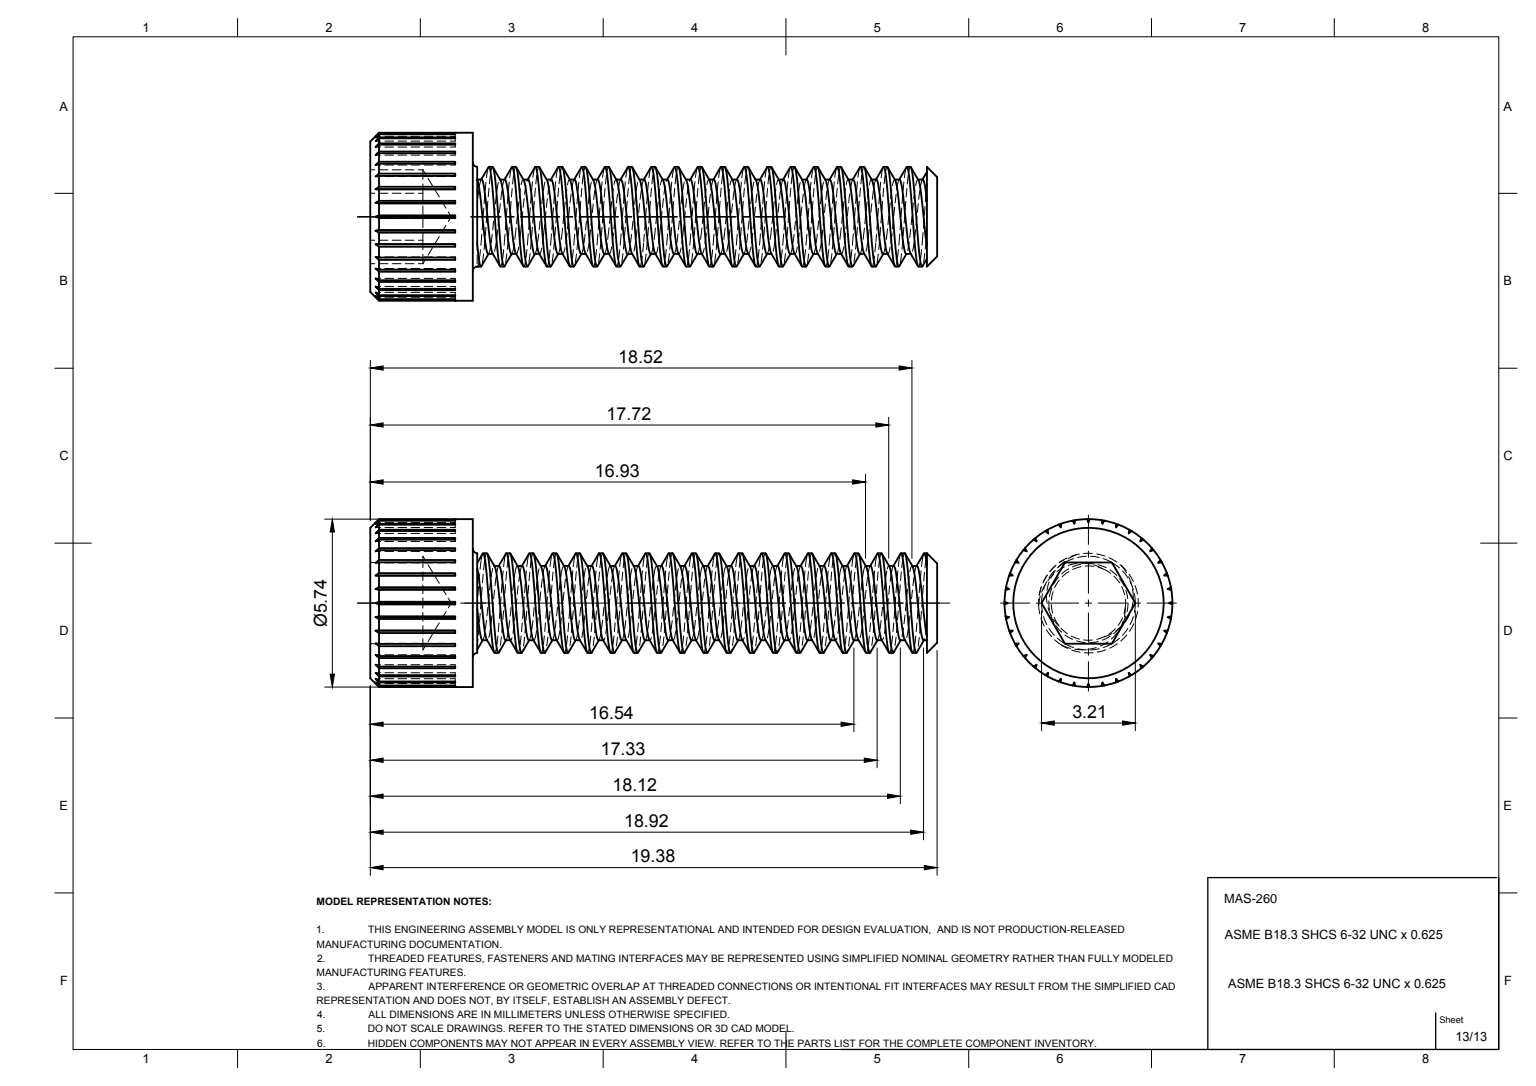
ISO-10303-21;
HEADER;
/* Generated by software containing ST-Developer
 * from STEP Tools, Inc. (www.steptools.com) 
 */

FILE_DESCRIPTION(
/* description */ (''),
/* implementation_level */ '2;1');

FILE_NAME(
/* name */ 'ASME B18.3 SHCS 6-32 UNC x 0.625.step',
/* time_stamp */ '2026-10-15T13:29:10-07:00',
/* author */ (''),
/* organization */ (''),
/* preprocessor_version */ 'ST-DEVELOPER v20.2',
/* originating_system */ 'Autodesk Translation Framework v15.15.0.0',
/* authorisation */ '');

FILE_SCHEMA (('AUTOMOTIVE_DESIGN { 1 0 10303 214 3 1 1 }'));
ENDSEC;

DATA;
#10=MECHANICAL_DESIGN_GEOMETRIC_PRESENTATION_REPRESENTATION('',(#944),#83219);
#425=(
BOUNDED_CURVE()
B_SPLINE_CURVE(2,(#82193,#82194,#82195),.UNSPECIFIED.,.F.,.F.)
B_SPLINE_CURVE_WITH_KNOTS((3,3),(0.,0.0169283274323949),.UNSPECIFIED.)
CURVE()
GEOMETRIC_REPRESENTATION_ITEM()
RATIONAL_B_SPLINE_CURVE((1.,1.00067437544385,1.00082963689528))
REPRESENTATION_ITEM('')
);
#426=(
BOUNDED_CURVE()
B_SPLINE_CURVE(2,(#82200,#82201,#82202),.UNSPECIFIED.,.F.,.F.)
B_SPLINE_CURVE_WITH_KNOTS((3,3),(0.027054491341878,0.0439828187741921),
 .UNSPECIFIED.)
CURVE()
GEOMETRIC_REPRESENTATION_ITEM()
RATIONAL_B_SPLINE_CURVE((1.00082963691689,1.00067437546141,1.))
REPRESENTATION_ITEM('')
);
#427=(
BOUNDED_CURVE()
B_SPLINE_CURVE(2,(#82209,#82210,#82211),.UNSPECIFIED.,.F.,.F.)
B_SPLINE_CURVE_WITH_KNOTS((3,3),(0.0270544913416899,0.0439828187741926),
 .UNSPECIFIED.)
CURVE()
GEOMETRIC_REPRESENTATION_ITEM()
RATIONAL_B_SPLINE_CURVE((1.00082963689398,1.0006743754428,1.))
REPRESENTATION_ITEM('')
);
#428=(
BOUNDED_CURVE()
B_SPLINE_CURVE(2,(#82215,#82216,#82217),.UNSPECIFIED.,.F.,.F.)
B_SPLINE_CURVE_WITH_KNOTS((3,3),(0.,0.016928327432378),.UNSPECIFIED.)
CURVE()
GEOMETRIC_REPRESENTATION_ITEM()
RATIONAL_B_SPLINE_CURVE((1.,1.00067437544454,1.00082963689613))
REPRESENTATION_ITEM('')
);
#429=(
BOUNDED_CURVE()
B_SPLINE_CURVE(2,(#82219,#82220,#82221),.UNSPECIFIED.,.F.,.F.)
B_SPLINE_CURVE_WITH_KNOTS((3,3),(0.0270544913417352,0.0439828187741927),
 .UNSPECIFIED.)
CURVE()
GEOMETRIC_REPRESENTATION_ITEM()
RATIONAL_B_SPLINE_CURVE((1.00082963690354,1.00067437545056,1.))
REPRESENTATION_ITEM('')
);
#430=(
BOUNDED_CURVE()
B_SPLINE_CURVE(2,(#82225,#82226,#82227),.UNSPECIFIED.,.F.,.F.)
B_SPLINE_CURVE_WITH_KNOTS((3,3),(0.,0.0169283274324875),.UNSPECIFIED.)
CURVE()
GEOMETRIC_REPRESENTATION_ITEM()
RATIONAL_B_SPLINE_CURVE((1.,1.00067437544421,1.00082963689573))
REPRESENTATION_ITEM('')
);
#431=(
BOUNDED_CURVE()
B_SPLINE_CURVE(2,(#82229,#82230,#82231),.UNSPECIFIED.,.F.,.F.)
B_SPLINE_CURVE_WITH_KNOTS((3,3),(0.0270544913417807,0.0439828187741914),
 .UNSPECIFIED.)
CURVE()
GEOMETRIC_REPRESENTATION_ITEM()
RATIONAL_B_SPLINE_CURVE((1.00082963690149,1.0006743754489,1.))
REPRESENTATION_ITEM('')
);
#432=(
BOUNDED_CURVE()
B_SPLINE_CURVE(2,(#82235,#82236,#82237),.UNSPECIFIED.,.F.,.F.)
B_SPLINE_CURVE_WITH_KNOTS((3,3),(0.,0.0169283274326477),.UNSPECIFIED.)
CURVE()
GEOMETRIC_REPRESENTATION_ITEM()
RATIONAL_B_SPLINE_CURVE((1.,1.00067437542316,1.00082963686982))
REPRESENTATION_ITEM('')
);
#433=(
BOUNDED_CURVE()
B_SPLINE_CURVE(2,(#82239,#82240,#82241),.UNSPECIFIED.,.F.,.F.)
B_SPLINE_CURVE_WITH_KNOTS((3,3),(0.0270544913419272,0.0439828187741907),
 .UNSPECIFIED.)
CURVE()
GEOMETRIC_REPRESENTATION_ITEM()
RATIONAL_B_SPLINE_CURVE((1.00082963692254,1.000674375466,1.))
REPRESENTATION_ITEM('')
);
#434=(
BOUNDED_CURVE()
B_SPLINE_CURVE(2,(#82245,#82246,#82247),.UNSPECIFIED.,.F.,.F.)
B_SPLINE_CURVE_WITH_KNOTS((3,3),(0.,0.0169283274324231),.UNSPECIFIED.)
CURVE()
GEOMETRIC_REPRESENTATION_ITEM()
RATIONAL_B_SPLINE_CURVE((1.,1.00067437544818,1.00082963690061))
REPRESENTATION_ITEM('')
);
#435=(
BOUNDED_CURVE()
B_SPLINE_CURVE(2,(#82249,#82250,#82251),.UNSPECIFIED.,.F.,.F.)
B_SPLINE_CURVE_WITH_KNOTS((3,3),(0.0270544913416623,0.0439828187741918),
 .UNSPECIFIED.)
CURVE()
GEOMETRIC_REPRESENTATION_ITEM()
RATIONAL_B_SPLINE_CURVE((1.00082963688688,1.00067437543703,1.))
REPRESENTATION_ITEM('')
);
#436=(
BOUNDED_CURVE()
B_SPLINE_CURVE(2,(#82255,#82256,#82257),.UNSPECIFIED.,.F.,.F.)
B_SPLINE_CURVE_WITH_KNOTS((3,3),(0.,0.016928327432524),.UNSPECIFIED.)
CURVE()
GEOMETRIC_REPRESENTATION_ITEM()
RATIONAL_B_SPLINE_CURVE((1.,1.00067437543311,1.00082963688207))
REPRESENTATION_ITEM('')
);
#437=(
BOUNDED_CURVE()
B_SPLINE_CURVE(2,(#82259,#82260,#82261),.UNSPECIFIED.,.F.,.F.)
B_SPLINE_CURVE_WITH_KNOTS((3,3),(0.0270544913417664,0.0439828187741907),
 .UNSPECIFIED.)
CURVE()
GEOMETRIC_REPRESENTATION_ITEM()
RATIONAL_B_SPLINE_CURVE((1.00082963689261,1.00067437544168,1.))
REPRESENTATION_ITEM('')
);
#438=(
BOUNDED_CURVE()
B_SPLINE_CURVE(2,(#82265,#82266,#82267),.UNSPECIFIED.,.F.,.F.)
B_SPLINE_CURVE_WITH_KNOTS((3,3),(0.,0.0169283274324059),.UNSPECIFIED.)
CURVE()
GEOMETRIC_REPRESENTATION_ITEM()
RATIONAL_B_SPLINE_CURVE((1.,1.00067437545304,1.00082963690658))
REPRESENTATION_ITEM('')
);
#439=(
BOUNDED_CURVE()
B_SPLINE_CURVE(2,(#82269,#82270,#82271),.UNSPECIFIED.,.F.,.F.)
B_SPLINE_CURVE_WITH_KNOTS((3,3),(0.0270544913417434,0.0439828187741902),
 .UNSPECIFIED.)
CURVE()
GEOMETRIC_REPRESENTATION_ITEM()
RATIONAL_B_SPLINE_CURVE((1.0008296368963,1.00067437544468,1.))
REPRESENTATION_ITEM('')
);
#440=(
BOUNDED_CURVE()
B_SPLINE_CURVE(2,(#82275,#82276,#82277),.UNSPECIFIED.,.F.,.F.)
B_SPLINE_CURVE_WITH_KNOTS((3,3),(0.,0.0169283274323925),.UNSPECIFIED.)
CURVE()
GEOMETRIC_REPRESENTATION_ITEM()
RATIONAL_B_SPLINE_CURVE((1.,1.00067437545304,1.00082963690659))
REPRESENTATION_ITEM('')
);
#441=(
BOUNDED_CURVE()
B_SPLINE_CURVE(2,(#82279,#82280,#82281),.UNSPECIFIED.,.F.,.F.)
B_SPLINE_CURVE_WITH_KNOTS((3,3),(0.0270544913417717,0.0439828187741908),
 .UNSPECIFIED.)
CURVE()
GEOMETRIC_REPRESENTATION_ITEM()
RATIONAL_B_SPLINE_CURVE((1.00082963689559,1.0006743754441,1.))
REPRESENTATION_ITEM('')
);
#442=(
BOUNDED_CURVE()
B_SPLINE_CURVE(2,(#82285,#82286,#82287),.UNSPECIFIED.,.F.,.F.)
B_SPLINE_CURVE_WITH_KNOTS((3,3),(0.,0.0169283274324336),.UNSPECIFIED.)
CURVE()
GEOMETRIC_REPRESENTATION_ITEM()
RATIONAL_B_SPLINE_CURVE((1.,1.00067437544179,1.00082963689274))
REPRESENTATION_ITEM('')
);
#443=(
BOUNDED_CURVE()
B_SPLINE_CURVE(2,(#82289,#82290,#82291),.UNSPECIFIED.,.F.,.F.)
B_SPLINE_CURVE_WITH_KNOTS((3,3),(0.0270544913417271,0.04398281877419),
 .UNSPECIFIED.)
CURVE()
GEOMETRIC_REPRESENTATION_ITEM()
RATIONAL_B_SPLINE_CURVE((1.00082963690167,1.00067437544904,1.))
REPRESENTATION_ITEM('')
);
#444=(
BOUNDED_CURVE()
B_SPLINE_CURVE(2,(#82295,#82296,#82297),.UNSPECIFIED.,.F.,.F.)
B_SPLINE_CURVE_WITH_KNOTS((3,3),(0.,0.0169283274323986),.UNSPECIFIED.)
CURVE()
GEOMETRIC_REPRESENTATION_ITEM()
RATIONAL_B_SPLINE_CURVE((1.,1.00067437544723,1.00082963689944))
REPRESENTATION_ITEM('')
);
#445=(
BOUNDED_CURVE()
B_SPLINE_CURVE(2,(#82299,#82300,#82301),.UNSPECIFIED.,.F.,.F.)
B_SPLINE_CURVE_WITH_KNOTS((3,3),(0.0270544913417658,0.0439828187741907),
 .UNSPECIFIED.)
CURVE()
GEOMETRIC_REPRESENTATION_ITEM()
RATIONAL_B_SPLINE_CURVE((1.00082963689458,1.00067437544328,1.))
REPRESENTATION_ITEM('')
);
#446=(
BOUNDED_CURVE()
B_SPLINE_CURVE(2,(#82305,#82306,#82307),.UNSPECIFIED.,.F.,.F.)
B_SPLINE_CURVE_WITH_KNOTS((3,3),(0.,0.0169283274323524),.UNSPECIFIED.)
CURVE()
GEOMETRIC_REPRESENTATION_ITEM()
RATIONAL_B_SPLINE_CURVE((1.,1.00067437545192,1.00082963690521))
REPRESENTATION_ITEM('')
);
#447=(
BOUNDED_CURVE()
B_SPLINE_CURVE(2,(#82309,#82310,#82311),.UNSPECIFIED.,.F.,.F.)
B_SPLINE_CURVE_WITH_KNOTS((3,3),(0.0270544913417437,0.0439828187741922),
 .UNSPECIFIED.)
CURVE()
GEOMETRIC_REPRESENTATION_ITEM()
RATIONAL_B_SPLINE_CURVE((1.0008296368979,1.00067437544598,1.))
REPRESENTATION_ITEM('')
);
#448=(
BOUNDED_CURVE()
B_SPLINE_CURVE(2,(#82315,#82316,#82317),.UNSPECIFIED.,.F.,.F.)
B_SPLINE_CURVE_WITH_KNOTS((3,3),(0.,0.0169283274322953),.UNSPECIFIED.)
CURVE()
GEOMETRIC_REPRESENTATION_ITEM()
RATIONAL_B_SPLINE_CURVE((1.,1.00067437546283,1.00082963691863))
REPRESENTATION_ITEM('')
);
#449=(
BOUNDED_CURVE()
B_SPLINE_CURVE(2,(#82319,#82320,#82321),.UNSPECIFIED.,.F.,.F.)
B_SPLINE_CURVE_WITH_KNOTS((3,3),(0.027054491341941,0.0439828187741898),
 .UNSPECIFIED.)
CURVE()
GEOMETRIC_REPRESENTATION_ITEM()
RATIONAL_B_SPLINE_CURVE((1.00082963692429,1.00067437546742,1.))
REPRESENTATION_ITEM('')
);
#450=(
BOUNDED_CURVE()
B_SPLINE_CURVE(2,(#82325,#82326,#82327),.UNSPECIFIED.,.F.,.F.)
B_SPLINE_CURVE_WITH_KNOTS((3,3),(0.,0.0169283274322328),.UNSPECIFIED.)
CURVE()
GEOMETRIC_REPRESENTATION_ITEM()
RATIONAL_B_SPLINE_CURVE((1.,1.00067437546617,1.00082963692274))
REPRESENTATION_ITEM('')
);
#451=(
BOUNDED_CURVE()
B_SPLINE_CURVE(2,(#82329,#82330,#82331),.UNSPECIFIED.,.F.,.F.)
B_SPLINE_CURVE_WITH_KNOTS((3,3),(0.0270544913418974,0.0439828187741896),
 .UNSPECIFIED.)
CURVE()
GEOMETRIC_REPRESENTATION_ITEM()
RATIONAL_B_SPLINE_CURVE((1.00082963691993,1.00067437546389,1.))
REPRESENTATION_ITEM('')
);
#452=(
BOUNDED_CURVE()
B_SPLINE_CURVE(2,(#82335,#82336,#82337),.UNSPECIFIED.,.F.,.F.)
B_SPLINE_CURVE_WITH_KNOTS((3,3),(0.,0.0169283274324175),.UNSPECIFIED.)
CURVE()
GEOMETRIC_REPRESENTATION_ITEM()
RATIONAL_B_SPLINE_CURVE((1.,1.00067437544813,1.00082963690054))
REPRESENTATION_ITEM('')
);
#453=(
BOUNDED_CURVE()
B_SPLINE_CURVE(2,(#82339,#82340,#82341),.UNSPECIFIED.,.F.,.F.)
B_SPLINE_CURVE_WITH_KNOTS((3,3),(0.0270544913419329,0.0439828187741885),
 .UNSPECIFIED.)
CURVE()
GEOMETRIC_REPRESENTATION_ITEM()
RATIONAL_B_SPLINE_CURVE((1.00082963691274,1.00067437545804,1.))
REPRESENTATION_ITEM('')
);
#454=(
BOUNDED_CURVE()
B_SPLINE_CURVE(2,(#82345,#82346,#82347),.UNSPECIFIED.,.F.,.F.)
B_SPLINE_CURVE_WITH_KNOTS((3,3),(0.,0.0169283274323868),.UNSPECIFIED.)
CURVE()
GEOMETRIC_REPRESENTATION_ITEM()
RATIONAL_B_SPLINE_CURVE((1.,1.00067437545154,1.00082963690474))
REPRESENTATION_ITEM('')
);
#455=(
BOUNDED_CURVE()
B_SPLINE_CURVE(2,(#82349,#82350,#82351),.UNSPECIFIED.,.F.,.F.)
B_SPLINE_CURVE_WITH_KNOTS((3,3),(0.0270544913418465,0.0439828187741911),
 .UNSPECIFIED.)
CURVE()
GEOMETRIC_REPRESENTATION_ITEM()
RATIONAL_B_SPLINE_CURVE((1.00082963692434,1.00067437546747,1.))
REPRESENTATION_ITEM('')
);
#456=(
BOUNDED_CURVE()
B_SPLINE_CURVE(2,(#82355,#82356,#82357),.UNSPECIFIED.,.F.,.F.)
B_SPLINE_CURVE_WITH_KNOTS((3,3),(0.,0.016928327432223),.UNSPECIFIED.)
CURVE()
GEOMETRIC_REPRESENTATION_ITEM()
RATIONAL_B_SPLINE_CURVE((1.,1.00067437546906,1.00082963692629))
REPRESENTATION_ITEM('')
);
#457=(
BOUNDED_CURVE()
B_SPLINE_CURVE(2,(#82359,#82360,#82361),.UNSPECIFIED.,.F.,.F.)
B_SPLINE_CURVE_WITH_KNOTS((3,3),(0.0270544913418792,0.0439828187741897),
 .UNSPECIFIED.)
CURVE()
GEOMETRIC_REPRESENTATION_ITEM()
RATIONAL_B_SPLINE_CURVE((1.0008296369223,1.00067437546581,1.))
REPRESENTATION_ITEM('')
);
#458=(
BOUNDED_CURVE()
B_SPLINE_CURVE(2,(#82365,#82366,#82367),.UNSPECIFIED.,.F.,.F.)
B_SPLINE_CURVE_WITH_KNOTS((3,3),(0.,0.0169283274325481),.UNSPECIFIED.)
CURVE()
GEOMETRIC_REPRESENTATION_ITEM()
RATIONAL_B_SPLINE_CURVE((1.,1.00067437544352,1.00082963689487))
REPRESENTATION_ITEM('')
);
#459=(
BOUNDED_CURVE()
B_SPLINE_CURVE(2,(#82369,#82370,#82371),.UNSPECIFIED.,.F.,.F.)
B_SPLINE_CURVE_WITH_KNOTS((3,3),(0.0270544913417793,0.0439828187741915),
 .UNSPECIFIED.)
CURVE()
GEOMETRIC_REPRESENTATION_ITEM()
RATIONAL_B_SPLINE_CURVE((1.00082963691087,1.00067437545653,1.))
REPRESENTATION_ITEM('')
);
#460=(
BOUNDED_CURVE()
B_SPLINE_CURVE(2,(#82375,#82376,#82377),.UNSPECIFIED.,.F.,.F.)
B_SPLINE_CURVE_WITH_KNOTS((3,3),(0.,0.0169283274323758),.UNSPECIFIED.)
CURVE()
GEOMETRIC_REPRESENTATION_ITEM()
RATIONAL_B_SPLINE_CURVE((1.,1.00067437544934,1.00082963690204))
REPRESENTATION_ITEM('')
);
#461=(
BOUNDED_CURVE()
B_SPLINE_CURVE(2,(#82379,#82380,#82381),.UNSPECIFIED.,.F.,.F.)
B_SPLINE_CURVE_WITH_KNOTS((3,3),(0.0270544913417685,0.0439828187741897),
 .UNSPECIFIED.)
CURVE()
GEOMETRIC_REPRESENTATION_ITEM()
RATIONAL_B_SPLINE_CURVE((1.00082963689898,1.00067437544686,1.))
REPRESENTATION_ITEM('')
);
#462=(
BOUNDED_CURVE()
B_SPLINE_CURVE(2,(#82385,#82386,#82387),.UNSPECIFIED.,.F.,.F.)
B_SPLINE_CURVE_WITH_KNOTS((3,3),(0.,0.0169283274324469),.UNSPECIFIED.)
CURVE()
GEOMETRIC_REPRESENTATION_ITEM()
RATIONAL_B_SPLINE_CURVE((1.,1.00067437544897,1.00082963690158))
REPRESENTATION_ITEM('')
);
#463=(
BOUNDED_CURVE()
B_SPLINE_CURVE(2,(#82389,#82390,#82391),.UNSPECIFIED.,.F.,.F.)
B_SPLINE_CURVE_WITH_KNOTS((3,3),(0.0270544913418427,0.04398281877419),
 .UNSPECIFIED.)
CURVE()
GEOMETRIC_REPRESENTATION_ITEM()
RATIONAL_B_SPLINE_CURVE((1.00082963692428,1.00067437546742,1.))
REPRESENTATION_ITEM('')
);
#464=(
BOUNDED_CURVE()
B_SPLINE_CURVE(2,(#82396,#82397,#82398),.UNSPECIFIED.,.F.,.F.)
B_SPLINE_CURVE_WITH_KNOTS((3,3),(0.,0.0169283274326309),.UNSPECIFIED.)
CURVE()
GEOMETRIC_REPRESENTATION_ITEM()
RATIONAL_B_SPLINE_CURVE((1.,1.00067437542865,1.00082963687657))
REPRESENTATION_ITEM('')
);
#465=(
BOUNDED_CURVE()
B_SPLINE_CURVE(2,(#82400,#82401,#82402),.UNSPECIFIED.,.F.,.F.)
B_SPLINE_CURVE_WITH_KNOTS((3,3),(0.0270544913417494,0.0439828187741933),
 .UNSPECIFIED.)
CURVE()
GEOMETRIC_REPRESENTATION_ITEM()
RATIONAL_B_SPLINE_CURVE((1.00082963689727,1.00067437544547,1.))
REPRESENTATION_ITEM('')
);
#466=(
BOUNDED_CURVE()
B_SPLINE_CURVE(2,(#82406,#82407,#82408),.UNSPECIFIED.,.F.,.F.)
B_SPLINE_CURVE_WITH_KNOTS((3,3),(0.,0.0169283274321813),.UNSPECIFIED.)
CURVE()
GEOMETRIC_REPRESENTATION_ITEM()
RATIONAL_B_SPLINE_CURVE((1.,1.00067437546612,1.00082963692269))
REPRESENTATION_ITEM('')
);
#467=(
BOUNDED_CURVE()
B_SPLINE_CURVE(2,(#82410,#82411,#82412),.UNSPECIFIED.,.F.,.F.)
B_SPLINE_CURVE_WITH_KNOTS((3,3),(0.0270544913418634,0.0439828187741926),
 .UNSPECIFIED.)
CURVE()
GEOMETRIC_REPRESENTATION_ITEM()
RATIONAL_B_SPLINE_CURVE((1.00082963691427,1.00067437545928,1.))
REPRESENTATION_ITEM('')
);
#468=(
BOUNDED_CURVE()
B_SPLINE_CURVE(2,(#82416,#82417,#82418),.UNSPECIFIED.,.F.,.F.)
B_SPLINE_CURVE_WITH_KNOTS((3,3),(0.,0.0169283274324664),.UNSPECIFIED.)
CURVE()
GEOMETRIC_REPRESENTATION_ITEM()
RATIONAL_B_SPLINE_CURVE((1.,1.00067437544028,1.00082963689088))
REPRESENTATION_ITEM('')
);
#469=(
BOUNDED_CURVE()
B_SPLINE_CURVE(2,(#82420,#82421,#82422),.UNSPECIFIED.,.F.,.F.)
B_SPLINE_CURVE_WITH_KNOTS((3,3),(0.0270544913418777,0.0439828187741926),
 .UNSPECIFIED.)
CURVE()
GEOMETRIC_REPRESENTATION_ITEM()
RATIONAL_B_SPLINE_CURVE((1.00082963691853,1.00067437546274,1.))
REPRESENTATION_ITEM('')
);
#470=(
BOUNDED_CURVE()
B_SPLINE_CURVE(2,(#82426,#82427,#82428),.UNSPECIFIED.,.F.,.F.)
B_SPLINE_CURVE_WITH_KNOTS((3,3),(0.,0.0169283274323108),.UNSPECIFIED.)
CURVE()
GEOMETRIC_REPRESENTATION_ITEM()
RATIONAL_B_SPLINE_CURVE((1.,1.00067437545943,1.00082963691444))
REPRESENTATION_ITEM('')
);
#471=(
BOUNDED_CURVE()
B_SPLINE_CURVE(2,(#82430,#82431,#82432),.UNSPECIFIED.,.F.,.F.)
B_SPLINE_CURVE_WITH_KNOTS((3,3),(0.0270544913417395,0.0439828187741916),
 .UNSPECIFIED.)
CURVE()
GEOMETRIC_REPRESENTATION_ITEM()
RATIONAL_B_SPLINE_CURVE((1.00082963689027,1.00067437543978,1.))
REPRESENTATION_ITEM('')
);
#472=(
BOUNDED_CURVE()
B_SPLINE_CURVE(2,(#82436,#82437,#82438),.UNSPECIFIED.,.F.,.F.)
B_SPLINE_CURVE_WITH_KNOTS((3,3),(0.,0.0169283274323638),.UNSPECIFIED.)
CURVE()
GEOMETRIC_REPRESENTATION_ITEM()
RATIONAL_B_SPLINE_CURVE((1.,1.00067437545187,1.00082963690515))
REPRESENTATION_ITEM('')
);
#473=(
BOUNDED_CURVE()
B_SPLINE_CURVE(2,(#82440,#82441,#82442),.UNSPECIFIED.,.F.,.F.)
B_SPLINE_CURVE_WITH_KNOTS((3,3),(0.0270544913417076,0.0439828187741916),
 .UNSPECIFIED.)
CURVE()
GEOMETRIC_REPRESENTATION_ITEM()
RATIONAL_B_SPLINE_CURVE((1.00082963689143,1.00067437544072,1.))
REPRESENTATION_ITEM('')
);
#474=(
BOUNDED_CURVE()
B_SPLINE_CURVE(2,(#82446,#82447,#82448),.UNSPECIFIED.,.F.,.F.)
B_SPLINE_CURVE_WITH_KNOTS((3,3),(0.,0.0169283274324132),.UNSPECIFIED.)
CURVE()
GEOMETRIC_REPRESENTATION_ITEM()
RATIONAL_B_SPLINE_CURVE((1.,1.00067437545166,1.00082963690489))
REPRESENTATION_ITEM('')
);
#475=(
BOUNDED_CURVE()
B_SPLINE_CURVE(2,(#82450,#82451,#82452),.UNSPECIFIED.,.F.,.F.)
B_SPLINE_CURVE_WITH_KNOTS((3,3),(0.0270544913417581,0.0439828187741926),
 .UNSPECIFIED.)
CURVE()
GEOMETRIC_REPRESENTATION_ITEM()
RATIONAL_B_SPLINE_CURVE((1.00082963689712,1.00067437544534,1.))
REPRESENTATION_ITEM('')
);
#476=(
BOUNDED_CURVE()
B_SPLINE_CURVE(2,(#82456,#82457,#82458),.UNSPECIFIED.,.F.,.F.)
B_SPLINE_CURVE_WITH_KNOTS((3,3),(0.,0.0169283274323258),.UNSPECIFIED.)
CURVE()
GEOMETRIC_REPRESENTATION_ITEM()
RATIONAL_B_SPLINE_CURVE((1.,1.00067437545421,1.00082963690803))
REPRESENTATION_ITEM('')
);
#477=(
BOUNDED_CURVE()
B_SPLINE_CURVE(2,(#82460,#82461,#82462),.UNSPECIFIED.,.F.,.F.)
B_SPLINE_CURVE_WITH_KNOTS((3,3),(0.0270544913417721,0.0439828187741926),
 .UNSPECIFIED.)
CURVE()
GEOMETRIC_REPRESENTATION_ITEM()
RATIONAL_B_SPLINE_CURVE((1.00082963689922,1.00067437544705,1.))
REPRESENTATION_ITEM('')
);
#478=(
BOUNDED_CURVE()
B_SPLINE_CURVE(2,(#82466,#82467,#82468),.UNSPECIFIED.,.F.,.F.)
B_SPLINE_CURVE_WITH_KNOTS((3,3),(0.,0.0169283274323368),.UNSPECIFIED.)
CURVE()
GEOMETRIC_REPRESENTATION_ITEM()
RATIONAL_B_SPLINE_CURVE((1.,1.00067437545165,1.00082963690488))
REPRESENTATION_ITEM('')
);
#479=(
BOUNDED_CURVE()
B_SPLINE_CURVE(2,(#82470,#82471,#82472),.UNSPECIFIED.,.F.,.F.)
B_SPLINE_CURVE_WITH_KNOTS((3,3),(0.0270544913418129,0.0439828187741918),
 .UNSPECIFIED.)
CURVE()
GEOMETRIC_REPRESENTATION_ITEM()
RATIONAL_B_SPLINE_CURVE((1.00082963690488,1.00067437545165,1.))
REPRESENTATION_ITEM('')
);
#480=(
BOUNDED_CURVE()
B_SPLINE_CURVE(2,(#82476,#82477,#82478),.UNSPECIFIED.,.F.,.F.)
B_SPLINE_CURVE_WITH_KNOTS((3,3),(0.,0.0169283274323829),.UNSPECIFIED.)
CURVE()
GEOMETRIC_REPRESENTATION_ITEM()
RATIONAL_B_SPLINE_CURVE((1.,1.00067437545407,1.00082963690785))
REPRESENTATION_ITEM('')
);
#481=(
BOUNDED_CURVE()
B_SPLINE_CURVE(2,(#82480,#82481,#82482),.UNSPECIFIED.,.F.,.F.)
B_SPLINE_CURVE_WITH_KNOTS((3,3),(0.0270544913418384,0.0439828187741921),
 .UNSPECIFIED.)
CURVE()
GEOMETRIC_REPRESENTATION_ITEM()
RATIONAL_B_SPLINE_CURVE((1.00082963690821,1.00067437545436,1.))
REPRESENTATION_ITEM('')
);
#482=(
BOUNDED_CURVE()
B_SPLINE_CURVE(2,(#82486,#82487,#82488),.UNSPECIFIED.,.F.,.F.)
B_SPLINE_CURVE_WITH_KNOTS((3,3),(0.,0.0169283274323058),.UNSPECIFIED.)
CURVE()
GEOMETRIC_REPRESENTATION_ITEM()
RATIONAL_B_SPLINE_CURVE((1.,1.00067437546416,1.00082963692027))
REPRESENTATION_ITEM('')
);
#483=(
BOUNDED_CURVE()
B_SPLINE_CURVE(2,(#82490,#82491,#82492),.UNSPECIFIED.,.F.,.F.)
B_SPLINE_CURVE_WITH_KNOTS((3,3),(0.0270544913418702,0.0439828187741907),
 .UNSPECIFIED.)
CURVE()
GEOMETRIC_REPRESENTATION_ITEM()
RATIONAL_B_SPLINE_CURVE((1.00082963692018,1.00067437546409,1.))
REPRESENTATION_ITEM('')
);
#484=(
BOUNDED_CURVE()
B_SPLINE_CURVE(2,(#82496,#82497,#82498),.UNSPECIFIED.,.F.,.F.)
B_SPLINE_CURVE_WITH_KNOTS((3,3),(0.,0.0169283274324372),.UNSPECIFIED.)
CURVE()
GEOMETRIC_REPRESENTATION_ITEM()
RATIONAL_B_SPLINE_CURVE((1.,1.00067437545102,1.0008296369041))
REPRESENTATION_ITEM('')
);
#485=(
BOUNDED_CURVE()
B_SPLINE_CURVE(2,(#82500,#82501,#82502),.UNSPECIFIED.,.F.,.F.)
B_SPLINE_CURVE_WITH_KNOTS((3,3),(0.0270544913418863,0.0439828187741916),
 .UNSPECIFIED.)
CURVE()
GEOMETRIC_REPRESENTATION_ITEM()
RATIONAL_B_SPLINE_CURVE((1.00082963691192,1.00067437545738,1.))
REPRESENTATION_ITEM('')
);
#486=(
BOUNDED_CURVE()
B_SPLINE_CURVE(2,(#82506,#82507,#82508),.UNSPECIFIED.,.F.,.F.)
B_SPLINE_CURVE_WITH_KNOTS((3,3),(0.,0.0169283274323833),.UNSPECIFIED.)
CURVE()
GEOMETRIC_REPRESENTATION_ITEM()
RATIONAL_B_SPLINE_CURVE((1.,1.00067437544615,1.00082963689811))
REPRESENTATION_ITEM('')
);
#487=(
BOUNDED_CURVE()
B_SPLINE_CURVE(2,(#82510,#82511,#82512),.UNSPECIFIED.,.F.,.F.)
B_SPLINE_CURVE_WITH_KNOTS((3,3),(0.0270544913417211,0.0439828187741927),
 .UNSPECIFIED.)
CURVE()
GEOMETRIC_REPRESENTATION_ITEM()
RATIONAL_B_SPLINE_CURVE((1.00082963690189,1.00067437544923,1.))
REPRESENTATION_ITEM('')
);
#488=(
BOUNDED_CURVE()
B_SPLINE_CURVE(2,(#82516,#82517,#82518),.UNSPECIFIED.,.F.,.F.)
B_SPLINE_CURVE_WITH_KNOTS((3,3),(0.,0.0169283274324049),.UNSPECIFIED.)
CURVE()
GEOMETRIC_REPRESENTATION_ITEM()
RATIONAL_B_SPLINE_CURVE((1.,1.00067437545222,1.00082963690557))
REPRESENTATION_ITEM('')
);
#489=(
BOUNDED_CURVE()
B_SPLINE_CURVE(2,(#82520,#82521,#82522),.UNSPECIFIED.,.F.,.F.)
B_SPLINE_CURVE_WITH_KNOTS((3,3),(0.0270544913418404,0.0439828187741917),
 .UNSPECIFIED.)
CURVE()
GEOMETRIC_REPRESENTATION_ITEM()
RATIONAL_B_SPLINE_CURVE((1.00082963691628,1.00067437546092,1.))
REPRESENTATION_ITEM('')
);
#490=(
BOUNDED_CURVE()
B_SPLINE_CURVE(2,(#82526,#82527,#82528),.UNSPECIFIED.,.F.,.F.)
B_SPLINE_CURVE_WITH_KNOTS((3,3),(0.,0.016928327432346),.UNSPECIFIED.)
CURVE()
GEOMETRIC_REPRESENTATION_ITEM()
RATIONAL_B_SPLINE_CURVE((1.,1.00067437545423,1.00082963690805))
REPRESENTATION_ITEM('')
);
#491=(
BOUNDED_CURVE()
B_SPLINE_CURVE(2,(#82530,#82531,#82532),.UNSPECIFIED.,.F.,.F.)
B_SPLINE_CURVE_WITH_KNOTS((3,3),(0.0270544913418446,0.0439828187741916),
 .UNSPECIFIED.)
CURVE()
GEOMETRIC_REPRESENTATION_ITEM()
RATIONAL_B_SPLINE_CURVE((1.00082963690992,1.00067437545575,1.))
REPRESENTATION_ITEM('')
);
#492=(
BOUNDED_CURVE()
B_SPLINE_CURVE(2,(#82536,#82537,#82538),.UNSPECIFIED.,.F.,.F.)
B_SPLINE_CURVE_WITH_KNOTS((3,3),(0.,0.0169283274324851),.UNSPECIFIED.)
CURVE()
GEOMETRIC_REPRESENTATION_ITEM()
RATIONAL_B_SPLINE_CURVE((1.,1.00067437545061,1.00082963690359))
REPRESENTATION_ITEM('')
);
#493=(
BOUNDED_CURVE()
B_SPLINE_CURVE(2,(#82540,#82541,#82542),.UNSPECIFIED.,.F.,.F.)
B_SPLINE_CURVE_WITH_KNOTS((3,3),(0.0270544913417195,0.0439828187741921),
 .UNSPECIFIED.)
CURVE()
GEOMETRIC_REPRESENTATION_ITEM()
RATIONAL_B_SPLINE_CURVE((1.00082963689352,1.00067437544242,1.))
REPRESENTATION_ITEM('')
);
#494=(
BOUNDED_CURVE()
B_SPLINE_CURVE(2,(#82546,#82547,#82548),.UNSPECIFIED.,.F.,.F.)
B_SPLINE_CURVE_WITH_KNOTS((3,3),(0.,0.0169283274324387),.UNSPECIFIED.)
CURVE()
GEOMETRIC_REPRESENTATION_ITEM()
RATIONAL_B_SPLINE_CURVE((1.,1.00067437545353,1.00082963690719))
REPRESENTATION_ITEM('')
);
#495=(
BOUNDED_CURVE()
B_SPLINE_CURVE(2,(#82550,#82551,#82552),.UNSPECIFIED.,.F.,.F.)
B_SPLINE_CURVE_WITH_KNOTS((3,3),(0.0270544913416745,0.0439828187741916),
 .UNSPECIFIED.)
CURVE()
GEOMETRIC_REPRESENTATION_ITEM()
RATIONAL_B_SPLINE_CURVE((1.00082963688426,1.00067437543489,1.))
REPRESENTATION_ITEM('')
);
#496=(
BOUNDED_CURVE()
B_SPLINE_CURVE(2,(#82555,#82556,#82557),.UNSPECIFIED.,.F.,.F.)
B_SPLINE_CURVE_WITH_KNOTS((3,3),(0.,0.0169283274326045),.UNSPECIFIED.)
CURVE()
GEOMETRIC_REPRESENTATION_ITEM()
RATIONAL_B_SPLINE_CURVE((1.,1.0006743754289,1.00082963687688))
REPRESENTATION_ITEM('')
);
#507=TOROIDAL_SURFACE('',#28959,1.85434,0.15);
#754=B_SPLINE_CURVE_WITH_KNOTS('',3,(#66842,#66843,#66844,#66845,#66846,
#66847,#66848,#66849,#66850,#66851,#66852,#66853,#66854,#66855,#66856,#66857,
#66858,#66859,#66860,#66861,#66862,#66863,#66864,#66865,#66866,#66867,#66868,
#66869,#66870,#66871,#66872,#66873,#66874,#66875,#66876,#66877,#66878,#66879,
#66880,#66881,#66882,#66883,#66884,#66885,#66886,#66887,#66888,#66889,#66890,
#66891,#66892,#66893,#66894,#66895,#66896,#66897,#66898,#66899,#66900,#66901,
#66902,#66903,#66904,#66905,#66906,#66907,#66908,#66909,#66910,#66911,#66912,
#66913,#66914,#66915,#66916,#66917,#66918,#66919,#66920,#66921,#66922,#66923,
#66924,#66925,#66926,#66927,#66928,#66929,#66930,#66931,#66932,#66933,#66934,
#66935,#66936,#66937,#66938,#66939,#66940,#66941,#66942,#66943,#66944,#66945,
#66946,#66947,#66948,#66949,#66950,#66951,#66952,#66953,#66954,#66955,#66956,
#66957,#66958,#66959,#66960,#66961,#66962,#66963,#66964,#66965,#66966,#66967,
#66968,#66969,#66970,#66971,#66972,#66973,#66974,#66975,#66976,#66977,#66978,
#66979,#66980,#66981,#66982,#66983,#66984,#66985,#66986,#66987,#66988,#66989,
#66990,#66991),.UNSPECIFIED.,.F.,.F.,(4,2,2,2,2,2,2,2,2,2,2,2,2,2,2,2,2,
2,2,2,2,2,2,2,2,2,2,2,2,2,2,2,2,2,2,2,2,2,2,2,2,2,2,2,2,2,2,2,2,2,2,2,2,
2,2,2,2,2,2,2,2,2,2,2,2,2,2,2,2,2,2,2,2,2,4),(-0.57814561136758,-0.576296413092534,
-0.573641255529324,-0.570575982215014,-0.565100054282956,-0.539917695991999,
-0.517394447378374,-0.513602331908594,-0.511741570723418,-0.510242310430281,
-0.508340948528616,-0.504346832441546,-0.498825097755031,-0.482729724369596,
-0.457683189040658,-0.452468380911234,-0.449158815326736,-0.44649911229893,
-0.443438658618413,-0.437998831205895,-0.420540876202223,-0.396348568164452,
-0.388039555375418,-0.385470635862254,-0.383865857222333,-0.382305956175603,
-0.379915741966088,-0.372455557398866,-0.358639298966442,-0.329684380929608,
-0.324675436110595,-0.321438891082664,-0.31880269342991,-0.315730719856977,
-0.310163725739934,-0.291420708773143,-0.262555131157506,-0.258796386401061,
-0.256948163636404,-0.25545280771485,-0.253551211796978,-0.249556076524077,
-0.244035210720099,-0.227979871153349,-0.202571226003975,-0.197332498520712,
-0.194009001551785,-0.191338924841252,-0.188267212494532,-0.182807842087583,
-0.165030475351221,-0.139231601339638,-0.132653249078248,-0.130320744596009,
-0.1288153480515,-0.127227747985358,-0.124700541689401,-0.116313972219858,
-0.0993334415849082,-0.0765628114683407,-0.0713569283432376,-0.0680324326380281,
-0.0653451663167553,-0.0622341911963431,-0.0566479026914896,-0.0370860220512205,
-0.017582256991236,-0.0174599552727001,-0.0173504481393084,-0.0172524828413307,
-0.0117389265183658,-0.00594267422071392,-0.00373663500168019,-0.00222440479797267,
-0.00170432960837967),.UNSPECIFIED.);
#755=B_SPLINE_CURVE_WITH_KNOTS('',3,(#66994,#66995,#66996,#66997,#66998,
#66999,#67000,#67001,#67002,#67003,#67004,#67005,#67006,#67007,#67008,#67009,
#67010,#67011,#67012,#67013,#67014,#67015,#67016,#67017,#67018,#67019,#67020,
#67021,#67022,#67023,#67024,#67025,#67026,#67027,#67028,#67029,#67030,#67031,
#67032,#67033,#67034,#67035,#67036,#67037,#67038,#67039,#67040,#67041,#67042,
#67043,#67044,#67045,#67046,#67047,#67048,#67049,#67050,#67051,#67052,#67053,
#67054,#67055,#67056,#67057,#67058,#67059,#67060,#67061,#67062,#67063,#67064,
#67065,#67066,#67067,#67068,#67069,#67070,#67071,#67072,#67073,#67074,#67075,
#67076,#67077,#67078,#67079,#67080,#67081,#67082,#67083,#67084,#67085,#67086,
#67087,#67088,#67089,#67090,#67091,#67092,#67093,#67094,#67095),
 .UNSPECIFIED.,.F.,.F.,(4,2,2,2,2,2,2,2,2,2,2,2,2,2,2,2,2,2,2,2,2,2,2,2,
2,2,2,2,2,2,2,2,2,2,2,2,2,2,2,2,2,2,2,2,2,2,2,2,2,2,4),(-1.318649661076,
-1.31743164617652,-1.31596386436676,-1.31264394085227,-1.29594709662516,
-1.28122934432088,-1.26838464214962,-1.26496788072465,-1.26168833677219,
-1.25870792832702,-1.25486579200619,-1.24618731091111,-1.21648393904188,
-1.20318656193115,-1.19816844726018,-1.19454224790336,-1.19301372216914,
-1.19149228574573,-1.1898443744577,-1.18691776961928,-1.17008318442145,
-1.14747114229976,-1.1394250167213,-1.13330473980141,-1.13019933198268,
-1.12766982200797,-1.12472587504508,-1.11956287795595,-1.08684999296772,
-1.0740249365971,-1.0669291365151,-1.06464970615256,-1.0631437366511,-1.06174272516908,
-1.05978387397002,-1.05448060749719,-1.02076562574725,-1.00652926771878,
-1.00219769891924,-0.999348512279982,-0.996615935546906,-0.992744443746673,
-0.983330401145941,-0.952120651371644,-0.941214068805748,-0.938480088912673,
-0.936816205379131,-0.935259751531581,-0.932908357310751,-0.926522568567024,
-0.912197827138135),.UNSPECIFIED.);
#756=B_SPLINE_CURVE_WITH_KNOTS('',3,(#67100,#67101,#67102,#67103,#67104,
#67105,#67106,#67107,#67108,#67109,#67110,#67111,#67112,#67113,#67114,#67115,
#67116,#67117,#67118,#67119,#67120,#67121,#67122,#67123,#67124,#67125,#67126,
#67127,#67128,#67129,#67130,#67131,#67132,#67133,#67134,#67135,#67136,#67137,
#67138,#67139,#67140,#67141,#67142,#67143,#67144,#67145,#67146,#67147,#67148,
#67149,#67150,#67151,#67152,#67153,#67154,#67155,#67156,#67157,#67158,#67159,
#67160,#67161,#67162,#67163,#67164,#67165,#67166,#67167,#67168,#67169,#67170,
#67171,#67172,#67173,#67174,#67175,#67176,#67177,#67178,#67179,#67180,#67181,
#67182,#67183,#67184,#67185,#67186,#67187,#67188,#67189,#67190,#67191,#67192,
#67193,#67194,#67195,#67196,#67197,#67198,#67199,#67200,#67201,#67202,#67203,
#67204,#67205,#67206,#67207,#67208,#67209,#67210,#67211,#67212,#67213,#67214,
#67215,#67216,#67217,#67218,#67219,#67220,#67221,#67222,#67223,#67224,#67225,
#67226,#67227,#67228,#67229,#67230,#67231,#67232,#67233,#67234,#67235,#67236,
#67237,#67238,#67239,#67240,#67241,#67242,#67243,#67244,#67245,#67246,#67247,
#67248,#67249,#67250,#67251,#67252,#67253,#67254,#67255,#67256,#67257,#67258,
#67259,#67260,#67261,#67262,#67263,#67264,#67265,#67266,#67267,#67268,#67269,
#67270,#67271,#67272,#67273,#67274,#67275,#67276,#67277,#67278,#67279,#67280,
#67281,#67282,#67283,#67284,#67285,#67286,#67287,#67288,#67289,#67290,#67291,
#67292,#67293,#67294,#67295,#67296,#67297,#67298,#67299,#67300,#67301,#67302,
#67303,#67304,#67305,#67306,#67307,#67308,#67309,#67310,#67311),
 .UNSPECIFIED.,.F.,.F.,(4,2,2,2,2,2,2,2,2,2,2,2,2,2,2,2,2,2,2,2,2,2,2,2,
2,2,2,2,2,2,2,2,2,2,2,2,2,2,2,2,2,2,2,2,2,2,2,2,2,2,2,2,2,2,2,2,2,2,2,2,
2,2,2,2,2,2,2,2,2,2,2,2,2,2,2,2,2,2,2,2,2,2,2,2,2,2,2,2,2,2,2,2,2,2,2,2,
2,2,2,2,2,2,2,2,2,4),(-1.38023582942697,-1.36727393991216,-1.35371560626455,
-1.34758612233084,-1.343921800107,-1.34061316589332,-1.34053112229902,-1.34043931642608,
-1.3403365203079,-1.34022134355601,-1.34016271070482,-1.34005242700723,
-1.3398468093432,-1.33815809251505,-1.3352377643514,-1.33045180817441,-1.30897662302457,
-1.29157501945926,-1.28356639925018,-1.27834115990851,-1.27623369214961,
-1.27471833837372,-1.2730058302725,-1.27001812086406,-1.25111770200688,
-1.23630570255573,-1.22495364593259,-1.21701636660591,-1.2134933524464,
-1.21081513541201,-1.20788795402808,-1.20306977280792,-1.18130948763523,
-1.16531976172926,-1.15249883204994,-1.14968381557519,-1.14802568515435,
-1.14650719484141,-1.14428686846135,-1.13870173312281,-1.11507890758532,
-1.09356250686361,-1.0881856924398,-1.08514186799305,-1.08248619566579,
-1.07916826209924,-1.07391367594643,-1.05284974270858,-1.03360977196564,
-1.02908537693002,-1.02372351079304,-1.02159526136499,-1.02007689873916,
-1.01837468805536,-1.01535478228218,-0.996529384285813,-0.981837080157525,
-0.970362461890046,-0.962365079993149,-0.958832057740846,-0.956152418464221,
-0.953229721601869,-0.948433077774452,-0.926850209827973,-0.909849783859956,
-0.897749210878761,-0.894973132600081,-0.89332330855354,-0.891799870665586,
-0.889554584404612,-0.883818167363212,-0.860336468657881,-0.838906369534903,
-0.833529741113932,-0.830485237382186,-0.827828474640885,-0.82450847685547,
-0.819249072614846,-0.796357484571786,-0.774587966790706,-0.769099095389485,
-0.766951592457606,-0.765430332989124,-0.763738186037086,-0.760761742328727,
-0.745207332653177,-0.712064927175208,-0.706929528343931,-0.703647324266641,
-0.70099576924898,-0.697929682490364,-0.692438811248146,-0.688696612541937,
-0.677483780053588,-0.66254578946903,-0.644895009679777,-0.641016489589638,
-0.639141075648444,-0.6376458447114,-0.635770121516414,-0.63189410665383,
-0.626587603279061,-0.611607150850109,-0.584751885349557,-0.579588767808115,
-0.57814561136758),.UNSPECIFIED.);
#757=B_SPLINE_CURVE_WITH_KNOTS('',3,(#67312,#67313,#67314,#67315,#67316,
#67317,#67318,#67319,#67320,#67321,#67322,#67323,#67324,#67325,#67326,#67327,
#67328,#67329,#67330,#67331,#67332,#67333,#67334,#67335,#67336,#67337,#67338,
#67339,#67340,#67341,#67342,#67343,#67344,#67345,#67346,#67347,#67348,#67349,
#67350,#67351,#67352,#67353,#67354,#67355,#67356,#67357,#67358,#67359,#67360,
#67361,#67362,#67363,#67364,#67365,#67366,#67367,#67368,#67369,#67370,#67371,
#67372,#67373,#67374,#67375,#67376,#67377,#67378,#67379,#67380,#67381,#67382,
#67383,#67384,#67385,#67386,#67387,#67388,#67389,#67390,#67391,#67392,#67393,
#67394,#67395,#67396,#67397,#67398,#67399,#67400,#67401,#67402,#67403,#67404,
#67405,#67406,#67407,#67408,#67409,#67410,#67411,#67412,#67413,#67414,#67415,
#67416,#67417,#67418,#67419,#67420,#67421,#67422,#67423,#67424,#67425,#67426,
#67427,#67428,#67429,#67430,#67431,#67432,#67433,#67434,#67435,#67436,#67437,
#67438,#67439,#67440,#67441,#67442,#67443,#67444,#67445,#67446,#67447,#67448,
#67449,#67450,#67451,#67452,#67453,#67454,#67455,#67456,#67457,#67458,#67459,
#67460,#67461,#67462,#67463,#67464,#67465,#67466,#67467,#67468,#67469,#67470,
#67471,#67472,#67473,#67474,#67475,#67476,#67477,#67478,#67479,#67480,#67481,
#67482,#67483,#67484,#67485,#67486,#67487,#67488,#67489,#67490,#67491,#67492,
#67493,#67494,#67495,#67496,#67497,#67498,#67499,#67500,#67501,#67502,#67503,
#67504,#67505,#67506,#67507,#67508,#67509,#67510,#67511,#67512,#67513),
 .UNSPECIFIED.,.F.,.F.,(4,2,2,2,2,2,2,2,2,2,2,2,2,2,2,2,2,2,2,2,2,2,2,2,
2,2,2,2,2,2,2,2,2,2,2,2,2,2,2,2,2,2,2,2,2,2,2,2,2,2,2,2,2,2,2,2,2,2,2,2,
2,2,2,2,2,2,2,2,2,2,2,2,2,2,2,2,2,2,2,2,2,2,2,2,2,2,2,2,2,2,2,2,2,2,2,2,
2,2,2,2,4),(-0.912197827138135,-0.900546199742846,-0.882740080166755,-0.877276848729105,
-0.87420458867794,-0.871534938336999,-0.868213171824111,-0.862979623827371,
-0.837294669421898,-0.821399737697169,-0.813292325056683,-0.810819299780855,
-0.80923232690993,-0.807836500252428,-0.805894466986116,-0.800715257100852,
-0.776732509135995,-0.761472510343384,-0.754898003265771,-0.749603032302451,
-0.746587085452515,-0.743945875155078,-0.740633716807298,-0.73536514512806,
-0.714333990831212,-0.694904842353685,-0.690355086583755,-0.684978663816953,
-0.682856691221549,-0.681344773564849,-0.679647540897774,-0.676651654041828,
-0.659567615862423,-0.630502651288208,-0.623210744390032,-0.619794566198917,
-0.617125366538986,-0.614134142471098,-0.609026791915333,-0.602763321734904,
-0.588717224411485,-0.567800480516633,-0.558812807840408,-0.556173769635394,
-0.554550706351212,-0.552988099678455,-0.550623966689748,-0.543493671585025,
-0.521319091753183,-0.499125206562843,-0.494346049589137,-0.491426211160512,
-0.488744113011381,-0.485200319950247,-0.477143785509341,-0.465548377900303,
-0.450939542629863,-0.432147184684293,-0.429128115647081,-0.427425965017967,
-0.425908121779637,-0.423780793358204,-0.418420538617579,-0.413897923689911,
-0.394664734957041,-0.373611549271333,-0.368362614572839,-0.36504734986907,
-0.362393387126308,-0.359351140731567,-0.353976464165174,-0.350340390713623,
-0.344436566516383,-0.321981988903486,-0.30472263868096,-0.301726802314854,
-0.300030506500816,-0.298510672817766,-0.296372371615432,-0.29094522638229,
-0.286342433098,-0.266490459338093,-0.244342140841239,-0.239561670201648,
-0.236641836214504,-0.233960285335861,-0.230418016471577,-0.222368375240227,
-0.210784316703314,-0.196186938439091,-0.177412056360276,-0.174428152598249,
-0.172716017721806,-0.171199851310539,-0.169089469839861,-0.163847025814943,
-0.155802938334471,-0.125431168164938,-0.11525581156426,-0.111303140211141,
-0.109929022958247),.UNSPECIFIED.);
#758=B_SPLINE_CURVE_WITH_KNOTS('',3,(#67519,#67520,#67521,#67522,#67523,
#67524,#67525,#67526,#67527,#67528),.UNSPECIFIED.,.F.,.F.,(4,1,1,1,1,1,
1,4),(21.9911545791849,22.3044925686794,23.3019991506414,24.2995057326034,
25.2970123145654,26.2945188965274,27.2920254784894,27.4168483341474),
 .UNSPECIFIED.);
#759=B_SPLINE_CURVE_WITH_KNOTS('',3,(#67529,#67530,#67531,#67532,#67533,
#67534,#67535,#67536,#67537,#67538,#67539,#67540,#67541,#67542,#67543,#67544,
#67545,#67546,#67547,#67548,#67549,#67550,#67551,#67552,#67553,#67554,#67555,
#67556,#67557,#67558,#67559,#67560),.UNSPECIFIED.,.F.,.F.,(4,2,2,2,2,2,
2,2,2,2,2,2,2,2,2,4),(-1.48989964064444,-1.47872022988109,-1.47217755902933,
-1.46929575414241,-1.46681092895138,-1.46413326237901,-1.46067282223444,
-1.45288472447889,-1.43040071064657,-1.40874861758075,-1.40514874379073,
-1.4032474542522,-1.40175146608248,-1.3998993055758,-1.39614539370723,-1.38023582942697),
 .UNSPECIFIED.);
#760=B_SPLINE_CURVE_WITH_KNOTS('',3,(#67562,#67563,#67564,#67565,#67566,
#67567,#67568,#67569,#67570,#67571,#67572,#67573,#67574,#67575,#67576,#67577,
#67578,#67579,#67580,#67581,#67582,#67583,#67584,#67585,#67586,#67587,#67588,
#67589,#67590,#67591,#67592,#67593,#67594,#67595,#67596,#67597,#67598,#67599,
#67600,#67601,#67602,#67603,#67604,#67605),.UNSPECIFIED.,.F.,.F.,(4,2,2,
2,2,2,2,2,2,2,2,2,2,2,2,2,2,2,2,2,2,4),(-0.109929022958247,-0.108827709523117,
-0.106248753533545,-0.106095865042436,-0.105952645963057,-0.105816458283612,
-0.105685184526301,-0.105557054470989,-0.105430525151244,-0.105304193208834,
-0.100925002687213,-0.0956454561187019,-0.0849423192460175,-0.0694325087816073,
-0.0514614323326723,-0.0475756570868673,-0.0456981019448579,-0.0442024164935431,
-0.0423276341335334,-0.0402635563262763,-0.0367985916153872,-0.000389969001955371),
 .UNSPECIFIED.);
#761=B_SPLINE_CURVE_WITH_KNOTS('',3,(#67606,#67607,#67608,#67609,#67610,
#67611,#67612,#67613,#67614,#67615,#67616,#67617,#67618,#67619,#67620,#67621,
#67622,#67623,#67624,#67625,#67626,#67627,#67628,#67629,#67630,#67631,#67632,
#67633,#67634,#67635,#67636,#67637,#67638,#67639,#67640,#67641,#67642,#67643,
#67644,#67645,#67646,#67647,#67648,#67649,#67650,#67651,#67652,#67653,#67654,
#67655,#67656,#67657,#67658,#67659,#67660,#67661,#67662,#67663,#67664,#67665,
#67666,#67667,#67668,#67669,#67670,#67671,#67672,#67673,#67674,#67675,#67676,
#67677,#67678,#67679,#67680,#67681,#67682,#67683,#67684,#67685,#67686,#67687,
#67688,#67689,#67690,#67691,#67692,#67693,#67694,#67695,#67696,#67697,#67698,
#67699,#67700,#67701,#67702,#67703,#67704,#67705,#67706,#67707,#67708,#67709,
#67710,#67711,#67712,#67713,#67714,#67715,#67716,#67717,#67718,#67719,#67720,
#67721,#67722,#67723,#67724,#67725,#67726,#67727,#67728,#67729,#67730,#67731,
#67732,#67733,#67734,#67735,#67736,#67737,#67738,#67739,#67740,#67741,#67742,
#67743,#67744,#67745,#67746,#67747,#67748,#67749,#67750,#67751,#67752,#67753,
#67754,#67755,#67756,#67757,#67758,#67759,#67760,#67761,#67762,#67763,#67764,
#67765,#67766,#67767,#67768,#67769,#67770,#67771,#67772,#67773,#67774,#67775,
#67776,#67777,#67778,#67779,#67780,#67781),.UNSPECIFIED.,.F.,.F.,(4,2,2,
2,2,2,2,2,2,2,2,2,2,2,2,2,2,2,2,2,2,2,2,2,2,2,2,2,2,2,2,2,2,2,2,2,2,2,2,
2,2,2,2,2,2,2,2,2,2,2,2,2,2,2,2,2,2,2,2,2,2,2,2,2,2,2,2,2,2,2,2,2,2,2,2,
2,2,2,2,2,2,2,2,2,2,2,2,4),(-1.60461143394934,-1.59295583522918,-1.58969687259461,
-1.58713600117349,-1.58451749098691,-1.58149594130956,-1.57635988095943,
-1.55789254442106,-1.53793233666413,-1.52799106328758,-1.52446079448715,
-1.52256847341829,-1.52107323202754,-1.51921418095462,-1.51542278630807,
-1.49295974405678,-1.47525451432197,-1.46808444180388,-1.46246476417511,
-1.45941196083208,-1.45749341864908,-1.45456735868366,-1.44975155583518,
-1.42814941060129,-1.40790908203135,-1.40325759170159,-1.40060691652397,
-1.39696135527566,-1.39513067587716,-1.39363427417778,-1.39170975578545,
-1.38771530778068,-1.36256333362951,-1.34692128107798,-1.3402419467513,
-1.33487658102878,-1.33183556894149,-1.32918028494435,-1.32586012847097,
-1.32059644333714,-1.29962069938713,-1.2803288228966,-1.27579792561704,
-1.27043101560275,-1.26830231871488,-1.26678420378276,-1.26508299821651,
-1.26206630302482,-1.24331580779254,-1.22875190546966,-1.2171608299765,
-1.20910765074542,-1.20556623807487,-1.20288623849692,-1.19996899848059,
-1.19519499774944,-1.17386657817923,-1.15334122879147,-1.1486545687781,
-1.14316002326754,-1.14101223813451,-1.13949113827345,-1.13779867465427,
-1.1348229722397,-1.11931676464173,-1.09624305828531,-1.08329387931814,
-1.07911748213852,-1.07632425774352,-1.07361263495037,-1.06971616812769,
-1.0599397115774,-1.03356449037147,-1.01873843399882,-1.01502843688923,
-1.01318511128668,-1.01183862153077,-1.0100068733807,-1.00635586413724,
-0.976963805699658,-0.958363358717214,-0.952935416933458,-0.949881461472766,
-0.947227494290107,-0.943925476865805,-0.938724461420196,-0.912842892704958,
-0.912048192097026),.UNSPECIFIED.);
#762=B_SPLINE_CURVE_WITH_KNOTS('',3,(#67787,#67788,#67789,#67790,#67791,
#67792,#67793,#67794,#67795,#67796,#67797,#67798,#67799,#67800,#67801,#67802,
#67803,#67804,#67805,#67806,#67807,#67808,#67809,#67810,#67811,#67812,#67813,
#67814,#67815,#67816,#67817,#67818,#67819,#67820,#67821,#67822,#67823,#67824,
#67825,#67826,#67827,#67828,#67829,#67830,#67831,#67832,#67833,#67834,#67835,
#67836,#67837,#67838,#67839,#67840,#67841,#67842,#67843,#67844,#67845,#67846,
#67847,#67848,#67849,#67850,#67851,#67852,#67853,#67854,#67855,#67856,#67857,
#67858,#67859,#67860,#67861,#67862,#67863,#67864,#67865,#67866,#67867,#67868,
#67869,#67870,#67871,#67872,#67873,#67874,#67875,#67876,#67877,#67878,#67879,
#67880,#67881,#67882,#67883,#67884,#67885,#67886,#67887,#67888,#67889,#67890,
#67891,#67892,#67893,#67894,#67895,#67896,#67897,#67898,#67899,#67900,#67901,
#67902,#67903,#67904,#67905,#67906,#67907,#67908,#67909,#67910,#67911,#67912,
#67913,#67914,#67915,#67916,#67917,#67918,#67919,#67920,#67921,#67922,#67923,
#67924,#67925,#67926,#67927,#67928,#67929,#67930,#67931,#67932,#67933,#67934,
#67935,#67936,#67937),.UNSPECIFIED.,.F.,.F.,(4,3,3,3,3,3,3,3,3,3,3,3,3,
3,3,3,3,3,3,3,3,3,3,3,3,3,3,3,3,3,3,3,3,3,3,3,3,3,3,3,3,3,3,3,3,3,3,3,3,
3,4),(28.274333882308,28.2895320604514,28.4070356534716,28.5243230424993,
28.641491343524,28.758590535659,28.8756704853353,28.9928648252044,29.1101222354136,
29.2275986095123,29.2870386424133,29.4045422337205,29.5218296210103,29.6389979202831,
29.7560971106555,29.8731770585619,29.9903713966644,30.1076288051063,30.2251051774572,
30.2845452243753,30.402048815337,30.5193362022627,30.6365045011601,30.7536036911465,
30.8706836386574,30.9878779763524,31.1051353843795,31.2226117563091,31.2820518063373,
31.3995553979145,31.516842785472,31.6340110850108,31.7511102756471,31.8681902238148,
31.9853845621724,32.1026419708661,32.220118343461,32.2795583882993,32.3970619796289,
32.5143493669347,32.6315176662193,32.7486168565995,32.8656968045097,32.9828911426097,
33.1001485510454,33.2176249233846,33.2770649702613,33.3945293996392,33.5118245182542,
33.6289923657488,33.6995813315044),.UNSPECIFIED.);
#763=B_SPLINE_CURVE_WITH_KNOTS('',3,(#67938,#67939,#67940,#67941),
 .UNSPECIFIED.,.F.,.F.,(4,4),(27.4168483341474,28.2743318237622),
 .UNSPECIFIED.);
#764=B_SPLINE_CURVE_WITH_KNOTS('',3,(#67942,#67943,#67944,#67945,#67946,
#67947,#67948,#67949,#67950,#67951,#67952,#67953,#67954,#67955,#67956,#67957,
#67958,#67959,#67960,#67961,#67962,#67963,#67964,#67965,#67966,#67967,#67968,
#67969,#67970,#67971,#67972,#67973,#67974,#67975,#67976,#67977,#67978,#67979,
#67980,#67981,#67982,#67983,#67984,#67985,#67986,#67987,#67988,#67989,#67990,
#67991,#67992,#67993,#67994,#67995,#67996,#67997,#67998,#67999,#68000,#68001,
#68002,#68003,#68004,#68005,#68006,#68007,#68008,#68009,#68010,#68011,#68012,
#68013,#68014,#68015,#68016,#68017,#68018,#68019,#68020,#68021,#68022,#68023,
#68024,#68025,#68026,#68027,#68028,#68029,#68030,#68031,#68032,#68033,#68034,
#68035,#68036,#68037,#68038,#68039,#68040,#68041,#68042,#68043,#68044,#68045,
#68046,#68047,#68048,#68049,#68050,#68051,#68052,#68053,#68054,#68055,#68056,
#68057,#68058,#68059,#68060,#68061,#68062,#68063,#68064,#68065,#68066,#68067,
#68068,#68069,#68070,#68071,#68072,#68073,#68074,#68075,#68076,#68077,#68078,
#68079,#68080,#68081,#68082,#68083,#68084,#68085,#68086,#68087,#68088,#68089,
#68090,#68091,#68092,#68093,#68094,#68095,#68096,#68097,#68098,#68099,#68100,
#68101,#68102,#68103,#68104,#68105,#68106,#68107,#68108,#68109,#68110,#68111,
#68112,#68113,#68114,#68115,#68116,#68117,#68118,#68119,#68120,#68121,#68122,
#68123,#68124,#68125,#68126,#68127,#68128,#68129,#68130,#68131,#68132,#68133,
#68134,#68135,#68136,#68137,#68138,#68139,#68140,#68141,#68142,#68143,#68144,
#68145,#68146,#68147,#68148,#68149,#68150,#68151,#68152,#68153,#68154,#68155,
#68156,#68157,#68158,#68159,#68160,#68161,#68162,#68163,#68164,#68165,#68166,
#68167,#68168,#68169,#68170,#68171,#68172,#68173,#68174,#68175,#68176,#68177),
 .UNSPECIFIED.,.F.,.F.,(4,2,2,2,2,2,2,2,2,2,2,2,2,2,2,2,2,2,2,2,2,2,2,2,
2,2,2,2,2,2,2,2,2,2,2,2,2,2,2,2,2,2,2,2,2,2,2,2,2,2,2,2,2,2,2,2,2,2,2,2,
2,2,2,2,2,2,2,2,2,2,2,2,2,2,2,2,2,2,2,2,2,2,2,2,2,2,2,2,2,2,2,2,2,2,2,2,
2,2,2,2,2,2,2,2,2,2,2,2,2,2,2,2,2,2,2,2,2,4),(-0.912048192097026,-0.897193903287954,
-0.891757102115713,-0.887811118919318,-0.885922525591254,-0.884427183118311,
-0.88256419929221,-0.878752693007088,-0.850190635474282,-0.836498509102547,
-0.827479694830447,-0.823787281105917,-0.821084199625904,-0.818569687361485,
-0.814391705207285,-0.802414353835596,-0.779607145104645,-0.762851750132384,
-0.7598577723789,-0.758161361658475,-0.756641500768136,-0.754502139473377,
-0.749064550920135,-0.74444826372594,-0.724483251978669,-0.702499382731449,
-0.697719977415738,-0.694801478857277,-0.692121624438214,-0.688582337773265,
-0.680543390283385,-0.668979946117005,-0.654359167188749,-0.635569575467892,
-0.632551594375238,-0.630850023407637,-0.629331811870553,-0.627203361849867,
-0.621838686723182,-0.617311109419045,-0.598038984964131,-0.577067020851179,
-0.571809318759909,-0.568490700330377,-0.56583530328618,-0.562792697539817,
-0.557420605019109,-0.553787263814848,-0.547889788586742,-0.525473155924292,
-0.508198632944983,-0.505202328971343,-0.50350533819836,-0.501985511723585,
-0.499846959060263,-0.494415466537649,-0.489806777428288,-0.469903386628048,
-0.447836519810407,-0.44305742056549,-0.440138840658775,-0.437458738378408,
-0.433918867993808,-0.425877396242107,-0.414309130225609,-0.399691403202778,
-0.380902685852573,-0.377884550080002,-0.376182865732762,-0.374664532663339,
-0.372535885587055,-0.367170577308199,-0.362642384942705,-0.343366735527645,
-0.322396451717294,-0.317137973073629,-0.313818991267101,-0.311163381019295,
-0.308120615355241,-0.302748470388934,-0.299115177246632,-0.293217966750355,
-0.270804648438807,-0.253522142301399,-0.250525578724478,-0.248828450724155,
-0.247308508850699,-0.245169803805127,-0.23973797677519,-0.235129035217801,
-0.215224924478593,-0.193155313723836,-0.188375855415121,-0.18545705244339,
-0.182776742868282,-0.179236595040061,-0.17119447587694,-0.159625261368032,
-0.145006469060257,-0.126229055672179,-0.123238412258239,-0.121525367815816,
-0.120055790287089,-0.120024690568117,-0.119993873759491,-0.119963297723458,
-0.119932922280232,-0.119902709036972,-0.119872621203619,-0.119842623226302,
-0.119812680682742,-0.119782760123177,-0.119752828823599,-0.119722854653954,
-0.117625590987786,-0.115048214893327,-0.110212516818048,-0.109970659150362),
 .UNSPECIFIED.);
#765=B_SPLINE_CURVE_WITH_KNOTS('',3,(#68183,#68184,#68185,#68186,#68187,
#68188,#68189,#68190,#68191,#68192,#68193,#68194,#68195,#68196,#68197,#68198,
#68199,#68200,#68201,#68202,#68203,#68204,#68205,#68206,#68207,#68208,#68209,
#68210,#68211,#68212,#68213,#68214,#68215,#68216,#68217,#68218,#68219,#68220,
#68221,#68222,#68223,#68224,#68225,#68226,#68227,#68228,#68229,#68230,#68231,
#68232,#68233,#68234,#68235,#68236,#68237,#68238,#68239,#68240,#68241,#68242,
#68243,#68244,#68245,#68246,#68247,#68248,#68249,#68250,#68251,#68252,#68253,
#68254,#68255,#68256,#68257,#68258,#68259,#68260,#68261,#68262,#68263,#68264,
#68265,#68266,#68267,#68268,#68269,#68270,#68271,#68272,#68273,#68274,#68275,
#68276,#68277,#68278,#68279,#68280,#68281,#68282,#68283,#68284,#68285,#68286,
#68287,#68288,#68289,#68290,#68291,#68292,#68293,#68294,#68295,#68296,#68297,
#68298,#68299,#68300,#68301,#68302,#68303,#68304,#68305,#68306,#68307,#68308,
#68309,#68310,#68311,#68312,#68313,#68314,#68315,#68316,#68317,#68318,#68319,
#68320,#68321,#68322,#68323,#68324,#68325,#68326,#68327,#68328,#68329,#68330,
#68331,#68332,#68333,#68334,#68335,#68336,#68337,#68338,#68339,#68340,#68341,
#68342,#68343,#68344,#68345,#68346,#68347,#68348,#68349,#68350,#68351,#68352,
#68353,#68354,#68355,#68356,#68357,#68358,#68359,#68360,#68361,#68362,#68363,
#68364,#68365,#68366,#68367,#68368,#68369,#68370,#68371,#68372,#68373,#68374,
#68375,#68376,#68377,#68378,#68379,#68380,#68381,#68382,#68383,#68384,#68385,
#68386,#68387,#68388,#68389,#68390),.UNSPECIFIED.,.F.,.F.,(4,2,2,2,2,2,
2,2,2,2,2,2,2,2,2,2,2,2,2,2,2,2,2,2,2,2,2,2,2,2,2,2,2,2,2,2,2,2,2,2,2,2,
2,2,2,2,2,2,2,2,2,2,2,2,2,2,2,2,2,2,2,2,2,2,2,2,2,2,2,2,2,2,2,2,2,2,2,2,
2,2,2,2,2,2,2,2,2,2,2,2,2,2,2,2,2,2,2,2,2,2,2,2,2,4),(-0.693066393259155,
-0.674906229938858,-0.669695437266216,-0.666390072292241,-0.663735182271511,
-0.660682084047088,-0.655260976408456,-0.648490228107516,-0.632483582971117,
-0.607027920981691,-0.603539708069288,-0.60171810338321,-0.600370683697547,
-0.598515383348405,-0.594745496399711,-0.579381515359838,-0.55142437542294,
-0.543304037998711,-0.540014044368528,-0.537299532118133,-0.534508079932375,
-0.530343570696701,-0.517522269532378,-0.494928775281844,-0.47876086670957,
-0.475771234080074,-0.474075444722218,-0.472554735866463,-0.470412193829133,
-0.464955793622309,-0.46031697425351,-0.44017427137986,-0.418475759716522,
-0.413662641585343,-0.410736487363225,-0.408057883529762,-0.404532424216253,
-0.396581116946435,-0.385198662333336,-0.370389535867719,-0.351483909403705,
-0.348496175341454,-0.346783637871101,-0.345268161446529,-0.343160519728219,
-0.337934638715828,-0.329926235081169,-0.31265927996927,-0.291108173467055,
-0.286312740235186,-0.283390244756187,-0.280710430450574,-0.277176655060345,
-0.26917546318399,-0.257690932346598,-0.242984492870763,-0.224144302180962,
-0.221123943979906,-0.219421521998448,-0.217902888230671,-0.215774257034712,
-0.210411162278677,-0.205886022501703,-0.186635319604914,-0.165623919848117,
-0.160369570075876,-0.157051343434937,-0.154395180834349,-0.154174079737939,
-0.154055433945555,-0.153992186195788,-0.153876447869909,-0.153773081919531,
-0.153680678727045,-0.153597999905942,-0.153523957238636,-0.153457593715937,
-0.153398066757247,-0.153344633533162,-0.153296638187705,-0.153253500756339,
-0.15321470760693,-0.15317980316396,-0.153148382734162,-0.153120086296268,
-0.149541605852723,-0.140967508289976,-0.128183370529552,-0.102955114776677,
-0.0957076419459197,-0.0932565679957738,-0.0918335628704321,-0.0902758157150152,
-0.0886796347272504,-0.0843793562968723,-0.0689392068738299,-0.044875813738082,
-0.0346653684092674,-0.030707667992101,-0.0282312462253062,-0.0257169962615631,
-0.0230399161961442,-0.0194315076543716,-0.000374860171283078),
 .UNSPECIFIED.);
#766=B_SPLINE_CURVE_WITH_KNOTS('',3,(#68391,#68392,#68393,#68394,#68395,
#68396,#68397,#68398,#68399,#68400,#68401,#68402,#68403,#68404,#68405,#68406,
#68407,#68408,#68409,#68410,#68411,#68412),.UNSPECIFIED.,.F.,.F.,(4,3,3,
3,3,3,3,4),(33.6995813315044,33.8166629614849,33.9338446683203,34.0510716663033,
34.168532981513,34.2745715522233,34.4195088297933,34.557519189051),
 .UNSPECIFIED.);
#767=B_SPLINE_CURVE_WITH_KNOTS('',3,(#68414,#68415,#68416,#68417,#68418,
#68419,#68420,#68421,#68422,#68423,#68424,#68425,#68426,#68427,#68428,#68429,
#68430,#68431,#68432,#68433,#68434,#68435),.UNSPECIFIED.,.F.,.F.,(4,2,2,
2,2,2,2,2,2,2,4),(-0.109970659150362,-0.0881264654925452,-0.0658920433884551,
-0.0610673507265949,-0.0581389916306896,-0.0554614768900394,-0.0519420341948714,
-0.0440255142552692,-0.0327138928635081,-0.0179861676643662,-0.000375331772795134),
 .UNSPECIFIED.);
#768=B_SPLINE_CURVE_WITH_KNOTS('',3,(#68436,#68437,#68438,#68439,#68440,
#68441,#68442,#68443,#68444,#68445,#68446,#68447,#68448,#68449,#68450,#68451,
#68452,#68453,#68454,#68455,#68456,#68457,#68458,#68459,#68460,#68461,#68462,
#68463,#68464,#68465,#68466,#68467,#68468,#68469,#68470,#68471,#68472,#68473,
#68474,#68475,#68476,#68477,#68478,#68479,#68480,#68481,#68482,#68483,#68484,
#68485,#68486,#68487,#68488,#68489,#68490,#68491,#68492,#68493,#68494,#68495,
#68496,#68497,#68498,#68499,#68500,#68501,#68502,#68503,#68504,#68505,#68506,
#68507,#68508,#68509,#68510,#68511,#68512,#68513,#68514,#68515,#68516,#68517,
#68518,#68519,#68520,#68521,#68522,#68523,#68524,#68525,#68526,#68527,#68528,
#68529,#68530,#68531,#68532,#68533,#68534,#68535,#68536,#68537,#68538,#68539,
#68540,#68541,#68542,#68543,#68544,#68545,#68546,#68547,#68548,#68549,#68550,
#68551,#68552,#68553,#68554,#68555,#68556,#68557,#68558,#68559,#68560,#68561,
#68562,#68563,#68564,#68565,#68566,#68567,#68568,#68569,#68570,#68571,#68572,
#68573,#68574,#68575,#68576,#68577,#68578,#68579,#68580,#68581,#68582,#68583,
#68584,#68585,#68586,#68587,#68588,#68589,#68590,#68591,#68592,#68593,#68594,
#68595,#68596,#68597,#68598,#68599,#68600,#68601,#68602,#68603,#68604,#68605,
#68606,#68607,#68608,#68609,#68610,#68611,#68612,#68613),.UNSPECIFIED.,
 .F.,.F.,(4,2,2,2,2,2,2,2,2,2,2,2,2,2,2,2,2,2,2,2,2,2,2,2,2,2,2,2,2,2,2,
2,2,2,2,2,2,2,2,2,2,2,2,2,2,2,2,2,2,2,2,2,2,2,2,2,2,2,2,2,2,2,2,2,2,2,2,
2,2,2,2,2,2,2,2,2,2,2,2,2,2,2,2,2,2,2,2,2,4),(-1.60470189091564,-1.60095296946403,
-1.59939692088769,-1.59798940636926,-1.59636898833446,-1.59372612825631,
-1.58456665102568,-1.55978920851748,-1.5439158864618,-1.53853080173819,
-1.53548568883745,-1.53283081567452,-1.52951641732134,-1.52427270745507,
-1.50351491174043,-1.48402315765339,-1.47792196713859,-1.4749089175248,
-1.47302320633092,-1.47130543585475,-1.47014973497877,-1.46833082152723,
-1.46485381500265,-1.43936845750963,-1.42340057789767,-1.41344590430104,
-1.409620351403,-1.40689432887467,-1.40440892972212,-1.4003946874682,-1.38976272433269,
-1.35972748074174,-1.34803177816093,-1.34528019380035,-1.34363605206564,
-1.34211094764519,-1.33985282440251,-1.33403117898286,-1.31061400033734,
-1.28919254965368,-1.28382908980427,-1.28078824474108,-1.27813258973901,
-1.2748112880841,-1.26954437090681,-1.24859297383053,-1.2292822783375,-1.22474869996889,
-1.21937938066883,-1.21725015513871,-1.21573180788214,-1.21403050204633,
-1.21101397507488,-1.19227787196204,-1.17774379359185,-1.16612242505057,
-1.15805428939221,-1.15451014228935,-1.15182947945072,-1.14891287937641,
-1.14414308683646,-1.12289296271921,-1.10521218902712,-1.09721589268933,
-1.09199644049164,-1.08989009137095,-1.08837514244797,-1.08666272030503,
-1.08367435703639,-1.06474582095933,-1.04960625416472,-1.03845921299609,
-1.03473264958251,-1.02925778352664,-1.02619393570368,-1.02354052724862,
-1.02025106870403,-1.01509398528379,-0.988145335134789,-0.973213482996621,
-0.967916857538369,-0.964046995923919,-0.962172691461779,-0.960677244249893,
-0.958799786534675,-0.954913358189951,-0.936681336444259,-0.914454034042733,
-0.912213000320031),.UNSPECIFIED.);
#769=B_SPLINE_CURVE_WITH_KNOTS('',3,(#68618,#68619,#68620,#68621,#68622,
#68623,#68624,#68625,#68626,#68627,#68628,#68629,#68630,#68631,#68632,#68633,
#68634,#68635,#68636,#68637,#68638,#68639,#68640,#68641,#68642,#68643,#68644,
#68645,#68646,#68647,#68648,#68649,#68650,#68651,#68652,#68653,#68654,#68655,
#68656,#68657,#68658,#68659,#68660,#68661,#68662,#68663,#68664,#68665,#68666,
#68667,#68668,#68669,#68670,#68671,#68672,#68673,#68674,#68675,#68676,#68677,
#68678,#68679,#68680,#68681,#68682,#68683,#68684,#68685,#68686,#68687,#68688,
#68689,#68690,#68691,#68692,#68693,#68694,#68695,#68696,#68697,#68698,#68699,
#68700,#68701,#68702,#68703,#68704,#68705,#68706,#68707,#68708,#68709,#68710,
#68711,#68712,#68713,#68714,#68715,#68716,#68717,#68718,#68719,#68720,#68721,
#68722,#68723,#68724,#68725,#68726,#68727,#68728,#68729,#68730,#68731,#68732,
#68733,#68734,#68735,#68736,#68737,#68738,#68739,#68740,#68741,#68742,#68743,
#68744,#68745,#68746,#68747,#68748,#68749,#68750,#68751,#68752,#68753,#68754,
#68755,#68756,#68757,#68758,#68759,#68760,#68761,#68762,#68763,#68764,#68765,
#68766,#68767,#68768,#68769,#68770,#68771,#68772,#68773,#68774,#68775,#68776,
#68777,#68778,#68779,#68780,#68781,#68782,#68783,#68784,#68785,#68786,#68787,
#68788,#68789,#68790,#68791,#68792,#68793,#68794,#68795,#68796,#68797,#68798,
#68799,#68800,#68801,#68802,#68803,#68804,#68805,#68806,#68807,#68808,#68809,
#68810,#68811,#68812,#68813,#68814,#68815,#68816,#68817,#68818,#68819,#68820,
#68821,#68822,#68823,#68824,#68825,#68826,#68827),.UNSPECIFIED.,.F.,.F.,
(4,2,2,2,2,2,2,2,2,2,2,2,2,2,2,2,2,2,2,2,2,2,2,2,2,2,2,2,2,2,2,2,2,2,2,
2,2,2,2,2,2,2,2,2,2,2,2,2,2,2,2,2,2,2,2,2,2,2,2,2,2,2,2,2,2,2,2,2,2,2,2,
2,2,2,2,2,2,2,2,2,2,2,2,2,2,2,2,2,2,2,2,2,2,2,2,2,2,2,2,2,2,2,2,2,4),(-1.49506358435903,
-1.49459316852251,-1.49295987179869,-1.49154761020416,-1.48962849527195,
-1.48551958585863,-1.46046986416288,-1.44482595301145,-1.43814582163569,
-1.43277974809073,-1.42973818189258,-1.42708230725347,-1.42376125009147,
-1.41849573727524,-1.39753559702045,-1.37823521492406,-1.37370308742887,
-1.36833490836962,-1.36620574026705,-1.36468728335974,-1.3629856394231,
-1.35996799539036,-1.34120155414277,-1.32660700712414,-1.31504458880383,
-1.30700497676871,-1.30346531738608,-1.30078506395088,-1.29786599430001,
-1.29308533386462,-1.27101074170306,-1.25108718660959,-1.24647507935482,
-1.2410411040156,-1.23890203920943,-1.23738204310009,-1.23568497927446,
-1.2326888299206,-1.21529497939766,-1.19300466725329,-1.18712646617886,
-1.18350184059288,-1.1781388591753,-1.17509792701522,-1.17244197261471,
-1.16911998099,-1.16385125390158,-1.14292542497544,-1.12360274830032,-1.11906770775998,
-1.11369711877518,-1.11156758305447,-1.11004906650738,-1.10834758789171,
-1.10533073310359,-1.08658844294957,-1.07203881844943,-1.06043475903791,
-1.05237497387356,-1.04883199938223,-1.04615127770301,-1.04323367904321,
-1.03846003478107,-1.01567016700984,-0.996298126047144,-0.991756634007073,
-0.986380699161068,-0.984250339448056,-0.982731681019322,-0.981030554158052,
-0.9780154135377,-0.959327927490739,-0.944888424427529,-0.933184684646064,
-0.925076761712725,-0.921525888972868,-0.918844029195806,-0.915929870677276,
-0.911172694588434,-0.890231472159465,-0.869370980182679,-0.864643600490223,
-0.86196101666687,-0.858282821276543,-0.856445487354999,-0.855098928911026,
-0.85326049452433,-0.84969181577703,-0.825081844443449,-0.802669500212144,
-0.797234870802052,-0.793865129126414,-0.791204984213659,-0.788195458326038,
-0.782983957580618,-0.757313399843094,-0.734785802988896,-0.730994798142771,
-0.729135461641677,-0.727639632896396,-0.725746069217201,-0.721775278484118,
-0.716293897360636,-0.700409747126883,-0.693066393259155),.UNSPECIFIED.);
#770=B_SPLINE_CURVE_WITH_KNOTS('',3,(#68828,#68829,#68830,#68831,#68832,
#68833,#68834,#68835,#68836,#68837,#68838,#68839,#68840,#68841,#68842,#68843,
#68844,#68845,#68846,#68847,#68848,#68849,#68850,#68851,#68852,#68853,#68854,
#68855,#68856,#68857,#68858,#68859,#68860,#68861,#68862,#68863,#68864,#68865,
#68866,#68867,#68868,#68869,#68870,#68871,#68872,#68873,#68874,#68875,#68876,
#68877,#68878,#68879,#68880,#68881,#68882,#68883,#68884,#68885,#68886,#68887,
#68888,#68889,#68890,#68891,#68892,#68893,#68894,#68895,#68896,#68897,#68898,
#68899,#68900,#68901,#68902,#68903,#68904,#68905,#68906,#68907,#68908,#68909,
#68910,#68911,#68912,#68913,#68914,#68915,#68916,#68917,#68918,#68919,#68920,
#68921,#68922,#68923,#68924,#68925,#68926,#68927,#68928,#68929,#68930,#68931,
#68932,#68933,#68934,#68935,#68936,#68937,#68938,#68939,#68940,#68941,#68942,
#68943,#68944,#68945,#68946,#68947,#68948,#68949,#68950,#68951,#68952,#68953,
#68954,#68955,#68956,#68957,#68958,#68959,#68960,#68961,#68962,#68963,#68964,
#68965,#68966,#68967,#68968,#68969,#68970,#68971,#68972,#68973,#68974,#68975,
#68976,#68977,#68978,#68979,#68980,#68981,#68982,#68983,#68984,#68985,#68986,
#68987,#68988,#68989,#68990,#68991,#68992,#68993,#68994,#68995,#68996,#68997,
#68998,#68999,#69000,#69001,#69002,#69003,#69004,#69005,#69006,#69007,#69008,
#69009,#69010,#69011,#69012,#69013,#69014,#69015,#69016,#69017,#69018,#69019,
#69020,#69021,#69022,#69023,#69024,#69025,#69026,#69027,#69028,#69029,#69030,
#69031,#69032,#69033,#69034,#69035),.UNSPECIFIED.,.F.,.F.,(4,2,2,2,2,2,
2,2,2,2,2,2,2,2,2,2,2,2,2,2,2,2,2,2,2,2,2,2,2,2,2,2,2,2,2,2,2,2,2,2,2,2,
2,2,2,2,2,2,2,2,2,2,2,2,2,2,2,2,2,2,2,2,2,2,2,2,2,2,2,2,2,2,2,2,2,2,2,2,
2,2,2,2,2,2,2,2,2,2,2,2,2,2,2,2,2,2,2,2,2,2,2,2,2,4),(-0.912213000320031,
-0.904185423138655,-0.900317621453881,-0.897583697094516,-0.895105821397266,
-0.891771599658252,-0.883373245940542,-0.855674846088848,-0.840393111228322,
-0.836632359294594,-0.834778978194245,-0.83343184280948,-0.831609016922357,
-0.828114371926604,-0.802747979360156,-0.780655750146395,-0.775386105046824,
-0.772063877217642,-0.769407992278481,-0.766367435977363,-0.76100606058388,
-0.754332480936613,-0.731470781708606,-0.713230871208786,-0.709343001741131,
-0.707465204914766,-0.705969674854692,-0.704095500623492,-0.70022664158367,
-0.694932836332411,-0.68001305162414,-0.653087045578872,-0.647931078922335,
-0.644641816397422,-0.641988270290673,-0.638923933862759,-0.633447353207738,
-0.629718945058427,-0.618563751311103,-0.603406768578255,-0.584458957476656,
-0.581470020876322,-0.579757389404236,-0.578242301674307,-0.576135894239818,
-0.570916648870514,-0.562922445546916,-0.545340521356904,-0.524037115108987,
-0.519263324649768,-0.516345708352359,-0.513665017725299,-0.510122185999156,
-0.502063748135204,-0.49046085173145,-0.475878189141995,-0.457107752539287,
-0.454090021396908,-0.452388338554731,-0.450869839211915,-0.448740729155319,
-0.443373053732892,-0.438842153232241,-0.419546980548521,-0.398603840424228,
-0.393341804662594,-0.390021650092343,-0.387365757321423,-0.384323381401009,
-0.378953868555389,-0.375323062539216,-0.352806882741564,-0.331041127461899,
-0.327245160261254,-0.32538486817583,-0.323889076332513,-0.321996624786792,
-0.318031747338709,-0.312561416596615,-0.296736860055886,-0.27113719570378,
-0.26592825929231,-0.262623433317465,-0.259968605248771,-0.256915189675632,
-0.251492511506997,-0.244719280205865,-0.228703630202243,-0.203251925941467,
-0.199762220196112,-0.197940303071016,-0.196592920664014,-0.194738055494788,
-0.190970402351699,-0.17562791302048,-0.147739595214316,-0.139545989277664,
-0.136244228670731,-0.13363872417429,-0.131130223575698,-0.128417538892109,
-0.124710172973325,-0.118469338295433,-0.110007165866594),.UNSPECIFIED.);
#771=B_SPLINE_CURVE_WITH_KNOTS('',3,(#69041,#69042,#69043,#69044,#69045,
#69046,#69047,#69048,#69049,#69050,#69051,#69052,#69053,#69054,#69055,#69056,
#69057,#69058,#69059,#69060,#69061,#69062,#69063,#69064,#69065,#69066,#69067,
#69068,#69069,#69070,#69071,#69072,#69073,#69074,#69075,#69076,#69077,#69078,
#69079,#69080,#69081,#69082,#69083,#69084,#69085,#69086,#69087,#69088,#69089,
#69090,#69091,#69092,#69093,#69094,#69095,#69096,#69097,#69098,#69099,#69100,
#69101,#69102,#69103,#69104,#69105,#69106,#69107,#69108,#69109,#69110,#69111,
#69112,#69113,#69114,#69115,#69116,#69117,#69118,#69119,#69120,#69121,#69122,
#69123,#69124,#69125,#69126,#69127,#69128,#69129,#69130,#69131,#69132,#69133,
#69134,#69135,#69136,#69137,#69138,#69139,#69140,#69141,#69142,#69143,#69144,
#69145,#69146,#69147,#69148,#69149,#69150,#69151,#69152,#69153,#69154,#69155,
#69156,#69157,#69158,#69159,#69160,#69161,#69162,#69163,#69164,#69165,#69166,
#69167,#69168,#69169,#69170,#69171,#69172,#69173,#69174,#69175,#69176,#69177,
#69178,#69179,#69180,#69181,#69182,#69183,#69184,#69185,#69186,#69187,#69188,
#69189,#69190,#69191,#69192,#69193,#69194,#69195,#69196,#69197,#69198,#69199,
#69200,#69201,#69202,#69203,#69204,#69205,#69206,#69207,#69208,#69209,#69210,
#69211,#69212,#69213,#69214,#69215,#69216,#69217,#69218,#69219,#69220,#69221,
#69222),.UNSPECIFIED.,.F.,.F.,(4,2,2,2,2,2,2,2,2,2,2,2,2,2,2,2,2,2,2,2,
2,2,2,2,2,2,2,2,2,2,2,2,2,2,2,2,2,2,2,2,2,2,2,2,2,2,2,2,2,2,2,2,2,2,2,2,
2,2,2,2,2,2,2,2,2,2,2,2,2,2,2,2,2,2,2,2,2,2,2,2,2,2,2,2,2,2,2,2,2,2,4),
(-0.692976027751027,-0.690677018759155,-0.67607130447192,-0.657289354510635,
-0.654305699491911,-0.652594027778611,-0.651078206133527,-0.648968571102928,
-0.643730147392798,-0.635694444396294,-0.604956671733111,-0.600515487569622,
-0.593586963882524,-0.59023955066128,-0.587581085193234,-0.584556430275175,
-0.579273628352794,-0.554770843352943,-0.530999517730569,-0.527332048054737,
-0.52549660458651,-0.524149656932507,-0.5223085422684,-0.518612169647566,
-0.503913952439148,-0.477897660548173,-0.467760697986265,-0.463813346606405,
-0.461338762878883,-0.458599929607237,-0.454708557941114,-0.444265211086943,
-0.426993496985563,-0.403687880719116,-0.399990519196653,-0.398149190010454,
-0.396802416097306,-0.394967212275677,-0.391301078978969,-0.388630827177835,
-0.383933295963051,-0.363314832917524,-0.342122444417286,-0.337354427756351,
-0.334437562698699,-0.33175574471474,-0.328208700088314,-0.320127680685125,
-0.308478835162429,-0.293945782556724,-0.275201555131824,-0.272184190010179,
-0.270482330080033,-0.268963364564397,-0.266833126430772,-0.261460020954143,
-0.256922903642597,-0.237581456219421,-0.214771826489122,-0.210003316459699,
-0.207086302125691,-0.204404445719564,-0.200857497082934,-0.192777387695453,
-0.181130547859992,-0.166594637629413,-0.149280265482203,-0.145396393218514,
-0.143519047756513,-0.143149369139958,-0.141661755510349,-0.13963305064656,
-0.137286949418663,-0.133083790273205,-0.122934175346161,-0.0886229696348173,
-0.0832480468122925,-0.080173330431059,-0.0775452588392117,-0.0742800389403422,
-0.0679988256869937,-0.0653883053324759,-0.0389927124813264,-0.0236378442675931,
-0.0186759487146624,-0.0167512895609681,-0.015218376560855,-0.0138244657348888,
-0.0121928527065857,-0.00981889569000219,-0.000374665579676547),
 .UNSPECIFIED.);
#772=B_SPLINE_CURVE_WITH_KNOTS('',3,(#69223,#69224,#69225,#69226,#69227,
#69228,#69229,#69230,#69231,#69232,#69233,#69234,#69235,#69236,#69237,#69238,
#69239,#69240,#69241,#69242,#69243,#69244,#69245,#69246,#69247,#69248),
 .UNSPECIFIED.,.F.,.F.,(4,2,2,2,2,2,2,2,2,2,2,2,4),(-1.60472169846197,-1.57239004611136,
-1.56559352016807,-1.56167378571222,-1.55812169644377,-1.55543974735561,
-1.55252629288628,-1.54777211810372,-1.52692702746105,-1.51024911685062,
-1.50136262048626,-1.49750125048159,-1.49506358435903),.UNSPECIFIED.);
#773=B_SPLINE_CURVE_WITH_KNOTS('',3,(#69250,#69251,#69252,#69253,#69254,
#69255,#69256,#69257,#69258,#69259,#69260,#69261,#69262,#69263,#69264,#69265,
#69266,#69267,#69268,#69269,#69270,#69271,#69272,#69273,#69274,#69275,#69276,
#69277,#69278,#69279,#69280,#69281),.UNSPECIFIED.,.F.,.F.,(4,2,2,2,2,2,
2,2,2,2,2,2,2,2,2,4),(-0.110007165866594,-0.104507449886709,-0.0838701566740523,
-0.0743878709420968,-0.0717087400849561,-0.070080137279803,-0.0685271391723869,
-0.0662040699472125,-0.0594070965096256,-0.0271399959987747,-0.0136759747962797,
-0.0094316992061634,-0.00659078795257742,-0.0040613220566676,-0.00213809552869001,
-0.000374875370209125),.UNSPECIFIED.);
#774=B_SPLINE_CURVE_WITH_KNOTS('',3,(#69282,#69283,#69284,#69285,#69286,
#69287,#69288,#69289,#69290,#69291,#69292,#69293,#69294,#69295,#69296,#69297,
#69298,#69299,#69300,#69301,#69302,#69303,#69304,#69305,#69306,#69307,#69308,
#69309,#69310,#69311,#69312,#69313,#69314,#69315,#69316,#69317,#69318,#69319,
#69320,#69321,#69322,#69323,#69324,#69325,#69326,#69327,#69328,#69329,#69330,
#69331,#69332,#69333,#69334,#69335,#69336,#69337,#69338,#69339,#69340,#69341,
#69342,#69343,#69344,#69345,#69346,#69347,#69348,#69349,#69350,#69351,#69352,
#69353,#69354,#69355,#69356,#69357,#69358,#69359,#69360,#69361,#69362,#69363,
#69364,#69365,#69366,#69367,#69368,#69369,#69370,#69371,#69372,#69373,#69374,
#69375,#69376,#69377,#69378,#69379,#69380,#69381,#69382,#69383,#69384,#69385,
#69386,#69387,#69388,#69389,#69390,#69391,#69392,#69393,#69394,#69395,#69396,
#69397,#69398,#69399,#69400,#69401,#69402,#69403,#69404,#69405,#69406,#69407,
#69408,#69409,#69410,#69411,#69412,#69413,#69414,#69415,#69416,#69417,#69418,
#69419,#69420,#69421,#69422,#69423,#69424,#69425,#69426,#69427,#69428,#69429,
#69430,#69431,#69432,#69433,#69434,#69435,#69436,#69437,#69438,#69439,#69440,
#69441,#69442,#69443,#69444,#69445,#69446,#69447,#69448,#69449,#69450,#69451,
#69452,#69453,#69454,#69455,#69456,#69457,#69458,#69459,#69460,#69461,#69462,
#69463,#69464,#69465,#69466,#69467,#69468,#69469),.UNSPECIFIED.,.F.,.F.,
(4,2,2,2,2,2,2,2,2,2,2,2,2,2,2,2,2,2,2,2,2,2,2,2,2,2,2,2,2,2,2,2,2,2,2,
2,2,2,2,2,2,2,2,2,2,2,2,2,2,2,2,2,2,2,2,2,2,2,2,2,2,2,2,2,2,2,2,2,2,2,2,
2,2,2,2,2,2,2,2,2,2,2,2,2,2,2,2,2,2,2,2,2,2,4),(-1.60452966110218,-1.60139615323569,
-1.59616027114913,-1.56214671608205,-1.55475260021891,-1.55132820008312,
-1.54855456450182,-1.54690569049585,-1.5453831863967,-1.54313905556618,
-1.53740448052939,-1.51391364726702,-1.50993883305555,-1.49735969596893,
-1.48883954439345,-1.48601194681116,-1.48583118372699,-1.48565234088406,
-1.48546628960481,-1.48526013381114,-1.48501062067329,-1.48465960553332,
-1.48430764242497,-1.48172843252811,-1.4785606293793,-1.47286449254571,
-1.45188293756239,-1.4325561589479,-1.42802054955213,-1.42264960637224,
-1.42052017864715,-1.4190018392707,-1.41730071655422,-1.41428488655772,
-1.39556802960809,-1.38107110745189,-1.36941682586789,-1.36133287342369,
-1.35778621133186,-1.35510526685074,-1.35218992934655,-1.34742584068909,
-1.32628988116273,-1.30847623438016,-1.30048590753895,-1.29526923715334,
-1.29316335962203,-1.29164851785947,-1.28993594881599,-1.28694677947623,
-1.26799407701781,-1.25313665781787,-1.24184119467159,-1.23393194577901,
-1.23041408233831,-1.22773709605892,-1.22480864945179,-1.21998228990476,
-1.19687346179318,-1.17782592331505,-1.1733269434758,-1.16798626922089,
-1.16586139991853,-1.16434373602964,-1.1626404142586,-1.15961434941508,
-1.14060822875449,-1.12571158699456,-1.11447183778685,-1.10658996355613,
-1.10307662914097,-1.10040022105723,-1.09746958854071,-1.09263296286064,
-1.07041839422467,-1.05068522648163,-1.04609718990203,-1.04068304386393,
-1.0385470867333,-1.03702771353008,-1.03532957428315,-1.03232783478608,
-1.014245127035,-0.983252200262885,-0.977814412117494,-0.97475835951896,
-0.972104490284592,-0.968805094204545,-0.963613320763827,-0.937452959056019,
-0.921995285602853,-0.916595328301845,-0.912669276484203,-0.912009248555571),
 .UNSPECIFIED.);
#775=B_SPLINE_CURVE_WITH_KNOTS('',3,(#69474,#69475,#69476,#69477,#69478,
#69479,#69480,#69481,#69482,#69483,#69484,#69485,#69486,#69487,#69488,#69489,
#69490,#69491,#69492,#69493,#69494,#69495,#69496,#69497,#69498,#69499,#69500,
#69501,#69502,#69503,#69504,#69505,#69506,#69507,#69508,#69509,#69510,#69511,
#69512,#69513,#69514,#69515,#69516,#69517,#69518,#69519,#69520,#69521,#69522,
#69523,#69524,#69525,#69526,#69527,#69528,#69529,#69530,#69531,#69532,#69533,
#69534,#69535,#69536,#69537,#69538,#69539,#69540,#69541,#69542,#69543,#69544,
#69545,#69546,#69547,#69548,#69549,#69550,#69551,#69552,#69553,#69554,#69555,
#69556,#69557,#69558,#69559,#69560,#69561,#69562,#69563,#69564,#69565,#69566,
#69567,#69568,#69569,#69570,#69571,#69572,#69573,#69574,#69575,#69576,#69577,
#69578,#69579,#69580,#69581,#69582,#69583,#69584,#69585,#69586,#69587,#69588,
#69589,#69590,#69591,#69592,#69593,#69594,#69595,#69596,#69597,#69598,#69599,
#69600,#69601,#69602,#69603,#69604,#69605,#69606,#69607,#69608,#69609,#69610,
#69611,#69612,#69613,#69614,#69615,#69616,#69617,#69618,#69619,#69620,#69621,
#69622,#69623,#69624,#69625,#69626,#69627,#69628,#69629,#69630,#69631,#69632,
#69633,#69634,#69635,#69636,#69637,#69638,#69639,#69640,#69641,#69642,#69643,
#69644,#69645,#69646,#69647,#69648,#69649,#69650,#69651,#69652,#69653,#69654,
#69655,#69656,#69657,#69658,#69659,#69660,#69661,#69662,#69663,#69664,#69665,
#69666,#69667,#69668,#69669,#69670,#69671,#69672,#69673,#69674,#69675),
 .UNSPECIFIED.,.F.,.F.,(4,2,2,2,2,2,2,2,2,2,2,2,2,2,2,2,2,2,2,2,2,2,2,2,
2,2,2,2,2,2,2,2,2,2,2,2,2,2,2,2,2,2,2,2,2,2,2,2,2,2,2,2,2,2,2,2,2,2,2,2,
2,2,2,2,2,2,2,2,2,2,2,2,2,2,2,2,2,2,2,2,2,2,2,2,2,2,2,2,2,2,2,2,2,2,2,2,
2,2,2,2,4),(-1.49507327327653,-1.48719252098069,-1.48294770072824,-1.4820471916439,
-1.48178889420644,-1.47920758896041,-1.47633380858346,-1.47168614324768,
-1.45076975322874,-1.42986725872078,-1.42513502986856,-1.42245047904512,
-1.41877036451753,-1.41693274391433,-1.41558627954368,-1.41374842139644,
-1.41006710169774,-1.38662246729157,-1.36946824406393,-1.35906816612427,
-1.35518316866157,-1.35244602895658,-1.34997111299487,-1.34601923465861,
-1.33584610277006,-1.3098440644049,-1.29514873571344,-1.29145317741713,
-1.28961248262459,-1.28826585624641,-1.28643085055956,-1.28276429775505,
-1.25903540462543,-1.24205589907407,-1.23171946657212,-1.22784265048085,
-1.22510693153952,-1.22263043708772,-1.21930260098999,-1.2109449171727,
-1.1832097842105,-1.1679168915106,-1.1641548948865,-1.16230119974309,-1.16095395506262,
-1.15913111019459,-1.15563670988857,-1.13027411397566,-1.10745742306897,
-1.10203240215106,-1.09897858837553,-1.09632388415331,-1.0930198071695,
-1.08781314627094,-1.06209783310039,-1.04633310700028,-1.038273538192,-1.03581018759626,
-1.03422838210289,-1.0328268861638,-1.03049017518235,-1.0241072203025,-1.00115569565784,
-0.986285478260796,-0.979802921366489,-0.974558925310408,-0.971542578166978,
-0.968883328041537,-0.96552406304279,-0.95852936884663,-0.929152067421189,
-0.917385045935987,-0.910624556790516,-0.908305906554551,-0.906753810124901,
-0.905123836536867,-0.902438423913228,-0.892879961160621,-0.872328133412494,
-0.853150142875389,-0.847512280971532,-0.844414736372729,-0.841763167617778,
-0.838515332400218,-0.833501665825086,-0.802416151828116,-0.78459835702781,
-0.781598364052852,-0.779900307080142,-0.778380266438147,-0.776242377865235,
-0.770817587207459,-0.766217481918612,-0.746383883285741,-0.724225942957317,
-0.719446862083394,-0.716527783055549,-0.713846873982377,-0.710305397760907,
-0.702257557507502,-0.692976027751027),.UNSPECIFIED.);
#776=B_SPLINE_CURVE_WITH_KNOTS('',3,(#69676,#69677,#69678,#69679,#69680,
#69681,#69682,#69683,#69684,#69685,#69686,#69687,#69688,#69689,#69690,#69691,
#69692,#69693,#69694,#69695,#69696,#69697,#69698,#69699,#69700,#69701,#69702,
#69703,#69704,#69705,#69706,#69707,#69708,#69709,#69710,#69711,#69712,#69713,
#69714,#69715,#69716,#69717,#69718,#69719,#69720,#69721,#69722,#69723,#69724,
#69725,#69726,#69727,#69728,#69729,#69730,#69731,#69732,#69733,#69734,#69735,
#69736,#69737,#69738,#69739,#69740,#69741,#69742,#69743,#69744,#69745,#69746,
#69747,#69748,#69749,#69750,#69751,#69752,#69753,#69754,#69755,#69756,#69757,
#69758,#69759,#69760,#69761,#69762,#69763,#69764,#69765,#69766,#69767,#69768,
#69769,#69770,#69771,#69772,#69773,#69774,#69775,#69776,#69777,#69778,#69779,
#69780,#69781,#69782,#69783,#69784,#69785,#69786,#69787,#69788,#69789,#69790,
#69791,#69792,#69793,#69794,#69795,#69796,#69797,#69798,#69799,#69800,#69801,
#69802,#69803,#69804,#69805,#69806,#69807,#69808,#69809,#69810,#69811,#69812,
#69813,#69814,#69815,#69816,#69817,#69818,#69819,#69820,#69821,#69822,#69823,
#69824,#69825,#69826,#69827,#69828,#69829,#69830,#69831,#69832,#69833,#69834,
#69835,#69836,#69837,#69838,#69839,#69840,#69841,#69842,#69843,#69844,#69845,
#69846,#69847,#69848,#69849,#69850,#69851,#69852,#69853,#69854,#69855,#69856,
#69857,#69858,#69859,#69860,#69861,#69862,#69863,#69864,#69865,#69866,#69867,
#69868,#69869,#69870,#69871,#69872,#69873,#69874,#69875,#69876,#69877,#69878,
#69879,#69880,#69881,#69882,#69883,#69884,#69885,#69886,#69887,#69888,#69889,
#69890,#69891,#69892,#69893,#69894,#69895,#69896,#69897,#69898,#69899,#69900,
#69901),.UNSPECIFIED.,.F.,.F.,(4,2,2,2,2,2,2,2,2,2,2,2,2,2,2,2,2,2,2,2,
2,2,2,2,2,2,2,2,2,2,2,2,2,2,2,2,2,2,2,2,2,2,2,2,2,2,2,2,2,2,2,2,2,2,2,2,
2,2,2,2,2,2,2,2,2,2,2,2,2,2,2,2,2,2,2,2,2,2,2,2,2,2,2,2,2,2,2,2,2,2,2,2,
2,2,2,2,2,2,2,2,2,2,2,2,2,2,2,2,2,2,2,2,4),(-0.912009248555571,-0.910784402950638,
-0.909289046644602,-0.907422346554824,-0.903591713258842,-0.882622942337099,
-0.857892692021188,-0.851255179280141,-0.847962350316943,-0.845308909839391,
-0.842247992512888,-0.836933299051704,-0.802333453471668,-0.787610984940254,
-0.784657787469567,-0.782969996709953,-0.781446841166061,-0.779287586836242,
-0.773716390919297,-0.768935809769165,-0.747617142306819,-0.727253846121918,
-0.722511273796812,-0.719600305866127,-0.716917635026592,-0.71336012745137,
-0.705211181541947,-0.693420146087121,-0.67904876763235,-0.660381678101204,
-0.657367245038164,-0.655666310339294,-0.654147654559383,-0.652017195344845,
-0.646640210832553,-0.642097950440716,-0.62271479616597,-0.599971427264624,
-0.595198129747397,-0.592280650322297,-0.589599979112614,-0.586057015314614,
-0.577997536755071,-0.566392401900445,-0.551812633455501,-0.533043935000858,
-0.53002630190573,-0.52832465831336,-0.526806182118072,-0.524677088241117,
-0.519309368641465,-0.514778380556536,-0.495482268357733,-0.474541513180881,
-0.469279357003971,-0.465959198765666,-0.463303347276791,-0.46026106673824,
-0.454891853230435,-0.448205641016518,-0.432539871035909,-0.407339320875792,
-0.403703025399402,-0.401854091509433,-0.400339962391701,-0.398672142284213,
-0.395812135928608,-0.382046510061183,-0.353888352905454,-0.343586289635233,
-0.339616483537676,-0.337138440253632,-0.334404328575102,-0.330536312694538,
-0.320268342622186,-0.29804531061308,-0.279761385634922,-0.275873065846176,
-0.273995136821017,-0.272499545497755,-0.270625349663056,-0.266756620995827,
-0.261463127026102,-0.246545373619972,-0.21961422785916,-0.214458269126216,
-0.211168935827046,-0.208515285377035,-0.205450776133082,-0.199973740285639,
-0.196244968139523,-0.18508846049105,-0.169931499658724,-0.15240719746132,
-0.148521090343444,-0.146643609415607,-0.145148054534646,-0.145134231998255,
-0.145121479732626,-0.145109713107917,-0.145091632015426,-0.145073850816049,
-0.145056362665238,-0.14503916083859,-0.145022238806452,-0.145005590256122,
-0.144989208963482,-0.144973088953973,-0.143073896434872,-0.13890559370743,
-0.132998811702847,-0.114716118291897,-0.109835420218483),.UNSPECIFIED.);
#777=B_SPLINE_CURVE_WITH_KNOTS('',3,(#69907,#69908,#69909,#69910,#69911,
#69912,#69913,#69914,#69915),.UNSPECIFIED.,.F.,.F.,(4,1,1,1,1,1,4),(59.690260418206,
60.2097426832351,61.2072492651971,62.2047558471591,63.2022624291211,64.1997690110831,
65.1147889235391),.UNSPECIFIED.);
#778=B_SPLINE_CURVE_WITH_KNOTS('',3,(#69916,#69917,#69918,#69919,#69920,
#69921,#69922,#69923,#69924,#69925,#69926,#69927,#69928,#69929,#69930,#69931,
#69932,#69933,#69934,#69935,#69936,#69937,#69938,#69939,#69940,#69941),
 .UNSPECIFIED.,.F.,.F.,(4,2,2,2,2,2,2,2,2,2,2,2,4),(-1.60461039696953,-1.60200406463946,
-1.59780060604424,-1.57558491424115,-1.55491332420186,-1.54748189968155,
-1.54508526809245,-1.54351756503159,-1.54190967647936,-1.53932531048012,
-1.53085774882649,-1.50084484460034,-1.49507327327653),.UNSPECIFIED.);
#779=B_SPLINE_CURVE_WITH_KNOTS('',3,(#69943,#69944,#69945,#69946,#69947,
#69948,#69949,#69950,#69951,#69952,#69953,#69954,#69955,#69956,#69957,#69958,
#69959,#69960,#69961,#69962,#69963,#69964,#69965,#69966,#69967,#69968,#69969,
#69970,#69971,#69972,#69973,#69974,#69975,#69976),.UNSPECIFIED.,.F.,.F.,
(4,2,2,2,2,2,2,2,2,2,2,2,2,2,2,2,4),(-0.109835420218483,-0.0924745669060319,
-0.0872107663617741,-0.0838901580985834,-0.0812343057745877,-0.0781924148245023,
-0.0750033992623017,-0.061516621270222,-0.0474361001445638,-0.0299384713519545,
-0.0225781465623608,-0.0201139955418309,-0.0186887094877936,-0.0172787991718988,
-0.0157260016506987,-0.0135557476351094,-0.000374706389804315),
 .UNSPECIFIED.);
#780=B_SPLINE_CURVE_WITH_KNOTS('',3,(#69977,#69978,#69979,#69980,#69981,
#69982,#69983,#69984,#69985,#69986,#69987,#69988,#69989,#69990,#69991,#69992,
#69993,#69994,#69995,#69996,#69997,#69998,#69999,#70000,#70001,#70002,#70003,
#70004,#70005,#70006,#70007,#70008,#70009,#70010,#70011,#70012,#70013,#70014,
#70015,#70016,#70017,#70018,#70019,#70020,#70021,#70022,#70023,#70024,#70025,
#70026,#70027,#70028,#70029,#70030,#70031,#70032,#70033,#70034,#70035,#70036,
#70037,#70038,#70039,#70040,#70041,#70042,#70043,#70044,#70045,#70046,#70047,
#70048,#70049,#70050,#70051,#70052,#70053,#70054,#70055,#70056,#70057,#70058,
#70059,#70060,#70061,#70062,#70063,#70064,#70065,#70066,#70067,#70068,#70069,
#70070,#70071,#70072,#70073,#70074,#70075,#70076,#70077,#70078,#70079,#70080,
#70081,#70082,#70083,#70084,#70085,#70086,#70087,#70088,#70089,#70090,#70091,
#70092,#70093,#70094,#70095,#70096,#70097,#70098,#70099,#70100,#70101,#70102,
#70103,#70104,#70105,#70106,#70107,#70108,#70109,#70110,#70111,#70112,#70113,
#70114,#70115,#70116,#70117,#70118,#70119,#70120,#70121,#70122,#70123,#70124,
#70125,#70126,#70127,#70128,#70129,#70130,#70131,#70132,#70133,#70134,#70135,
#70136,#70137,#70138,#70139,#70140,#70141,#70142,#70143,#70144),
 .UNSPECIFIED.,.F.,.F.,(4,2,2,2,2,2,2,2,2,2,2,2,2,2,2,2,2,2,2,2,2,2,2,2,
2,2,2,2,2,2,2,2,2,2,2,2,2,2,2,2,2,2,2,2,2,2,2,2,2,2,2,2,2,2,2,2,2,2,2,2,
2,2,2,2,2,2,2,2,2,2,2,2,2,2,2,2,2,2,2,2,2,2,2,4),(-1.60478364820448,-1.57115448853031,
-1.56635300154545,-1.56321387126241,-1.56020659854018,-1.5575477017934,
-1.55417855953096,-1.54874276073197,-1.51825690335156,-1.5062124376139,
-1.50154189002089,-1.49902450528996,-1.4969785366282,-1.49550094237346,
-1.49408266666979,-1.4916529469648,-1.48457165850096,-1.45311605841662,
-1.43925390729897,-1.43499091462708,-1.43218068451344,-1.42948235261338,
-1.42565685690423,-1.41637553110808,-1.38953899675086,-1.37455458675071,
-1.37082748447105,-1.36898112650074,-1.36763485471576,-1.36580697276272,
-1.36217406317925,-1.33785388788463,-1.31342209163813,-1.30840985105733,
-1.30544298884162,-1.30277673980584,-1.29933828806008,-1.29365777363457,
-1.26048375949418,-1.24581753131842,-1.24292066522155,-1.24124532974193,
-1.23971798647798,-1.23753123862588,-1.23215100308795,-1.20835597851232,
-1.1931707862611,-1.18352613860254,-1.17974369018884,-1.17702561955487,
-1.17419654673821,-1.16984309552342,-1.15622264911892,-1.12860700237905,
-1.1180834423465,-1.1154096542646,-1.11378261507004,-1.11224801931406,-1.10993826485808,
-1.10373299486374,-1.08063609601986,-1.06571065011332,-1.05921431399649,
-1.05396209768192,-1.05094464888596,-1.04828655012033,-1.04493161547065,
-1.03954686131757,-1.00898348915641,-0.996918994379538,-0.990051595207271,
-0.987720418930485,-0.986166194615606,-0.984740923599546,-0.982275776062266,
-0.9749031956904,-0.952741745009379,-0.938177046670485,-0.92878641440501,
-0.925039659073643,-0.922327497260759,-0.919825768727951,-0.915718712436704,
-0.912212879656785),.UNSPECIFIED.);
#781=B_SPLINE_CURVE_WITH_KNOTS('',3,(#70150,#70151,#70152,#70153,#70154,
#70155,#70156,#70157,#70158,#70159,#70160,#70161,#70162,#70163,#70164,#70165,
#70166,#70167,#70168,#70169,#70170,#70171,#70172,#70173,#70174,#70175,#70176,
#70177,#70178,#70179,#70180,#70181,#70182,#70183,#70184,#70185,#70186,#70187,
#70188,#70189,#70190,#70191,#70192,#70193,#70194,#70195,#70196,#70197,#70198,
#70199,#70200,#70201,#70202,#70203,#70204,#70205,#70206,#70207,#70208,#70209,
#70210,#70211,#70212,#70213,#70214,#70215,#70216,#70217,#70218,#70219,#70220,
#70221,#70222,#70223,#70224,#70225,#70226,#70227,#70228,#70229,#70230,#70231,
#70232,#70233,#70234,#70235,#70236,#70237,#70238,#70239,#70240,#70241,#70242,
#70243,#70244,#70245,#70246,#70247,#70248,#70249,#70250,#70251,#70252,#70253,
#70254,#70255,#70256,#70257,#70258,#70259,#70260,#70261,#70262,#70263,#70264,
#70265,#70266,#70267,#70268,#70269,#70270,#70271,#70272,#70273,#70274,#70275,
#70276,#70277,#70278,#70279,#70280,#70281,#70282,#70283,#70284,#70285,#70286,
#70287,#70288,#70289,#70290,#70291,#70292,#70293,#70294,#70295,#70296,#70297),
 .UNSPECIFIED.,.F.,.F.,(4,3,3,3,3,3,3,3,3,3,3,3,3,3,3,3,3,3,3,3,3,3,3,3,
3,3,3,3,3,3,3,3,3,3,3,3,3,3,3,3,3,3,3,3,3,3,3,3,3,4),(65.9734457253856,
66.133557022025,66.1947821750071,66.3122857663604,66.4295731536894,66.546741452997,
66.6638406433999,66.7809205913324,66.8981149294539,67.0153723379108,67.1328487102704,
67.1922887569691,67.3097923483223,67.4270797356512,67.5442480349588,67.6613472253615,
67.778427173294,67.8956215114154,68.0128789198722,68.1303552922317,68.189795338931,
68.3072989302843,68.4245863176133,68.5417546169209,68.6588538073237,68.7759337552562,
68.8931280933777,69.0103855018346,69.1278618741942,69.187301920893,69.3048055122463,
69.4220928995753,69.5392611988829,69.6563603892858,69.7734403372183,69.8906346753398,
70.0078920837967,70.1253684561562,70.184808502855,70.3023120942082,70.4195994815371,
70.5367677808447,70.6538669712475,70.77094691918,70.8881412573014,71.0053986657582,
71.1228750381177,71.182315084817,71.2997780450628,71.3990564536364),
 .UNSPECIFIED.);
#782=B_SPLINE_CURVE_WITH_KNOTS('',3,(#70298,#70299,#70300,#70301,#70302),
 .UNSPECIFIED.,.F.,.F.,(4,1,4),(65.1147889235391,65.1972755930451,65.9734445059395),
 .UNSPECIFIED.);
#783=B_SPLINE_CURVE_WITH_KNOTS('',3,(#70303,#70304,#70305,#70306,#70307,
#70308,#70309,#70310,#70311,#70312,#70313,#70314,#70315,#70316,#70317,#70318,
#70319,#70320,#70321,#70322,#70323,#70324,#70325,#70326,#70327,#70328,#70329,
#70330,#70331,#70332,#70333,#70334,#70335,#70336,#70337,#70338,#70339,#70340,
#70341,#70342,#70343,#70344,#70345,#70346,#70347,#70348,#70349,#70350,#70351,
#70352,#70353,#70354,#70355,#70356,#70357,#70358,#70359,#70360,#70361,#70362,
#70363,#70364,#70365,#70366,#70367,#70368,#70369,#70370,#70371,#70372,#70373,
#70374,#70375,#70376,#70377,#70378,#70379,#70380,#70381,#70382,#70383,#70384,
#70385,#70386,#70387,#70388,#70389,#70390,#70391,#70392,#70393,#70394,#70395,
#70396,#70397,#70398,#70399,#70400,#70401,#70402,#70403,#70404,#70405,#70406,
#70407,#70408,#70409,#70410,#70411,#70412,#70413,#70414,#70415,#70416,#70417,
#70418,#70419,#70420,#70421,#70422,#70423,#70424,#70425,#70426,#70427,#70428,
#70429,#70430,#70431,#70432,#70433,#70434,#70435,#70436,#70437,#70438,#70439,
#70440,#70441,#70442,#70443,#70444,#70445,#70446,#70447,#70448,#70449,#70450,
#70451,#70452,#70453,#70454,#70455,#70456,#70457,#70458,#70459,#70460,#70461,
#70462,#70463,#70464,#70465,#70466,#70467,#70468,#70469,#70470,#70471,#70472,
#70473,#70474,#70475,#70476,#70477,#70478,#70479,#70480,#70481,#70482,#70483,
#70484,#70485,#70486,#70487,#70488,#70489,#70490,#70491,#70492,#70493,#70494,
#70495,#70496,#70497,#70498,#70499,#70500,#70501,#70502,#70503,#70504,#70505,
#70506,#70507,#70508,#70509,#70510,#70511,#70512,#70513,#70514,#70515,#70516),
 .UNSPECIFIED.,.F.,.F.,(4,2,2,2,2,2,2,2,2,2,2,2,2,2,2,2,2,2,2,2,2,2,2,2,
2,2,2,2,2,2,2,2,2,2,2,2,2,2,2,2,2,2,2,2,2,2,2,2,2,2,2,2,2,2,2,2,2,2,2,2,
2,2,2,2,2,2,2,2,2,2,2,2,2,2,2,2,2,2,2,2,2,2,2,2,2,2,2,2,2,2,2,2,2,2,2,2,
2,2,2,2,2,2,2,2,2,2,4),(-0.912212879656785,-0.904371023607735,-0.874306003962147,
-0.863460301095778,-0.860763645895146,-0.859131476399047,-0.857599657718553,
-0.855677862819302,-0.850732756831442,-0.81681297279783,-0.802644312257033,
-0.798352856704789,-0.795536211207104,-0.792809628977875,-0.788981056755466,
-0.77900505257007,-0.762980505090563,-0.737558646023001,-0.734067190034405,
-0.732245167146209,-0.73089814192859,-0.729044322108487,-0.725280651839922,
-0.70997001926422,-0.682171892283217,-0.673899944774947,-0.670586203926304,
-0.668113286334403,-0.6653747036933,-0.661480597784054,-0.651009109632286,
-0.633656527188981,-0.610502002417735,-0.606789446568505,-0.60494556068299,
-0.603449632879506,-0.601540053871971,-0.597482183921184,-0.59183827278793,
-0.575073595157904,-0.550799656332624,-0.545560952547799,-0.542247835313155,
-0.539592858237777,-0.536546390060784,-0.531155599761763,-0.524433982851252,
-0.508624802674593,-0.482798063832198,-0.479351863405705,-0.47753936378189,
-0.47605587827031,-0.474116912829285,-0.469898755145193,-0.463951470801384,
-0.445421494855018,-0.423541019803515,-0.418257253800974,-0.414930997133296,
-0.412274861624346,-0.409237239261976,-0.403889774184179,-0.397238729715074,
-0.374475878611681,-0.373538116545626,-0.354661842154876,-0.351675452247035,
-0.34996339990879,-0.348448161193592,-0.346340641175164,-0.341114116742738,
-0.333103969458632,-0.315874414649614,-0.294292184712198,-0.289493868571186,
-0.286571105885082,-0.283892023278006,-0.280360677471308,-0.272371971044671,
-0.260912639243567,-0.246179196378392,-0.227321233872595,-0.224335396498194,
-0.22262343337322,-0.221108102011787,-0.219000219591661,-0.213771625021999,
-0.205757062073263,-0.18861438593341,-0.166965720783982,-0.162159427933233,
-0.159234922758008,-0.156556243405086,-0.156505138420624,-0.156459189880959,
-0.156417850125568,-0.156380634240671,-0.156347112193308,-0.156316902003047,
-0.156289663828868,-0.156265094916364,-0.156201398460163,-0.152846107066361,
-0.144582070318634,-0.132469209821949,-0.118242870080311,-0.110044856416793),
 .UNSPECIFIED.);
#784=B_SPLINE_CURVE_WITH_KNOTS('',3,(#70522,#70523,#70524,#70525,#70526,
#70527,#70528,#70529,#70530,#70531,#70532,#70533,#70534,#70535,#70536,#70537,
#70538,#70539,#70540,#70541,#70542,#70543,#70544,#70545,#70546,#70547,#70548,
#70549,#70550,#70551,#70552,#70553,#70554,#70555,#70556,#70557,#70558,#70559,
#70560,#70561,#70562,#70563,#70564,#70565,#70566,#70567,#70568,#70569,#70570,
#70571,#70572,#70573,#70574,#70575,#70576,#70577,#70578,#70579,#70580,#70581,
#70582,#70583,#70584,#70585,#70586,#70587,#70588,#70589,#70590,#70591,#70592,
#70593,#70594,#70595,#70596,#70597,#70598,#70599,#70600,#70601,#70602,#70603,
#70604,#70605,#70606,#70607,#70608,#70609,#70610,#70611,#70612,#70613,#70614,
#70615,#70616,#70617,#70618,#70619,#70620,#70621,#70622,#70623,#70624,#70625,
#70626,#70627,#70628,#70629,#70630,#70631,#70632,#70633,#70634,#70635,#70636,
#70637,#70638,#70639,#70640,#70641,#70642,#70643,#70644,#70645,#70646,#70647,
#70648,#70649,#70650,#70651,#70652,#70653,#70654,#70655,#70656,#70657,#70658,
#70659,#70660,#70661,#70662,#70663,#70664,#70665,#70666,#70667,#70668,#70669,
#70670,#70671,#70672,#70673,#70674,#70675,#70676,#70677,#70678,#70679,#70680,
#70681,#70682,#70683,#70684,#70685,#70686,#70687,#70688,#70689,#70690,#70691,
#70692,#70693,#70694,#70695,#70696,#70697,#70698,#70699,#70700,#70701,#70702,
#70703,#70704,#70705,#70706,#70707,#70708,#70709,#70710,#70711,#70712,#70713),
 .UNSPECIFIED.,.F.,.F.,(4,2,2,2,2,2,2,2,2,2,2,2,2,2,2,2,2,2,2,2,2,2,2,2,
2,2,2,2,2,2,2,2,2,2,2,2,2,2,2,2,2,2,2,2,2,2,2,2,2,2,2,2,2,2,2,2,2,2,2,2,
2,2,2,2,2,2,2,2,2,2,2,2,2,2,2,2,2,2,2,2,2,2,2,2,2,2,2,2,2,2,2,2,2,2,2,4),
(-0.69301358421698,-0.692651839720984,-0.689997439699259,-0.68694559874889,
-0.681528636664272,-0.674764223940749,-0.658780911705467,-0.633293456051878,
-0.629810067409437,-0.627989707350097,-0.626642519687764,-0.624786662532745,
-0.621012692447938,-0.605607129871799,-0.577522375407419,-0.56953077172595,
-0.566262071179798,-0.563553257195185,-0.560755589122205,-0.55655815072856,
-0.543401469059281,-0.516228515719477,-0.504734770090803,-0.501919654233641,
-0.500261671577866,-0.49872574929122,-0.496492062971919,-0.490390835768222,
-0.480343646828524,-0.445788418525292,-0.440472968659646,-0.437411809619531,
-0.434758236749855,-0.431465325104831,-0.42482799887066,-0.396265834611555,
-0.377728404492275,-0.374717728866283,-0.373017625702815,-0.371498731206136,
-0.369366539035901,-0.363977739667874,-0.359420975068708,-0.339922934576411,
-0.319206360071356,-0.313970189202,-0.310657650025399,-0.308002484140076,
-0.304955068711174,-0.299560535638158,-0.292832920138985,-0.276999533907002,
-0.251226283849575,-0.247774474934284,-0.245960688112422,-0.244477141256913,
-0.242539318569282,-0.23832804645846,-0.232393990958186,-0.21394425479506,
-0.191950651278511,-0.186675840411542,-0.183352016030964,-0.180695844430751,
-0.177656015967709,-0.172298729586701,-0.168678963246298,-0.162811409843366,
-0.14060334161294,-0.123121664605095,-0.120122388135064,-0.118407363266069,
-0.1169410962558,-0.116912876081689,-0.116885059993081,-0.116857609770681,
-0.116830489399522,-0.11680366485246,-0.116777103751712,-0.116750775342384,
-0.116724650321081,-0.116698700532801,-0.116672898932253,-0.116647219376421,
-0.114611867096337,-0.112104789323589,-0.107463970549589,-0.0955484402159176,
-0.0655653205561749,-0.0592040382829809,-0.055922620910389,-0.0532693913354477,
-0.0501987205217863,-0.0446919243745535,-0.0377807281459007,-0.000375412795531045),
 .UNSPECIFIED.);
#785=B_SPLINE_CURVE_WITH_KNOTS('',3,(#70714,#70715,#70716,#70717,#70718,
#70719,#70720,#70721,#70722,#70723,#70724,#70725,#70726,#70727,#70728,#70729,
#70730,#70731,#70732,#70733,#70734,#70735,#70736,#70737,#70738),
 .UNSPECIFIED.,.F.,.F.,(4,3,3,3,3,3,3,3,4),(71.3990564536364,71.5162398299033,
71.6333464109936,71.750426076489,71.8676146843092,71.9848594751022,72.1023289823989,
72.179821666779,72.2566310325652),.UNSPECIFIED.);
#786=B_SPLINE_CURVE_WITH_KNOTS('',3,(#70740,#70741,#70742,#70743,#70744,
#70745,#70746,#70747,#70748,#70749,#70750,#70751,#70752,#70753,#70754,#70755,
#70756,#70757,#70758,#70759,#70760,#70761,#70762,#70763,#70764,#70765,#70766,
#70767,#70768,#70769,#70770,#70771,#70772,#70773),.UNSPECIFIED.,.F.,.F.,
(4,2,2,2,2,2,2,2,2,2,2,2,2,2,2,2,4),(-0.110044856416793,-0.0999516129579047,
-0.0969458658991607,-0.0952467203932099,-0.0937273466900666,-0.0922007675905067,
-0.088597535396166,-0.0812378620567708,-0.060149807966156,-0.0395065387801758,
-0.0347576557653405,-0.0318451886373184,-0.0291626819211827,-0.0265368828350931,
-0.0230751872387385,-0.0156249266252038,-0.000374946432257026),
 .UNSPECIFIED.);
#787=B_SPLINE_CURVE_WITH_KNOTS('',3,(#70774,#70775,#70776,#70777,#70778,
#70779,#70780,#70781,#70782,#70783),.UNSPECIFIED.,.F.,.F.,(4,1,1,1,1,1,
1,4),(72.256633207435,72.5146276293805,73.5121342113425,74.5096407933045,
75.5071473752665,76.5046539572285,77.5021605391904,77.6824992212595),
 .UNSPECIFIED.);
#788=B_SPLINE_CURVE_WITH_KNOTS('',3,(#70788,#70789,#70790,#70791,#70792,
#70793,#70794,#70795,#70796,#70797,#70798,#70799,#70800,#70801,#70802,#70803,
#70804,#70805,#70806,#70807,#70808,#70809,#70810,#70811,#70812,#70813,#70814,
#70815,#70816,#70817,#70818,#70819,#70820,#70821,#70822,#70823,#70824,#70825,
#70826,#70827,#70828,#70829,#70830,#70831,#70832,#70833,#70834,#70835,#70836,
#70837,#70838,#70839,#70840,#70841,#70842,#70843,#70844,#70845,#70846,#70847,
#70848,#70849,#70850,#70851,#70852,#70853,#70854,#70855,#70856,#70857,#70858,
#70859,#70860,#70861,#70862,#70863,#70864,#70865,#70866,#70867,#70868,#70869,
#70870,#70871,#70872,#70873,#70874,#70875,#70876,#70877,#70878,#70879,#70880,
#70881,#70882,#70883,#70884,#70885,#70886,#70887,#70888,#70889,#70890,#70891,
#70892,#70893,#70894,#70895,#70896,#70897,#70898,#70899,#70900,#70901,#70902,
#70903,#70904,#70905,#70906,#70907,#70908,#70909,#70910,#70911,#70912,#70913,
#70914,#70915,#70916,#70917,#70918,#70919,#70920,#70921,#70922,#70923,#70924,
#70925,#70926,#70927,#70928,#70929,#70930,#70931,#70932,#70933,#70934,#70935,
#70936,#70937,#70938,#70939,#70940,#70941,#70942,#70943,#70944,#70945,#70946,
#70947,#70948,#70949,#70950,#70951,#70952,#70953,#70954,#70955,#70956,#70957,
#70958,#70959,#70960,#70961,#70962,#70963,#70964,#70965,#70966,#70967,#70968,
#70969,#70970,#70971,#70972,#70973,#70974,#70975,#70976,#70977,#70978,#70979,
#70980,#70981,#70982,#70983,#70984,#70985,#70986,#70987,#70988,#70989,#70990,
#70991,#70992,#70993,#70994,#70995,#70996,#70997),.UNSPECIFIED.,.F.,.F.,
(4,2,2,2,2,2,2,2,2,2,2,2,2,2,2,2,2,2,2,2,2,2,2,2,2,2,2,2,2,2,2,2,2,2,2,
2,2,2,2,2,2,2,2,2,2,2,2,2,2,2,2,2,2,2,2,2,2,2,2,2,2,2,2,2,2,2,2,2,2,2,2,
2,2,2,2,2,2,2,2,2,2,2,2,2,2,2,2,2,2,2,2,2,2,2,2,2,2,2,2,2,2,2,2,2,4),(-1.49489110793716,
-1.48851040879273,-1.4815898616485,-1.46911976787942,-1.46330136573139,
-1.45975864243683,-1.45653421167254,-1.45643215106401,-1.45631773706341,
-1.45626507241238,-1.4561656573116,-1.45597971139256,-1.45422673620739,
-1.45130121023412,-1.4464882301232,-1.42476291827683,-1.40462053524107,
-1.39998137273359,-1.39452557009446,-1.3923834918489,-1.39086324111583,
-1.38916804628255,-1.38617973320417,-1.36999707459897,-1.3474561383648,
-1.33465279488333,-1.33049113140621,-1.32770080481675,-1.32498678840093,
-1.32107757767587,-1.31121166510398,-1.2849274715219,-1.2701344794187,-1.26642823951693,
-1.26458562220613,-1.26308967815517,-1.26117870018267,-1.25711307255161,
-1.23198765055204,-1.21635515041228,-1.20967825166179,-1.20431433655919,
-1.20127347739827,-1.19861792781786,-1.1952968919721,-1.19003061365599,
-1.16891656839967,-1.14974347581927,-1.14522828139264,-1.13987431459827,
-1.13774747125555,-1.13622952878083,-1.13452714947313,-1.13150539284095,
-1.11261184818741,-1.09780820284829,-1.08645208681706,-1.07851331677216,
-1.07499059162102,-1.07231295798725,-1.06938677477583,-1.06457109503359,
-1.04282597521714,-1.02270129219182,-1.01806423800433,-1.01261008017155,
-1.01046818500423,-1.00894790785714,-1.00725250510562,-1.00426344994474,
-0.988031737189969,-0.965526664071109,-0.952732955666407,-0.948572140588679,
-0.945781892831736,-0.943067587007926,-0.939157306054541,-0.929283382176771,
-0.903004796771474,-0.892066615130021,-0.885616074874488,-0.883336533471173,
-0.881792225656302,-0.880150375395943,-0.877409292505431,-0.867133189761485,
-0.838886489321326,-0.825531915485326,-0.821315606433368,-0.818514221513337,
-0.815808310668869,-0.8119440112042,-0.802457429459729,-0.787203173805783,
-0.763230843010317,-0.758031460640131,-0.756082502699792,-0.754682122929671,
-0.753099385250855,-0.750630871632608,-0.742516188656957,-0.726556737874347,
-0.701170071687919,-0.695957382235664,-0.69301358421698),.UNSPECIFIED.);
#789=B_SPLINE_CURVE_WITH_KNOTS('',3,(#70999,#71000,#71001,#71002,#71003),
 .UNSPECIFIED.,.F.,.F.,(4,1,4),(77.6824992212595,78.4996671211524,78.5398163397448),
 .UNSPECIFIED.);
#790=B_SPLINE_CURVE_WITH_KNOTS('',3,(#71004,#71005,#71006,#71007,#71008,
#71009,#71010,#71011,#71012,#71013,#71014,#71015,#71016,#71017,#71018,#71019,
#71020,#71021,#71022,#71023,#71024,#71025,#71026,#71027,#71028,#71029,#71030,
#71031,#71032,#71033,#71034,#71035,#71036,#71037,#71038,#71039,#71040,#71041,
#71042,#71043,#71044,#71045,#71046,#71047,#71048,#71049,#71050,#71051,#71052,
#71053,#71054,#71055,#71056,#71057,#71058,#71059,#71060,#71061,#71062,#71063,
#71064,#71065,#71066,#71067,#71068,#71069,#71070,#71071,#71072,#71073,#71074,
#71075,#71076,#71077,#71078,#71079,#71080,#71081,#71082,#71083,#71084,#71085,
#71086,#71087,#71088,#71089,#71090,#71091,#71092,#71093,#71094,#71095,#71096,
#71097,#71098,#71099,#71100,#71101,#71102,#71103,#71104,#71105,#71106,#71107,
#71108,#71109,#71110,#71111,#71112,#71113,#71114,#71115,#71116,#71117,#71118,
#71119,#71120,#71121,#71122,#71123,#71124,#71125,#71126,#71127,#71128,#71129,
#71130,#71131,#71132,#71133,#71134,#71135,#71136,#71137,#71138,#71139,#71140,
#71141,#71142,#71143,#71144,#71145,#71146,#71147,#71148,#71149,#71150,#71151,
#71152,#71153,#71154,#71155,#71156,#71157,#71158,#71159,#71160,#71161,#71162,
#71163,#71164,#71165,#71166,#71167,#71168,#71169,#71170,#71171,#71172,#71173,
#71174,#71175,#71176,#71177,#71178,#71179,#71180,#71181,#71182,#71183,#71184,
#71185,#71186,#71187,#71188,#71189,#71190,#71191,#71192,#71193,#71194,#71195,
#71196,#71197,#71198,#71199,#71200,#71201,#71202,#71203,#71204,#71205,#71206,
#71207,#71208,#71209,#71210,#71211,#71212,#71213,#71214,#71215,#71216,#71217,
#71218,#71219,#71220,#71221,#71222,#71223,#71224,#71225,#71226,#71227,#71228,
#71229),.UNSPECIFIED.,.F.,.F.,(4,2,2,2,2,2,2,2,2,2,2,2,2,2,2,2,2,2,2,2,
2,2,2,2,2,2,2,2,2,2,2,2,2,2,2,2,2,2,2,2,2,2,2,2,2,2,2,2,2,2,2,2,2,2,2,2,
2,2,2,2,2,2,2,2,2,2,2,2,2,2,2,2,2,2,2,2,2,2,2,2,2,2,2,2,2,2,2,2,2,2,2,2,
2,2,2,2,2,2,2,2,2,2,2,2,2,2,2,2,2,2,2,2,4),(-1.6048292035244,-1.59977016780302,
-1.58369609630493,-1.56532874704923,-1.55717465345672,-1.55093370317585,
-1.54771677533232,-1.54532523492503,-1.54230190317608,-1.53715853994253,
-1.52985404874484,-1.50360614078768,-1.48882453445654,-1.48618944707944,
-1.48404047097112,-1.48400618512232,-1.48397210208206,-1.48393818271339,
-1.48390438758405,-1.48387067670807,-1.48383700946711,-1.48380334434472,
-1.48376963865202,-1.48373584836451,-1.48370192782456,-1.48366782941582,
-1.48363350321742,-1.48359889658574,-1.4835639537953,-1.48352861554711,
-1.48351226427847,-1.48349456571752,-1.48347534461706,-1.483454392456,-1.48343145888499,
-1.48340624008951,-1.48337836303173,-1.4833473637114,-1.48331265593475,
-1.48327348604044,-1.483228864582,-1.48178632787584,-1.47987800423348,-1.47607785317775,
-1.45861624182952,-1.4435051744279,-1.43232140124349,-1.42858586549684,
-1.42310130926748,-1.42003563270498,-1.41738262651398,-1.4140962314904,
-1.40894915091509,-1.38183228838697,-1.36701262699752,-1.36173867674794,
-1.35788130004178,-1.35600947324365,-1.35451414372993,-1.352634498102,-1.34873605710163,
-1.32868801370663,-1.31767133521675,-1.30560431244284,-1.29732319936252,
-1.29374462308699,-1.29105909868377,-1.28815749128966,-1.28345866517345,
-1.27504977123215,-1.24890771844801,-1.23416232697371,-1.23046119416122,
-1.22861950041388,-1.227272955156,-1.22543929882858,-1.22177914054929,-1.19789922684563,
-1.18100947473718,-1.17070589808303,-1.16683355125372,-1.16409883109408,
-1.16162183084412,-1.15765727761269,-1.14739249045719,-1.11711709508438,
-1.10906575684174,-1.10382104466066,-1.10171070130384,-1.10019507853645,
-1.09848443107537,-1.09550434949171,-1.07682833895893,-1.06241912056978,
-1.05068395189443,-1.04256076877221,-1.03900746110207,-1.03632533882571,
-1.03341243455468,-1.02866090998084,-1.00793103249446,-0.986884379719522,
-0.982134528404293,-0.976588426122863,-0.97443276454899,-0.972910167875554,
-0.971220686528546,-0.968259849336341,-0.953297302979803,-0.929783491563662,
-0.916717145604933,-0.912528510920155,-0.912282028493777),.UNSPECIFIED.);
#791=B_SPLINE_CURVE_WITH_KNOTS('',3,(#71235,#71236,#71237,#71238,#71239,
#71240,#71241,#71242,#71243,#71244,#71245,#71246,#71247,#71248,#71249,#71250,
#71251,#71252,#71253,#71254,#71255,#71256,#71257,#71258,#71259,#71260,#71261,
#71262,#71263,#71264,#71265,#71266,#71267,#71268,#71269,#71270,#71271,#71272,
#71273,#71274,#71275,#71276,#71277,#71278,#71279,#71280,#71281,#71282,#71283,
#71284,#71285,#71286,#71287,#71288,#71289,#71290,#71291,#71292,#71293,#71294,
#71295,#71296,#71297,#71298,#71299,#71300,#71301,#71302,#71303,#71304,#71305,
#71306,#71307,#71308,#71309,#71310,#71311,#71312,#71313,#71314,#71315,#71316,
#71317,#71318,#71319,#71320,#71321,#71322,#71323,#71324,#71325,#71326,#71327,
#71328,#71329,#71330,#71331,#71332,#71333,#71334,#71335,#71336,#71337,#71338,
#71339,#71340,#71341,#71342,#71343,#71344,#71345,#71346,#71347,#71348,#71349,
#71350,#71351,#71352,#71353,#71354,#71355,#71356,#71357,#71358,#71359,#71360,
#71361,#71362,#71363,#71364,#71365,#71366,#71367,#71368,#71369,#71370,#71371,
#71372,#71373,#71374,#71375,#71376,#71377,#71378,#71379,#71380,#71381,#71382,
#71383,#71384,#71385,#71386,#71387,#71388,#71389,#71390,#71391,#71392,#71393,
#71394,#71395,#71396,#71397,#71398,#71399,#71400,#71401,#71402,#71403,#71404,
#71405,#71406,#71407,#71408,#71409,#71410,#71411,#71412),.UNSPECIFIED.,
 .F.,.F.,(4,2,2,2,2,2,2,2,2,2,2,2,2,2,2,2,2,2,2,2,2,2,2,2,2,2,2,2,2,2,2,
2,2,2,2,2,2,2,2,2,2,2,2,2,2,2,2,2,2,2,2,2,2,2,2,2,2,2,2,2,2,2,2,2,2,2,2,
2,2,2,2,2,2,2,2,2,2,2,2,2,2,2,2,2,2,2,2,2,4),(-0.693006869784502,-0.683654895915191,
-0.680632241890465,-0.67892916620703,-0.677410422659474,-0.675282285877349,
-0.669923812895553,-0.665404567543853,-0.646201277630175,-0.625122720119772,
-0.619867266461999,-0.616548442518697,-0.613891862921112,-0.61084677504362,
-0.605467160615383,-0.584062758715741,-0.560645558149656,-0.554787517645369,
-0.552523173264645,-0.550996404234677,-0.5493531378566,-0.546608003167671,
-0.535028882294789,-0.499892492568089,-0.492685423233125,-0.489287528570774,
-0.48662397875073,-0.483630296632608,-0.478497087801861,-0.475078931304347,
-0.465150603687295,-0.448547445733901,-0.430313633403777,-0.426425137698383,
-0.424546883634213,-0.423050892590864,-0.421175971196141,-0.417304964550807,
-0.412007668153858,-0.397072685306411,-0.370166859036,-0.365008821866856,
-0.361718427598524,-0.359064063480933,-0.355998869004036,-0.350520929986073,
-0.346791624930591,-0.335633632963646,-0.320476656624734,-0.301529826584575,
-0.298505458805393,-0.296802076892572,-0.295283547217215,-0.293156376862039,
-0.287803803991192,-0.28329158080209,-0.264140945808024,-0.241107310771599,
-0.236327661557132,-0.233408254661632,-0.230727056925715,-0.227185217835719,
-0.219136639401312,-0.207555124624643,-0.192947515188004,-0.174163353272465,
-0.171144582805802,-0.169442370902138,-0.167923417592538,-0.165793643794449,
-0.160424045492456,-0.155891272854231,-0.136583959723365,-0.11372975454215,
-0.108960302987224,-0.106042996823378,-0.103477221228301,-0.100170748419366,
-0.0930081796813826,-0.0830831313090248,-0.0664776508816948,-0.0482386868303266,
-0.0443500357766238,-0.0424717165716612,-0.0409756787534045,-0.0391007051399124,
-0.037036502167314,-0.0335716462315504,-0.000375349248106819),
 .UNSPECIFIED.);
#792=B_SPLINE_CURVE_WITH_KNOTS('',3,(#71413,#71414,#71415,#71416,#71417,
#71418,#71419,#71420,#71421,#71422,#71423,#71424,#71425,#71426,#71427,#71428,
#71429,#71430,#71431,#71432,#71433,#71434,#71435,#71436,#71437,#71438,#71439,
#71440,#71441,#71442,#71443,#71444),.UNSPECIFIED.,.F.,.F.,(4,2,2,2,2,2,
2,2,2,2,2,2,2,2,2,4),(-1.604518044356,-1.59482654117459,-1.58877374327812,
-1.58575879969892,-1.58325763982483,-1.58060476826667,-1.57731770622977,
-1.57092568823115,-1.54959306788281,-1.52432379448028,-1.52103104075161,
-1.51918967991357,-1.51784327588204,-1.51600961624893,-1.51234881403237,
-1.49489110793716),.UNSPECIFIED.);
#793=B_SPLINE_CURVE_WITH_KNOTS('',3,(#71445,#71446,#71447,#71448,#71449,
#71450,#71451,#71452,#71453,#71454,#71455,#71456,#71457,#71458,#71459,#71460,
#71461,#71462,#71463,#71464,#71465,#71466,#71467,#71468,#71469,#71470,#71471,
#71472,#71473,#71474,#71475,#71476,#71477,#71478,#71479,#71480,#71481,#71482,
#71483,#71484,#71485,#71486,#71487,#71488,#71489,#71490,#71491,#71492,#71493,
#71494,#71495,#71496,#71497,#71498,#71499,#71500,#71501,#71502,#71503,#71504,
#71505,#71506,#71507,#71508,#71509,#71510,#71511,#71512,#71513,#71514,#71515,
#71516,#71517,#71518,#71519,#71520,#71521,#71522,#71523,#71524,#71525,#71526,
#71527,#71528,#71529,#71530,#71531,#71532,#71533,#71534,#71535,#71536,#71537,
#71538,#71539,#71540,#71541,#71542,#71543,#71544,#71545,#71546,#71547,#71548,
#71549,#71550,#71551,#71552,#71553,#71554,#71555,#71556,#71557,#71558,#71559,
#71560,#71561,#71562,#71563,#71564,#71565,#71566,#71567,#71568,#71569,#71570,
#71571,#71572,#71573,#71574,#71575,#71576,#71577,#71578,#71579,#71580,#71581,
#71582,#71583,#71584,#71585,#71586,#71587,#71588,#71589,#71590,#71591,#71592,
#71593,#71594,#71595,#71596,#71597,#71598,#71599,#71600,#71601,#71602,#71603,
#71604,#71605,#71606,#71607,#71608,#71609,#71610,#71611,#71612,#71613,#71614,
#71615,#71616,#71617,#71618,#71619,#71620,#71621,#71622,#71623,#71624,#71625,
#71626,#71627,#71628,#71629,#71630,#71631,#71632,#71633,#71634,#71635,#71636,
#71637,#71638,#71639,#71640,#71641,#71642,#71643,#71644,#71645,#71646,#71647,
#71648),.UNSPECIFIED.,.F.,.F.,(4,2,2,2,2,2,2,2,2,2,2,2,2,2,2,2,2,2,2,2,
2,2,2,2,2,2,2,2,2,2,2,2,2,2,2,2,2,2,2,2,2,2,2,2,2,2,2,2,2,2,2,2,2,2,2,2,
2,2,2,2,2,2,2,2,2,2,2,2,2,2,2,2,2,2,2,2,2,2,2,2,2,2,2,2,2,2,2,2,2,2,2,2,
2,2,2,2,2,2,2,2,2,4),(-0.912282028493777,-0.909732451909759,-0.907022044663811,
-0.903134350440392,-0.893467012592433,-0.866991641093441,-0.855997791384227,
-0.849525498317699,-0.847242989102264,-0.845697990491516,-0.844056883709189,
-0.841319784346746,-0.83110537098309,-0.802787555749626,-0.789604516959915,
-0.785298561161931,-0.78247868405242,-0.779753589220489,-0.775934866291146,
-0.766033762026051,-0.750203385085449,-0.724412086452443,-0.720961308019087,
-0.719147750631595,-0.717664220469517,-0.715726249183874,-0.711514104312759,
-0.705578484861349,-0.687121135556323,-0.665127566259059,-0.659851753887868,
-0.656527652725764,-0.65387149951668,-0.650831970491827,-0.645476031024791,
-0.638811386089502,-0.615989702041514,-0.597688900341373,-0.593800441729262,
-0.591922474985267,-0.590426868758181,-0.5885526732148,-0.584684005300306,
-0.579390640141005,-0.564473646400988,-0.537540844470895,-0.532384909793752,
-0.529095565737712,-0.52644189034469,-0.523377334284261,-0.517900164386236,
-0.514171282351249,-0.50301436850133,-0.48785747772316,-0.468909757636497,
-0.465885849437866,-0.464182828917149,-0.462664721096335,-0.460538330203103,
-0.455188804679728,-0.450679891147248,-0.431552868369006,-0.408518642444654,
-0.403724554954122,-0.40080258671598,-0.39812308615128,-0.394589497767307,
-0.386587864175764,-0.375102234407785,-0.360394480624298,-0.341551944608335,
-0.338531707374926,-0.33682944509048,-0.335311045494618,-0.333182920236384,
-0.32782213331912,-0.323299652381592,-0.304069588409059,-0.283019022764621,
-0.277768698271046,-0.274451856078361,-0.271796115757312,-0.268751194295786,
-0.263369764956323,-0.241183609572746,-0.216304108732404,-0.212379121615335,
-0.210460756325435,-0.208929591944377,-0.20729528686359,-0.204590090842878,
-0.1936227821569,-0.162492732686161,-0.152091753769073,-0.148108231108423,
-0.145627727844826,-0.143533168328323,-0.140825610111392,-0.137411158688223,
-0.131919259359916,-0.12053744697573,-0.110043953422301),.UNSPECIFIED.);
#794=B_SPLINE_CURVE_WITH_KNOTS('',3,(#71653,#71654,#71655,#71656,#71657,
#71658,#71659,#71660,#71661,#71662,#71663,#71664,#71665,#71666,#71667,#71668,
#71669,#71670,#71671,#71672,#71673,#71674,#71675,#71676,#71677,#71678,#71679,
#71680,#71681,#71682,#71683,#71684,#71685,#71686,#71687,#71688,#71689,#71690,
#71691,#71692,#71693,#71694,#71695,#71696,#71697,#71698,#71699,#71700,#71701,
#71702,#71703,#71704,#71705,#71706,#71707,#71708,#71709,#71710,#71711,#71712,
#71713,#71714,#71715,#71716,#71717,#71718,#71719,#71720,#71721,#71722,#71723,
#71724,#71725,#71726,#71727,#71728,#71729,#71730,#71731,#71732,#71733,#71734,
#71735,#71736,#71737,#71738,#71739,#71740,#71741,#71742,#71743,#71744,#71745,
#71746,#71747,#71748,#71749,#71750,#71751,#71752,#71753,#71754,#71755,#71756,
#71757,#71758,#71759,#71760,#71761,#71762,#71763,#71764,#71765,#71766,#71767,
#71768,#71769,#71770,#71771,#71772,#71773,#71774,#71775,#71776,#71777,#71778,
#71779,#71780,#71781,#71782,#71783,#71784,#71785,#71786,#71787,#71788,#71789,
#71790,#71791,#71792,#71793,#71794,#71795,#71796,#71797,#71798,#71799,#71800,
#71801,#71802,#71803,#71804,#71805,#71806,#71807,#71808,#71809,#71810,#71811,
#71812,#71813,#71814,#71815,#71816,#71817,#71818,#71819,#71820,#71821,#71822,
#71823,#71824,#71825,#71826,#71827,#71828,#71829,#71830,#71831,#71832,#71833,
#71834,#71835,#71836,#71837,#71838,#71839,#71840,#71841,#71842,#71843,#71844,
#71845,#71846,#71847,#71848),.UNSPECIFIED.,.F.,.F.,(4,2,2,2,2,2,2,2,2,2,
2,2,2,2,2,2,2,2,2,2,2,2,2,2,2,2,2,2,2,2,2,2,2,2,2,2,2,2,2,2,2,2,2,2,2,2,
2,2,2,2,2,2,2,2,2,2,2,2,2,2,2,2,2,2,2,2,2,2,2,2,2,2,2,2,2,2,2,2,2,2,2,2,
2,2,2,2,2,2,2,2,2,2,2,2,2,2,2,4),(-1.49528681114923,-1.46855272369361,-1.45428468371154,
-1.44912259759338,-1.44532634671494,-1.44346577193218,-1.44211788915904,
-1.44030054743845,-1.43683332844687,-1.41121315842747,-1.38848868021727,
-1.3831234700149,-1.38008157632856,-1.37742495327045,-1.37410235085635,
-1.3688331232657,-1.34789204676443,-1.3285707942032,-1.32403541681642,-1.31866412829265,
-1.31653414524756,-1.31501525121085,-1.3133132825484,-1.31029541555486,
-1.29154122720412,-1.27697453213141,-1.26537970380373,-1.25732375253172,
-1.25378083068097,-1.25109954987935,-1.2481807616687,-1.24340382021235,
-1.22205381702392,-1.20448858781943,-1.19648564712618,-1.19126272168435,
-1.18915538199024,-1.18763985238451,-1.18592688296747,-1.1829377339115,
-1.16400776002152,-1.14886623739257,-1.13771725512934,-1.13398995122727,
-1.12851381892228,-1.1254490228485,-1.12279463976138,-1.11950375375368,
-1.11434392984272,-1.08742109191882,-1.07246850212864,-1.06716714906454,
-1.06329440981626,-1.06141915504791,-1.05992316280081,-1.05804524014052,
-1.0541584817971,-1.03599725474525,-1.00638550074406,-1.00103327809424,
-0.997994085100304,-0.995337174967629,-0.992010721152651,-0.986728122815143,
-0.964753447519439,-0.946256017487257,-0.940312343212254,-0.936096313763103,
-0.934157349015302,-0.932673422108751,-0.930859760031999,-0.927409761503957,
-0.90163963893137,-0.885821903589034,-0.875924423632804,-0.872105609015954,
-0.869379886381196,-0.866558847922251,-0.862250080075497,-0.849049229967423,
-0.820972039672042,-0.810381009023976,-0.80770130321436,-0.806072349638351,
-0.804537392727648,-0.802605348585925,-0.79714509209623,-0.792501934915703,
-0.772327587767281,-0.75065317915987,-0.745842806773145,-0.742916871218985,
-0.740237537532097,-0.736709749514559,-0.728746881905702,-0.717341698123835,
-0.702550424108753,-0.693006869784502),.UNSPECIFIED.);
#795=B_SPLINE_CURVE_WITH_KNOTS('',3,(#71850,#71851,#71852,#71853,#71854,
#71855,#71856,#71857,#71858,#71859,#71860,#71861,#71862,#71863,#71864,#71865,
#71866,#71867,#71868,#71869,#71870,#71871,#71872,#71873,#71874,#71875,#71876,
#71877,#71878,#71879,#71880,#71881),.UNSPECIFIED.,.F.,.F.,(4,2,2,2,2,2,
2,2,2,2,2,2,2,2,2,4),(-0.110043953422301,-0.105723948072265,-0.0868134336401754,
-0.083790770499327,-0.0820879709152286,-0.0805697053593665,-0.0784426078136448,
-0.0735379468835575,-0.0438475112799801,-0.0261388361933189,-0.0214822246042773,
-0.0185891436469133,-0.0160354833484494,-0.013420339260892,-0.00999057246888134,
-0.000374718360681822),.UNSPECIFIED.);
#796=B_SPLINE_CURVE_WITH_KNOTS('',3,(#71882,#71883,#71884,#71885,#71886,
#71887,#71888,#71889,#71890,#71891,#71892,#71893,#71894,#71895,#71896,#71897,
#71898,#71899,#71900,#71901,#71902,#71903,#71904,#71905,#71906,#71907,#71908,
#71909,#71910,#71911,#71912,#71913,#71914,#71915,#71916,#71917,#71918,#71919,
#71920,#71921,#71922,#71923,#71924,#71925,#71926,#71927,#71928,#71929,#71930,
#71931,#71932,#71933,#71934,#71935,#71936,#71937,#71938,#71939,#71940,#71941,
#71942,#71943,#71944,#71945,#71946,#71947,#71948,#71949,#71950,#71951,#71952,
#71953,#71954,#71955,#71956,#71957,#71958,#71959,#71960,#71961,#71962,#71963,
#71964,#71965,#71966,#71967,#71968,#71969,#71970,#71971,#71972,#71973,#71974,
#71975,#71976,#71977,#71978,#71979,#71980,#71981,#71982,#71983,#71984,#71985,
#71986,#71987,#71988,#71989,#71990,#71991,#71992,#71993,#71994,#71995,#71996,
#71997,#71998,#71999,#72000,#72001,#72002,#72003,#72004,#72005,#72006,#72007,
#72008,#72009,#72010,#72011,#72012,#72013,#72014,#72015,#72016,#72017,#72018,
#72019,#72020,#72021,#72022,#72023,#72024,#72025,#72026,#72027,#72028,#72029,
#72030,#72031,#72032,#72033,#72034,#72035,#72036,#72037,#72038,#72039,#72040,
#72041,#72042,#72043,#72044,#72045,#72046,#72047,#72048,#72049,#72050,#72051,
#72052,#72053,#72054,#72055,#72056,#72057,#72058,#72059,#72060,#72061,#72062,
#72063),.UNSPECIFIED.,.F.,.F.,(4,2,2,2,2,2,2,2,2,2,2,2,2,2,2,2,2,2,2,2,
2,2,2,2,2,2,2,2,2,2,2,2,2,2,2,2,2,2,2,2,2,2,2,2,2,2,2,2,2,2,2,2,2,2,2,2,
2,2,2,2,2,2,2,2,2,2,2,2,2,2,2,2,2,2,2,2,2,2,2,2,2,2,2,2,2,2,2,2,2,2,4),
(-2.40676737505766,-2.36885811930424,-2.36539243889984,-2.36332834988335,
-2.36145385669369,-2.35995866505869,-2.35808203778825,-2.35419895511609,
-2.33623601044081,-2.32060916989795,-2.31000876570412,-2.3047626346255,
-2.30040444525601,-2.30027274855213,-2.30014099121797,-2.30000764581859,
-2.29987103087719,-2.29722856429417,-2.29451931915846,-2.2912480939647,
-2.28315200209121,-2.25511701496819,-2.24370005186781,-2.23706883417478,
-2.2347665378962,-2.23321793657518,-2.23158360508162,-2.2288768215928,-2.21906637476102,
-2.1986970470316,-2.1791581740144,-2.17379302171211,-2.17075200161204,-2.16809663777398,
-2.16477628523681,-2.15951208693814,-2.13721650032768,-2.11894980169944,
-2.11304512246817,-2.10884992630379,-2.10691524696749,-2.1054321951931,
-2.10361665105082,-2.10015555029197,-2.07449770850116,-2.05862615101731,
-2.04870888370183,-2.0448884177559,-2.04216330686692,-2.03967691703059,
-2.0363059735757,-2.02763478336961,-2.00020914183136,-1.98502087527762,
-1.98127062914168,-1.97941942847561,-1.97807255577222,-1.9762481484466,
-1.97274535820892,-1.94746155372281,-1.93138704444944,-1.92460025860737,
-1.91916884660418,-1.91611404308323,-1.91345995559178,-1.91015859168998,
-1.90496024985769,-1.8789836033319,-1.86339829114684,-1.8579735724623,-1.85403406252968,
-1.85214660975268,-1.85065117813065,-1.84878684399256,-1.84496872606216,
-1.81643888396224,-1.79713350677552,-1.79176468352873,-1.78872281261131,
-1.7860674015248,-1.78274790590747,-1.77748696564915,-1.75648150480151,
-1.73720627442121,-1.73267741279706,-1.72731205921512,-1.72518348954293,
-1.7236652941129,-1.72196379626685,-1.71894615478858,-1.71427609505927),
 .UNSPECIFIED.);
#797=B_SPLINE_CURVE_WITH_KNOTS('',3,(#72069,#72070,#72071,#72072,#72073,
#72074,#72075,#72076,#72077,#72078,#72079,#72080,#72081,#72082,#72083,#72084,
#72085,#72086,#72087,#72088,#72089,#72090,#72091,#72092,#72093,#72094,#72095,
#72096,#72097,#72098,#72099,#72100,#72101,#72102,#72103,#72104,#72105,#72106,
#72107,#72108,#72109,#72110,#72111,#72112,#72113,#72114,#72115,#72116,#72117,
#72118,#72119,#72120,#72121,#72122,#72123,#72124,#72125,#72126,#72127,#72128,
#72129,#72130,#72131,#72132,#72133,#72134,#72135,#72136,#72137,#72138,#72139,
#72140,#72141,#72142,#72143,#72144,#72145,#72146,#72147,#72148,#72149,#72150,
#72151,#72152,#72153,#72154,#72155,#72156,#72157,#72158,#72159,#72160,#72161,
#72162,#72163,#72164,#72165,#72166,#72167,#72168,#72169,#72170,#72171,#72172,
#72173,#72174,#72175,#72176,#72177,#72178,#72179,#72180,#72181,#72182,#72183,
#72184,#72185,#72186,#72187,#72188,#72189,#72190,#72191,#72192,#72193,#72194,
#72195,#72196,#72197,#72198,#72199,#72200,#72201,#72202,#72203,#72204,#72205,
#72206,#72207,#72208,#72209,#72210,#72211,#72212,#72213,#72214,#72215,#72216,
#72217,#72218,#72219,#72220,#72221,#72222,#72223,#72224,#72225,#72226,#72227,
#72228,#72229,#72230,#72231,#72232,#72233,#72234,#72235,#72236,#72237,#72238,
#72239,#72240,#72241,#72242,#72243,#72244,#72245,#72246),.UNSPECIFIED.,
 .F.,.F.,(4,2,2,2,2,2,2,2,2,2,2,2,2,2,2,2,2,2,2,2,2,2,2,2,2,2,2,2,2,2,2,
2,2,2,2,2,2,2,2,2,2,2,2,2,2,2,2,2,2,2,2,2,2,2,2,2,2,2,2,2,2,2,2,2,2,2,2,
2,2,2,2,2,2,2,2,2,2,2,2,2,2,2,2,2,2,2,2,2,4),(-0.693097973780701,-0.674549641960477,
-0.669769327196677,-0.666850111379091,-0.664169475107421,-0.660628949477002,
-0.652586032237884,-0.641015331240216,-0.626400811058394,-0.607614692510139,
-0.604596273449597,-0.602894319605062,-0.601375640929368,-0.599246312987551,
-0.593878156109545,-0.589346788109495,-0.570047575324775,-0.549117048286052,
-0.543854108710772,-0.540533489627345,-0.537877266572495,-0.534834538807356,
-0.529464413475491,-0.5258331620478,-0.51994071445516,-0.497561490725128,
-0.480235875503355,-0.477238771902252,-0.475541319703888,-0.474021049270523,
-0.471881777337472,-0.466447844962255,-0.461836612463552,-0.4419151443869,
-0.41986999739315,-0.415089819908908,-0.412170485508472,-0.409489609605992,
-0.4059485738069,-0.397903591193224,-0.386329015522499,-0.371716560840827,
-0.352930761147811,-0.349912167527107,-0.348210094899348,-0.346691295159436,
-0.344561776821192,-0.339193032123336,-0.334661104104818,-0.315358786849685,
-0.294429194368609,-0.289165590683144,-0.285844640913248,-0.283188207344413,
-0.280145297173966,-0.274775009919012,-0.268087397708659,-0.252417314302911,
-0.227201442056148,-0.223578551418683,-0.221732704114275,-0.220219043687819,
-0.218548932402678,-0.215679356975658,-0.201704586611215,-0.172437607876477,
-0.163140267015902,-0.159310171578589,-0.156609605734997,-0.154153034911004,
-0.150304655941825,-0.145856576375551,-0.137621381185388,-0.114452245743204,
-0.0981607023113854,-0.0951691819174354,-0.093472860190305,-0.0919520782547177,
-0.0904229041201003,-0.086798293467879,-0.0737300039025831,-0.0479322634489471,
-0.0364539992731121,-0.0323301275026648,-0.029824580290477,-0.02711313506907,
-0.0244320123183317,-0.0208122799601177,-0.000374898576945566),
 .UNSPECIFIED.);
#798=B_SPLINE_CURVE_WITH_KNOTS('',3,(#72247,#72248,#72249,#72250,#72251,
#72252,#72253,#72254,#72255,#72256,#72257,#72258,#72259,#72260,#72261,#72262,
#72263,#72264,#72265,#72266,#72267,#72268,#72269,#72270,#72271,#72272,#72273,
#72274,#72275,#72276,#72277,#72278,#72279,#72280,#72281,#72282,#72283,#72284,
#72285,#72286,#72287,#72288,#72289,#72290,#72291,#72292,#72293,#72294,#72295,
#72296,#72297,#72298,#72299,#72300,#72301,#72302,#72303,#72304),
 .UNSPECIFIED.,.F.,.F.,(4,2,2,2,2,2,2,2,2,2,2,2,2,2,2,2,2,2,2,2,2,2,2,2,
2,2,2,2,4),(-1.60473182869979,-1.57950221225551,-1.57499179546473,-1.57286135670865,
-1.57132330223305,-1.56979822383723,-1.5681137886786,-1.56517774394569,
-1.55095382492133,-1.52912947981169,-1.51420712342516,-1.50981965579016,
-1.50970266867535,-1.50958436993072,-1.50946351888462,-1.50933871895019,
-1.50920833971582,-1.50907040950528,-1.50892246071234,-1.50876129769517,
-1.50858263340586,-1.50838049388529,-1.50814618906318,-1.50791857137058,
-1.5075808029852,-1.50492808808717,-1.5016648820731,-1.49659976078895,-1.49528681114923),
 .UNSPECIFIED.);
#799=B_SPLINE_CURVE_WITH_KNOTS('',3,(#72305,#72306,#72307,#72308,#72309,
#72310,#72311,#72312,#72313,#72314,#72315,#72316,#72317,#72318,#72319,#72320,
#72321,#72322,#72323,#72324,#72325,#72326,#72327,#72328,#72329,#72330,#72331,
#72332,#72333,#72334,#72335,#72336,#72337,#72338,#72339,#72340,#72341,#72342,
#72343,#72344,#72345,#72346,#72347,#72348,#72349,#72350,#72351,#72352,#72353,
#72354,#72355,#72356,#72357,#72358,#72359,#72360,#72361,#72362,#72363,#72364,
#72365,#72366,#72367,#72368,#72369,#72370,#72371,#72372,#72373,#72374,#72375,
#72376,#72377,#72378,#72379,#72380,#72381,#72382,#72383,#72384,#72385,#72386,
#72387,#72388,#72389,#72390,#72391,#72392,#72393,#72394,#72395,#72396,#72397,
#72398,#72399,#72400,#72401,#72402,#72403,#72404,#72405,#72406,#72407,#72408,
#72409,#72410,#72411,#72412,#72413,#72414,#72415,#72416,#72417,#72418,#72419,
#72420,#72421,#72422,#72423,#72424,#72425,#72426,#72427,#72428,#72429,#72430,
#72431,#72432,#72433,#72434,#72435,#72436,#72437,#72438,#72439,#72440,#72441,
#72442,#72443,#72444,#72445,#72446,#72447,#72448,#72449,#72450,#72451,#72452,
#72453,#72454,#72455,#72456,#72457,#72458,#72459,#72460,#72461,#72462,#72463,
#72464,#72465,#72466,#72467,#72468,#72469,#72470,#72471,#72472,#72473,#72474,
#72475,#72476,#72477,#72478,#72479,#72480,#72481,#72482,#72483,#72484,#72485,
#72486,#72487,#72488,#72489,#72490,#72491,#72492,#72493,#72494,#72495,#72496,
#72497,#72498,#72499,#72500),.UNSPECIFIED.,.F.,.F.,(4,2,2,2,2,2,2,2,2,2,
2,2,2,2,2,2,2,2,2,2,2,2,2,2,2,2,2,2,2,2,2,2,2,2,2,2,2,2,2,2,2,2,2,2,2,2,
2,2,2,2,2,2,2,2,2,2,2,2,2,2,2,2,2,2,2,2,2,2,2,2,2,2,2,2,2,2,2,2,2,2,2,2,
2,2,2,2,2,2,2,2,2,2,2,2,2,2,2,4),(-1.71427609505927,-1.70017303108593,-1.68556904885637,
-1.67401337215023,-1.66597714801641,-1.66243832947086,-1.65975850435754,
-1.65683971639778,-1.65205913441651,-1.62999996772187,-1.61006058655689,
-1.60544646022636,-1.60001096042517,-1.59787184069993,-1.59635200523981,
-1.59465539127848,-1.59166066478746,-1.57454439136803,-1.55204064591276,
-1.54392032541994,-1.53769856415861,-1.53448515206266,-1.53209369373478,
-1.52906712745507,-1.52390994022624,-1.49237913026035,-1.48007144990521,
-1.47311729244318,-1.47077555213529,-1.46921909128428,-1.46779583423245,
-1.46534176224731,-1.45806426073014,-1.43582571772125,-1.41394917988829,
-1.40921063025882,-1.40630065135319,-1.40361792659188,-1.40011999009848,
-1.39210156497417,-1.36382223443214,-1.34834535786019,-1.34456347882511,
-1.34270605794405,-1.34121041764444,-1.3393154315555,-1.33533623270764,
-1.31011207241857,-1.29444636538617,-1.28776063683116,-1.28239112492061,
-1.27934893572701,-1.2766932874654,-1.27337354889257,-1.26811233456746,
-1.24710313926716,-1.22782728057926,-1.22329815384168,-1.21793243338644,
-1.21580368829209,-1.21428535744858,-1.21258369603666,-1.20956573923473,
-1.190789692139,-1.17618220113236,-1.164627513391,-1.15659154746579,-1.15305256930436,
-1.15037252280154,-1.14745339606362,-1.142672031759,-1.12065324374132,-1.10382899749774,
-1.09579036606485,-1.09055149765998,-1.08844209345814,-1.0869266444777,
-1.08521561540114,-1.08223368898902,-1.06349601681706,-1.04895993334718,
-1.03733921609711,-1.02927127916442,-1.02572705924817,-1.02304628270159,
-1.02012950208988,-1.01535928236584,-0.994104480282265,-0.976427234666432,
-0.968430370325362,-0.963210584308027,-0.96110412203481,-0.959589099409234,
-0.95787660282681,-0.954888127845239,-0.935959519200394,-0.920819904523672,
-0.912183428409147),.UNSPECIFIED.);
#800=B_SPLINE_CURVE_WITH_KNOTS('',3,(#72505,#72506,#72507,#72508,#72509,
#72510,#72511,#72512,#72513,#72514,#72515,#72516,#72517,#72518,#72519,#72520,
#72521,#72522,#72523,#72524,#72525,#72526,#72527,#72528,#72529,#72530,#72531,
#72532,#72533,#72534,#72535,#72536,#72537,#72538,#72539,#72540,#72541,#72542,
#72543,#72544,#72545,#72546,#72547,#72548,#72549,#72550,#72551,#72552,#72553,
#72554,#72555,#72556,#72557,#72558,#72559,#72560,#72561,#72562,#72563,#72564,
#72565,#72566,#72567,#72568,#72569,#72570,#72571,#72572,#72573,#72574,#72575,
#72576,#72577,#72578,#72579,#72580,#72581,#72582,#72583,#72584,#72585,#72586,
#72587,#72588,#72589,#72590,#72591,#72592,#72593,#72594,#72595,#72596,#72597,
#72598,#72599,#72600,#72601,#72602,#72603,#72604,#72605,#72606,#72607,#72608,
#72609,#72610,#72611,#72612,#72613,#72614,#72615,#72616,#72617,#72618,#72619,
#72620,#72621,#72622,#72623,#72624,#72625,#72626,#72627,#72628,#72629,#72630,
#72631,#72632,#72633,#72634,#72635,#72636,#72637,#72638,#72639,#72640,#72641,
#72642,#72643,#72644,#72645,#72646,#72647,#72648,#72649,#72650,#72651,#72652,
#72653,#72654,#72655,#72656,#72657,#72658,#72659,#72660,#72661,#72662,#72663,
#72664,#72665,#72666,#72667,#72668,#72669,#72670,#72671,#72672,#72673,#72674,
#72675,#72676,#72677,#72678,#72679,#72680,#72681,#72682,#72683,#72684,#72685,
#72686,#72687,#72688,#72689,#72690,#72691,#72692,#72693,#72694,#72695,#72696,
#72697,#72698,#72699,#72700,#72701,#72702,#72703,#72704),.UNSPECIFIED.,
 .F.,.F.,(4,2,2,2,2,2,2,2,2,2,2,2,2,2,2,2,2,2,2,2,2,2,2,2,2,2,2,2,2,2,2,
2,2,2,2,2,2,2,2,2,2,2,2,2,2,2,2,2,2,2,2,2,2,2,2,2,2,2,2,2,2,2,2,2,2,2,2,
2,2,2,2,2,2,2,2,2,2,2,2,2,2,2,2,2,2,2,2,2,2,2,2,2,2,2,2,2,2,2,2,4),(-1.4951650948055,
-1.49447528564397,-1.49306392442721,-1.49114658335287,-1.48704743911027,
-1.46198518424821,-1.44633910347216,-1.43965837595818,-1.43429191177407,
-1.43125022808202,-1.42859430966004,-1.42527327522059,-1.42000795915998,
-1.39904446496783,-1.37974559744137,-1.37521362934586,-1.36984555104675,
-1.36771637310754,-1.36619789203425,-1.36449620136358,-1.36147843240729,
-1.34270960496494,-1.32811110531228,-1.31655189904539,-1.30851379808812,
-1.30497434467855,-1.30229407833229,-1.29937483058712,-1.29459349643746,
-1.27258931935542,-1.2526103525059,-1.24799122551831,-1.24255147102499,
-1.24041151808989,-1.23889136123176,-1.23719465521174,-1.23420027177389,
-1.21722321120531,-1.19461703595385,-1.18647907616479,-1.1802470460008,
-1.17703133033609,-1.17463932956751,-1.17161360477339,-1.16646160399906,
-1.13489545098283,-1.1226079945036,-1.11566084740704,-1.11331972259105,
-1.11176321112413,-1.11033949068955,-1.1078837926122,-1.10059450541295,
-1.07836686979375,-1.05767422533776,-1.05230033791561,-1.04925704616846,
-1.04660119293673,-1.04328217373071,-1.03802406050656,-1.01513600159545,
-0.993369745695994,-0.98788151275423,-0.985734286299891,-0.98421293067608,
-0.982519408292301,-0.979540132601306,-0.963905513812062,-0.940931343280396,
-0.928008123093209,-0.923833616043403,-0.921040227947654,-0.918327367378527,
-0.914427176960801,-0.90462177412823,-0.87826978273584,-0.863451787979356,
-0.859742236505118,-0.857898694544346,-0.856551834473005,-0.854719226595905,
-0.851065418715158,-0.82705142425113,-0.802685988624029,-0.797538249940807,
-0.794513351679398,-0.792121100846208,-0.788903851833482,-0.782664700127272,
-0.774513009440679,-0.751837935199026,-0.734906975750591,-0.731911709645646,
-0.730214732144666,-0.728694462938626,-0.726554609811127,-0.721116098971184,
-0.716499119787935,-0.696530704436245,-0.693097973780701),.UNSPECIFIED.);
#801=B_SPLINE_CURVE_WITH_KNOTS('',3,(#72705,#72706,#72707,#72708,#72709,
#72710,#72711,#72712,#72713,#72714,#72715,#72716,#72717,#72718,#72719,#72720,
#72721,#72722,#72723,#72724,#72725,#72726,#72727,#72728,#72729,#72730,#72731,
#72732,#72733,#72734,#72735,#72736,#72737,#72738,#72739,#72740,#72741,#72742,
#72743,#72744,#72745,#72746,#72747,#72748,#72749,#72750,#72751,#72752,#72753,
#72754,#72755,#72756,#72757,#72758,#72759,#72760,#72761,#72762,#72763,#72764,
#72765,#72766,#72767,#72768,#72769,#72770,#72771,#72772,#72773,#72774,#72775,
#72776,#72777,#72778,#72779,#72780,#72781,#72782,#72783,#72784,#72785,#72786,
#72787,#72788,#72789,#72790,#72791,#72792,#72793,#72794,#72795,#72796,#72797,
#72798,#72799,#72800,#72801,#72802,#72803,#72804,#72805,#72806,#72807,#72808,
#72809,#72810,#72811,#72812,#72813,#72814,#72815,#72816,#72817,#72818,#72819,
#72820,#72821,#72822,#72823,#72824,#72825,#72826,#72827,#72828,#72829,#72830,
#72831,#72832,#72833,#72834,#72835,#72836,#72837,#72838,#72839,#72840,#72841,
#72842,#72843,#72844,#72845,#72846,#72847,#72848,#72849,#72850,#72851,#72852,
#72853,#72854,#72855,#72856,#72857,#72858,#72859,#72860,#72861,#72862,#72863,
#72864,#72865,#72866,#72867,#72868,#72869,#72870,#72871,#72872,#72873,#72874,
#72875,#72876,#72877,#72878,#72879,#72880,#72881,#72882,#72883,#72884,#72885,
#72886,#72887,#72888,#72889,#72890,#72891,#72892,#72893,#72894,#72895,#72896,
#72897,#72898,#72899,#72900,#72901,#72902,#72903,#72904,#72905,#72906,#72907,
#72908,#72909,#72910),.UNSPECIFIED.,.F.,.F.,(4,2,2,2,2,2,2,2,2,2,2,2,2,
2,2,2,2,2,2,2,2,2,2,2,2,2,2,2,2,2,2,2,2,2,2,2,2,2,2,2,2,2,2,2,2,2,2,2,2,
2,2,2,2,2,2,2,2,2,2,2,2,2,2,2,2,2,2,2,2,2,2,2,2,2,2,2,2,2,2,2,2,2,2,2,2,
2,2,2,2,2,2,2,2,2,2,2,2,2,2,2,2,2,4),(-0.912183428409147,-0.909671435824856,
-0.905944473968316,-0.900469105869615,-0.897405062984082,-0.894751533133857,
-0.891461985557897,-0.886304887334374,-0.859350711777633,-0.844420931988362,
-0.839124610941128,-0.835254869517453,-0.833380534110074,-0.831885015905191,
-0.830007410952487,-0.826120492190165,-0.807839026955135,-0.785036967355285,
-0.778375912782796,-0.77302154311998,-0.769982418601881,-0.767326319316143,
-0.764001893366411,-0.758724683002095,-0.736684389957623,-0.71823188451559,
-0.712296011234923,-0.708084289277837,-0.706146412716717,-0.704662927355313,
-0.702849364172057,-0.699398483790527,-0.673641249020921,-0.657817582749607,
-0.651092349110172,-0.645698508893679,-0.642651213017173,-0.639995994759288,
-0.636683208998828,-0.631446267963429,-0.606945776447085,-0.590310389252202,
-0.584688771737222,-0.580643193787097,-0.578735751186671,-0.577239722480526,
-0.575393501099614,-0.571669662655668,-0.54863484980516,-0.523540002267338,
-0.51825073883406,-0.515225132315514,-0.512567408565113,-0.509223062416149,
-0.503876677550803,-0.496252349283697,-0.476421512166381,-0.457052206429446,
-0.453186629666559,-0.451313076497196,-0.449817540386607,-0.447939106896463,
-0.444047895177174,-0.438713157543517,-0.423587361373984,-0.396972971280271,
-0.391801323230041,-0.388507488665556,-0.385853631066752,-0.38279266684416,
-0.377332523307534,-0.370497839597455,-0.35422988640262,-0.329243467800514,
-0.325705504763716,-0.323873526356167,-0.322526754420353,-0.320682921081915,
-0.316971451281173,-0.302135988458375,-0.275726905019111,-0.266013434072886,
-0.262122173922496,-0.259411064736845,-0.256615759259425,-0.252431177050569,
-0.2394087109049,-0.216071193352779,-0.200847480271835,-0.197878256551177,
-0.196186931659452,-0.194664868018181,-0.192513070827879,-0.186993485177083,
-0.182276967053412,-0.16150058880361,-0.140594532836167,-0.135874386843129,
-0.132925957423104,-0.130419423273389,-0.127841855145072,-0.124529608056003,
-0.109984215976658),.UNSPECIFIED.);
#802=B_SPLINE_CURVE_WITH_KNOTS('',3,(#72916,#72917,#72918,#72919,#72920,
#72921,#72922,#72923,#72924,#72925,#72926,#72927,#72928,#72929,#72930,#72931,
#72932,#72933,#72934,#72935,#72936,#72937,#72938,#72939,#72940,#72941,#72942,
#72943,#72944,#72945,#72946,#72947,#72948,#72949,#72950,#72951,#72952,#72953,
#72954,#72955,#72956,#72957,#72958,#72959,#72960,#72961,#72962,#72963,#72964,
#72965,#72966,#72967,#72968,#72969,#72970,#72971,#72972,#72973,#72974,#72975,
#72976,#72977,#72978,#72979,#72980,#72981,#72982,#72983,#72984,#72985,#72986,
#72987,#72988,#72989,#72990,#72991,#72992,#72993,#72994,#72995,#72996,#72997,
#72998,#72999,#73000,#73001,#73002,#73003,#73004,#73005,#73006,#73007,#73008,
#73009,#73010,#73011,#73012,#73013,#73014,#73015,#73016,#73017,#73018,#73019,
#73020,#73021,#73022,#73023,#73024,#73025,#73026,#73027,#73028,#73029,#73030,
#73031,#73032,#73033,#73034,#73035,#73036,#73037,#73038,#73039,#73040,#73041,
#73042,#73043,#73044,#73045,#73046,#73047,#73048,#73049,#73050,#73051,#73052,
#73053,#73054,#73055,#73056,#73057,#73058,#73059,#73060,#73061,#73062,#73063,
#73064,#73065,#73066,#73067,#73068,#73069,#73070,#73071,#73072,#73073,#73074,
#73075,#73076,#73077,#73078,#73079,#73080,#73081,#73082,#73083,#73084,#73085,
#73086,#73087,#73088,#73089,#73090,#73091,#73092,#73093),.UNSPECIFIED.,
 .F.,.F.,(4,2,2,2,2,2,2,2,2,2,2,2,2,2,2,2,2,2,2,2,2,2,2,2,2,2,2,2,2,2,2,
2,2,2,2,2,2,2,2,2,2,2,2,2,2,2,2,2,2,2,2,2,2,2,2,2,2,2,2,2,2,2,2,2,2,2,2,
2,2,2,2,2,2,2,2,2,2,2,2,2,2,2,2,2,2,2,2,2,4),(-0.692866832200926,-0.692429841896259,
-0.677564642022375,-0.65860681414682,-0.65561734955069,-0.653904485899281,
-0.652389220739771,-0.650282554339005,-0.645062507749672,-0.637066663952617,
-0.619534767965853,-0.598195365700189,-0.593418847644417,-0.590500442820064,
-0.587819576856678,-0.584277303563173,-0.576223648773558,-0.564630744430341,
-0.550040282648017,-0.531267419531168,-0.528249450010645,-0.526547598542327,
-0.525028900155804,-0.522899391304837,-0.517529975729226,-0.512997069945273,
-0.493685947566791,-0.472774422140611,-0.46750966263123,-0.464188529998434,
-0.461532284157875,-0.458489952235369,-0.45312167465568,-0.431151421593968,
-0.406740703957918,-0.402028112199817,-0.400143080609763,-0.398620233435407,
-0.39697042339584,-0.394194188743825,-0.382084872669531,-0.365235832692922,
-0.343572521515228,-0.338763872908473,-0.335838590220417,-0.333159600641532,
-0.329631892310251,-0.321667481345501,-0.310258397245341,-0.295475021956934,
-0.276586065095174,-0.273564000444231,-0.271861210906231,-0.270342688413377,
-0.268214814823387,-0.262856762593005,-0.25833772914005,-0.239133741195724,
-0.218059994578015,-0.212806940996901,-0.20948908364662,-0.206832941453479,
-0.203787988550606,-0.198407612120565,-0.176555692585955,-0.152330650292729,
-0.147418826773976,-0.145501521755874,-0.14397049987697,-0.142368283753846,
-0.139771155769888,-0.136568396477909,-0.129885128383817,-0.106156268801215,
-0.0885737715830057,-0.0839176749963868,-0.0810243844670173,-0.0783345105395892,
-0.0747317980163937,-0.0664631824218435,-0.0433552328482521,-0.0266755417178896,
-0.0204804644227642,-0.0181713332211261,-0.0166363156174901,-0.0152426914363794,
-0.0136145686663947,-0.0112495068105053,-0.000374704675043261),
 .UNSPECIFIED.);
#803=B_SPLINE_CURVE_WITH_KNOTS('',3,(#73094,#73095,#73096,#73097,#73098,
#73099,#73100,#73101,#73102,#73103,#73104,#73105,#73106,#73107,#73108,#73109,
#73110,#73111,#73112,#73113,#73114,#73115,#73116,#73117,#73118,#73119,#73120,
#73121),.UNSPECIFIED.,.F.,.F.,(4,2,2,2,2,2,2,2,2,2,2,2,2,4),(-1.60482636128448,
-1.57369633890873,-1.56700004022034,-1.56311826205165,-1.55959258294555,
-1.55691425521273,-1.5539888304229,-1.54917796400828,-1.52747173937229,
-1.51170533182018,-1.5028548534436,-1.49900355783005,-1.49609325357449,
-1.4951650948055),.UNSPECIFIED.);
#804=B_SPLINE_CURVE_WITH_KNOTS('',3,(#73123,#73124,#73125,#73126,#73127,
#73128,#73129,#73130,#73131,#73132,#73133,#73134,#73135,#73136,#73137,#73138,
#73139,#73140,#73141,#73142,#73143,#73144,#73145,#73146,#73147,#73148,#73149,
#73150,#73151,#73152,#73153,#73154,#73155,#73156),.UNSPECIFIED.,.F.,.F.,
(4,2,2,2,2,2,2,2,2,2,2,2,2,2,2,2,4),(-0.109984215976658,-0.108466704677333,
-0.0929800570091766,-0.0750124521263942,-0.0711272018396201,-0.0692498278984506,
-0.0677541996645172,-0.0658793571402882,-0.0620073879157499,-0.0511499299104798,
-0.0284204838189786,-0.0198058823455182,-0.0109766423492752,-0.0072974848453584,
-0.0046289889386618,-0.00236675908727173,-0.000393535835646313),
 .UNSPECIFIED.);
#805=B_SPLINE_CURVE_WITH_KNOTS('',3,(#73157,#73158,#73159,#73160,#73161,
#73162,#73163,#73164,#73165),.UNSPECIFIED.,.F.,.F.,(4,1,1,1,1,1,4),(109.955745458758,
110.419877743936,111.417384325898,112.41489090786,113.412397489822,114.409904071784,
115.380591207589),.UNSPECIFIED.);
#806=B_SPLINE_CURVE_WITH_KNOTS('',3,(#73170,#73171,#73172,#73173,#73174,
#73175,#73176,#73177,#73178,#73179,#73180,#73181,#73182,#73183,#73184,#73185,
#73186,#73187,#73188,#73189,#73190,#73191,#73192,#73193,#73194,#73195,#73196,
#73197,#73198,#73199,#73200,#73201,#73202,#73203,#73204,#73205,#73206,#73207,
#73208,#73209,#73210,#73211,#73212,#73213,#73214,#73215,#73216,#73217,#73218,
#73219,#73220,#73221,#73222,#73223,#73224,#73225,#73226,#73227,#73228,#73229,
#73230,#73231,#73232,#73233,#73234,#73235,#73236,#73237,#73238,#73239,#73240,
#73241,#73242,#73243,#73244,#73245,#73246,#73247,#73248,#73249,#73250,#73251,
#73252,#73253,#73254,#73255,#73256,#73257,#73258,#73259,#73260,#73261,#73262,
#73263,#73264,#73265,#73266,#73267,#73268,#73269,#73270,#73271,#73272,#73273,
#73274,#73275,#73276,#73277,#73278,#73279,#73280,#73281,#73282,#73283,#73284,
#73285,#73286,#73287,#73288,#73289,#73290,#73291,#73292,#73293,#73294,#73295,
#73296,#73297,#73298,#73299,#73300,#73301,#73302,#73303,#73304,#73305,#73306,
#73307,#73308,#73309,#73310,#73311,#73312,#73313,#73314,#73315,#73316,#73317,
#73318,#73319,#73320,#73321,#73322,#73323,#73324,#73325,#73326,#73327,#73328,
#73329,#73330,#73331,#73332,#73333,#73334,#73335,#73336,#73337,#73338,#73339,
#73340,#73341,#73342,#73343,#73344,#73345,#73346,#73347,#73348,#73349,#73350,
#73351,#73352,#73353,#73354,#73355,#73356,#73357,#73358,#73359,#73360,#73361,
#73362,#73363,#73364,#73365,#73366,#73367,#73368,#73369,#73370,#73371,#73372,
#73373,#73374,#73375,#73376,#73377,#73378,#73379),.UNSPECIFIED.,.F.,.F.,
(4,2,2,2,2,2,2,2,2,2,2,2,2,2,2,2,2,2,2,2,2,2,2,2,2,2,2,2,2,2,2,2,2,2,2,
2,2,2,2,2,2,2,2,2,2,2,2,2,2,2,2,2,2,2,2,2,2,2,2,2,2,2,2,2,2,2,2,2,2,2,2,
2,2,2,2,2,2,2,2,2,2,2,2,2,2,2,2,2,2,2,2,2,2,2,2,2,2,2,2,2,2,2,2,2,4),(-1.49484735329919,
-1.49484548901206,-1.48674394087996,-1.4839536958272,-1.48351580354143,
-1.48306057098407,-1.48293853263072,-1.4803502913914,-1.47746324147295,
-1.47275409837007,-1.45158379469974,-1.43390306301323,-1.42590944699101,
-1.4206916357885,-1.4185858469295,-1.41707121592934,-1.41535893770416,-1.41237061585787,
-1.39343189219521,-1.37828272968426,-1.36715911855713,-1.36343853441178,
-1.35797040008061,-1.35490814343165,-1.35225488253909,-1.34896398869188,
-1.34380129057227,-1.31699938277325,-1.30198523054024,-1.29667275036799,
-1.29279439127633,-1.29091857199719,-1.28942327352004,-1.28754764365696,
-1.28367002008495,-1.26601815451493,-1.25073985275118,-1.23976218660559,
-1.2360777320863,-1.23064916854066,-1.22759503359207,-1.22494098479056,
-1.22163894194219,-1.21643798574239,-1.19057483620645,-1.17491973908619,
-1.1694819540276,-1.1655354693624,-1.16364676100844,-1.16215137738946,-1.16028835999769,
-1.15647676786762,-1.13494336649669,-1.10767686376367,-1.10283125577838,
-1.09989869333012,-1.09722271970327,-1.09377241829604,-1.08634130077601,
-1.05475867166893,-1.04499675958336,-1.03901212495264,-1.03679422347914,
-1.0352611145489,-1.03359713622626,-1.03075458245268,-1.0188465865962,-0.992079180076298,
-0.979005382801924,-0.974816139563256,-0.972019986638176,-0.969309702161997,
-0.966035601471855,-0.958012128188596,-0.929930811708622,-0.914521581428813,
-0.910747012175014,-0.908890930492542,-0.907395147213971,-0.905498384784684,
-0.901510071644215,-0.876299941408438,-0.86064015035326,-0.850805503732773,
-0.846995895977954,-0.844272312627503,-0.841783114440567,-0.838401865113623,
-0.829634538140932,-0.802297646701117,-0.785878197715148,-0.782885869073012,
-0.781189565407821,-0.779669157251544,-0.777528087703224,-0.772081042854728,
-0.76745354877006,-0.747400586835847,-0.725614204714521,-0.72078946134825,
-0.717860973303176,-0.715183259198693,-0.711663411498443,-0.703745144296636,
-0.692866832200926),.UNSPECIFIED.);
#807=B_SPLINE_CURVE_WITH_KNOTS('',3,(#73381,#73382,#73383,#73384,#73385),
 .UNSPECIFIED.,.F.,.F.,(4,1,4),(115.380591207589,115.407410653746,116.238922074783),
 .UNSPECIFIED.);
#808=B_SPLINE_CURVE_WITH_KNOTS('',3,(#73386,#73387,#73388,#73389,#73390,
#73391,#73392,#73393,#73394,#73395,#73396,#73397,#73398,#73399,#73400,#73401,
#73402,#73403,#73404,#73405,#73406,#73407,#73408,#73409,#73410,#73411,#73412,
#73413,#73414,#73415,#73416,#73417,#73418,#73419,#73420,#73421,#73422,#73423,
#73424,#73425,#73426,#73427,#73428,#73429,#73430,#73431,#73432,#73433,#73434,
#73435,#73436,#73437,#73438,#73439,#73440,#73441,#73442,#73443,#73444,#73445,
#73446,#73447,#73448,#73449,#73450,#73451,#73452,#73453,#73454,#73455,#73456,
#73457,#73458,#73459,#73460,#73461,#73462,#73463,#73464,#73465,#73466,#73467,
#73468,#73469,#73470,#73471,#73472,#73473,#73474,#73475,#73476,#73477,#73478,
#73479,#73480,#73481,#73482,#73483,#73484,#73485,#73486,#73487,#73488,#73489,
#73490,#73491,#73492,#73493,#73494,#73495,#73496,#73497,#73498,#73499,#73500,
#73501,#73502,#73503,#73504,#73505,#73506,#73507,#73508,#73509,#73510,#73511,
#73512,#73513,#73514,#73515,#73516,#73517,#73518,#73519,#73520,#73521,#73522,
#73523,#73524,#73525,#73526,#73527,#73528,#73529,#73530,#73531,#73532,#73533),
 .UNSPECIFIED.,.F.,.F.,(4,3,3,3,3,3,3,3,3,3,3,3,3,3,3,3,3,3,3,3,3,3,3,3,
3,3,3,3,3,3,3,3,3,3,3,3,3,3,3,3,3,3,3,3,3,3,3,3,3,4),(116.238928182822,
116.404917235708,116.522420828224,116.639708216653,116.756876517021,116.873975708443,
116.991055657352,117.108249996379,117.225507405703,117.342983778858,117.40242381767,
117.519927421395,117.637214821166,117.754383132948,117.871482335835,117.988562296238,
118.105756646709,118.223014067466,118.340490451903,118.399930399632,118.51743395948,
118.634721315403,118.751889583392,118.868988742619,118.986068659578,119.10326296727,
119.220520345564,119.337996688525,119.397436981594,119.514940591803,119.632227997493,
119.74939631484,119.866495522933,119.983575488175,120.100769842902,120.218027267589,
120.335503655412,120.394943563556,120.512447240091,120.629734713282,120.7469030988,
120.864002375596,120.981082409943,121.098276833821,121.215534327787,121.333010784262,
121.392450145518,121.509946639959,121.627240956719,121.664501811606),
 .UNSPECIFIED.);
#809=B_SPLINE_CURVE_WITH_KNOTS('',3,(#73539,#73540,#73541,#73542,#73543,
#73544,#73545,#73546,#73547,#73548,#73549,#73550,#73551,#73552,#73553,#73554,
#73555,#73556,#73557,#73558,#73559,#73560,#73561,#73562,#73563,#73564,#73565,
#73566,#73567,#73568,#73569,#73570,#73571,#73572,#73573,#73574,#73575,#73576,
#73577,#73578,#73579,#73580,#73581,#73582,#73583,#73584,#73585,#73586,#73587,
#73588,#73589,#73590,#73591,#73592,#73593,#73594,#73595,#73596,#73597,#73598,
#73599,#73600,#73601,#73602,#73603,#73604,#73605,#73606,#73607,#73608,#73609,
#73610,#73611,#73612,#73613,#73614,#73615,#73616,#73617,#73618,#73619,#73620,
#73621,#73622,#73623,#73624,#73625,#73626,#73627,#73628,#73629,#73630,#73631,
#73632,#73633,#73634,#73635,#73636,#73637,#73638,#73639,#73640,#73641,#73642,
#73643,#73644,#73645,#73646,#73647,#73648,#73649,#73650,#73651,#73652,#73653,
#73654,#73655,#73656,#73657,#73658,#73659,#73660,#73661,#73662,#73663,#73664,
#73665,#73666,#73667,#73668,#73669,#73670,#73671,#73672,#73673,#73674,#73675,
#73676,#73677,#73678,#73679,#73680,#73681,#73682,#73683,#73684,#73685,#73686,
#73687,#73688,#73689,#73690,#73691,#73692,#73693,#73694,#73695,#73696,#73697,
#73698,#73699,#73700,#73701,#73702,#73703,#73704,#73705,#73706,#73707,#73708,
#73709,#73710,#73711,#73712,#73713,#73714,#73715,#73716),.UNSPECIFIED.,
 .F.,.F.,(4,2,2,2,2,2,2,2,2,2,2,2,2,2,2,2,2,2,2,2,2,2,2,2,2,2,2,2,2,2,2,
2,2,2,2,2,2,2,2,2,2,2,2,2,2,2,2,2,2,2,2,2,2,2,2,2,2,2,2,2,2,2,2,2,2,2,2,
2,2,2,2,2,2,2,2,2,2,2,2,2,2,2,2,2,2,2,2,2,4),(-0.693046076597336,-0.67984367033363,
-0.657314152795425,-0.650710899261982,-0.645398194889328,-0.64237851699963,
-0.639737645699231,-0.636430661683604,-0.631180142899999,-0.607317004738094,
-0.583659683272591,-0.579984035916418,-0.5781545758962,-0.576812305898406,
-0.574979657766784,-0.571326877153677,-0.568669832407123,-0.564004018590832,
-0.543649580028403,-0.522133931197164,-0.517337810503212,-0.514411653907558,
-0.511726202112982,-0.508181299774085,-0.500134417949507,-0.488553912624194,
-0.47402647844802,-0.455327241911143,-0.452308382772382,-0.450603032831665,
-0.449080856939599,-0.446943006495797,-0.441527973681299,-0.436941316139848,
-0.417217420032999,-0.394939896062259,-0.39016139982296,-0.38724141816417,
-0.384558816089793,-0.381013781139237,-0.372951530440752,-0.361344608985499,
-0.34675015436894,-0.327966938021777,-0.324947921403686,-0.323245627857243,
-0.321727506028327,-0.319599527645496,-0.314236176964177,-0.309709986991027,
-0.290449445942093,-0.269445252832055,-0.264191031941215,-0.260873983802779,
-0.258219522360854,-0.255177697464234,-0.249806411144251,-0.243116288392084,
-0.227434139712926,-0.202197602112536,-0.198582957905506,-0.196739843945332,
-0.195212367729667,-0.193536227487522,-0.190639190152574,-0.17599882191069,
-0.142967169524369,-0.136696940021199,-0.133468587600331,-0.130864095882273,
-0.127909473341464,-0.124774710473348,-0.112133632282807,-0.090175540155627,
-0.0731777383191034,-0.0701813756983897,-0.068483582301325,-0.0669627322876045,
-0.0648218228567381,-0.0593784514073219,-0.0575108321596313,-0.0516968829590682,
-0.0292266003357285,-0.0203116323057249,-0.010850371782216,-0.00707572352057534,
-0.0043886250177014,-0.00223372215546031,-0.000389518114393014),
 .UNSPECIFIED.);
#810=B_SPLINE_CURVE_WITH_KNOTS('',3,(#73717,#73718,#73719,#73720,#73721,
#73722,#73723,#73724,#73725,#73726,#73727,#73728,#73729,#73730,#73731,#73732,
#73733,#73734,#73735,#73736,#73737,#73738,#73739,#73740,#73741,#73742),
 .UNSPECIFIED.,.F.,.F.,(4,2,2,2,2,2,2,2,2,2,2,2,4),(-1.60432934360076,-1.6017175531892,
-1.59737603752716,-1.57573503141855,-1.55340729196558,-1.54803406782767,
-1.54590447709287,-1.54438628912393,-1.54268566933008,-1.53967125642436,
-1.52098345817347,-1.50653753337139,-1.49484735329919),.UNSPECIFIED.);
#811=B_SPLINE_CURVE_WITH_KNOTS('',3,(#73744,#73745,#73746,#73747,#73748,
#73749,#73750,#73751,#73752,#73753,#73754,#73755,#73756,#73757,#73758,#73759,
#73760,#73761,#73762,#73763,#73764,#73765,#73766,#73767,#73768),
 .UNSPECIFIED.,.F.,.F.,(4,3,3,3,3,3,3,3,4),(121.664501811606,121.781642468112,
121.898729879809,122.021536591726,122.138748597292,122.256040087996,122.373537832758,
122.38995672748,122.522113490002),.UNSPECIFIED.);
#812=B_SPLINE_CURVE_WITH_KNOTS('',3,(#73769,#73770,#73771,#73772,#73773,
#73774,#73775,#73776,#73777,#73778,#73779,#73780,#73781,#73782,#73783,#73784,
#73785,#73786,#73787,#73788,#73789,#73790,#73791,#73792,#73793,#73794,#73795,
#73796,#73797,#73798,#73799,#73800,#73801,#73802,#73803,#73804,#73805,#73806,
#73807,#73808,#73809,#73810,#73811,#73812,#73813,#73814,#73815,#73816,#73817,
#73818,#73819,#73820,#73821,#73822,#73823,#73824,#73825,#73826,#73827,#73828,
#73829,#73830,#73831,#73832,#73833,#73834,#73835,#73836,#73837,#73838,#73839,
#73840,#73841,#73842,#73843,#73844,#73845,#73846,#73847,#73848,#73849,#73850,
#73851,#73852,#73853,#73854,#73855,#73856,#73857,#73858,#73859,#73860,#73861,
#73862,#73863,#73864,#73865,#73866,#73867,#73868,#73869,#73870,#73871,#73872,
#73873,#73874,#73875,#73876,#73877,#73878,#73879,#73880,#73881,#73882,#73883,
#73884,#73885,#73886,#73887,#73888,#73889,#73890,#73891,#73892,#73893,#73894,
#73895,#73896,#73897,#73898,#73899,#73900,#73901,#73902,#73903,#73904,#73905,
#73906,#73907,#73908,#73909,#73910,#73911,#73912,#73913,#73914,#73915,#73916,
#73917,#73918,#73919,#73920,#73921,#73922,#73923,#73924,#73925,#73926,#73927,
#73928,#73929,#73930,#73931,#73932,#73933,#73934,#73935,#73936,#73937,#73938,
#73939,#73940,#73941,#73942,#73943,#73944),.UNSPECIFIED.,.F.,.F.,(4,2,2,
2,2,2,2,2,2,2,2,2,2,2,2,2,2,2,2,2,2,2,2,2,2,2,2,2,2,2,2,2,2,2,2,2,2,2,2,
2,2,2,2,2,2,2,2,2,2,2,2,2,2,2,2,2,2,2,2,2,2,2,2,2,2,2,2,2,2,2,2,2,2,2,2,
2,2,2,2,2,2,2,2,2,2,2,2,4),(0.693071669236789,0.698139480370448,0.701159145804299,
0.703549748828527,0.706767878550367,0.713019731837982,0.721193300910815,
0.744007185647916,0.760744345774809,0.763736737013293,0.765432136789302,
0.766951918442264,0.76909125399323,0.774526537050775,0.779140034139169,
0.799071535765026,0.82115054123654,0.825932508069584,0.828852336482292,
0.831533270601716,0.835073826443107,0.843115720755329,0.854682594518121,
0.86926813760988,0.88802725884411,0.89101038689015,0.892722152931211,0.894238006802906,
0.896348044187626,0.901589764195582,0.909634290722259,0.940249205308818,
0.94861430045093,0.953326133262378,0.956230627265531,0.958915444628075,
0.962487990685922,0.97073041562263,0.982715138785732,0.99327613972987,1.01404218243176,
1.01786618427992,1.01973164475163,1.0212270070191,1.02311312686503,1.02704593738579,
1.03245836805485,1.04798026679867,1.07405043982704,1.07924558177018,1.08254590067681,
1.08519974830861,1.08825492680061,1.09368877397592,1.10047962213288,1.11657082973311,
1.1418275443702,1.14533339886679,1.14715837449832,1.14850518700561,1.15035567698938,
1.15410208217629,1.16925486562512,1.19657645759496,1.20536281344284,1.20874555568777,
1.21123487604378,1.21395764252497,1.21776428684172,1.2275796837714,1.24319127644046,
1.26815672914931,1.2719479951072,1.27383431523484,1.27535716237261,1.27698857654572,
1.2794642809716,1.28262848955899,1.28919300781133,1.31196240089643,1.33064817936872,
1.33535100676426,1.33825327154474,1.34093821051274,1.34451420554197,1.3484685323124,
1.35535731767862,1.38572530886986),.UNSPECIFIED.);
#813=B_SPLINE_CURVE_WITH_KNOTS('',3,(#73948,#73949,#73950,#73951,#73952,
#73953,#73954,#73955,#73956,#73957,#73958,#73959,#73960,#73961,#73962,#73963,
#73964,#73965,#73966,#73967,#73968,#73969,#73970,#73971,#73972,#73973,#73974,
#73975,#73976,#73977,#73978,#73979,#73980,#73981,#73982,#73983,#73984,#73985,
#73986,#73987,#73988,#73989,#73990,#73991,#73992,#73993,#73994,#73995,#73996,
#73997,#73998,#73999,#74000,#74001,#74002,#74003,#74004,#74005,#74006,#74007,
#74008),.UNSPECIFIED.,.F.,.F.,(4,3,3,3,3,3,3,3,3,3,3,3,3,3,3,3,3,3,3,3,
4),(-4.04123713824992,-3.99002632784797,-3.88065880480044,-3.76964142243613,
-3.66057630191354,-3.55157904186602,-3.44260994457981,-3.33008739490635,
-3.22098672178644,-3.10675323383621,-2.99251974588598,-2.88328166339718,
-2.77224810096303,-2.66330470611944,-2.5544259875385,-2.4455720800857,-2.33293235104527,
-2.22393731289834,-2.10947523841116,-1.99501316392398,-1.98502202421803),
 .UNSPECIFIED.);
#814=B_SPLINE_CURVE_WITH_KNOTS('',3,(#74012,#74013,#74014,#74015,#74016),
 .UNSPECIFIED.,.F.,.F.,(4,1,4),(0.,0.997506581961993,1.08537753955764),
 .UNSPECIFIED.);
#815=B_SPLINE_CURVE_WITH_KNOTS('',3,(#74018,#74019,#74020,#74021,#74022,
#74023,#74024,#74025,#74026,#74027,#74028,#74029,#74030,#74031,#74032,#74033,
#74034,#74035,#74036,#74037,#74038,#74039,#74040,#74041,#74042,#74043,#74044,
#74045,#74046,#74047,#74048,#74049,#74050,#74051,#74052,#74053,#74054,#74055,
#74056,#74057,#74058,#74059,#74060,#74061,#74062,#74063,#74064,#74065,#74066,
#74067,#74068,#74069,#74070,#74071,#74072,#74073,#74074,#74075,#74076,#74077,
#74078,#74079,#74080,#74081,#74082,#74083,#74084,#74085,#74086,#74087,#74088,
#74089,#74090,#74091,#74092,#74093,#74094,#74095,#74096,#74097,#74098,#74099,
#74100,#74101,#74102,#74103,#74104,#74105,#74106,#74107,#74108,#74109,#74110,
#74111,#74112,#74113,#74114,#74115,#74116,#74117,#74118,#74119,#74120,#74121,
#74122,#74123,#74124,#74125,#74126,#74127,#74128,#74129,#74130,#74131,#74132,
#74133,#74134,#74135,#74136,#74137,#74138,#74139,#74140,#74141,#74142,#74143,
#74144,#74145,#74146,#74147,#74148,#74149,#74150,#74151,#74152,#74153,#74154,
#74155,#74156,#74157,#74158,#74159,#74160,#74161,#74162,#74163,#74164,#74165,
#74166,#74167,#74168,#74169,#74170,#74171,#74172,#74173,#74174,#74175,#74176,
#74177,#74178,#74179,#74180,#74181,#74182,#74183,#74184,#74185,#74186,#74187,
#74188,#74189,#74190,#74191,#74192,#74193,#74194,#74195),.UNSPECIFIED.,
 .F.,.F.,(4,3,3,3,3,3,3,3,3,3,3,3,3,3,3,3,3,3,3,3,3,3,3,3,3,3,3,3,3,3,3,
3,3,3,3,3,3,3,3,3,3,3,3,3,3,3,3,3,3,3,3,3,3,3,3,3,3,3,3,4),(1.08537753955764,
1.19237208039302,1.29918413117133,1.40589593993818,1.51255020384418,1.61918951761686,
1.72592914702087,1.83272395932984,1.93970883738257,1.99501316392399,2.10426582070635,
2.21529756135381,2.32424717166913,2.43312898501853,2.54198287098267,2.65461708970849,
2.76360437795769,2.87806206192184,2.99251974588598,3.10186876550467,3.21288846079758,
3.32194593157733,3.43093959586529,3.53990914493888,3.65243844066615,3.76154958654277,
3.87578795719537,3.99002632784798,4.09908565806964,4.21014156453718,4.31889683448837,
4.42758448166435,4.5362447001632,4.64906675257489,4.75786389897493,4.86673806894133,
4.97579377032075,4.98753290980997,5.09672274281777,5.20776233643704,5.31665180314716,
5.42547465207295,5.53427085876912,5.64696301701983,5.7558965477232,5.87046801974758,
5.98503949177196,6.09423082675942,6.20527023263123,6.31416227081442,6.4229880838998,
6.5317876437074,6.64447725121404,6.75341507275383,6.86798057324389,6.98254607373395,
7.10492809094954,7.2268464510175,7.34802169307296,7.36856284629668),
 .UNSPECIFIED.);
#816=B_SPLINE_CURVE_WITH_KNOTS('',3,(#74197,#74198,#74199,#74200,#74201,
#74202,#74203,#74204,#74205,#74206,#74207,#74208,#74209,#74210,#74211,#74212,
#74213,#74214,#74215,#74216,#74217,#74218,#74219,#74220,#74221,#74222,#74223,
#74224,#74225,#74226,#74227,#74228,#74229,#74230,#74231,#74232,#74233,#74234,
#74235,#74236,#74237,#74238,#74239,#74240,#74241,#74242,#74243,#74244,#74245,
#74246,#74247,#74248,#74249,#74250,#74251,#74252,#74253,#74254,#74255,#74256,
#74257,#74258,#74259,#74260,#74261,#74262,#74263,#74264,#74265,#74266,#74267,
#74268,#74269,#74270,#74271,#74272,#74273,#74274,#74275,#74276,#74277,#74278,
#74279,#74280,#74281,#74282,#74283,#74284,#74285,#74286,#74287,#74288,#74289,
#74290,#74291,#74292,#74293,#74294,#74295,#74296,#74297,#74298,#74299,#74300,
#74301,#74302,#74303,#74304,#74305,#74306,#74307,#74308,#74309,#74310,#74311,
#74312,#74313,#74314,#74315,#74316,#74317,#74318,#74319,#74320,#74321,#74322,
#74323,#74324,#74325,#74326,#74327,#74328,#74329,#74330,#74331,#74332,#74333,
#74334,#74335,#74336,#74337,#74338,#74339,#74340,#74341,#74342,#74343,#74344,
#74345,#74346,#74347,#74348,#74349,#74350,#74351,#74352,#74353,#74354,#74355,
#74356,#74357,#74358,#74359,#74360,#74361,#74362,#74363,#74364,#74365,#74366,
#74367,#74368,#74369,#74370,#74371),.UNSPECIFIED.,.F.,.F.,(4,3,3,3,3,3,
3,3,3,3,3,3,3,3,3,3,3,3,3,3,3,3,3,3,3,3,3,3,3,3,3,3,3,3,3,3,3,3,3,3,3,3,
3,3,3,3,3,3,3,3,3,3,3,3,3,3,3,3,4),(7.36856284673721,7.47844486294954,7.58835513743192,
7.69841751039424,7.8085631522594,7.91893214887187,7.98005265569595,8.08922828502025,
8.20026965409996,8.3091450252022,8.4179538590293,8.52673615478103,8.63944192550026,
8.74836197033257,8.86296060399525,8.97755923765794,9.08673359194986,9.19777512040862,
9.30664929434707,9.41545696352864,9.52423812919371,9.63694505180026,9.74586406663919,
9.86046494312956,9.97506581961993,10.0842364222147,10.1952784196356,10.3041486612738,
10.4129523417652,10.5217294688119,10.6344402020044,10.7433551001326,10.8579637508572,
10.9725724015819,11.0817453572512,11.1927870605378,11.3016597337144,11.4104658681936,
11.519245467665,11.6319538466347,11.7408712345231,11.8554751090335,11.9700789835439,
12.0792516006844,12.1902933462871,12.299165683508,12.4079714839463,12.5167507518537,
12.6294594552667,12.7383765217031,12.8529810436045,12.9675855655059,13.0763258634871,
13.1849044295828,13.2933621425984,13.4017517461816,13.5101030392779,13.6184871728317,
13.6517481539168),.UNSPECIFIED.);
#817=B_SPLINE_CURVE_WITH_KNOTS('',3,(#74373,#74374,#74375,#74376,#74377,
#74378,#74379,#74380,#74381,#74382,#74383,#74384,#74385,#74386,#74387,#74388,
#74389,#74390,#74391,#74392,#74393,#74394,#74395,#74396,#74397,#74398,#74399,
#74400,#74401,#74402,#74403,#74404,#74405,#74406,#74407,#74408,#74409,#74410,
#74411,#74412,#74413,#74414,#74415,#74416,#74417,#74418,#74419,#74420,#74421,
#74422,#74423,#74424,#74425,#74426,#74427,#74428,#74429,#74430,#74431,#74432,
#74433,#74434,#74435,#74436,#74437,#74438,#74439,#74440,#74441,#74442,#74443,
#74444,#74445,#74446,#74447,#74448,#74449,#74450,#74451,#74452,#74453,#74454,
#74455,#74456,#74457,#74458,#74459,#74460,#74461,#74462,#74463,#74464,#74465,
#74466,#74467,#74468,#74469,#74470,#74471,#74472,#74473,#74474,#74475,#74476,
#74477,#74478,#74479,#74480,#74481,#74482,#74483,#74484,#74485,#74486,#74487,
#74488,#74489,#74490,#74491,#74492,#74493,#74494,#74495,#74496,#74497,#74498,
#74499,#74500,#74501,#74502,#74503,#74504,#74505,#74506,#74507,#74508,#74509,
#74510,#74511,#74512,#74513,#74514,#74515,#74516,#74517,#74518,#74519,#74520,
#74521,#74522,#74523,#74524,#74525,#74526,#74527,#74528,#74529,#74530,#74531,
#74532,#74533,#74534,#74535,#74536,#74537,#74538,#74539,#74540,#74541,#74542,
#74543,#74544),.UNSPECIFIED.,.F.,.F.,(4,3,3,3,3,3,3,3,3,3,3,3,3,3,3,3,3,
3,3,3,3,3,3,3,3,3,3,3,3,3,3,3,3,3,3,3,3,3,3,3,3,3,3,3,3,3,3,3,3,3,3,3,3,
3,3,3,3,4),(13.6517481542948,13.7807998321804,13.9114792371605,13.9650921474679,
14.0742646640749,14.1853064222443,14.2941786486733,14.4029843347975,14.5117634850477,
14.6244722961433,14.7333892379024,14.8479939836662,14.9625987294299,15.0717711822896,
15.1828129484274,15.2916851105296,15.4004907322928,15.5092698182548,15.621978691539,
15.7308955699467,15.8455004406693,15.9601053113919,16.0692777228638,16.1803194941751,
16.2891916125174,16.3979971897579,16.5067762305057,16.6194851462177,16.7284019782044,
16.8430069357792,16.9576118933539,17.066784343201,17.1778261097154,17.2866982678641,
17.3955038853332,17.5042829666664,17.6169918438287,17.7259087168211,17.8405135960685,
17.9551184753159,18.0642909146953,18.1753326825181,18.2842048300158,18.3930104367955,
18.5017895074187,18.6144983948835,18.7234152572394,18.8380201572587,18.9526250572779,
19.0615109035367,19.1706887231708,19.2792768455527,19.3877990279444,19.4962957334554,
19.605955165244,19.7145896233196,19.8247615419647,19.9349334606099),
 .UNSPECIFIED.);
#818=B_SPLINE_CURVE_WITH_KNOTS('',3,(#74546,#74547,#74548,#74549,#74550,
#74551,#74552,#74553,#74554,#74555,#74556,#74557,#74558,#74559,#74560,#74561,
#74562,#74563,#74564,#74565,#74566,#74567,#74568,#74569,#74570,#74571,#74572,
#74573,#74574,#74575,#74576,#74577,#74578,#74579,#74580,#74581,#74582,#74583,
#74584,#74585,#74586,#74587,#74588,#74589,#74590,#74591,#74592,#74593,#74594,
#74595,#74596,#74597,#74598,#74599,#74600,#74601,#74602,#74603,#74604,#74605,
#74606,#74607,#74608,#74609,#74610,#74611,#74612,#74613,#74614,#74615,#74616,
#74617,#74618,#74619,#74620,#74621,#74622,#74623,#74624,#74625,#74626,#74627,
#74628,#74629,#74630,#74631,#74632,#74633,#74634,#74635,#74636,#74637,#74638,
#74639,#74640,#74641,#74642,#74643,#74644,#74645,#74646,#74647,#74648,#74649,
#74650,#74651,#74652,#74653,#74654,#74655,#74656,#74657,#74658,#74659,#74660,
#74661,#74662,#74663,#74664,#74665,#74666,#74667,#74668,#74669,#74670,#74671,
#74672,#74673,#74674,#74675,#74676,#74677,#74678,#74679,#74680,#74681,#74682,
#74683,#74684,#74685,#74686,#74687,#74688,#74689,#74690,#74691,#74692,#74693,
#74694,#74695,#74696,#74697,#74698,#74699,#74700,#74701,#74702,#74703,#74704,
#74705,#74706,#74707,#74708,#74709,#74710,#74711,#74712,#74713,#74714,#74715,
#74716,#74717,#74718,#74719,#74720),.UNSPECIFIED.,.F.,.F.,(4,3,3,3,3,3,
3,3,3,3,3,3,3,3,3,3,3,3,3,3,3,3,3,3,3,3,3,3,3,3,3,3,3,3,3,3,3,3,3,3,3,3,
3,3,3,3,3,3,3,3,3,3,3,3,3,3,3,3,4),(19.9349334610964,19.9501316392399,20.059304079444,
20.1703458471637,20.2792179954136,20.3880236029164,20.496802674232,20.6095115609745,
20.7184284239382,20.83303332257,20.9476382212018,21.0568106598144,21.167852427733,
21.2767245743552,21.3855301802213,21.494309249894,21.6070181382114,21.7159349995358,
21.8305399013498,21.9451448031638,22.0543172414554,22.1653590094142,22.2742311556886,
22.3830367611979,22.4918158305054,22.6045247191605,22.7134415801027,22.8280464826142,
22.9426513851258,23.0518238239892,23.1628655918765,23.2717377387463,23.3805433448581,
23.4893224147742,23.6020313028526,23.7109481644118,23.8255530657498,23.9401579670878,
24.0493304057212,24.1603721736373,24.269244320271,24.3780499261452,24.4868289958225,
24.5995378841293,24.7084547454493,24.8230596472496,24.9376645490498,25.0468369876651,
25.1578787555834,25.2667509021965,25.375556508049,25.4843355777038,25.5970444660308,
25.7059613273264,25.8205662291691,25.9351711310118,26.0766449493812,26.2101144995944,
26.2181187677507),.UNSPECIFIED.);
#819=B_SPLINE_CURVE_WITH_KNOTS('',3,(#74722,#74723,#74724,#74725,#74726,
#74727,#74728,#74729,#74730,#74731,#74732,#74733,#74734,#74735,#74736,#74737,
#74738,#74739,#74740,#74741,#74742,#74743,#74744,#74745,#74746,#74747,#74748,
#74749,#74750,#74751,#74752,#74753,#74754,#74755,#74756,#74757,#74758,#74759,
#74760,#74761,#74762,#74763,#74764,#74765,#74766,#74767,#74768,#74769,#74770,
#74771,#74772,#74773,#74774,#74775,#74776,#74777,#74778,#74779,#74780,#74781,
#74782,#74783,#74784,#74785,#74786,#74787,#74788,#74789,#74790,#74791,#74792,
#74793,#74794,#74795,#74796,#74797,#74798,#74799,#74800,#74801,#74802,#74803,
#74804,#74805,#74806,#74807,#74808,#74809,#74810,#74811,#74812,#74813,#74814,
#74815,#74816,#74817,#74818,#74819,#74820,#74821,#74822,#74823,#74824,#74825,
#74826,#74827,#74828,#74829,#74830,#74831,#74832,#74833,#74834,#74835,#74836,
#74837,#74838,#74839,#74840,#74841,#74842,#74843,#74844,#74845,#74846,#74847,
#74848,#74849,#74850,#74851,#74852,#74853,#74854,#74855,#74856,#74857,#74858,
#74859,#74860,#74861,#74862,#74863,#74864,#74865,#74866,#74867,#74868,#74869,
#74870,#74871,#74872,#74873,#74874,#74875,#74876,#74877,#74878,#74879,#74880,
#74881,#74882,#74883,#74884,#74885,#74886,#74887,#74888,#74889,#74890,#74891,
#74892,#74893,#74894,#74895,#74896),.UNSPECIFIED.,.F.,.F.,(4,3,3,3,3,3,
3,3,3,3,3,3,3,3,3,3,3,3,3,3,3,3,3,3,3,3,3,3,3,3,3,3,3,3,3,3,3,3,3,3,3,3,
3,3,3,3,3,3,3,3,3,3,3,3,3,3,3,3,4),(26.218118768276,26.3260897132672,26.4340090703127,
26.5419180814198,26.6499336004416,26.7580059949489,26.8662760152752,26.9326777129738,
27.0418501516244,27.1528919195383,27.2617640661886,27.3705696720791,27.4793487417723,
27.5920576300632,27.7009744913982,27.815579393167,27.9301842949358,28.0393567335869,
28.1503985015008,28.2592706481514,28.3680762540422,28.4768553237355,28.5895642120261,
28.6984810733612,28.8130859751295,28.9276908768978,29.0368633155567,29.1479050834696,
29.2567772301283,29.3655828360272,29.4743619057289,29.5870707940116,29.6959876553551,
29.8105925571075,29.9251974588598,30.0343698975143,30.1454116654277,30.2542838120819,
30.3630894179761,30.4718684876732,30.5845773759603,30.693494237299,30.8080991390604,
30.9227040408218,31.0318764794768,31.1429182473902,31.2517903940449,31.3605959999397,
31.4693750696373,31.5820839579239,31.6910008192631,31.8056057210235,31.9202106227838,
32.0315396882388,32.1426749812362,32.2536208585234,32.3644559905224,32.4752076844519,
32.5013040754555),.UNSPECIFIED.);
#820=B_SPLINE_CURVE_WITH_KNOTS('',3,(#74898,#74899,#74900,#74901,#74902,
#74903,#74904,#74905,#74906,#74907,#74908,#74909,#74910,#74911,#74912,#74913,
#74914,#74915,#74916,#74917,#74918,#74919,#74920,#74921,#74922,#74923,#74924,
#74925,#74926,#74927,#74928,#74929,#74930,#74931,#74932,#74933,#74934,#74935,
#74936,#74937,#74938,#74939,#74940,#74941,#74942,#74943,#74944,#74945,#74946,
#74947,#74948,#74949,#74950,#74951,#74952,#74953,#74954,#74955,#74956,#74957,
#74958,#74959,#74960,#74961,#74962,#74963,#74964,#74965,#74966,#74967,#74968,
#74969,#74970,#74971,#74972,#74973,#74974,#74975,#74976,#74977,#74978,#74979,
#74980,#74981,#74982,#74983,#74984,#74985,#74986,#74987,#74988,#74989,#74990,
#74991,#74992,#74993,#74994,#74995,#74996,#74997,#74998,#74999,#75000,#75001,
#75002,#75003,#75004,#75005,#75006,#75007,#75008,#75009,#75010,#75011,#75012,
#75013,#75014,#75015,#75016,#75017,#75018,#75019,#75020,#75021,#75022,#75023,
#75024,#75025,#75026,#75027,#75028,#75029,#75030,#75031,#75032,#75033,#75034,
#75035,#75036,#75037,#75038,#75039,#75040,#75041,#75042,#75043,#75044,#75045,
#75046,#75047,#75048,#75049,#75050,#75051,#75052,#75053,#75054,#75055,#75056,
#75057,#75058,#75059,#75060,#75061,#75062,#75063,#75064,#75065,#75066,#75067,
#75068,#75069,#75070,#75071,#75072),.UNSPECIFIED.,.F.,.F.,(4,3,3,3,3,3,
3,3,3,3,3,3,3,3,3,3,3,3,3,3,3,3,3,3,3,3,3,3,3,3,3,3,3,3,3,3,3,3,3,3,3,3,
3,3,3,3,3,3,3,3,3,3,3,3,3,3,3,3,4),(32.501304075825,32.6202820172976,32.7396425606215,
32.8595408410294,32.9177172047458,33.026889643401,33.1379314113144,33.2468035579693,
33.3556091638644,33.4643882335622,33.5770971218486,33.6860139831881,33.800618884948,
33.9152237867078,34.0243962253632,34.1354379932765,34.2443101399316,34.3531157458268,
34.4618948155248,34.574603703811,34.6835205651507,34.7981254669102,34.9127303686697,
35.0219028073251,35.1329445752384,35.2418167218935,35.3506223277888,35.4594013974868,
35.5721102857731,35.6810271471128,35.7956320488722,35.9102369506317,36.019409389287,
36.1304511572004,36.2393233038555,36.3481289097506,36.4569079794486,36.5696168677349,
36.6785337290746,36.7931386308341,36.9077435325937,37.0169159712491,37.1279577391624,
37.2368298858175,37.3456354917128,37.4544145614108,37.567123449697,37.6760403110367,
37.7906452127962,37.9052501145557,38.0151550230095,38.1226501109105,38.2300416406864,
38.3373717088353,38.449151127173,38.5565434348571,38.6639882702517,38.7715852654564,
38.7844893821862),.UNSPECIFIED.);
#821=B_SPLINE_CURVE_WITH_KNOTS('',3,(#75074,#75075,#75076,#75077,#75078,
#75079,#75080,#75081,#75082,#75083,#75084,#75085,#75086,#75087,#75088,#75089,
#75090,#75091,#75092,#75093,#75094,#75095,#75096,#75097,#75098,#75099,#75100,
#75101,#75102,#75103,#75104,#75105,#75106,#75107,#75108,#75109,#75110,#75111,
#75112,#75113,#75114,#75115,#75116,#75117,#75118,#75119,#75120,#75121,#75122,
#75123,#75124,#75125,#75126,#75127,#75128,#75129,#75130,#75131,#75132,#75133,
#75134,#75135,#75136,#75137,#75138,#75139,#75140,#75141,#75142,#75143,#75144,
#75145,#75146,#75147,#75148,#75149,#75150,#75151,#75152,#75153,#75154,#75155,
#75156,#75157,#75158,#75159,#75160,#75161,#75162,#75163,#75164,#75165,#75166,
#75167,#75168,#75169,#75170,#75171,#75172,#75173,#75174,#75175,#75176,#75177,
#75178,#75179,#75180,#75181,#75182,#75183,#75184,#75185,#75186,#75187,#75188,
#75189,#75190,#75191,#75192,#75193,#75194,#75195,#75196,#75197,#75198,#75199,
#75200,#75201,#75202,#75203,#75204,#75205,#75206,#75207,#75208,#75209,#75210,
#75211,#75212,#75213,#75214,#75215,#75216,#75217,#75218,#75219,#75220,#75221,
#75222,#75223,#75224,#75225,#75226,#75227,#75228,#75229,#75230,#75231,#75232,
#75233,#75234,#75235,#75236,#75237,#75238,#75239,#75240,#75241,#75242,#75243,
#75244,#75245),.UNSPECIFIED.,.F.,.F.,(4,3,3,3,3,3,3,3,3,3,3,3,3,3,3,3,3,
3,3,3,3,3,3,3,3,3,3,3,3,3,3,3,3,3,3,3,3,3,3,3,3,3,3,3,3,3,3,3,3,3,3,3,3,
3,3,3,3,4),(38.7844893826352,38.9027566965177,39.0119291351729,39.1229709030862,
39.2318430497411,39.3406486556361,39.4494277253338,39.5621366136203,39.6710534749597,
39.7856583767197,39.9002632784797,40.0094357171351,40.1204774850484,40.2293496317034,
40.3381552375986,40.4469343072967,40.5596431955829,40.6685600569226,40.7831649586822,
40.8977698604417,41.0069422990971,41.1179840670104,41.2268562136655,41.3356618195608,
41.4444408892588,41.557149777545,41.6660666388848,41.7806715406442,41.8952764424037,
42.0044488810591,42.1154906489724,42.2243627956275,42.3331684015227,42.4419474712208,
42.554656359507,42.6635732208467,42.7781781226062,42.8927830243657,43.001955463021,
43.1129972309344,43.2218693775894,43.3306749834846,43.4394540531826,43.5521629414689,
43.6610798028085,43.7756847045681,43.8902896063277,43.9994620449831,44.1105038128964,
44.2193759595516,44.3281815654469,44.4369606351449,44.5496695234311,44.6585863847709,
44.7731912865303,44.8877961882897,45.0529483136957,45.0676746898147),
 .UNSPECIFIED.);
#822=B_SPLINE_CURVE_WITH_KNOTS('',3,(#75247,#75248,#75249,#75250,#75251,
#75252,#75253,#75254,#75255,#75256,#75257,#75258,#75259,#75260,#75261,#75262,
#75263,#75264,#75265,#75266,#75267,#75268,#75269,#75270,#75271,#75272,#75273,
#75274,#75275,#75276,#75277,#75278,#75279,#75280,#75281,#75282,#75283,#75284,
#75285,#75286,#75287,#75288,#75289,#75290,#75291,#75292,#75293,#75294,#75295,
#75296,#75297,#75298,#75299,#75300,#75301,#75302,#75303,#75304,#75305,#75306,
#75307,#75308,#75309,#75310,#75311,#75312,#75313,#75314,#75315,#75316,#75317,
#75318,#75319,#75320,#75321,#75322,#75323,#75324,#75325,#75326,#75327,#75328,
#75329,#75330,#75331,#75332,#75333,#75334,#75335,#75336,#75337,#75338,#75339,
#75340,#75341,#75342,#75343,#75344,#75345,#75346,#75347,#75348,#75349,#75350,
#75351,#75352,#75353,#75354,#75355,#75356,#75357,#75358,#75359,#75360,#75361,
#75362,#75363,#75364,#75365,#75366,#75367,#75368,#75369,#75370,#75371,#75372,
#75373,#75374,#75375,#75376,#75377,#75378,#75379,#75380,#75381,#75382,#75383,
#75384,#75385,#75386,#75387,#75388,#75389,#75390,#75391,#75392,#75393,#75394,
#75395,#75396,#75397,#75398,#75399,#75400,#75401,#75402,#75403,#75404,#75405,
#75406,#75407,#75408,#75409,#75410,#75411,#75412,#75413,#75414,#75415,#75416,
#75417,#75418,#75419,#75420,#75421),.UNSPECIFIED.,.F.,.F.,(4,3,3,3,3,3,
3,3,3,3,3,3,3,3,3,3,3,3,3,3,3,3,3,3,3,3,3,3,3,3,3,3,3,3,3,3,3,3,3,3,3,3,
3,3,3,3,3,3,3,3,3,3,3,3,3,3,3,3,4),(45.0676746903426,45.1750415219094,45.2823049101596,
45.3895070927842,45.4966902086682,45.6039694274682,45.711299424467,45.8188205351401,
45.8853027702517,45.994475208907,46.1055169768203,46.2143891234754,46.3231947293705,
46.4319737990685,46.5446826873548,46.6535995486945,46.7682044504541,46.8828093522137,
46.9919817908691,47.1030235587824,47.2118957054375,47.3207013113326,47.4294803810306,
47.5421892693169,47.6511061306565,47.765711032416,47.8803159341756,47.989488372831,
48.1005301407443,48.2094022873994,48.3182078932946,48.4269869629926,48.5396958512789,
48.6486127126186,48.7632176143781,48.8778225161376,48.9869949547929,49.0980367227062,
49.2069088693613,49.3157144752566,49.4244935449546,49.5372024332409,49.6461192945806,
49.7607241963401,49.8753290980996,49.9845015367549,50.0955433046682,50.2044154513233,
50.3132210572187,50.4220001269168,50.534709015203,50.6436258765428,50.7582307783022,
50.8728356800616,50.9923417591862,51.1078495281233,51.2231187442687,51.3380919842859,
51.35085999656),.UNSPECIFIED.);
#823=B_SPLINE_CURVE_WITH_KNOTS('',3,(#75423,#75424,#75425,#75426,#75427,
#75428,#75429,#75430,#75431,#75432,#75433,#75434,#75435,#75436,#75437,#75438,
#75439,#75440,#75441,#75442,#75443,#75444,#75445,#75446,#75447,#75448,#75449,
#75450,#75451,#75452,#75453,#75454,#75455,#75456,#75457,#75458,#75459,#75460,
#75461,#75462,#75463,#75464,#75465,#75466,#75467,#75468,#75469,#75470,#75471,
#75472,#75473,#75474,#75475,#75476,#75477,#75478,#75479,#75480,#75481,#75482,
#75483,#75484,#75485,#75486,#75487,#75488,#75489,#75490,#75491,#75492,#75493,
#75494,#75495,#75496,#75497,#75498,#75499,#75500,#75501,#75502,#75503,#75504,
#75505,#75506,#75507,#75508,#75509,#75510,#75511,#75512,#75513,#75514,#75515,
#75516,#75517,#75518,#75519,#75520,#75521,#75522,#75523,#75524,#75525,#75526,
#75527,#75528,#75529,#75530,#75531,#75532,#75533,#75534,#75535,#75536,#75537,
#75538,#75539,#75540,#75541,#75542,#75543,#75544,#75545,#75546,#75547,#75548,
#75549,#75550,#75551,#75552,#75553,#75554,#75555,#75556,#75557,#75558,#75559,
#75560,#75561,#75562,#75563,#75564,#75565,#75566,#75567,#75568,#75569,#75570,
#75571,#75572,#75573,#75574,#75575,#75576,#75577,#75578,#75579,#75580,#75581,
#75582,#75583,#75584,#75585,#75586,#75587,#75588,#75589,#75590,#75591,#75592,
#75593,#75594,#75595,#75596,#75597),.UNSPECIFIED.,.F.,.F.,(4,3,3,3,3,3,
3,3,3,3,3,3,3,3,3,3,3,3,3,3,3,3,3,3,3,3,3,3,3,3,3,3,3,3,3,3,3,3,3,3,3,3,
3,3,3,3,3,3,3,3,3,3,3,3,3,3,3,3,4),(51.3508599969944,51.4638640035928,51.5771436363338,
51.6905694161473,51.8042913248099,51.8703422620236,51.9795147006789,52.0905564685923,
52.1994286152473,52.3082342211425,52.4170132908405,52.5297221791268,52.6386390404664,
52.753243942226,52.8678488439856,52.977021282641,53.0880630505543,53.1969351972094,
53.3057408031046,53.4145198728028,53.527228761089,53.6361456224286,53.7507505241881,
53.8653554259476,53.9745278646031,54.0855696325164,54.1944417791714,54.3032473850665,
54.4120264547646,54.5247353430508,54.6336522043904,54.74825710615,54.8628620079096,
54.9720344465651,55.0830762144784,55.1919483611336,55.3007539670289,55.4095330367269,
55.5222419250131,55.6311587863528,55.7457636881122,55.8603685898716,55.969541028527,
56.0805827964403,56.1894549430954,56.2982605489907,56.4070396186886,56.5197485069748,
56.6286653683146,56.7432702700741,56.8578751718336,56.9655412073146,57.0730567352133,
57.1804640188214,57.2878051514156,57.3951602707806,57.5025261982831,57.6099931887045,
57.6340453036562),.UNSPECIFIED.);
#824=B_SPLINE_CURVE_WITH_KNOTS('',3,(#75599,#75600,#75601,#75602,#75603,
#75604,#75605,#75606,#75607,#75608,#75609,#75610,#75611,#75612,#75613,#75614,
#75615,#75616,#75617,#75618,#75619,#75620,#75621,#75622,#75623,#75624,#75625,
#75626,#75627,#75628,#75629,#75630,#75631,#75632,#75633,#75634,#75635,#75636,
#75637,#75638,#75639,#75640,#75641,#75642,#75643,#75644,#75645,#75646,#75647,
#75648,#75649,#75650,#75651,#75652,#75653,#75654,#75655,#75656,#75657,#75658,
#75659,#75660,#75661,#75662,#75663,#75664,#75665,#75666,#75667,#75668,#75669,
#75670,#75671,#75672,#75673,#75674,#75675,#75676,#75677,#75678,#75679,#75680,
#75681,#75682,#75683,#75684,#75685,#75686,#75687,#75688,#75689,#75690,#75691,
#75692,#75693,#75694,#75695,#75696,#75697,#75698,#75699,#75700,#75701,#75702,
#75703,#75704,#75705,#75706,#75707,#75708,#75709,#75710,#75711,#75712,#75713,
#75714,#75715,#75716,#75717,#75718,#75719,#75720,#75721,#75722,#75723,#75724,
#75725,#75726,#75727,#75728,#75729,#75730,#75731,#75732,#75733,#75734,#75735,
#75736,#75737,#75738,#75739,#75740,#75741,#75742,#75743,#75744,#75745,#75746,
#75747,#75748,#75749,#75750,#75751,#75752,#75753,#75754,#75755,#75756,#75757,
#75758,#75759,#75760,#75761,#75762,#75763,#75764,#75765,#75766,#75767,#75768,
#75769,#75770),.UNSPECIFIED.,.F.,.F.,(4,3,3,3,3,3,3,3,3,3,3,3,3,3,3,3,3,
3,3,3,3,3,3,3,3,3,3,3,3,3,3,3,3,3,3,3,3,3,3,3,3,3,3,3,3,3,3,3,3,3,3,3,3,
3,3,3,3,4),(57.6340453041739,57.7828045081191,57.8553817537956,57.9645541924508,
58.0755959603642,58.1844681070192,58.2932737129144,58.4020527826123,58.5147616708987,
58.6236785322383,58.7382834339979,58.8528883357576,58.9620607744129,59.0731025423262,
59.1819746889812,59.2907802948764,59.3995593645744,59.5122682528606,59.6211851142003,
59.7357900159599,59.8503949177195,59.9595673563749,60.0706091242882,60.1794812709433,
60.2882868768386,60.3970659465366,60.5097748348228,60.6186916961625,60.733296597922,
60.8479014996815,60.9570739383369,61.0681157062502,61.1769878529053,61.2857934588005,
61.3945725284986,61.5072814167848,61.6161982781245,61.730803179884,61.8454080816435,
61.9545805202989,62.0656222882122,62.1744944348673,62.2833000407625,62.3920791104606,
62.5047879987468,62.6137048600865,62.728309761846,62.8429146636055,62.9520871022609,
63.0631288701742,63.1720010168293,63.2808066227245,63.3895856924226,63.5022945807089,
63.6112114420486,63.725816343808,63.8404212455675,63.9172306113535),
 .UNSPECIFIED.);
#825=B_SPLINE_CURVE_WITH_KNOTS('',3,(#75772,#75773,#75774,#75775,#75776,
#75777,#75778,#75779,#75780,#75781,#75782,#75783,#75784,#75785,#75786,#75787,
#75788,#75789,#75790,#75791,#75792,#75793,#75794,#75795,#75796,#75797,#75798,
#75799,#75800,#75801,#75802,#75803,#75804,#75805,#75806,#75807,#75808,#75809,
#75810,#75811,#75812,#75813,#75814,#75815,#75816,#75817,#75818,#75819,#75820,
#75821,#75822,#75823,#75824,#75825,#75826,#75827,#75828,#75829,#75830,#75831,
#75832,#75833,#75834,#75835,#75836,#75837,#75838,#75839,#75840,#75841,#75842,
#75843,#75844,#75845,#75846,#75847,#75848,#75849,#75850,#75851,#75852,#75853,
#75854,#75855,#75856,#75857,#75858,#75859,#75860,#75861,#75862,#75863,#75864,
#75865,#75866,#75867,#75868,#75869,#75870,#75871,#75872,#75873,#75874,#75875,
#75876,#75877,#75878,#75879,#75880,#75881,#75882,#75883,#75884,#75885,#75886,
#75887,#75888,#75889,#75890,#75891,#75892,#75893,#75894,#75895,#75896,#75897,
#75898,#75899,#75900,#75901,#75902,#75903,#75904,#75905,#75906,#75907,#75908,
#75909,#75910,#75911,#75912,#75913,#75914,#75915,#75916,#75917,#75918,#75919,
#75920,#75921,#75922,#75923,#75924,#75925,#75926,#75927,#75928,#75929,#75930,
#75931,#75932,#75933,#75934,#75935,#75936,#75937,#75938,#75939,#75940,#75941,
#75942,#75943),.UNSPECIFIED.,.F.,.F.,(4,3,3,3,3,3,3,3,3,3,3,3,3,3,3,3,3,
3,3,3,3,3,3,3,3,3,3,3,3,3,3,3,3,3,3,3,3,3,3,3,3,3,3,3,3,3,3,3,3,3,3,3,3,
3,3,3,3,4),(63.9172306117697,64.0252086767897,64.133012703545,64.2407214388638,
64.3483765813558,64.456019747366,64.5637655410965,64.6715675260603,64.7795605025846,
64.8379278275295,64.9471002661847,65.0581420340981,65.1670141807532,65.2758197866484,
65.3845988563465,65.4973077446327,65.6062246059724,65.720829507732,65.8354344094915,
65.9446068481468,66.0556486160601,66.1645207627152,66.2733263686105,66.3821054383085,
66.4948143265948,66.6037311879345,66.718336089694,66.8329409914535,66.9421134301088,
67.0531551980222,67.1620273446773,67.2708329505726,67.3796120202706,67.4923209085568,
67.6012377698965,67.715842671656,67.8304475734155,67.9396200120708,68.0506617799842,
68.1595339266392,68.2683395325344,68.3771186022324,68.4898274905187,68.5987443518583,
68.7133492536179,68.8279541553775,68.9371265940329,69.0481683619462,69.1570405086014,
69.2658461144964,69.3746251841943,69.4873340724806,69.5962509338203,69.7108558355799,
69.8254607373395,69.9489215589145,70.0746687384978,70.2004159180811),
 .UNSPECIFIED.);
#826=B_SPLINE_CURVE_WITH_KNOTS('',3,(#75945,#75946,#75947,#75948,#75949,
#75950,#75951,#75952,#75953,#75954,#75955,#75956,#75957,#75958,#75959,#75960,
#75961,#75962,#75963,#75964,#75965,#75966,#75967,#75968,#75969,#75970,#75971,
#75972,#75973,#75974,#75975,#75976,#75977,#75978,#75979,#75980,#75981,#75982,
#75983,#75984,#75985,#75986,#75987,#75988,#75989,#75990,#75991,#75992,#75993,
#75994,#75995,#75996,#75997,#75998,#75999,#76000,#76001,#76002,#76003,#76004,
#76005,#76006,#76007,#76008,#76009,#76010,#76011,#76012,#76013,#76014,#76015,
#76016,#76017,#76018,#76019,#76020,#76021,#76022,#76023,#76024,#76025,#76026,
#76027,#76028,#76029,#76030,#76031,#76032,#76033,#76034,#76035,#76036,#76037,
#76038,#76039,#76040,#76041,#76042,#76043,#76044,#76045,#76046,#76047,#76048,
#76049,#76050,#76051,#76052,#76053,#76054,#76055,#76056,#76057,#76058,#76059,
#76060,#76061,#76062,#76063,#76064,#76065,#76066,#76067,#76068,#76069,#76070,
#76071,#76072,#76073,#76074,#76075,#76076,#76077,#76078,#76079,#76080,#76081,
#76082,#76083,#76084,#76085,#76086,#76087,#76088,#76089,#76090,#76091,#76092,
#76093,#76094,#76095,#76096,#76097,#76098,#76099,#76100,#76101,#76102,#76103,
#76104,#76105,#76106,#76107,#76108,#76109,#76110,#76111,#76112,#76113,#76114,
#76115,#76116,#76117,#76118,#76119),.UNSPECIFIED.,.F.,.F.,(4,3,3,3,3,3,
3,3,3,3,3,3,3,3,3,3,3,3,3,3,3,3,3,3,3,3,3,3,3,3,3,3,3,3,3,3,3,3,3,3,3,3,
3,3,3,3,3,3,3,3,3,3,3,3,3,3,3,3,4),(70.2004159185332,70.3100324153458,70.4196665537124,
70.5294427104895,70.6392940861559,70.7493686748722,70.8229673193015,70.9321397579569,
71.0431815258702,71.1520536725254,71.2608592784206,71.3696383481187,71.4823472364049,
71.5912640977445,71.705868999504,71.8204739012635,71.9296463399186,72.040688107832,
72.149560254487,72.2583658603823,72.3671449300802,72.4798538183665,72.5887706797061,
72.7033755814658,72.8179804832255,72.9271529218808,73.0381946897941,73.1470668364492,
73.2558724423444,73.3646515120424,73.4773604003287,73.5862772616684,73.7008821634279,
73.8154870651875,73.924659503843,74.0357012717563,74.1445734184114,74.2533790243066,
74.3621580940044,74.4748669822907,74.5837838436304,74.6983887453899,74.8129936471494,
74.9221660858047,75.0332078537181,75.1420800003732,75.2508856062684,75.3596646759663,
75.4723735642526,75.5812904255922,75.6958953273518,75.8105002291114,75.9194429915219,
76.0282218606248,76.1420667018968,76.250645200874,76.3591846308122,76.4677479638505,
76.4836012257127),.UNSPECIFIED.);
#827=B_SPLINE_CURVE_WITH_KNOTS('',3,(#76121,#76122,#76123,#76124,#76125,
#76126,#76127,#76128,#76129,#76130,#76131,#76132,#76133,#76134,#76135,#76136,
#76137,#76138,#76139,#76140,#76141,#76142,#76143,#76144,#76145,#76146,#76147,
#76148,#76149,#76150,#76151,#76152,#76153,#76154,#76155,#76156,#76157,#76158,
#76159,#76160,#76161,#76162,#76163,#76164,#76165,#76166,#76167,#76168,#76169,
#76170,#76171,#76172,#76173,#76174,#76175,#76176,#76177,#76178,#76179,#76180,
#76181,#76182,#76183,#76184,#76185,#76186,#76187,#76188,#76189,#76190,#76191,
#76192,#76193,#76194,#76195,#76196,#76197,#76198,#76199,#76200,#76201,#76202,
#76203,#76204,#76205,#76206,#76207,#76208,#76209,#76210,#76211,#76212,#76213,
#76214,#76215,#76216,#76217,#76218,#76219,#76220,#76221,#76222,#76223,#76224,
#76225,#76226,#76227,#76228,#76229,#76230,#76231,#76232,#76233,#76234,#76235,
#76236,#76237,#76238,#76239,#76240,#76241,#76242,#76243,#76244,#76245,#76246,
#76247,#76248,#76249,#76250,#76251,#76252,#76253,#76254,#76255,#76256,#76257,
#76258,#76259,#76260,#76261,#76262,#76263,#76264,#76265,#76266,#76267,#76268,
#76269,#76270,#76271,#76272,#76273,#76274,#76275,#76276,#76277,#76278,#76279,
#76280,#76281,#76282,#76283,#76284,#76285,#76286,#76287,#76288,#76289,#76290,
#76291,#76292),.UNSPECIFIED.,.F.,.F.,(4,3,3,3,3,3,3,3,3,3,3,3,3,3,3,3,3,
3,3,3,3,3,3,3,3,3,3,3,3,3,3,3,3,3,3,3,3,3,3,3,3,3,3,3,3,3,3,3,3,3,3,3,3,
3,3,3,3,4),(76.4836012261201,76.6112555507849,76.740372532373,76.8080068110734,
76.9171792497287,77.028221017642,77.1370931642971,77.2458987701923,77.3546778398902,
77.4673867281765,77.5763035895162,77.6909084912758,77.8055133930354,77.9146858316908,
78.0257275996041,78.1345997462592,78.2434053521544,78.3521844218525,78.4648933101387,
78.5738101714784,78.6884150732379,78.8030199749974,78.9121924136527,79.0232341815661,
79.1321063282212,79.2409119341164,79.3496910038144,79.4623998921006,79.5713167534403,
79.6859216551999,79.8005265569594,79.9096989956147,80.0207407635281,80.1296129101831,
80.2384185160783,80.3471975857763,80.4599064740625,80.5688233354022,80.6834282371618,
80.7980331389214,80.9072055775768,81.0182473454901,81.1271194921453,81.2359250980405,
81.3447041677386,81.4574130560248,81.5663299173645,81.680934819124,81.7955397208834,
81.9042355427827,82.0127410724368,82.1211403939236,82.2294743442541,82.3377836693491,
82.4461876480963,82.5546348576525,82.6632882530645,82.7667865324968),
 .UNSPECIFIED.);
#828=B_SPLINE_CURVE_WITH_KNOTS('',3,(#76294,#76295,#76296,#76297,#76298,
#76299,#76300,#76301,#76302,#76303,#76304,#76305,#76306,#76307,#76308,#76309,
#76310,#76311,#76312,#76313,#76314,#76315,#76316,#76317,#76318,#76319,#76320,
#76321,#76322,#76323,#76324,#76325,#76326,#76327,#76328,#76329,#76330,#76331,
#76332,#76333,#76334,#76335,#76336,#76337,#76338,#76339,#76340,#76341,#76342,
#76343,#76344,#76345,#76346,#76347,#76348,#76349,#76350,#76351,#76352,#76353,
#76354,#76355,#76356,#76357,#76358,#76359,#76360,#76361,#76362,#76363,#76364,
#76365,#76366,#76367,#76368,#76369,#76370,#76371,#76372,#76373,#76374,#76375,
#76376,#76377,#76378,#76379,#76380,#76381,#76382,#76383,#76384,#76385,#76386,
#76387,#76388,#76389,#76390,#76391,#76392,#76393,#76394,#76395,#76396,#76397,
#76398,#76399,#76400,#76401,#76402,#76403,#76404,#76405,#76406,#76407,#76408,
#76409,#76410,#76411,#76412,#76413,#76414,#76415,#76416,#76417,#76418,#76419,
#76420,#76421,#76422,#76423,#76424,#76425,#76426,#76427,#76428,#76429,#76430,
#76431,#76432,#76433,#76434,#76435,#76436,#76437,#76438,#76439,#76440,#76441,
#76442,#76443,#76444,#76445,#76446,#76447,#76448,#76449,#76450,#76451,#76452,
#76453,#76454,#76455,#76456,#76457,#76458,#76459,#76460,#76461,#76462,#76463,
#76464,#76465),.UNSPECIFIED.,.F.,.F.,(4,3,3,3,3,3,3,3,3,3,3,3,3,3,3,3,3,
3,3,3,3,3,3,3,3,3,3,3,3,3,3,3,3,3,3,3,3,3,3,3,3,3,3,3,3,3,3,3,3,3,3,3,3,
3,3,3,3,4),(82.7667865328923,82.7930463028454,82.9022187415008,83.0132605094141,
83.1221326560692,83.2309382619644,83.3397173316625,83.4524262199487,83.5613430812884,
83.6759479830479,83.7905528848074,83.8997253234628,84.0107670913761,84.1196392380312,
84.2284448439264,84.3372239136245,84.4499328019107,84.5588496632504,84.6734545650099,
84.7880594667694,84.8972319054247,85.0082736733381,85.1171458199932,85.2259514258884,
85.3347304955864,85.4474393838727,85.5563562452124,85.6709611469719,85.7855660487314,
85.8947384873868,86.0057802553001,86.1146524019552,86.2234580078504,86.3322370775484,
86.4449459658347,86.5538628271744,86.6684677289339,86.7830726306934,86.8922450693488,
87.0032868372621,87.1121589839172,87.2209645898124,87.3297436595103,87.4424525477966,
87.5513694091363,87.6659743108958,87.7805792126554,87.8897516513109,88.0007934192242,
88.1096655658794,88.2184711717746,88.3272502414726,88.4399591297588,88.5488759910986,
88.663480892858,88.7780857946174,88.9147451508073,89.0499718396522),
 .UNSPECIFIED.);
#829=B_SPLINE_CURVE_WITH_KNOTS('',3,(#76467,#76468,#76469,#76470,#76471,
#76472,#76473,#76474,#76475,#76476,#76477,#76478,#76479,#76480,#76481,#76482,
#76483,#76484,#76485,#76486,#76487,#76488,#76489,#76490,#76491,#76492,#76493,
#76494,#76495,#76496,#76497,#76498,#76499,#76500,#76501,#76502,#76503,#76504,
#76505,#76506,#76507,#76508,#76509,#76510,#76511,#76512,#76513,#76514,#76515,
#76516,#76517,#76518,#76519,#76520,#76521,#76522,#76523,#76524,#76525,#76526,
#76527,#76528,#76529,#76530,#76531,#76532,#76533,#76534,#76535,#76536,#76537,
#76538,#76539,#76540,#76541,#76542,#76543,#76544,#76545,#76546,#76547,#76548,
#76549,#76550,#76551,#76552,#76553,#76554,#76555,#76556,#76557,#76558,#76559,
#76560,#76561,#76562,#76563,#76564,#76565,#76566,#76567,#76568,#76569,#76570,
#76571,#76572,#76573,#76574,#76575,#76576,#76577,#76578,#76579,#76580,#76581,
#76582,#76583,#76584,#76585,#76586,#76587,#76588,#76589,#76590,#76591,#76592,
#76593,#76594,#76595,#76596,#76597,#76598,#76599,#76600,#76601,#76602,#76603,
#76604,#76605,#76606,#76607,#76608,#76609,#76610,#76611,#76612,#76613,#76614,
#76615,#76616,#76617,#76618,#76619,#76620,#76621,#76622,#76623,#76624,#76625,
#76626,#76627,#76628,#76629,#76630,#76631,#76632,#76633,#76634,#76635,#76636,
#76637,#76638),.UNSPECIFIED.,.F.,.F.,(4,3,3,3,3,3,3,3,3,3,3,3,3,3,3,3,3,
3,3,3,3,3,3,3,3,3,3,3,3,3,3,3,3,3,3,3,3,3,3,3,3,3,3,3,3,3,3,3,3,3,3,3,3,
3,3,3,3,4),(89.0499718400719,89.1578186100854,89.2656072096612,89.3733790748927,
89.4812520864616,89.5891766087315,89.6973011055592,89.7755923765794,89.8847648152346,
89.9958065831479,90.1046787298029,90.213484335698,90.3222634053958,90.4349722936822,
90.5438891550218,90.6584940567815,90.7730989585413,90.8822713971971,90.9933131651104,
91.1021853117659,91.2109909176616,91.3197699873602,91.432478875646,91.5413957369861,
91.6560006387447,91.7706055405033,91.8797779791581,91.9908197470715,92.0996918937262,
92.2084974996209,92.3172765693185,92.4299854576052,92.5389023189444,92.6535072207049,
92.7681121224653,92.8772845611197,92.9883263290332,93.0971984756875,93.2060040815818,
93.314783151279,93.4274920395661,93.5364089009049,93.6510138026661,93.7656187044273,
93.8747911430863,93.9858329109992,94.094705057658,94.2035106635569,94.3122897332586,
94.4249986215413,94.5339154828846,94.6485203846369,94.7631252863893,94.8748360662789,
94.989416336522,95.1007236987982,95.2169404230248,95.3331571472515),
 .UNSPECIFIED.);
#830=B_SPLINE_CURVE_WITH_KNOTS('',3,(#76640,#76641,#76642,#76643,#76644,
#76645,#76646,#76647,#76648,#76649,#76650,#76651,#76652,#76653,#76654,#76655,
#76656,#76657,#76658,#76659,#76660,#76661,#76662,#76663,#76664,#76665,#76666,
#76667,#76668,#76669,#76670,#76671,#76672,#76673,#76674,#76675,#76676,#76677,
#76678,#76679,#76680,#76681,#76682,#76683,#76684,#76685,#76686,#76687,#76688,
#76689,#76690,#76691,#76692,#76693,#76694,#76695,#76696,#76697,#76698,#76699,
#76700,#76701,#76702,#76703,#76704,#76705,#76706,#76707,#76708,#76709,#76710,
#76711,#76712,#76713,#76714,#76715,#76716,#76717,#76718,#76719,#76720,#76721,
#76722,#76723,#76724,#76725,#76726,#76727,#76728,#76729,#76730,#76731,#76732,
#76733,#76734,#76735,#76736,#76737,#76738,#76739,#76740,#76741,#76742,#76743,
#76744,#76745,#76746,#76747,#76748,#76749,#76750,#76751,#76752,#76753,#76754,
#76755,#76756,#76757,#76758,#76759,#76760,#76761,#76762,#76763,#76764,#76765,
#76766,#76767,#76768,#76769,#76770,#76771,#76772,#76773,#76774,#76775,#76776,
#76777,#76778,#76779,#76780,#76781,#76782,#76783,#76784,#76785,#76786,#76787,
#76788,#76789,#76790,#76791,#76792,#76793,#76794,#76795,#76796,#76797,#76798,
#76799,#76800,#76801,#76802,#76803,#76804,#76805,#76806,#76807,#76808,#76809,
#76810,#76811),.UNSPECIFIED.,.F.,.F.,(4,3,3,3,3,3,3,3,3,3,3,3,3,3,3,3,3,
3,3,3,3,3,3,3,3,3,3,3,3,3,3,3,3,3,3,3,3,3,3,3,3,3,3,3,3,3,3,3,3,3,3,3,3,
3,3,3,3,4),(95.3331571475866,95.4513555745942,95.5698952158399,95.6889447197994,
95.7606318683513,95.8698043070021,95.980846074916,96.0897182215664,96.1985238274569,
96.3073028971503,96.420011785441,96.5289286467759,96.6435335485446,96.7581384503133,
96.8673108889975,96.9783526569072,97.0872248035911,97.1960304095152,97.3048094792419,
97.4175183675002,97.526435228868,97.6410401305717,97.7556450322753,97.8648174708862,
97.9758592388051,98.0847313854162,98.1935369912679,98.3023160609226,98.4150249492513,
98.5239418105492,98.6385467123932,98.7531516142373,98.8623240528741,98.9733658207898,
99.082237967425,99.1910435732999,99.2998226429772,99.4125315312828,99.521448392601,
99.6360532944001,99.7506581961993,99.8598306350725,99.9708724029585,100.079744549832,
100.188550155946,100.297329225862,100.410038113937,100.51895497549,100.633559876826,
100.748164778161,100.856686987641,100.964128213411,101.071465293244,101.178740384828,
101.28814090212,101.39547392521,101.505908189604,101.616342453998),
 .UNSPECIFIED.);
#831=B_SPLINE_CURVE_WITH_KNOTS('',3,(#76813,#76814,#76815,#76816,#76817,
#76818,#76819,#76820,#76821,#76822,#76823,#76824,#76825,#76826,#76827,#76828,
#76829,#76830,#76831,#76832,#76833,#76834,#76835,#76836,#76837,#76838,#76839,
#76840,#76841,#76842,#76843,#76844,#76845,#76846,#76847,#76848,#76849,#76850,
#76851,#76852,#76853,#76854,#76855,#76856,#76857,#76858,#76859,#76860,#76861,
#76862,#76863,#76864,#76865,#76866,#76867,#76868,#76869,#76870,#76871,#76872,
#76873,#76874,#76875,#76876,#76877,#76878,#76879,#76880,#76881,#76882,#76883,
#76884,#76885,#76886,#76887,#76888,#76889,#76890,#76891,#76892,#76893,#76894,
#76895,#76896,#76897,#76898,#76899,#76900,#76901,#76902,#76903,#76904,#76905,
#76906,#76907,#76908,#76909,#76910,#76911,#76912,#76913,#76914,#76915,#76916,
#76917,#76918,#76919,#76920,#76921,#76922,#76923,#76924,#76925,#76926,#76927,
#76928,#76929,#76930,#76931,#76932,#76933,#76934,#76935,#76936,#76937,#76938,
#76939,#76940,#76941,#76942,#76943,#76944,#76945,#76946,#76947,#76948,#76949,
#76950,#76951,#76952,#76953,#76954,#76955,#76956,#76957,#76958,#76959,#76960,
#76961,#76962,#76963,#76964,#76965,#76966,#76967,#76968,#76969,#76970,#76971,
#76972,#76973,#76974,#76975,#76976,#76977,#76978,#76979,#76980,#76981),
 .UNSPECIFIED.,.F.,.F.,(4,3,3,3,3,3,3,3,3,3,3,3,3,3,3,3,3,3,3,3,3,3,3,3,
3,3,3,3,3,3,3,3,3,3,3,3,3,3,3,3,3,3,3,3,3,3,3,3,3,3,3,3,3,3,3,3,4),(101.616342454431,
101.745671360123,101.854843798772,101.965885566686,102.074757713323,102.183563319196,
102.292342388868,102.405051277172,102.513968138477,102.628573040281,102.743177942085,
102.852350382351,102.963392150063,103.072264298338,103.181069905853,103.289848977168,
103.402557863888,103.511474726817,103.626079625432,103.740684524047,103.849856959235,
103.960898727582,104.069770870792,104.178576473261,104.287355539555,104.400064431169,
104.508981289201,104.623586197605,104.738191106009,104.847363545745,104.958405313523,
105.067277461168,105.176083068018,105.284862138634,105.397571025968,105.506487888124,
105.621092788048,105.735697687971,105.844870138156,105.955911904628,106.064784062917,
106.173589680453,106.282368761779,106.395077638818,106.50399451162,106.618599390777,
106.733204269933,106.842376679246,106.953418450827,107.062290568273,107.171096145088,
107.279875185881,107.392584102385,107.501500935583,107.616105893739,107.730710851895,
107.899527761611),.UNSPECIFIED.);
#832=B_SPLINE_CURVE_WITH_KNOTS('',3,(#76983,#76984,#76985,#76986,#76987,
#76988,#76989,#76990,#76991,#76992,#76993,#76994,#76995,#76996,#76997,#76998,
#76999,#77000,#77001,#77002,#77003,#77004,#77005,#77006,#77007,#77008,#77009,
#77010,#77011,#77012,#77013,#77014,#77015,#77016,#77017,#77018,#77019,#77020,
#77021,#77022,#77023,#77024,#77025,#77026,#77027,#77028,#77029,#77030,#77031,
#77032,#77033,#77034,#77035,#77036,#77037,#77038,#77039,#77040,#77041,#77042,
#77043,#77044,#77045,#77046,#77047,#77048,#77049,#77050,#77051,#77052,#77053,
#77054,#77055,#77056,#77057,#77058,#77059,#77060,#77061,#77062,#77063,#77064,
#77065,#77066,#77067,#77068,#77069,#77070,#77071,#77072,#77073,#77074,#77075,
#77076,#77077,#77078,#77079,#77080,#77081,#77082,#77083,#77084,#77085,#77086,
#77087,#77088,#77089,#77090,#77091,#77092,#77093,#77094,#77095,#77096,#77097,
#77098,#77099,#77100,#77101,#77102,#77103,#77104,#77105,#77106,#77107,#77108,
#77109,#77110,#77111,#77112,#77113,#77114,#77115,#77116,#77117,#77118,#77119,
#77120,#77121,#77122,#77123,#77124,#77125,#77126,#77127,#77128,#77129,#77130,
#77131,#77132,#77133,#77134,#77135,#77136,#77137,#77138,#77139,#77140,#77141,
#77142,#77143,#77144,#77145,#77146,#77147,#77148,#77149,#77150,#77151,#77152,
#77153,#77154),.UNSPECIFIED.,.F.,.F.,(4,3,3,3,3,3,3,3,3,3,3,3,3,3,3,3,3,
3,3,3,3,3,3,3,3,3,3,3,3,3,3,3,3,3,3,3,3,3,3,3,3,3,3,3,3,3,3,3,3,3,3,3,3,
3,3,3,3,4),(107.899527761921,108.006900864593,108.114166062461,108.221365614772,
108.328541675354,108.435810646325,108.543126437004,108.650636673681,108.728217433857,
108.837389951873,108.948431709866,109.05730393688,109.166109623282,109.274888773503,
109.387597584082,109.49651452505,109.611119270435,109.725724015819,109.834896212092,
109.945938010303,110.054809915234,110.16361528031,110.272394110473,110.3851032323,
110.494019860034,110.608625228907,110.723230597781,110.83240324485,110.943444986712,
111.052317336357,111.161123142689,111.269902409969,111.382611102413,111.491528152047,
111.606132665895,111.720737179743,111.82991013605,111.940951839257,112.049824512698,
112.158630647303,112.267410246761,112.380118625497,112.489036013027,112.603639887366,
112.718243761705,112.827414243178,112.938456255739,113.047326447098,113.156130103738,
113.264907233319,113.377618010906,113.486532977032,113.60114166035,113.715750343667,
113.832491024865,113.948637158773,114.065675113617,114.182713068461),
 .UNSPECIFIED.);
#833=B_SPLINE_CURVE_WITH_KNOTS('',3,(#77156,#77157,#77158,#77159,#77160,
#77161,#77162,#77163,#77164,#77165,#77166,#77167,#77168,#77169,#77170,#77171,
#77172,#77173,#77174,#77175,#77176,#77177,#77178,#77179,#77180,#77181,#77182,
#77183,#77184,#77185,#77186,#77187,#77188,#77189,#77190,#77191,#77192,#77193,
#77194,#77195,#77196,#77197,#77198,#77199,#77200,#77201,#77202,#77203,#77204,
#77205,#77206,#77207,#77208,#77209,#77210,#77211,#77212,#77213,#77214,#77215,
#77216,#77217,#77218,#77219,#77220,#77221,#77222,#77223,#77224,#77225,#77226,
#77227,#77228,#77229,#77230,#77231,#77232,#77233,#77234,#77235,#77236,#77237,
#77238,#77239,#77240,#77241,#77242,#77243,#77244,#77245,#77246,#77247,#77248,
#77249,#77250,#77251,#77252,#77253,#77254,#77255,#77256,#77257,#77258,#77259,
#77260,#77261,#77262,#77263,#77264,#77265,#77266,#77267,#77268,#77269,#77270,
#77271,#77272,#77273,#77274,#77275,#77276,#77277,#77278,#77279,#77280,#77281,
#77282,#77283,#77284,#77285,#77286,#77287,#77288,#77289,#77290,#77291,#77292,
#77293,#77294,#77295,#77296,#77297,#77298,#77299,#77300,#77301,#77302,#77303,
#77304,#77305,#77306,#77307,#77308,#77309,#77310,#77311,#77312,#77313,#77314,
#77315,#77316,#77317,#77318,#77319,#77320,#77321,#77322,#77323,#77324,#77325,
#77326,#77327,#77328,#77329,#77330),.UNSPECIFIED.,.F.,.F.,(4,3,3,3,3,3,
3,3,3,3,3,3,3,3,3,3,3,3,3,3,3,3,3,3,3,3,3,3,3,3,3,3,3,3,3,3,3,3,3,3,3,3,
3,3,3,3,3,3,3,3,3,3,3,3,3,3,3,3,4),(114.18271306879,114.295259121202,114.40805768734,
114.520987722838,114.634207955653,114.713256925629,114.822432474766,114.933473853869,
115.042349191685,115.151158009723,115.259940307156,115.372646107264,115.481566197116,
115.596164852353,115.710763507591,115.819920495038,115.930964194352,116.039820877543,
116.148611057667,116.257374763845,116.370098595272,116.479000423707,116.59363525663,
116.708270089553,116.817463632358,116.928502762252,117.037395716857,117.14622196453,
117.255021477854,117.367710276269,117.476646858088,117.591211764801,117.705776671515,
117.814965193221,117.926004950753,118.03489387316,118.143716463952,118.252512698232,
118.365205337043,118.47413960404,118.588711428758,118.703283253477,118.8123366592,
118.92339330623,119.032146115717,119.140832593708,119.249492932242,119.362317158041,
119.471117626952,119.579996228259,119.689057881339,119.700789835439,119.808769052271,
119.916596187234,120.024313170425,120.134709471811,120.242364817779,120.354131596875,
120.46589837597),.UNSPECIFIED.);
#834=B_SPLINE_CURVE_WITH_KNOTS('',3,(#77332,#77333,#77334,#77335,#77336,
#77337,#77338,#77339,#77340,#77341,#77342,#77343,#77344,#77345,#77346,#77347,
#77348,#77349,#77350,#77351,#77352,#77353,#77354,#77355,#77356,#77357,#77358,
#77359,#77360,#77361,#77362,#77363,#77364,#77365,#77366,#77367,#77368),
 .UNSPECIFIED.,.F.,.F.,(4,3,3,3,3,3,3,3,3,3,3,3,4),(120.465898376338,120.611331523754,
120.698296417401,120.80753478414,120.918568311043,121.027511991089,121.136390994414,
121.245245185674,121.357884639096,121.466879955347,121.581341477355,121.695802999363,
121.705794139069),.UNSPECIFIED.);
#835=B_SPLINE_CURVE_WITH_KNOTS('',3,(#77372,#77373,#77374,#77375,#77376,
#77377,#77378),.UNSPECIFIED.,.F.,.F.,(4,3,4),(-123.690816163287,-123.552129947919,
-123.421758301599),.UNSPECIFIED.);
#836=B_SPLINE_CURVE_WITH_KNOTS('',3,(#77380,#77381,#77382,#77383,#77384,
#77385,#77386,#77387,#77388,#77389),.UNSPECIFIED.,.F.,.F.,(4,1,1,1,1,1,
1,4),(-123.421757974662,-122.693309581325,-121.695802999363,-120.698296417401,
-119.700789835439,-118.703283253477,-117.705776671515,-117.138572667483),
 .UNSPECIFIED.);
#837=B_SPLINE_CURVE_WITH_KNOTS('',3,(#77391,#77392,#77393,#77394,#77395,
#77396,#77397,#77398,#77399,#77400,#77401,#77402,#77403,#77404,#77405,#77406,
#77407,#77408,#77409,#77410,#77411,#77412,#77413,#77414,#77415,#77416,#77417,
#77418,#77419,#77420,#77421,#77422,#77423,#77424,#77425,#77426,#77427,#77428,
#77429,#77430,#77431,#77432,#77433,#77434,#77435,#77436,#77437,#77438,#77439,
#77440,#77441,#77442,#77443,#77444,#77445,#77446,#77447,#77448,#77449,#77450,
#77451,#77452,#77453,#77454,#77455,#77456,#77457,#77458,#77459,#77460,#77461,
#77462,#77463,#77464,#77465,#77466,#77467,#77468,#77469,#77470,#77471,#77472,
#77473,#77474,#77475,#77476,#77477,#77478,#77479,#77480,#77481,#77482,#77483,
#77484,#77485,#77486,#77487,#77488,#77489,#77490,#77491,#77492,#77493,#77494,
#77495,#77496,#77497,#77498,#77499,#77500,#77501,#77502,#77503,#77504,#77505,
#77506,#77507,#77508,#77509,#77510,#77511,#77512,#77513,#77514,#77515,#77516,
#77517,#77518,#77519,#77520,#77521,#77522,#77523,#77524,#77525,#77526,#77527,
#77528,#77529,#77530,#77531,#77532,#77533,#77534,#77535,#77536,#77537,#77538,
#77539,#77540,#77541,#77542,#77543,#77544,#77545,#77546,#77547,#77548,#77549,
#77550,#77551,#77552,#77553,#77554,#77555,#77556,#77557,#77558,#77559,#77560,
#77561,#77562),.UNSPECIFIED.,.F.,.F.,(4,3,3,3,3,3,3,3,3,3,3,3,3,3,3,3,3,
3,3,3,3,3,3,3,3,3,3,3,3,3,3,3,3,3,3,3,3,3,3,3,3,3,3,3,3,3,3,3,3,3,3,3,3,
3,3,3,3,4),(-117.138572329772,-117.020515175888,-116.902124778381,-116.783229707864,
-116.708270089553,-116.599112217178,-116.488068628479,-116.379211566519,
-116.270421196485,-116.161657488991,-116.048933993641,-115.940032632066,
-115.825398069829,-115.710763507591,-115.601587885419,-115.490546515445,
-115.381671151657,-115.272862325182,-115.164080036811,-115.051374259016,
-114.942454221547,-114.827855573588,-114.713256925629,-114.604082572887,
-114.493041044235,-114.384166871964,-114.27535920449,-114.166578040568,
-114.053871116343,-113.944952103319,-113.830351223493,-113.715750343667,
-113.606579738047,-113.495537741004,-113.386667496225,-113.277863812558,
-113.169086682307,-113.056375952157,-112.947461050788,-112.832852406246,
-112.718243761705,-112.609070807295,-112.498029103851,-112.389156431964,
-112.280350298782,-112.171570700614,-112.058862320396,-111.94994493381,
-111.835341056776,-111.720737179743,-111.612568452366,-111.505138681501,
-111.397813214992,-111.290549882046,-111.181759251717,-111.074439119888,
-110.964913240309,-110.85538736073),.UNSPECIFIED.);
#838=B_SPLINE_CURVE_WITH_KNOTS('',3,(#77564,#77565,#77566,#77567,#77568,
#77569,#77570,#77571,#77572,#77573,#77574,#77575,#77576,#77577,#77578,#77579,
#77580,#77581,#77582,#77583,#77584,#77585,#77586,#77587,#77588,#77589,#77590,
#77591,#77592,#77593,#77594,#77595,#77596,#77597,#77598,#77599,#77600,#77601,
#77602,#77603,#77604,#77605,#77606,#77607,#77608,#77609,#77610,#77611,#77612,
#77613,#77614,#77615,#77616,#77617,#77618,#77619,#77620,#77621,#77622,#77623,
#77624,#77625,#77626,#77627,#77628,#77629,#77630,#77631,#77632,#77633,#77634,
#77635,#77636,#77637,#77638,#77639,#77640,#77641,#77642,#77643,#77644,#77645,
#77646,#77647,#77648,#77649,#77650,#77651,#77652,#77653,#77654,#77655,#77656,
#77657,#77658,#77659,#77660,#77661,#77662,#77663,#77664,#77665,#77666,#77667,
#77668,#77669,#77670,#77671,#77672,#77673,#77674,#77675,#77676,#77677,#77678,
#77679,#77680,#77681,#77682,#77683,#77684,#77685,#77686,#77687,#77688,#77689,
#77690,#77691,#77692,#77693,#77694,#77695,#77696,#77697,#77698,#77699,#77700,
#77701,#77702,#77703,#77704,#77705,#77706,#77707,#77708,#77709,#77710,#77711,
#77712,#77713,#77714,#77715,#77716,#77717,#77718,#77719,#77720,#77721,#77722,
#77723,#77724,#77725,#77726,#77727,#77728,#77729,#77730,#77731,#77732),
 .UNSPECIFIED.,.F.,.F.,(4,3,3,3,3,3,3,3,3,3,3,3,3,3,3,3,3,3,3,3,3,3,3,3,
3,3,3,3,3,3,3,3,3,3,3,3,3,3,3,3,3,3,3,3,3,3,3,3,3,3,3,3,3,3,3,3,4),(-110.855387360303,
-110.723230597781,-110.614058384659,-110.503016588554,-110.394144676341,
-110.285339307555,-110.176560477246,-110.06385136189,-109.954934742862,
-109.84032937934,-109.725724015819,-109.616551499424,-109.505509741228,
-109.396637515017,-109.287831829112,-109.179052679082,-109.066343867775,
-108.957426926237,-108.842822180047,-108.728217433857,-108.619044981008,
-108.508003214869,-108.399131052779,-108.29032543103,-108.181546345082,
-108.068837471785,-107.959920593393,-107.845315722644,-107.730710851895,
-107.621538440357,-107.510496669054,-107.401624550643,-107.292818973334,
-107.184039932516,-107.07133101687,-106.962414184812,-106.847809227373,
-106.733204269933,-106.62403182012,-106.512990053601,-106.404117895488,
-106.295312278054,-106.186533196756,-106.07382431956,-105.964907446603,
-105.850302567287,-105.735697687971,-105.626525248591,-105.515483480768,
-105.40661133327,-105.297805726489,-105.189026655866,-105.076317768402,
-104.967400906045,-104.852796006027,-104.738191106009,-104.572202053123),
 .UNSPECIFIED.);
#839=B_SPLINE_CURVE_WITH_KNOTS('',3,(#77734,#77735,#77736,#77737,#77738,
#77739,#77740,#77741,#77742,#77743,#77744,#77745,#77746,#77747,#77748,#77749,
#77750,#77751,#77752,#77753,#77754,#77755,#77756,#77757,#77758,#77759,#77760,
#77761,#77762,#77763,#77764,#77765,#77766,#77767,#77768,#77769,#77770,#77771,
#77772,#77773,#77774,#77775,#77776,#77777,#77778,#77779,#77780,#77781,#77782,
#77783,#77784,#77785,#77786,#77787,#77788,#77789,#77790,#77791,#77792,#77793,
#77794,#77795,#77796,#77797,#77798,#77799,#77800,#77801,#77802,#77803,#77804,
#77805,#77806,#77807,#77808,#77809,#77810,#77811,#77812,#77813,#77814,#77815,
#77816,#77817,#77818,#77819,#77820,#77821,#77822,#77823,#77824,#77825,#77826,
#77827,#77828,#77829,#77830,#77831,#77832,#77833,#77834,#77835,#77836,#77837,
#77838,#77839,#77840,#77841,#77842,#77843,#77844,#77845,#77846,#77847,#77848,
#77849,#77850,#77851,#77852,#77853,#77854,#77855,#77856,#77857,#77858,#77859,
#77860,#77861,#77862,#77863,#77864,#77865,#77866,#77867,#77868,#77869,#77870,
#77871,#77872,#77873,#77874,#77875,#77876,#77877,#77878,#77879,#77880,#77881,
#77882,#77883,#77884,#77885,#77886,#77887,#77888,#77889,#77890,#77891,#77892,
#77893,#77894,#77895,#77896,#77897,#77898,#77899,#77900,#77901,#77902,#77903,
#77904,#77905),.UNSPECIFIED.,.F.,.F.,(4,3,3,3,3,3,3,3,3,3,3,3,3,3,3,3,3,
3,3,3,3,3,3,3,3,3,3,3,3,3,3,3,3,3,3,3,3,3,3,3,3,3,3,3,3,3,3,3,3,3,3,3,3,
3,3,3,3,4),(-104.572202052802,-104.464825203815,-104.357557368283,-104.250356283725,
-104.143179794702,-104.035911189414,-103.928596755901,-103.821086998969,
-103.740684524047,-103.631512083848,-103.520470316128,-103.411598167883,
-103.302792560386,-103.194013489076,-103.081304602328,-102.97238773937,
-102.857782840727,-102.743177942085,-102.634005503472,-102.522963735553,
-102.41409158893,-102.305285983064,-102.19650691339,-102.083798025074,-101.974881163749,
-101.860276261936,-101.745671360123,-101.63649892183,-101.525457153872,
-101.416585007596,-101.307779402086,-101.199000332777,-101.086291444123,
-100.97737458318,-100.86276968067,-100.748164778161,-100.638992339298,-100.527950571411,
-100.419078424542,-100.310272818431,-100.201493748516,-100.088784860437,
-99.9798679988786,-99.865263097539,-99.7506581961993,-99.6414857575659,
-99.5304439896498,-99.4215718430159,-99.3127662371415,-99.2039871674642,
-99.0912782791575,-98.9823614178373,-98.8677565160373,-98.7531516142373,
-98.6365755860952,-98.52026925052,-98.4043629935902,-98.2890167463),
 .UNSPECIFIED.);
#840=B_SPLINE_CURVE_WITH_KNOTS('',3,(#77907,#77908,#77909,#77910,#77911,
#77912,#77913,#77914,#77915,#77916,#77917,#77918,#77919,#77920,#77921,#77922,
#77923,#77924,#77925,#77926,#77927,#77928,#77929,#77930,#77931,#77932,#77933,
#77934,#77935,#77936,#77937,#77938,#77939,#77940,#77941,#77942,#77943,#77944,
#77945,#77946,#77947,#77948,#77949,#77950,#77951,#77952,#77953,#77954,#77955,
#77956,#77957,#77958,#77959,#77960,#77961,#77962,#77963,#77964,#77965,#77966,
#77967,#77968,#77969,#77970,#77971,#77972,#77973,#77974,#77975,#77976,#77977,
#77978,#77979,#77980,#77981,#77982,#77983,#77984,#77985,#77986,#77987,#77988,
#77989,#77990,#77991,#77992,#77993,#77994,#77995,#77996,#77997,#77998,#77999,
#78000,#78001,#78002,#78003,#78004,#78005,#78006,#78007,#78008,#78009,#78010,
#78011,#78012,#78013,#78014,#78015,#78016,#78017,#78018,#78019,#78020,#78021,
#78022,#78023,#78024,#78025,#78026,#78027,#78028,#78029,#78030,#78031,#78032,
#78033,#78034,#78035,#78036,#78037,#78038,#78039,#78040,#78041,#78042,#78043,
#78044,#78045,#78046,#78047,#78048,#78049,#78050,#78051,#78052,#78053,#78054,
#78055,#78056,#78057,#78058,#78059,#78060,#78061,#78062,#78063,#78064,#78065,
#78066,#78067,#78068,#78069,#78070,#78071,#78072,#78073,#78074,#78075,#78076,
#78077,#78078),.UNSPECIFIED.,.F.,.F.,(4,3,3,3,3,3,3,3,3,3,3,3,3,3,3,3,3,
3,3,3,3,3,3,3,3,3,3,3,3,3,3,3,3,3,3,3,3,3,3,3,3,3,3,3,3,3,3,3,3,3,3,3,3,
3,3,3,3,4),(-98.2890167459438,-98.1765832750562,-98.0639026838957,-97.9510940965738,
-97.8379965452098,-97.7556450322753,-97.6464725935929,-97.535430825683,
-97.4265586789999,-97.3177530730765,-97.20897400335,-97.0962651150908,-96.9873482537224,
-96.8727433520178,-96.7581384503133,-96.6489660116626,-96.5379242437487,
-96.4290520970982,-96.3202464912076,-96.2114674215143,-96.0987585332235,
-95.9898416718884,-95.8752367701198,-95.7606318683513,-95.6514594297002,
-95.5404176617863,-95.4315455151358,-95.3227399092451,-95.2139608395516,
-95.101251951261,-94.9923350899261,-94.8777301881577,-94.7631252863893,
-94.6539528477305,-94.5429110798176,-94.434038933159,-94.3252333272602,
-94.2164542575586,-94.1037453692758,-93.9948285079324,-93.8802236061799,
-93.7656187044273,-93.6564462657728,-93.5454044978594,-93.4365323512051,
-93.3277267453107,-93.2189476756135,-93.1062387873264,-92.9973219259875,
-92.8827170242264,-92.7681121224653,-92.660350082923,-92.5527396333652,
-92.4452386139182,-92.3353868201298,-92.2279447729249,-92.1168881058446,
-92.0058314387643),.UNSPECIFIED.);
#841=B_SPLINE_CURVE_WITH_KNOTS('',3,(#78080,#78081,#78082,#78083,#78084,
#78085,#78086,#78087,#78088,#78089,#78090,#78091,#78092,#78093,#78094,#78095,
#78096,#78097,#78098,#78099,#78100,#78101,#78102,#78103,#78104,#78105,#78106,
#78107,#78108,#78109,#78110,#78111,#78112,#78113,#78114,#78115,#78116,#78117,
#78118,#78119,#78120,#78121,#78122,#78123,#78124,#78125,#78126,#78127,#78128,
#78129,#78130,#78131,#78132,#78133,#78134,#78135,#78136,#78137,#78138,#78139,
#78140,#78141,#78142,#78143,#78144,#78145,#78146,#78147,#78148,#78149,#78150,
#78151,#78152,#78153,#78154,#78155,#78156,#78157,#78158,#78159,#78160,#78161,
#78162,#78163,#78164,#78165,#78166,#78167,#78168,#78169,#78170,#78171,#78172,
#78173,#78174,#78175,#78176,#78177,#78178,#78179,#78180,#78181,#78182,#78183,
#78184,#78185,#78186,#78187,#78188,#78189,#78190,#78191,#78192,#78193,#78194,
#78195,#78196,#78197,#78198,#78199,#78200,#78201,#78202,#78203,#78204,#78205,
#78206,#78207,#78208,#78209,#78210,#78211,#78212,#78213,#78214,#78215,#78216,
#78217,#78218,#78219,#78220,#78221,#78222,#78223,#78224,#78225,#78226,#78227,
#78228,#78229,#78230,#78231,#78232,#78233,#78234,#78235,#78236,#78237,#78238,
#78239,#78240,#78241,#78242,#78243,#78244,#78245,#78246,#78247,#78248,#78249,
#78250,#78251),.UNSPECIFIED.,.F.,.F.,(4,3,3,3,3,3,3,3,3,3,3,3,3,3,3,3,3,
3,3,3,3,3,3,3,3,3,3,3,3,3,3,3,3,3,3,3,3,3,3,3,3,3,3,3,3,3,3,3,3,3,3,3,3,
3,3,3,3,4),(-92.0058314383864,-91.8610046365001,-91.7706055405034,-91.6614331018477,
-91.5503913339344,-91.441519187279,-91.3327135813835,-91.2239345116852,
-91.1112256233992,-91.0023087620593,-90.8877038603003,-90.7730989585413,
-90.6639265198859,-90.5528847519726,-90.4440126053175,-90.3352069994222,
-90.2264279297242,-90.1137190414379,-90.0048021800982,-89.8901972783387,
-89.7755923765793,-89.666419937924,-89.5553781700107,-89.4465060233557,
-89.3377004174606,-89.2289213477627,-89.1162124594764,-89.0072955981368,
-88.8926906963771,-88.7780857946174,-88.668913355962,-88.5578715880487,
-88.4489994413936,-88.3401938354983,-88.2314147658003,-88.1187058775141,
-88.0097890161743,-87.8951841144149,-87.7805792126554,-87.671406774,-87.5603650060866,
-87.4514928594315,-87.3426872535362,-87.2339081838382,-87.121199295552,
-87.0122824342123,-86.8976775324528,-86.7830726306934,-86.673900192038,
-86.5628584241247,-86.4539862774696,-86.3451806715744,-86.2364016018764,
-86.1236927135901,-86.0147758522505,-85.9001709504909,-85.7855660487314,
-85.7226461315846),.UNSPECIFIED.);
#842=B_SPLINE_CURVE_WITH_KNOTS('',3,(#78253,#78254,#78255,#78256,#78257,
#78258,#78259,#78260,#78261,#78262,#78263,#78264,#78265,#78266,#78267,#78268,
#78269,#78270,#78271,#78272,#78273,#78274,#78275,#78276,#78277,#78278,#78279,
#78280,#78281,#78282,#78283,#78284,#78285,#78286,#78287,#78288,#78289,#78290,
#78291,#78292,#78293,#78294,#78295,#78296,#78297,#78298,#78299,#78300,#78301,
#78302,#78303,#78304,#78305,#78306,#78307,#78308,#78309,#78310,#78311,#78312,
#78313,#78314,#78315,#78316,#78317,#78318,#78319,#78320,#78321,#78322,#78323,
#78324,#78325,#78326,#78327,#78328,#78329,#78330,#78331,#78332,#78333,#78334,
#78335,#78336,#78337,#78338,#78339,#78340,#78341,#78342,#78343,#78344,#78345,
#78346,#78347,#78348,#78349,#78350,#78351,#78352,#78353,#78354,#78355,#78356,
#78357,#78358,#78359,#78360,#78361,#78362,#78363,#78364,#78365,#78366,#78367,
#78368,#78369,#78370,#78371,#78372,#78373,#78374,#78375,#78376,#78377,#78378,
#78379,#78380,#78381,#78382,#78383,#78384,#78385,#78386,#78387,#78388,#78389,
#78390,#78391,#78392,#78393,#78394,#78395,#78396,#78397,#78398,#78399,#78400,
#78401,#78402,#78403,#78404,#78405,#78406,#78407,#78408,#78409,#78410,#78411,
#78412,#78413,#78414,#78415,#78416,#78417,#78418,#78419,#78420,#78421,#78422,
#78423,#78424),.UNSPECIFIED.,.F.,.F.,(4,3,3,3,3,3,3,3,3,3,3,3,3,3,3,3,3,
3,3,3,3,3,3,3,3,3,3,3,3,3,3,3,3,3,3,3,3,3,3,3,3,3,3,3,3,3,3,3,3,3,3,3,3,
3,3,3,3,4),(-85.72264613121,-85.6145003567967,-85.5065334315114,-85.3986650150454,
-85.2908535890857,-85.1830577204263,-85.0751612384323,-84.9672121288341,
-84.8590675344965,-84.7880594667694,-84.6788870281141,-84.5678452602007,
-84.4589731135457,-84.3501675076505,-84.2413884379525,-84.1286795496662,
-84.0197626883265,-83.9051577865669,-83.7905528848074,-83.681380446152,
-83.5703386782387,-83.4614665315836,-83.3526609256883,-83.2438818559903,
-83.1311729677041,-83.0222561063644,-82.9076512046049,-82.7930463028454,
-82.6838738641901,-82.5728320962768,-82.4639599496218,-82.3551543437266,
-82.2463752740285,-82.1336663857422,-82.0247495244026,-81.910144622643,
-81.7955397208834,-81.686367282228,-81.5753255143147,-81.4664533676596,
-81.3576477617644,-81.2488686920663,-81.1361598037801,-81.0272429424404,
-80.9126380406809,-80.7980331389214,-80.6888607002659,-80.5778189323526,
-80.4689467856975,-80.3601411798021,-80.2513621101042,-80.138653221818,
-80.0297363604782,-79.9151314587188,-79.8005265569594,-79.6756486279101,
-79.5517871056718,-79.4394608248622),.UNSPECIFIED.);
#843=B_SPLINE_CURVE_WITH_KNOTS('',3,(#78426,#78427,#78428,#78429,#78430,
#78431,#78432,#78433,#78434,#78435,#78436,#78437,#78438,#78439,#78440,#78441,
#78442,#78443,#78444,#78445,#78446,#78447,#78448,#78449,#78450,#78451,#78452,
#78453,#78454,#78455,#78456,#78457,#78458,#78459,#78460,#78461,#78462,#78463,
#78464,#78465,#78466,#78467,#78468,#78469,#78470,#78471,#78472,#78473,#78474,
#78475,#78476,#78477,#78478,#78479,#78480,#78481,#78482,#78483,#78484,#78485,
#78486,#78487,#78488,#78489,#78490,#78491,#78492,#78493,#78494,#78495,#78496,
#78497,#78498,#78499,#78500,#78501,#78502,#78503,#78504,#78505,#78506,#78507,
#78508,#78509,#78510,#78511,#78512,#78513,#78514,#78515,#78516,#78517,#78518,
#78519,#78520,#78521,#78522,#78523,#78524,#78525,#78526,#78527,#78528,#78529,
#78530,#78531,#78532,#78533,#78534,#78535,#78536,#78537,#78538,#78539,#78540,
#78541,#78542,#78543,#78544,#78545,#78546,#78547,#78548,#78549,#78550,#78551,
#78552,#78553,#78554,#78555,#78556,#78557,#78558,#78559,#78560,#78561,#78562,
#78563,#78564,#78565,#78566,#78567,#78568,#78569,#78570,#78571,#78572,#78573,
#78574,#78575,#78576,#78577,#78578,#78579,#78580,#78581,#78582,#78583,#78584,
#78585,#78586,#78587,#78588,#78589,#78590,#78591,#78592,#78593,#78594,#78595,
#78596,#78597),.UNSPECIFIED.,.F.,.F.,(4,3,3,3,3,3,3,3,3,3,3,3,3,3,3,3,3,
3,3,3,3,3,3,3,3,3,3,3,3,3,3,3,3,3,3,3,3,3,3,3,3,3,3,3,3,3,3,3,3,3,3,3,3,
3,3,3,3,4),(-79.4394608244051,-79.3301673042638,-79.2208686887329,-79.1114399455883,
-79.0019456137403,-78.8922276554658,-78.8030199749974,-78.6938475363419,
-78.5828057684286,-78.4739336217734,-78.3651280158782,-78.2563489461802,
-78.143640057894,-78.0347231965542,-77.9201182947948,-77.8055133930354,
-77.6963409543801,-77.5852991864668,-77.4764270398118,-77.3676214339166,
-77.2588423642185,-77.1461334759323,-77.0372166145927,-76.9226117128331,
-76.8080068110735,-76.6988343724183,-76.5877926045049,-76.4789204578498,
-76.3701148519545,-76.2613357822566,-76.1486268939703,-76.0397100326307,
-75.9251051308711,-75.8105002291115,-75.7013277904561,-75.5902860225428,
-75.4814138758876,-75.3726082699924,-75.2638292002946,-75.1511203120083,
-75.0422034506686,-74.9275985489091,-74.8129936471495,-74.7038212084941,
-74.5927794405808,-74.4839072939257,-74.3751016880306,-74.2663226183327,
-74.1536137300464,-74.0446968687067,-73.9300919669471,-73.8154870651875,
-73.7062663965449,-73.5972126760366,-73.4869783863338,-73.3781347024253,
-73.2672051098253,-73.1562755172254),.UNSPECIFIED.);
#844=B_SPLINE_CURVE_WITH_KNOTS('',3,(#78599,#78600,#78601,#78602,#78603,
#78604,#78605,#78606,#78607,#78608,#78609,#78610,#78611,#78612,#78613,#78614,
#78615,#78616,#78617,#78618,#78619,#78620,#78621,#78622,#78623,#78624,#78625,
#78626,#78627,#78628,#78629,#78630,#78631,#78632,#78633,#78634,#78635,#78636,
#78637,#78638,#78639,#78640,#78641,#78642,#78643,#78644,#78645,#78646,#78647,
#78648,#78649,#78650,#78651,#78652,#78653,#78654,#78655,#78656,#78657,#78658,
#78659,#78660,#78661,#78662,#78663,#78664,#78665,#78666,#78667,#78668,#78669,
#78670,#78671,#78672,#78673,#78674,#78675,#78676,#78677,#78678,#78679,#78680,
#78681,#78682,#78683,#78684,#78685,#78686,#78687,#78688,#78689,#78690,#78691,
#78692,#78693,#78694,#78695,#78696,#78697,#78698,#78699,#78700,#78701,#78702,
#78703,#78704,#78705,#78706,#78707,#78708,#78709,#78710,#78711,#78712,#78713,
#78714,#78715,#78716,#78717,#78718,#78719,#78720,#78721,#78722,#78723,#78724,
#78725,#78726,#78727,#78728,#78729,#78730,#78731,#78732,#78733,#78734,#78735,
#78736,#78737,#78738,#78739,#78740,#78741,#78742,#78743,#78744,#78745,#78746,
#78747,#78748,#78749,#78750,#78751,#78752,#78753,#78754,#78755,#78756,#78757,
#78758,#78759,#78760,#78761,#78762,#78763,#78764,#78765,#78766,#78767,#78768,
#78769,#78770),.UNSPECIFIED.,.F.,.F.,(4,3,3,3,3,3,3,3,3,3,3,3,3,3,3,3,3,
3,3,3,3,3,3,3,3,3,3,3,3,3,3,3,3,3,3,3,3,3,3,3,3,3,3,3,3,3,3,3,3,3,3,3,3,
3,3,3,3,4),(-73.1562755167914,-73.0302440560829,-72.9029247194667,-72.8179804832255,
-72.70880804457,-72.5977662766567,-72.4888941300014,-72.380088524106,-72.2713094544078,
-72.1586005661217,-72.0496837047819,-71.9350788030227,-71.8204739012635,
-71.7113014626082,-71.6002596946948,-71.4913875480398,-71.3825819421446,
-71.2738028724466,-71.1610939841603,-71.0521771228207,-70.9375722210611,
-70.8229673193015,-70.7137948806462,-70.6027531127328,-70.4938809660778,
-70.3850753601826,-70.2762962904846,-70.1635874021983,-70.0546705408586,
-69.9400656390991,-69.8254607373395,-69.7162882986841,-69.6052465307708,
-69.4963743841157,-69.3875687782204,-69.2787897085223,-69.1660808202361,
-69.0571639588964,-68.9425590571369,-68.8279541553775,-68.7187817167221,
-68.6077399488088,-68.4988678021537,-68.3900621962585,-68.2812831265604,
-68.1685742382742,-68.0596573769345,-67.945052475175,-67.8304475734155,
-67.7219687232105,-67.6136797702115,-67.5054965122317,-67.3973778082143,
-67.2892826089374,-67.1810938588446,-67.0728602415266,-66.9644273644967,
-66.8730902106081),.UNSPECIFIED.);
#845=B_SPLINE_CURVE_WITH_KNOTS('',3,(#78772,#78773,#78774,#78775,#78776,
#78777,#78778,#78779,#78780,#78781,#78782,#78783,#78784,#78785,#78786,#78787,
#78788,#78789,#78790,#78791,#78792,#78793,#78794,#78795,#78796,#78797,#78798,
#78799,#78800,#78801,#78802,#78803,#78804,#78805,#78806,#78807,#78808,#78809,
#78810,#78811,#78812,#78813,#78814,#78815,#78816,#78817,#78818,#78819,#78820,
#78821,#78822,#78823,#78824,#78825,#78826,#78827,#78828,#78829,#78830,#78831,
#78832,#78833,#78834,#78835,#78836,#78837,#78838,#78839,#78840,#78841,#78842,
#78843,#78844,#78845,#78846,#78847,#78848,#78849,#78850,#78851,#78852,#78853,
#78854,#78855,#78856,#78857,#78858,#78859,#78860,#78861,#78862,#78863,#78864,
#78865,#78866,#78867,#78868,#78869,#78870,#78871,#78872,#78873,#78874,#78875,
#78876,#78877,#78878,#78879,#78880,#78881,#78882,#78883,#78884,#78885,#78886,
#78887,#78888,#78889,#78890,#78891,#78892,#78893,#78894,#78895,#78896,#78897,
#78898,#78899,#78900,#78901,#78902,#78903,#78904,#78905,#78906,#78907,#78908,
#78909,#78910,#78911,#78912,#78913,#78914,#78915,#78916,#78917,#78918,#78919,
#78920,#78921,#78922,#78923,#78924,#78925,#78926,#78927,#78928,#78929,#78930,
#78931,#78932,#78933,#78934,#78935,#78936,#78937,#78938,#78939,#78940,#78941,
#78942,#78943),.UNSPECIFIED.,.F.,.F.,(4,3,3,3,3,3,3,3,3,3,3,3,3,3,3,3,3,
3,3,3,3,3,3,3,3,3,3,3,3,3,3,3,3,3,3,3,3,3,3,3,3,3,3,3,3,3,3,3,3,3,3,3,3,
3,3,3,3,4),(-66.8730902100459,-66.8329409914535,-66.7237685527981,-66.6127267848848,
-66.5038546382296,-66.3950490323343,-66.2862699626363,-66.1735610743501,
-66.0646442130104,-65.9500393112509,-65.8354344094915,-65.7262619708361,
-65.6152202029228,-65.5063480562677,-65.3975424503725,-65.2887633806745,
-65.1760544923882,-65.0671376310485,-64.952532729289,-64.8379278275295,
-64.7287553888741,-64.6177136209608,-64.5088414743057,-64.4000358684105,
-64.2912567987124,-64.1785479104262,-64.0696310490865,-63.955026147327,
-63.8404212455675,-63.7312488069121,-63.6202070389988,-63.5113348923437,
-63.4025292864485,-63.2937502167505,-63.1810413284643,-63.0721244671246,
-62.957519565365,-62.8429146636055,-62.7337422249501,-62.6227004570368,
-62.5138283103817,-62.4050227044865,-62.2962436347884,-62.1835347465022,
-62.0746178851625,-61.960012983403,-61.8454080816435,-61.7362356429881,
-61.6251938750748,-61.5163217284197,-61.4075161225244,-61.2987370528264,
-61.1860281645402,-61.0771113032005,-60.962506401441,-60.8479014996816,
-60.708459556948,-60.5899049034139),.UNSPECIFIED.);
#846=B_SPLINE_CURVE_WITH_KNOTS('',3,(#78945,#78946,#78947,#78948,#78949,
#78950,#78951,#78952,#78953,#78954,#78955,#78956,#78957,#78958,#78959,#78960,
#78961,#78962,#78963,#78964,#78965,#78966,#78967,#78968,#78969,#78970,#78971,
#78972,#78973,#78974,#78975,#78976,#78977,#78978,#78979,#78980,#78981,#78982,
#78983,#78984,#78985,#78986,#78987,#78988,#78989,#78990,#78991,#78992,#78993,
#78994,#78995,#78996,#78997,#78998,#78999,#79000,#79001,#79002,#79003,#79004,
#79005,#79006,#79007,#79008,#79009,#79010,#79011,#79012,#79013,#79014,#79015,
#79016,#79017,#79018,#79019,#79020,#79021,#79022,#79023,#79024,#79025,#79026,
#79027,#79028,#79029,#79030,#79031,#79032,#79033,#79034,#79035,#79036,#79037,
#79038,#79039,#79040,#79041,#79042,#79043,#79044,#79045,#79046,#79047,#79048,
#79049,#79050,#79051,#79052,#79053,#79054,#79055,#79056,#79057,#79058,#79059,
#79060,#79061,#79062,#79063,#79064,#79065,#79066,#79067,#79068,#79069,#79070,
#79071,#79072,#79073,#79074,#79075,#79076,#79077,#79078,#79079,#79080,#79081,
#79082,#79083,#79084,#79085,#79086,#79087,#79088,#79089,#79090,#79091,#79092,
#79093,#79094,#79095,#79096,#79097,#79098,#79099,#79100,#79101,#79102,#79103,
#79104,#79105,#79106,#79107,#79108,#79109,#79110,#79111,#79112,#79113,#79114,
#79115,#79116),.UNSPECIFIED.,.F.,.F.,(4,3,3,3,3,3,3,3,3,3,3,3,3,3,3,3,3,
3,3,3,3,3,3,3,3,3,3,3,3,3,3,3,3,3,3,3,3,3,3,3,3,3,3,3,3,3,3,3,3,3,3,3,3,
3,3,3,3,4),(-60.5899049028662,-60.4821931879117,-60.3745475152884,-60.2669262422658,
-60.1592102498021,-60.0514492410922,-59.9434849929317,-59.8503949177196,
-59.7412224790642,-59.6301807111508,-59.5213085644957,-59.4125029586005,
-59.3037238889025,-59.1910150006163,-59.0820981392765,-58.9674932375171,
-58.8528883357576,-58.7437158971022,-58.6326741291889,-58.5238019825338,
-58.4149963766385,-58.3062173069406,-58.1935084186543,-58.0845915573146,
-57.9699866555551,-57.8553817537956,-57.7462093151402,-57.6351675472269,
-57.5262954005718,-57.4174897946765,-57.3087107249786,-57.1960018366923,
-57.0870849753527,-56.9724800735931,-56.8578751718336,-56.7487027331782,
-56.6376609652649,-56.5287888186098,-56.4199832127146,-56.3112041430166,
-56.1984952547304,-56.0895783933908,-55.9749734916312,-55.8603685898716,
-55.7511961512163,-55.640154383303,-55.5312822366479,-55.4224766307527,
-55.3136975610548,-55.2009886727685,-55.0920718114288,-54.9774669096692,
-54.8628620079096,-54.75063905054,-54.6386821891945,-54.5268818601967,-54.4152297097849,
-54.3067195956867),.UNSPECIFIED.);
#847=B_SPLINE_CURVE_WITH_KNOTS('',3,(#79118,#79119,#79120,#79121,#79122,
#79123,#79124,#79125,#79126,#79127,#79128,#79129,#79130,#79131,#79132,#79133,
#79134,#79135,#79136,#79137,#79138,#79139,#79140,#79141,#79142,#79143,#79144,
#79145,#79146,#79147,#79148,#79149,#79150,#79151,#79152,#79153,#79154,#79155,
#79156,#79157,#79158,#79159,#79160,#79161,#79162,#79163,#79164,#79165,#79166,
#79167,#79168,#79169,#79170,#79171,#79172,#79173,#79174,#79175,#79176,#79177,
#79178,#79179,#79180,#79181,#79182,#79183,#79184,#79185,#79186,#79187,#79188,
#79189,#79190,#79191,#79192,#79193,#79194,#79195,#79196,#79197,#79198,#79199,
#79200,#79201,#79202,#79203,#79204,#79205,#79206,#79207,#79208,#79209,#79210,
#79211,#79212,#79213,#79214,#79215,#79216,#79217,#79218,#79219,#79220,#79221,
#79222,#79223,#79224,#79225,#79226,#79227,#79228,#79229,#79230,#79231,#79232,
#79233,#79234,#79235,#79236,#79237,#79238,#79239,#79240,#79241,#79242,#79243,
#79244,#79245,#79246,#79247,#79248,#79249,#79250,#79251,#79252,#79253,#79254,
#79255,#79256,#79257,#79258,#79259,#79260,#79261,#79262,#79263,#79264,#79265,
#79266,#79267,#79268,#79269,#79270,#79271,#79272,#79273,#79274,#79275,#79276,
#79277,#79278,#79279,#79280,#79281,#79282,#79283,#79284,#79285,#79286,#79287,
#79288,#79289),.UNSPECIFIED.,.F.,.F.,(4,3,3,3,3,3,3,3,3,3,3,3,3,3,3,3,3,
3,3,3,3,3,3,3,3,3,3,3,3,3,3,3,3,3,3,3,3,3,3,3,3,3,3,3,3,3,3,3,3,3,3,3,3,
3,3,3,3,4),(-54.3067195951254,-54.189439388817,-54.0718637479082,-53.9538094079238,
-53.8653554259476,-53.7561829872923,-53.645141219379,-53.536269072724,-53.4274634668289,
-53.318684397131,-53.2059755088446,-53.0970586475051,-52.9824537457453,
-52.8678488439856,-52.7586764053301,-52.6476346374168,-52.5387624907616,
-52.4299568848663,-52.3211778151681,-52.208468926882,-52.0995520655422,
-51.9849471637829,-51.8703422620236,-51.7611698233683,-51.6501280554549,
-51.5412559087998,-51.4324503029046,-51.3236712332067,-51.2109623449204,
-51.1020454835807,-50.9874405818212,-50.8728356800616,-50.7636632414063,
-50.6526214734929,-50.5437493268379,-50.4349437209427,-50.3261646512448,
-50.2134557629585,-50.1045389016188,-49.9899339998592,-49.8753290980996,
-49.7661566594441,-49.6551148915308,-49.5462427448756,-49.4374371389804,
-49.3286580692823,-49.2159491809961,-49.1070323196563,-48.992427417897,
-48.8778225161376,-48.770283184556,-48.6628909290572,-48.5556033712,-48.4483782985246,
-48.3411132279635,-48.2338352157278,-48.1263962591731,-48.0235342889076),
 .UNSPECIFIED.);
#848=B_SPLINE_CURVE_WITH_KNOTS('',3,(#79291,#79292,#79293,#79294,#79295,
#79296,#79297,#79298,#79299,#79300,#79301,#79302,#79303,#79304,#79305,#79306,
#79307,#79308,#79309,#79310,#79311,#79312,#79313,#79314,#79315,#79316,#79317,
#79318,#79319,#79320,#79321,#79322,#79323,#79324,#79325,#79326,#79327,#79328,
#79329,#79330,#79331,#79332,#79333,#79334,#79335,#79336,#79337,#79338,#79339,
#79340,#79341,#79342,#79343,#79344,#79345,#79346,#79347,#79348,#79349,#79350,
#79351,#79352,#79353,#79354,#79355,#79356,#79357,#79358,#79359,#79360,#79361,
#79362,#79363,#79364,#79365,#79366,#79367,#79368,#79369,#79370,#79371,#79372,
#79373,#79374,#79375,#79376,#79377,#79378,#79379,#79380,#79381,#79382,#79383,
#79384,#79385,#79386,#79387,#79388,#79389,#79390,#79391,#79392,#79393,#79394,
#79395,#79396,#79397,#79398,#79399,#79400,#79401,#79402,#79403,#79404,#79405,
#79406,#79407,#79408,#79409,#79410,#79411,#79412,#79413,#79414,#79415,#79416,
#79417,#79418,#79419,#79420,#79421,#79422,#79423,#79424,#79425,#79426,#79427,
#79428,#79429,#79430,#79431,#79432,#79433,#79434,#79435,#79436,#79437,#79438,
#79439,#79440,#79441,#79442,#79443,#79444,#79445,#79446,#79447,#79448,#79449,
#79450,#79451,#79452,#79453,#79454,#79455,#79456,#79457,#79458,#79459),
 .UNSPECIFIED.,.F.,.F.,(4,3,3,3,3,3,3,3,3,3,3,3,3,3,3,3,3,3,3,3,3,3,3,3,
3,3,3,3,3,3,3,3,3,3,3,3,3,3,3,3,3,3,3,3,3,3,3,3,3,3,3,3,3,3,3,3,4),(-48.0235342885071,
-47.8803159341757,-47.77114349552,-47.6601017276067,-47.5512295809513,-47.4424239750557,
-47.3336449053574,-47.2209360170715,-47.1120191557314,-46.9974142539726,
-46.8828093522137,-46.7736369135582,-46.6625951456449,-46.5537229989897,
-46.4449173930943,-46.3361383233961,-46.22342943511,-46.1145125737702,-45.9999076720109,
-45.8853027702517,-45.7761303315965,-45.6650885636831,-45.5562164170282,
-45.4474108111331,-45.3386317414353,-45.2259228531489,-45.1170059918093,
-45.0024010900495,-44.8877961882897,-44.7786237496343,-44.667581981721,
-44.5587098350659,-44.4499042291706,-44.3411251594726,-44.2284162711863,
-44.1194994098466,-44.0048945080872,-43.8902896063277,-43.7811171676722,
-43.6700753997589,-43.5612032531037,-43.4523976472084,-43.3436185775103,
-43.2309096892242,-43.1219928278844,-43.0073879261251,-42.8927830243657,
-42.7836105857104,-42.6725688177971,-42.563696671142,-42.4548910652469,
-42.346111995549,-42.2334031072627,-42.1244862459231,-42.0098813441634,
-41.8952764424037,-41.7403489813275),.UNSPECIFIED.);
#849=B_SPLINE_CURVE_WITH_KNOTS('',3,(#79461,#79462,#79463,#79464,#79465,
#79466,#79467,#79468,#79469,#79470,#79471,#79472,#79473,#79474,#79475,#79476,
#79477,#79478,#79479,#79480,#79481,#79482,#79483,#79484,#79485,#79486,#79487,
#79488,#79489,#79490,#79491,#79492,#79493,#79494,#79495,#79496,#79497,#79498,
#79499,#79500,#79501,#79502,#79503,#79504,#79505,#79506,#79507,#79508,#79509,
#79510,#79511,#79512,#79513,#79514,#79515,#79516,#79517,#79518,#79519,#79520,
#79521,#79522,#79523,#79524,#79525,#79526,#79527,#79528,#79529,#79530,#79531,
#79532,#79533,#79534,#79535,#79536,#79537,#79538,#79539,#79540,#79541,#79542,
#79543,#79544,#79545,#79546,#79547,#79548,#79549,#79550,#79551,#79552,#79553,
#79554,#79555,#79556,#79557,#79558,#79559,#79560,#79561,#79562,#79563,#79564,
#79565,#79566,#79567,#79568,#79569,#79570,#79571,#79572,#79573,#79574,#79575,
#79576,#79577,#79578,#79579,#79580,#79581,#79582,#79583,#79584,#79585,#79586,
#79587,#79588,#79589,#79590,#79591,#79592,#79593,#79594,#79595,#79596,#79597,
#79598,#79599,#79600,#79601,#79602,#79603,#79604,#79605,#79606,#79607,#79608,
#79609,#79610,#79611,#79612,#79613,#79614,#79615,#79616,#79617,#79618,#79619,
#79620,#79621,#79622,#79623,#79624,#79625,#79626,#79627,#79628,#79629,#79630,
#79631,#79632),.UNSPECIFIED.,.F.,.F.,(4,3,3,3,3,3,3,3,3,3,3,3,3,3,3,3,3,
3,3,3,3,3,3,3,3,3,3,3,3,3,3,3,3,3,3,3,3,3,3,3,3,3,3,3,3,3,3,3,3,3,3,3,3,
3,3,3,3,4),(-41.7403489809666,-41.6329490692741,-41.5256623867346,-41.4184466672188,
-41.3112597576395,-41.2039837574797,-41.096665730506,-40.9891488560991,
-40.8977698604417,-40.7885974217861,-40.6775556538728,-40.5686835072176,
-40.4598779013223,-40.3510988316241,-40.238389943338,-40.1294730819981,
-40.0148681802389,-39.9002632784797,-39.7910908398243,-39.680049071911,
-39.571176925256,-39.4623713193608,-39.3535922496629,-39.2408833613766,
-39.131966500037,-39.0173615982773,-38.9027566965177,-38.7935842578622,
-38.6825424899489,-38.5736703432938,-38.4648647373985,-38.3560856677007,
-38.2433767794144,-38.1344599180748,-38.0198550163152,-37.9052501145557,
-37.7960776759003,-37.6850359079869,-37.5761637613317,-37.4673581554365,
-37.3585790857385,-37.2458701974523,-37.1369533361124,-37.0223484343531,
-36.9077435325937,-36.7985710939385,-36.6875293260252,-36.5786571793702,
-36.469851573475,-36.3610725037773,-36.2483636154909,-36.1394467541514,
-36.0248418523915,-35.9102369506317,-35.792973733972,-35.6759975257706,
-35.5594572831808,-35.4571636746066),.UNSPECIFIED.);
#850=B_SPLINE_CURVE_WITH_KNOTS('',3,(#79634,#79635,#79636,#79637,#79638,
#79639,#79640,#79641,#79642,#79643,#79644,#79645,#79646,#79647,#79648,#79649,
#79650,#79651,#79652,#79653,#79654,#79655,#79656,#79657,#79658,#79659,#79660,
#79661,#79662,#79663,#79664,#79665,#79666,#79667,#79668,#79669,#79670,#79671,
#79672,#79673,#79674,#79675,#79676,#79677,#79678,#79679,#79680,#79681,#79682,
#79683,#79684,#79685,#79686,#79687,#79688,#79689,#79690,#79691,#79692,#79693,
#79694,#79695,#79696,#79697,#79698,#79699,#79700,#79701,#79702,#79703,#79704,
#79705,#79706,#79707,#79708,#79709,#79710,#79711,#79712,#79713,#79714,#79715,
#79716,#79717,#79718,#79719,#79720,#79721,#79722,#79723,#79724,#79725,#79726,
#79727,#79728,#79729,#79730,#79731,#79732,#79733,#79734,#79735,#79736,#79737,
#79738,#79739,#79740,#79741,#79742,#79743,#79744,#79745,#79746,#79747,#79748,
#79749,#79750,#79751,#79752,#79753,#79754,#79755,#79756,#79757,#79758,#79759,
#79760,#79761,#79762,#79763,#79764,#79765,#79766,#79767,#79768,#79769,#79770,
#79771,#79772,#79773,#79774,#79775,#79776,#79777,#79778,#79779,#79780,#79781,
#79782,#79783,#79784,#79785,#79786,#79787,#79788,#79789,#79790,#79791,#79792,
#79793,#79794,#79795,#79796,#79797,#79798,#79799,#79800,#79801,#79802,#79803,
#79804,#79805),.UNSPECIFIED.,.F.,.F.,(4,3,3,3,3,3,3,3,3,3,3,3,3,3,3,3,3,
3,3,3,3,3,3,3,3,3,3,3,3,3,3,3,3,3,3,3,3,3,3,3,3,3,3,3,3,3,3,3,3,3,3,3,3,
3,3,3,3,4),(-35.4571636741479,-35.3451567223982,-35.2329232796229,-35.1205751861138,
-35.0079430284769,-34.9127303686697,-34.8035579300143,-34.692516162101,
-34.583644015446,-34.4748384095508,-34.3660593398529,-34.2533504515666,
-34.144433590227,-34.0298286884674,-33.9152237867078,-33.8060513480526,
-33.6950095801392,-33.5861374334843,-33.4773318275893,-33.3685527578914,
-33.255843869605,-33.1469270082655,-33.0323221065056,-32.9177172047458,
-32.8085447660899,-32.6975029981766,-32.588630851521,-32.4798252456253,
-32.371046175927,-32.2583372876412,-32.149420426301,-32.0348155245424,-31.9202106227838,
-31.8110381841289,-31.6999964162155,-31.5911242695608,-31.482318663666,
-31.3735395939685,-31.2608307056818,-31.1519138443426,-31.0373089425822,
-30.9227040408218,-30.8135316021673,-30.7024898342538,-30.5936176875995,
-30.4848120817052,-30.3760330120079,-30.2633241237209,-30.1544072623821,
-30.039802360621,-29.9251974588598,-29.8173426398448,-29.7096404023268,
-29.602048690314,-29.4944927141703,-29.3869653894048,-29.2793456073155,
-29.1739783669683),.UNSPECIFIED.);
#851=B_SPLINE_CURVE_WITH_KNOTS('',3,(#79807,#79808,#79809,#79810,#79811,
#79812,#79813,#79814,#79815,#79816,#79817,#79818,#79819,#79820,#79821,#79822,
#79823,#79824,#79825,#79826,#79827,#79828,#79829,#79830,#79831,#79832,#79833,
#79834,#79835,#79836,#79837,#79838,#79839,#79840,#79841,#79842,#79843,#79844,
#79845,#79846,#79847,#79848,#79849,#79850,#79851,#79852,#79853,#79854,#79855,
#79856,#79857,#79858,#79859,#79860,#79861,#79862,#79863,#79864,#79865,#79866,
#79867,#79868,#79869,#79870,#79871,#79872,#79873,#79874,#79875,#79876,#79877,
#79878,#79879,#79880,#79881,#79882,#79883,#79884,#79885,#79886,#79887,#79888,
#79889,#79890,#79891,#79892,#79893,#79894,#79895,#79896,#79897,#79898,#79899,
#79900,#79901,#79902,#79903,#79904,#79905,#79906,#79907,#79908,#79909,#79910,
#79911,#79912,#79913,#79914,#79915,#79916,#79917,#79918,#79919,#79920,#79921,
#79922,#79923,#79924,#79925,#79926,#79927,#79928,#79929,#79930,#79931,#79932,
#79933,#79934,#79935,#79936,#79937,#79938,#79939,#79940,#79941,#79942,#79943,
#79944,#79945,#79946,#79947,#79948,#79949,#79950,#79951,#79952,#79953,#79954,
#79955,#79956,#79957,#79958,#79959,#79960,#79961,#79962,#79963,#79964,#79965,
#79966,#79967,#79968,#79969,#79970,#79971,#79972,#79973,#79974,#79975,#79976,
#79977,#79978),.UNSPECIFIED.,.F.,.F.,(4,3,3,3,3,3,3,3,3,3,3,3,3,3,3,3,3,
3,3,3,3,3,3,3,3,3,3,3,3,3,3,3,3,3,3,3,3,3,3,3,3,3,3,3,3,3,3,3,3,3,3,3,3,
3,3,3,3,4),(-29.1739783663998,-29.0319114532481,-28.9276908768978,-28.818518438247,
-28.7074766703331,-28.5986045236825,-28.4897989177918,-28.3810198480982,
-28.2683109598076,-28.1593940984721,-28.044789196704,-27.9301842949358,
-27.8210118562849,-27.709970088371,-27.6010979417206,-27.4922923358301,
-27.3835132661369,-27.2708043778461,-27.1618875165112,-27.0472826147425,
-26.9326777129738,-26.8235052742899,-26.7124635063801,-26.6035913596964,
-26.4947857537726,-26.3860066840462,-26.2732977957876,-26.16438093442,-26.0497760327159,
-25.9351711310118,-25.8259986924006,-25.7149569244818,-25.6060847778703,
-25.4972791720185,-25.3885001023634,-25.275791214035,-25.1668743527369,
-25.0522694508933,-24.9376645490498,-24.8284921104129,-24.7174503424973,
-24.608578195862,-24.499772589987,-24.3909935203097,-24.2782846320042,-24.169367770686,
-24.0547628688869,-23.9401579670878,-23.8309855282153,-23.7199437603291,
-23.611071613456,-23.5022660073431,-23.393486937428,-23.2807780493524,-23.1718611877997,
-23.0572562864627,-22.9426513851258,-22.8907930597887),.UNSPECIFIED.);
#852=B_SPLINE_CURVE_WITH_KNOTS('',3,(#79980,#79981,#79982,#79983,#79984,
#79985,#79986,#79987,#79988,#79989,#79990,#79991,#79992,#79993,#79994,#79995,
#79996,#79997,#79998,#79999,#80000,#80001,#80002,#80003,#80004,#80005,#80006,
#80007,#80008,#80009,#80010,#80011,#80012,#80013,#80014,#80015,#80016,#80017,
#80018,#80019,#80020,#80021,#80022,#80023,#80024,#80025,#80026,#80027,#80028,
#80029,#80030,#80031,#80032,#80033,#80034,#80035,#80036,#80037,#80038,#80039,
#80040,#80041,#80042,#80043,#80044,#80045,#80046,#80047,#80048,#80049,#80050,
#80051,#80052,#80053,#80054,#80055,#80056,#80057,#80058,#80059,#80060,#80061,
#80062,#80063,#80064,#80065,#80066,#80067,#80068,#80069,#80070,#80071,#80072,
#80073,#80074,#80075,#80076,#80077,#80078,#80079,#80080,#80081,#80082,#80083,
#80084,#80085,#80086,#80087,#80088,#80089,#80090,#80091,#80092,#80093,#80094,
#80095,#80096,#80097,#80098,#80099,#80100,#80101,#80102,#80103,#80104,#80105,
#80106,#80107,#80108,#80109,#80110,#80111,#80112,#80113,#80114,#80115,#80116,
#80117,#80118,#80119,#80120,#80121,#80122,#80123,#80124,#80125,#80126,#80127,
#80128,#80129,#80130,#80131,#80132,#80133,#80134,#80135,#80136,#80137,#80138,
#80139,#80140,#80141,#80142,#80143,#80144,#80145,#80146,#80147,#80148,#80149,
#80150,#80151),.UNSPECIFIED.,.F.,.F.,(4,3,3,3,3,3,3,3,3,3,3,3,3,3,3,3,3,
3,3,3,3,3,3,3,3,3,3,3,3,3,3,3,3,3,3,3,3,3,3,3,3,3,3,3,3,3,3,3,3,3,3,3,3,
3,3,3,3,4),(-22.8907930594592,-22.7824986164422,-22.6743864007115,-22.5663749719121,
-22.4584229836816,-22.3504891765429,-22.2424561812702,-22.1343732431433,
-22.0260911452468,-21.9451448031638,-21.835972364515,-21.7249305966008,
-21.6160584499633,-21.5072528440898,-21.3984737744173,-21.2857648861134,
-21.1768480248088,-21.0622431230053,-20.9476382212018,-20.8384657809417,
-20.727424013229,-20.618551864959,-20.5097462574496,-20.4009671861407,-20.2882582994155,
-20.1793414364916,-20.0647365378658,-19.9501316392399,-19.840959204042,
-19.7299174356965,-19.6210452924763,-19.5122396899983,-19.4034606236942,
-19.2907517320901,-19.1818348740486,-19.0672299656633,-18.9526250572779,
-18.8434526175422,-18.7324108497639,-18.623538702118,-18.5147330952675,
-18.4059540246515,-18.2932451373176,-18.1843282751608,-18.0697233752383,
-17.9551184753159,-17.845946025166,-17.7349042586895,-17.6260321004361,
-17.517226482936,-17.4084474016456,-17.2957385245727,-17.1868216518051,
-17.0722167725795,-16.9576118933539,-16.8315168208368,-16.7065414420316,
-16.6076077530562),.UNSPECIFIED.);
#853=B_SPLINE_CURVE_WITH_KNOTS('',3,(#80153,#80154,#80155,#80156,#80157,
#80158,#80159,#80160,#80161,#80162,#80163,#80164,#80165,#80166,#80167,#80168,
#80169,#80170,#80171,#80172,#80173,#80174,#80175,#80176,#80177,#80178,#80179,
#80180,#80181,#80182,#80183,#80184,#80185,#80186,#80187,#80188,#80189,#80190,
#80191,#80192,#80193,#80194,#80195,#80196,#80197,#80198,#80199,#80200,#80201,
#80202,#80203,#80204,#80205,#80206,#80207,#80208,#80209,#80210,#80211,#80212,
#80213,#80214,#80215,#80216,#80217,#80218,#80219,#80220,#80221,#80222,#80223,
#80224,#80225,#80226,#80227,#80228,#80229,#80230,#80231,#80232,#80233,#80234,
#80235,#80236,#80237,#80238,#80239,#80240,#80241,#80242,#80243,#80244,#80245,
#80246,#80247,#80248,#80249,#80250,#80251,#80252,#80253,#80254,#80255,#80256,
#80257,#80258,#80259,#80260,#80261,#80262,#80263,#80264,#80265,#80266,#80267,
#80268,#80269,#80270,#80271,#80272,#80273,#80274,#80275,#80276,#80277,#80278,
#80279,#80280,#80281,#80282,#80283,#80284,#80285,#80286,#80287,#80288,#80289,
#80290,#80291,#80292,#80293,#80294,#80295,#80296,#80297,#80298,#80299,#80300,
#80301,#80302,#80303,#80304,#80305,#80306,#80307,#80308,#80309,#80310,#80311,
#80312,#80313,#80314,#80315,#80316,#80317,#80318,#80319,#80320,#80321,#80322,
#80323,#80324),.UNSPECIFIED.,.F.,.F.,(4,3,3,3,3,3,3,3,3,3,3,3,3,3,3,3,3,
3,3,3,3,3,3,3,3,3,3,3,3,3,3,3,3,3,3,3,3,3,3,3,3,3,3,3,3,3,3,3,3,3,3,3,3,
3,3,3,3,4),(-16.6076077526091,-16.4985515258746,-16.3894995583923,-16.2803263451299,
-16.1710948393509,-16.061638988216,-15.9601053113919,-15.8509328552173,
-15.7398910894939,-15.6310189260239,-15.5222133036192,-15.4134342177412,
-15.3007253456633,-15.1918084691386,-15.0772035992843,-14.9625987294299,
-14.8534262116324,-14.7423844536118,-14.6335122268185,-14.5247065406372,
-14.4159273906366,-14.3032185798444,-14.1943016390933,-14.0796968932806,
-13.9650921474679,-13.8559199507005,-13.7448781525512,-13.636006247127,
-13.5272008815609,-13.4184220509095,-13.3057129295586,-13.1967963013489,
-13.0821909334274,-12.9675855655059,-12.8584129186525,-12.7473711767639,
-12.6384988273246,-12.529693021194,-12.42091375411,-12.3082050614685,-12.1992880120175,
-12.0846834977807,-11.9700789835439,-11.8609060285232,-11.7498643251556,
-11.6409916530149,-11.532185519713,-11.4234059215571,-11.3106975415633,
-11.2017801553197,-11.0871762784508,-10.9725724015819,-10.8631125115013,
-10.7538223022557,-10.6446684475115,-10.5355975774757,-10.4265343818605,
-10.3244224454296),.UNSPECIFIED.);
#854=B_SPLINE_CURVE_WITH_KNOTS('',3,(#80325,#80326,#80327,#80328,#80329,
#80330,#80331,#80332,#80333,#80334,#80335,#80336,#80337,#80338,#80339,#80340,
#80341,#80342,#80343,#80344,#80345,#80346,#80347,#80348,#80349,#80350,#80351,
#80352,#80353,#80354,#80355,#80356,#80357,#80358,#80359,#80360,#80361,#80362,
#80363,#80364,#80365,#80366,#80367,#80368,#80369,#80370,#80371,#80372,#80373,
#80374,#80375,#80376,#80377,#80378,#80379,#80380,#80381,#80382,#80383,#80384,
#80385,#80386,#80387,#80388,#80389,#80390,#80391,#80392,#80393,#80394,#80395,
#80396,#80397,#80398,#80399,#80400,#80401,#80402,#80403,#80404,#80405,#80406,
#80407,#80408,#80409,#80410,#80411,#80412,#80413,#80414,#80415,#80416,#80417,
#80418,#80419,#80420,#80421,#80422,#80423,#80424,#80425,#80426,#80427,#80428,
#80429,#80430,#80431,#80432,#80433,#80434,#80435,#80436,#80437,#80438,#80439,
#80440,#80441,#80442,#80443,#80444,#80445,#80446,#80447,#80448,#80449,#80450,
#80451,#80452,#80453,#80454,#80455,#80456,#80457,#80458,#80459,#80460,#80461,
#80462,#80463,#80464,#80465,#80466,#80467,#80468,#80469,#80470,#80471,#80472,
#80473,#80474,#80475,#80476,#80477,#80478,#80479,#80480,#80481,#80482,#80483,
#80484,#80485,#80486,#80487,#80488,#80489,#80490,#80491,#80492,#80493,#80494,
#80495,#80496),.UNSPECIFIED.,.F.,.F.,(4,3,3,3,3,3,3,3,3,3,3,3,3,3,3,3,3,
3,3,3,3,3,3,3,3,3,3,3,3,3,3,3,3,3,3,3,3,3,3,3,3,3,3,3,3,3,3,3,3,3,3,3,3,
3,3,3,3,4),(-10.3244224449829,-10.1995927077105,-10.073593116902,-9.97506581961992,
-9.86589120680441,-9.7548497106611,-9.64597543043115,-9.53716771174615,
-9.4283865532732,-9.31567972436938,-9.20676085735733,-9.09216004750763,
-8.97755923765793,-8.86838369578316,-8.75734231577226,-8.64846698531538,
-8.53965817465189,-8.43087588459778,-8.31817007737232,-8.20924999482244,
-8.09465132525919,-7.98005265569594,-7.87089564873598,-7.75985195186073,
-7.6509952491671,-7.54220504959516,-7.43344132405663,-7.32071751147596,
-7.2118156641143,-7.09718086892413,-6.98254607373395,-6.87335254294226,
-6.76231341154597,-6.65342046864044,-6.54459423251996,-6.43579473058479,
-6.32310592088158,-6.21416934992145,-6.0996044208467,-5.98503949177195,
-5.87585101044478,-5.76481124786543,-5.65592236636929,-5.54709981657177,
-5.43830362330433,-5.32561094493074,-5.21667671851355,-5.10210481416175,
-4.98753290980996,-4.87932161623076,-4.77130015508177,-4.66338411673174,
-4.55553201849392,-4.44770247128745,-4.33977959528017,-4.231810353224,-4.1236459576977,
-4.04123713858906),.UNSPECIFIED.);
#855=B_SPLINE_CURVE_WITH_KNOTS('',3,(#80499,#80500,#80501,#80502,#80503,
#80504,#80505,#80506,#80507,#80508,#80509,#80510,#80511,#80512,#80513,#80514,
#80515,#80516,#80517,#80518,#80519,#80520,#80521,#80522,#80523,#80524,#80525,
#80526,#80527,#80528,#80529,#80530,#80531,#80532,#80533,#80534,#80535,#80536,
#80537,#80538,#80539,#80540,#80541,#80542,#80543,#80544,#80545,#80546,#80547,
#80548,#80549,#80550,#80551,#80552,#80553,#80554,#80555,#80556,#80557,#80558,
#80559,#80560,#80561,#80562,#80563,#80564,#80565,#80566,#80567,#80568,#80569,
#80570,#80571,#80572,#80573,#80574,#80575,#80576,#80577,#80578,#80579,#80580,
#80581,#80582,#80583,#80584,#80585,#80586,#80587,#80588,#80589,#80590,#80591,
#80592,#80593,#80594,#80595,#80596,#80597,#80598,#80599,#80600,#80601,#80602,
#80603,#80604,#80605,#80606,#80607,#80608,#80609,#80610,#80611,#80612,#80613,
#80614,#80615,#80616,#80617,#80618,#80619,#80620,#80621,#80622,#80623,#80624,
#80625,#80626,#80627,#80628,#80629,#80630,#80631,#80632,#80633,#80634,#80635,
#80636,#80637,#80638,#80639,#80640,#80641,#80642,#80643,#80644,#80645,#80646,
#80647,#80648,#80649,#80650,#80651,#80652,#80653,#80654,#80655,#80656,#80657,
#80658,#80659,#80660,#80661,#80662,#80663,#80664,#80665,#80666,#80667,#80668,
#80669,#80670,#80671,#80672,#80673,#80674,#80675,#80676,#80677,#80678,#80679,
#80680,#80681,#80682),.UNSPECIFIED.,.F.,.F.,(4,2,2,2,2,2,2,2,2,2,2,2,2,
2,2,2,2,2,2,2,2,2,2,2,2,2,2,2,2,2,2,2,2,2,2,2,2,2,2,2,2,2,2,2,2,2,2,2,2,
2,2,2,2,2,2,2,2,2,2,2,2,2,2,2,2,2,2,2,2,2,2,2,2,2,2,2,2,2,2,2,2,2,2,2,2,
2,2,2,2,2,2,4),(0.00170434132766192,0.00222412714886743,0.00373601697648723,
0.0059415231071054,0.0117360227398377,0.017247955900676,0.017345838820968,
0.0174552527306371,0.0175774491000871,0.0374495435397178,0.0564270685292465,
0.0621405782386566,0.0652770672322874,0.0679619515167662,0.0712524927571661,
0.0763431234435016,0.102928841043105,0.123180376523087,0.126539422500572,
0.128307276186441,0.129676046129487,0.131560486136817,0.135367328950562,
0.152782962332486,0.167564078927962,0.178903712896266,0.182678939142569,
0.18821226293721,0.191298880215098,0.193967152687614,0.197269305304302,
0.202435535612447,0.22966587140207,0.244485620429274,0.249765905044866,
0.253630236470186,0.255506916157342,0.257001517832908,0.258873224420235,
0.262755254770772,0.281475463725533,0.303371544332112,0.313561671749094,
0.317406143038283,0.320124030405426,0.32258720604536,0.325900736712319,
0.334235710145613,0.362108165961765,0.377483591113132,0.381245848717689,
0.38309199948349,0.384434512856435,0.386250802041238,0.389713645455654,
0.415420966420263,0.431318841396034,0.438066890234673,0.443476504489122,
0.446530575575806,0.449190669476744,0.452508468110459,0.457752142300946,
0.478430974805413,0.497830187895307,0.502372988413577,0.507752871488063,
0.509887545386098,0.511409903047414,0.513114681621342,0.516141724622532,
0.535119214841241,0.550306121472088,0.561411665912576,0.565127868494102,
0.570591548050806,0.573654184871182,0.576309378965146,0.579604763978552,
0.586248897086325,0.616023804690947,0.627890307045252,0.634688156072327,
0.637011355795411,0.638564255999007,0.639990803976973,0.642464443964867,
0.649913308050295,0.672047429990563,0.686608283213725,0.693008730419268,
0.693071669236789),.UNSPECIFIED.);
#856=B_SPLINE_CURVE_WITH_KNOTS('',3,(#80685,#80686,#80687,#80688,#80689,
#80690,#80691,#80692,#80693,#80694,#80695,#80696,#80697,#80698,#80699,#80700,
#80701,#80702,#80703,#80704,#80705,#80706,#80707,#80708,#80709,#80710,#80711,
#80712,#80713,#80714,#80715,#80716,#80717,#80718,#80719,#80720,#80721,#80722,
#80723,#80724,#80725,#80726,#80727,#80728,#80729,#80730,#80731,#80732,#80733,
#80734,#80735,#80736,#80737,#80738,#80739,#80740,#80741,#80742,#80743,#80744,
#80745,#80746,#80747,#80748,#80749,#80750,#80751,#80752,#80753,#80754,#80755,
#80756,#80757,#80758,#80759,#80760,#80761,#80762,#80763,#80764,#80765,#80766,
#80767,#80768,#80769,#80770,#80771,#80772,#80773,#80774,#80775,#80776,#80777,
#80778,#80779,#80780,#80781,#80782,#80783,#80784,#80785,#80786,#80787,#80788,
#80789,#80790,#80791,#80792,#80793,#80794,#80795,#80796,#80797,#80798,#80799,
#80800,#80801,#80802,#80803,#80804,#80805,#80806,#80807,#80808,#80809,#80810,
#80811,#80812,#80813,#80814,#80815,#80816,#80817,#80818),.UNSPECIFIED.,
 .F.,.F.,(4,2,2,2,2,2,2,2,2,2,2,2,2,2,2,2,2,2,2,2,2,2,2,2,2,2,2,2,2,2,2,
2,2,2,2,2,2,2,2,2,2,2,2,2,2,2,2,2,2,2,2,2,2,2,2,2,2,2,2,2,2,2,2,2,2,2,4),
(-1.21432109392595,-1.21309489238909,-1.21161499497023,-1.20825651986386,
-1.19086412431765,-1.17341047878535,-1.16320924961495,-1.16000169195814,
-1.15685872449779,-1.15385408419519,-1.15026350757091,-1.14160636751801,
-1.11192084073898,-1.09879692054717,-1.09381828270841,-1.09021572424298,
-1.0886892369214,-1.08716890249636,-1.08551775590911,-1.08257570974892,
-1.06466749901094,-1.04288623040399,-1.03112489252229,-1.02718586039154,
-1.02452873706152,-1.02193600082763,-1.01819402636549,-1.00884615489993,
-0.978163101527409,-0.968318526508513,-0.962341623811722,-0.960198655696911,
-0.958712428561933,-0.957078828496771,-0.954369277831652,-0.944505008315516,
-0.92406809812312,-0.904827116101953,-0.89914520706868,-0.896014892835797,
-0.893329234251391,-0.890030050485331,-0.884910586675138,-0.858803055882306,
-0.844148749484679,-0.838902933278007,-0.835050012219561,-0.833154148950896,
-0.831632301850252,-0.82970469115684,-0.825608588436889,-0.796933686108921,
-0.778625224269768,-0.773093220731051,-0.770006727556216,-0.767338178168486,
-0.764035169042359,-0.758866437518332,-0.731636077449794,-0.716792357624474,
-0.711506749238995,-0.707639951393525,-0.705762701889296,-0.704267960777809,
-0.702396420488034,-0.698515765632526,-0.693046076597336),.UNSPECIFIED.);
#857=B_SPLINE_CURVE_WITH_KNOTS('',3,(#80823,#80824,#80825,#80826,#80827,
#80828,#80829,#80830,#80831,#80832,#80833,#80834,#80835,#80836,#80837,#80838,
#80839,#80840,#80841,#80842,#80843,#80844,#80845,#80846,#80847,#80848,#80849,
#80850,#80851,#80852,#80853,#80854,#80855,#80856,#80857,#80858,#80859,#80860,
#80861,#80862,#80863,#80864,#80865,#80866,#80867,#80868,#80869,#80870,#80871,
#80872,#80873,#80874,#80875,#80876,#80877,#80878,#80879,#80880,#80881,#80882,
#80883,#80884,#80885,#80886,#80887,#80888,#80889,#80890,#80891,#80892,#80893,
#80894,#80895,#80896,#80897,#80898),.UNSPECIFIED.,.F.,.F.,(4,3,3,3,3,3,
3,3,3,3,3,3,3,3,3,3,3,3,3,3,3,3,3,3,3,4),(-0.295806004217947,-0.276346276763905,
-0.259134503548442,-0.254903097588525,-0.235929794728117,-0.223290645753993,
-0.218631610496081,-0.200430896336404,-0.182506041781569,-0.171709967209082,
-0.162747187230736,-0.158780673832424,-0.1416815104781,-0.139485560058239,
-0.121912858869917,-0.106673751511178,-0.103639837841612,-0.0867995465133564,
-0.0700962905132021,-0.0537853027443874,-0.0504514462069721,-0.0476210400737898,
-0.0318234390049184,-0.0159117195024592,-0.000873246935291439,0.),
 .UNSPECIFIED.);
#858=B_SPLINE_CURVE_WITH_KNOTS('',3,(#80900,#80901,#80902,#80903),
 .UNSPECIFIED.,.F.,.F.,(4,4),(0.,0.0104675605378427),.UNSPECIFIED.);
#859=B_SPLINE_CURVE_WITH_KNOTS('',3,(#80904,#80905,#80906,#80907,#80908,
#80909,#80910,#80911,#80912,#80913,#80914,#80915,#80916,#80917,#80918,#80919,
#80920,#80921,#80922,#80923,#80924,#80925,#80926,#80927,#80928,#80929,#80930,
#80931,#80932,#80933,#80934,#80935,#80936,#80937,#80938,#80939,#80940,#80941,
#80942,#80943,#80944,#80945,#80946,#80947,#80948,#80949,#80950,#80951,#80952,
#80953,#80954,#80955,#80956,#80957,#80958,#80959,#80960,#80961,#80962,#80963,
#80964,#80965,#80966,#80967,#80968,#80969,#80970,#80971,#80972,#80973,#80974,
#80975,#80976,#80977,#80978,#80979,#80980,#80981,#80982),.UNSPECIFIED.,
 .F.,.F.,(4,3,3,3,3,3,3,3,3,3,3,3,3,3,3,3,3,3,3,3,3,3,3,3,3,3,4),(-0.300067541140031,
-0.284903583137558,-0.273513846777917,-0.269501705381138,-0.253425057571093,
-0.24192514309105,-0.238272923892424,-0.221674243793147,-0.204570474865403,
-0.187512420545603,-0.184305757918836,-0.181394803662524,-0.163580075937423,
-0.161367923522646,-0.144185213822354,-0.13484192266634,-0.12798949631024,
-0.123541197591128,-0.10530462789074,-0.0870680581903524,-0.0684458915674173,
-0.0648760934804545,-0.0612715484369567,-0.0420158017011555,-0.0227263924376532,
-0.00360798048806816,0.),.UNSPECIFIED.);
#860=B_SPLINE_CURVE_WITH_KNOTS('',3,(#81492,#81493,#81494,#81495),
 .UNSPECIFIED.,.F.,.F.,(4,4),(-0.0234817857221697,0.),.UNSPECIFIED.);
#861=B_SPLINE_CURVE_WITH_KNOTS('',3,(#81497,#81498,#81499,#81500,#81501,
#81502,#81503,#81504,#81505,#81506,#81507,#81508,#81509,#81510,#81511,#81512,
#81513,#81514,#81515,#81516,#81517,#81518,#81519,#81520,#81521,#81522,#81523,
#81524,#81525,#81526,#81527,#81528,#81529,#81530,#81531,#81532,#81533,#81534,
#81535,#81536,#81537,#81538,#81539,#81540,#81541,#81542,#81543,#81544,#81545,
#81546,#81547,#81548,#81549,#81550,#81551,#81552,#81553,#81554,#81555,#81556,
#81557,#81558,#81559,#81560,#81561,#81562,#81563,#81564,#81565,#81566,#81567,
#81568,#81569,#81570,#81571,#81572,#81573,#81574,#81575),.UNSPECIFIED.,
 .F.,.F.,(4,3,3,3,3,3,3,3,3,3,3,3,3,3,3,3,3,3,3,3,3,3,3,3,3,3,4),(-0.300067541140086,
-0.28490359311403,-0.273513832743188,-0.26950170426489,-0.253425062718846,
-0.241925147594606,-0.238272927914922,-0.221674254034694,-0.20457048503947,
-0.193769844660272,-0.184305769912281,-0.181394826747799,-0.163580099041372,
-0.161367923522675,-0.144185214827314,-0.134841924365739,-0.127989499740197,
-0.123541196970117,-0.105507157043589,-0.0870680627985426,-0.0684461374457819,
-0.06487607603814,-0.0612715444558154,-0.0420000585199136,-0.0227107712124592,
-0.00360796795722674,-1.56163160422294E-14),.UNSPECIFIED.);
#862=B_SPLINE_CURVE_WITH_KNOTS('',3,(#81576,#81577,#81578,#81579),
 .UNSPECIFIED.,.F.,.F.,(4,4),(-0.0104673718805252,0.),.UNSPECIFIED.);
#863=B_SPLINE_CURVE_WITH_KNOTS('',3,(#81584,#81585,#81586,#81587,#81588,
#81589,#81590,#81591,#81592,#81593,#81594,#81595,#81596,#81597,#81598,#81599,
#81600,#81601,#81602,#81603,#81604,#81605,#81606,#81607,#81608,#81609,#81610,
#81611,#81612,#81613,#81614,#81615,#81616,#81617,#81618,#81619,#81620,#81621,
#81622,#81623,#81624,#81625,#81626,#81627,#81628,#81629,#81630,#81631,#81632,
#81633,#81634,#81635,#81636,#81637,#81638,#81639,#81640,#81641,#81642,#81643,
#81644,#81645,#81646,#81647,#81648,#81649,#81650,#81651,#81652,#81653,#81654,
#81655,#81656,#81657,#81658,#81659),.UNSPECIFIED.,.F.,.F.,(4,3,3,3,3,3,
3,3,3,3,3,3,3,3,3,3,3,3,3,3,3,3,3,3,3,4),(-0.295805969970282,-0.276346242507802,
-0.259134493682388,-0.254903093723924,-0.235948130553021,-0.223290631511216,
-0.218631609492188,-0.200430890716852,-0.182506029139112,-0.171709957912945,
-0.162747174009377,-0.158780670974258,-0.141681498829962,-0.139485560058265,
-0.121907132417156,-0.106673752808531,-0.10363984067179,-0.0867987766194497,
-0.0702234074835109,-0.0537853237239207,-0.0504510919926865,-0.047620967918163,
-0.0318233773104902,-0.0159116886552451,-0.000873229362510297,0.),
 .UNSPECIFIED.);
#864=B_SPLINE_CURVE_WITH_KNOTS('',3,(#82169,#82170,#82171,#82172),
 .UNSPECIFIED.,.F.,.F.,(4,4),(-0.0234821165293861,0.),.UNSPECIFIED.);
#903=B_SPLINE_SURFACE_WITH_KNOTS('',3,3,((#80984,#80985,#80986,#80987,#80988,
#80989,#80990,#80991,#80992,#80993,#80994,#80995,#80996,#80997,#80998,#80999,
#81000,#81001,#81002,#81003,#81004,#81005,#81006,#81007,#81008,#81009,#81010,
#81011,#81012,#81013,#81014,#81015,#81016,#81017,#81018,#81019,#81020,#81021,
#81022,#81023,#81024,#81025,#81026,#81027,#81028,#81029,#81030,#81031,#81032,
#81033,#81034,#81035,#81036,#81037,#81038,#81039,#81040,#81041,#81042,#81043,
#81044,#81045,#81046,#81047,#81048,#81049,#81050,#81051,#81052,#81053,#81054,
#81055,#81056,#81057,#81058,#81059,#81060,#81061,#81062,#81063,#81064,#81065,
#81066,#81067,#81068,#81069,#81070,#81071,#81072,#81073,#81074,#81075,#81076,
#81077,#81078,#81079,#81080,#81081,#81082,#81083,#81084,#81085,#81086,#81087,
#81088,#81089,#81090,#81091,#81092,#81093,#81094,#81095,#81096,#81097,#81098,
#81099,#81100,#81101,#81102,#81103,#81104,#81105,#81106,#81107,#81108,#81109,
#81110),(#81111,#81112,#81113,#81114,#81115,#81116,#81117,#81118,#81119,
#81120,#81121,#81122,#81123,#81124,#81125,#81126,#81127,#81128,#81129,#81130,
#81131,#81132,#81133,#81134,#81135,#81136,#81137,#81138,#81139,#81140,#81141,
#81142,#81143,#81144,#81145,#81146,#81147,#81148,#81149,#81150,#81151,#81152,
#81153,#81154,#81155,#81156,#81157,#81158,#81159,#81160,#81161,#81162,#81163,
#81164,#81165,#81166,#81167,#81168,#81169,#81170,#81171,#81172,#81173,#81174,
#81175,#81176,#81177,#81178,#81179,#81180,#81181,#81182,#81183,#81184,#81185,
#81186,#81187,#81188,#81189,#81190,#81191,#81192,#81193,#81194,#81195,#81196,
#81197,#81198,#81199,#81200,#81201,#81202,#81203,#81204,#81205,#81206,#81207,
#81208,#81209,#81210,#81211,#81212,#81213,#81214,#81215,#81216,#81217,#81218,
#81219,#81220,#81221,#81222,#81223,#81224,#81225,#81226,#81227,#81228,#81229,
#81230,#81231,#81232,#81233,#81234,#81235,#81236,#81237),(#81238,#81239,
#81240,#81241,#81242,#81243,#81244,#81245,#81246,#81247,#81248,#81249,#81250,
#81251,#81252,#81253,#81254,#81255,#81256,#81257,#81258,#81259,#81260,#81261,
#81262,#81263,#81264,#81265,#81266,#81267,#81268,#81269,#81270,#81271,#81272,
#81273,#81274,#81275,#81276,#81277,#81278,#81279,#81280,#81281,#81282,#81283,
#81284,#81285,#81286,#81287,#81288,#81289,#81290,#81291,#81292,#81293,#81294,
#81295,#81296,#81297,#81298,#81299,#81300,#81301,#81302,#81303,#81304,#81305,
#81306,#81307,#81308,#81309,#81310,#81311,#81312,#81313,#81314,#81315,#81316,
#81317,#81318,#81319,#81320,#81321,#81322,#81323,#81324,#81325,#81326,#81327,
#81328,#81329,#81330,#81331,#81332,#81333,#81334,#81335,#81336,#81337,#81338,
#81339,#81340,#81341,#81342,#81343,#81344,#81345,#81346,#81347,#81348,#81349,
#81350,#81351,#81352,#81353,#81354,#81355,#81356,#81357,#81358,#81359,#81360,
#81361,#81362,#81363,#81364),(#81365,#81366,#81367,#81368,#81369,#81370,
#81371,#81372,#81373,#81374,#81375,#81376,#81377,#81378,#81379,#81380,#81381,
#81382,#81383,#81384,#81385,#81386,#81387,#81388,#81389,#81390,#81391,#81392,
#81393,#81394,#81395,#81396,#81397,#81398,#81399,#81400,#81401,#81402,#81403,
#81404,#81405,#81406,#81407,#81408,#81409,#81410,#81411,#81412,#81413,#81414,
#81415,#81416,#81417,#81418,#81419,#81420,#81421,#81422,#81423,#81424,#81425,
#81426,#81427,#81428,#81429,#81430,#81431,#81432,#81433,#81434,#81435,#81436,
#81437,#81438,#81439,#81440,#81441,#81442,#81443,#81444,#81445,#81446,#81447,
#81448,#81449,#81450,#81451,#81452,#81453,#81454,#81455,#81456,#81457,#81458,
#81459,#81460,#81461,#81462,#81463,#81464,#81465,#81466,#81467,#81468,#81469,
#81470,#81471,#81472,#81473,#81474,#81475,#81476,#81477,#81478,#81479,#81480,
#81481,#81482,#81483,#81484,#81485,#81486,#81487,#81488,#81489,#81490,#81491)),
 .UNSPECIFIED.,.F.,.F.,.F.,(4,4),(4,1,1,1,1,1,1,1,1,1,1,1,1,1,1,1,1,1,1,
1,1,1,1,1,1,1,1,1,1,1,1,1,1,1,1,1,1,1,1,1,1,1,1,1,1,1,1,1,1,1,1,1,1,1,1,
1,1,1,1,1,1,1,1,1,1,1,1,1,1,1,1,1,1,1,1,1,1,1,1,1,1,1,1,1,1,1,1,1,1,1,1,
1,1,1,1,1,1,1,1,1,1,1,1,1,1,1,1,1,1,1,1,1,1,1,1,1,1,1,1,1,1,1,1,1,4),(-0.000266755740803004,
0.0504104417085662),(8.3394004212115,9.33690700317349,10.3344135851355,
11.3319201670975,12.3294267490595,13.3269333310215,14.3244399129835,15.3219464949454,
16.3194530769074,17.3169596588694,18.3144662408314,19.3119728227934,20.3094794047554,
21.3069859867174,22.3044925686794,23.3019991506414,24.2995057326034,25.2970123145654,
26.2945188965274,27.2920254784894,28.2895320604514,29.2870386424133,30.2845452243753,
31.2820518063373,32.2795583882993,33.2770649702613,34.2745715522233,35.2720781341853,
36.2695847161473,37.2670912981093,38.2645978800713,39.2621044620333,40.2596110439953,
41.2571176259573,42.2546242079192,43.2521307898812,44.2496373718432,45.2471439538052,
46.2446505357672,47.2421571177292,48.2396636996912,49.2371702816532,50.2346768636152,
51.2321834455772,52.2296900275392,53.2271966095012,54.2247031914632,55.2222097734252,
56.2197163553871,57.2172229373491,58.2147295193111,59.2122361012731,60.2097426832351,
61.2072492651971,62.2047558471591,63.2022624291211,64.1997690110831,65.1972755930451,
66.1947821750071,67.1922887569691,68.189795338931,69.187301920893,70.184808502855,
71.182315084817,72.179821666779,73.177328248741,74.174834830703,75.172341412665,
76.169847994627,77.167354576589,78.164861158551,79.162367740513,80.159874322475,
81.157380904437,82.154887486399,83.1523940683609,84.1499006503229,85.1474072322849,
86.1449138142469,87.1424203962089,88.1399269781709,89.1374335601329,90.1349401420949,
91.1324467240569,92.1299533060189,93.1274598879809,94.1249664699429,95.1224730519048,
96.1199796338668,97.1174862158288,98.1149927977908,99.1124993797528,100.110005961715,
101.107512543677,102.105019125639,103.102525707601,104.100032289563,105.097538871525,
106.095045453487,107.092552035449,108.090058617411,109.087565199373,110.085071781335,
111.082578363297,112.080084945259,113.077591527221,114.075098109183,115.072604691145,
116.070111273107,117.067617855069,118.065124437031,119.062631018993,120.060137600955,
121.057644182917,122.055150764879,123.052657346841,124.050163928803,125.047670510765,
126.045177092727,127.042683674689,128.040190256651,129.037696838613,130.035203420575,
131.032710002537,132.03048334024),.UNSPECIFIED.);
#904=B_SPLINE_SURFACE_WITH_KNOTS('',3,3,((#81661,#81662,#81663,#81664,#81665,
#81666,#81667,#81668,#81669,#81670,#81671,#81672,#81673,#81674,#81675,#81676,
#81677,#81678,#81679,#81680,#81681,#81682,#81683,#81684,#81685,#81686,#81687,
#81688,#81689,#81690,#81691,#81692,#81693,#81694,#81695,#81696,#81697,#81698,
#81699,#81700,#81701,#81702,#81703,#81704,#81705,#81706,#81707,#81708,#81709,
#81710,#81711,#81712,#81713,#81714,#81715,#81716,#81717,#81718,#81719,#81720,
#81721,#81722,#81723,#81724,#81725,#81726,#81727,#81728,#81729,#81730,#81731,
#81732,#81733,#81734,#81735,#81736,#81737,#81738,#81739,#81740,#81741,#81742,
#81743,#81744,#81745,#81746,#81747,#81748,#81749,#81750,#81751,#81752,#81753,
#81754,#81755,#81756,#81757,#81758,#81759,#81760,#81761,#81762,#81763,#81764,
#81765,#81766,#81767,#81768,#81769,#81770,#81771,#81772,#81773,#81774,#81775,
#81776,#81777,#81778,#81779,#81780,#81781,#81782,#81783,#81784,#81785,#81786,
#81787),(#81788,#81789,#81790,#81791,#81792,#81793,#81794,#81795,#81796,
#81797,#81798,#81799,#81800,#81801,#81802,#81803,#81804,#81805,#81806,#81807,
#81808,#81809,#81810,#81811,#81812,#81813,#81814,#81815,#81816,#81817,#81818,
#81819,#81820,#81821,#81822,#81823,#81824,#81825,#81826,#81827,#81828,#81829,
#81830,#81831,#81832,#81833,#81834,#81835,#81836,#81837,#81838,#81839,#81840,
#81841,#81842,#81843,#81844,#81845,#81846,#81847,#81848,#81849,#81850,#81851,
#81852,#81853,#81854,#81855,#81856,#81857,#81858,#81859,#81860,#81861,#81862,
#81863,#81864,#81865,#81866,#81867,#81868,#81869,#81870,#81871,#81872,#81873,
#81874,#81875,#81876,#81877,#81878,#81879,#81880,#81881,#81882,#81883,#81884,
#81885,#81886,#81887,#81888,#81889,#81890,#81891,#81892,#81893,#81894,#81895,
#81896,#81897,#81898,#81899,#81900,#81901,#81902,#81903,#81904,#81905,#81906,
#81907,#81908,#81909,#81910,#81911,#81912,#81913,#81914),(#81915,#81916,
#81917,#81918,#81919,#81920,#81921,#81922,#81923,#81924,#81925,#81926,#81927,
#81928,#81929,#81930,#81931,#81932,#81933,#81934,#81935,#81936,#81937,#81938,
#81939,#81940,#81941,#81942,#81943,#81944,#81945,#81946,#81947,#81948,#81949,
#81950,#81951,#81952,#81953,#81954,#81955,#81956,#81957,#81958,#81959,#81960,
#81961,#81962,#81963,#81964,#81965,#81966,#81967,#81968,#81969,#81970,#81971,
#81972,#81973,#81974,#81975,#81976,#81977,#81978,#81979,#81980,#81981,#81982,
#81983,#81984,#81985,#81986,#81987,#81988,#81989,#81990,#81991,#81992,#81993,
#81994,#81995,#81996,#81997,#81998,#81999,#82000,#82001,#82002,#82003,#82004,
#82005,#82006,#82007,#82008,#82009,#82010,#82011,#82012,#82013,#82014,#82015,
#82016,#82017,#82018,#82019,#82020,#82021,#82022,#82023,#82024,#82025,#82026,
#82027,#82028,#82029,#82030,#82031,#82032,#82033,#82034,#82035,#82036,#82037,
#82038,#82039,#82040,#82041),(#82042,#82043,#82044,#82045,#82046,#82047,
#82048,#82049,#82050,#82051,#82052,#82053,#82054,#82055,#82056,#82057,#82058,
#82059,#82060,#82061,#82062,#82063,#82064,#82065,#82066,#82067,#82068,#82069,
#82070,#82071,#82072,#82073,#82074,#82075,#82076,#82077,#82078,#82079,#82080,
#82081,#82082,#82083,#82084,#82085,#82086,#82087,#82088,#82089,#82090,#82091,
#82092,#82093,#82094,#82095,#82096,#82097,#82098,#82099,#82100,#82101,#82102,
#82103,#82104,#82105,#82106,#82107,#82108,#82109,#82110,#82111,#82112,#82113,
#82114,#82115,#82116,#82117,#82118,#82119,#82120,#82121,#82122,#82123,#82124,
#82125,#82126,#82127,#82128,#82129,#82130,#82131,#82132,#82133,#82134,#82135,
#82136,#82137,#82138,#82139,#82140,#82141,#82142,#82143,#82144,#82145,#82146,
#82147,#82148,#82149,#82150,#82151,#82152,#82153,#82154,#82155,#82156,#82157,
#82158,#82159,#82160,#82161,#82162,#82163,#82164,#82165,#82166,#82167,#82168)),
 .UNSPECIFIED.,.F.,.F.,.F.,(4,4),(4,1,1,1,1,1,1,1,1,1,1,1,1,1,1,1,1,1,1,
1,1,1,1,1,1,1,1,1,1,1,1,1,1,1,1,1,1,1,1,1,1,1,1,1,1,1,1,1,1,1,1,1,1,1,1,
1,1,1,1,1,1,1,1,1,1,1,1,1,1,1,1,1,1,1,1,1,1,1,1,1,1,1,1,1,1,1,1,1,1,1,1,
1,1,1,1,1,1,1,1,1,1,1,1,1,1,1,1,1,1,1,1,1,1,1,1,1,1,1,1,1,1,1,1,1,4),(-0.000246377393080283,
0.0504200384722922),(11.6664593544106,12.6642327116609,13.6617392936229,
14.6592458755849,15.6567524575469,16.6542590395089,17.6517656214709,18.6492722034329,
19.6467787853949,20.6442853673569,21.6417919493189,22.6392985312808,23.6368051132428,
24.6343116952048,25.6318182771668,26.6293248591288,27.6268314410908,28.6243380230528,
29.6218446050148,30.6193511869768,31.6168577689388,32.6143643509008,33.6118709328628,
34.6093775148248,35.6068840967868,36.6043906787487,37.6018972607107,38.5994038426727,
39.5969104246347,40.5944170065967,41.5919235885587,42.5894301705207,43.5869367524827,
44.5844433344447,45.5819499164067,46.5794564983687,47.5769630803307,48.5744696622927,
49.5719762442546,50.5694828262166,51.5669894081786,52.5644959901406,53.5620025721026,
54.5595091540646,55.5570157360266,56.5545223179886,57.5520288999506,58.5495354819126,
59.5470420638746,60.5445486458366,61.5420552277986,62.5395618097606,63.5370683917225,
64.5345749736845,65.5320815556465,66.5295881376085,67.5270947195705,68.5246013015325,
69.5221078834945,70.5196144654565,71.5171210474185,72.5146276293805,73.5121342113425,
74.5096407933045,75.5071473752665,76.5046539572285,77.5021605391904,78.4996671211524,
79.4971737031144,80.4946802850764,81.4921868670384,82.4896934490004,83.4872000309624,
84.4847066129244,85.4822131948864,86.4797197768484,87.4772263588104,88.4747329407724,
89.4722395227344,90.4697461046964,91.4672526866584,92.4647592686204,93.4622658505823,
94.4597724325443,95.4572790145063,96.4547855964683,97.4522921784303,98.4497987603923,
99.4473053423543,100.444811924316,101.442318506278,102.43982508824,103.437331670202,
104.434838252164,105.432344834126,106.429851416088,107.42735799805,108.424864580012,
109.422371161974,110.419877743936,111.417384325898,112.41489090786,113.412397489822,
114.409904071784,115.407410653746,116.404917235708,117.40242381767,118.399930399632,
119.397436981594,120.394943563556,121.392450145518,122.38995672748,123.387463309442,
124.384969891404,125.382476473366,126.379983055328,127.37748963729,128.374996219252,
129.372502801214,130.370009383176,131.367515965138,132.3650225471,133.362529129062,
134.360035711024,135.357542292986),.UNSPECIFIED.);
#916=SHAPE_REPRESENTATION_RELATIONSHIP('SRR','None',#83311,#930);
#930=ADVANCED_BREP_SHAPE_REPRESENTATION('',(#958),#83216);
#944=STYLED_ITEM('',(#83390),#958);
#958=MANIFOLD_SOLID_BREP('Body1',#26940);
#1115=FACE_BOUND('',#5121,.T.);
#1116=FACE_BOUND('',#5235,.T.);
#2005=PLANE('',#28953);
#2006=PLANE('',#28956);
#2007=PLANE('',#28962);
#2008=PLANE('',#28966);
#2009=PLANE('',#28967);
#2010=PLANE('',#28968);
#2011=PLANE('',#28969);
#2012=PLANE('',#29009);
#2013=PLANE('',#29010);
#2014=PLANE('',#29011);
#2015=PLANE('',#29013);
#2016=PLANE('',#29014);
#2017=PLANE('',#29015);
#2018=PLANE('',#29017);
#2019=PLANE('',#29018);
#2020=PLANE('',#29019);
#2021=PLANE('',#29021);
#2022=PLANE('',#29022);
#2023=PLANE('',#29023);
#2024=PLANE('',#29025);
#2025=PLANE('',#29026);
#2026=PLANE('',#29027);
#2027=PLANE('',#29029);
#2028=PLANE('',#29030);
#2029=PLANE('',#29031);
#2030=PLANE('',#29033);
#2031=PLANE('',#29034);
#2032=PLANE('',#29035);
#2033=PLANE('',#29037);
#2034=PLANE('',#29038);
#2035=PLANE('',#29039);
#2036=PLANE('',#29041);
#2037=PLANE('',#29042);
#2038=PLANE('',#29043);
#2039=PLANE('',#29045);
#2040=PLANE('',#29046);
#2041=PLANE('',#29047);
#2042=PLANE('',#29049);
#2043=PLANE('',#29050);
#2044=PLANE('',#29051);
#2045=PLANE('',#29053);
#2046=PLANE('',#29054);
#2047=PLANE('',#29055);
#2048=PLANE('',#29057);
#2049=PLANE('',#29058);
#2050=PLANE('',#29059);
#2051=PLANE('',#29061);
#2052=PLANE('',#29062);
#2053=PLANE('',#29063);
#2054=PLANE('',#29065);
#2055=PLANE('',#29066);
#2056=PLANE('',#29067);
#2057=PLANE('',#29069);
#2058=PLANE('',#29070);
#2059=PLANE('',#29071);
#2060=PLANE('',#29073);
#2061=PLANE('',#29074);
#2062=PLANE('',#29075);
#2063=PLANE('',#29078);
#2064=PLANE('',#29079);
#2065=PLANE('',#29080);
#2066=PLANE('',#29082);
#2067=PLANE('',#29083);
#2068=PLANE('',#29084);
#2069=PLANE('',#29086);
#2070=PLANE('',#29087);
#2071=PLANE('',#29088);
#2072=PLANE('',#29090);
#2073=PLANE('',#29091);
#2074=PLANE('',#29092);
#2075=PLANE('',#29094);
#2076=PLANE('',#29095);
#2077=PLANE('',#29096);
#2078=PLANE('',#29098);
#2079=PLANE('',#29099);
#2080=PLANE('',#29100);
#2081=PLANE('',#29102);
#2082=PLANE('',#29103);
#2083=PLANE('',#29104);
#2084=PLANE('',#29106);
#2085=PLANE('',#29107);
#2086=PLANE('',#29108);
#2087=PLANE('',#29110);
#2088=PLANE('',#29111);
#2089=PLANE('',#29112);
#2090=PLANE('',#29114);
#2091=PLANE('',#29115);
#2092=PLANE('',#29116);
#2093=PLANE('',#29118);
#2094=PLANE('',#29119);
#2095=PLANE('',#29120);
#2096=PLANE('',#29122);
#2097=PLANE('',#29123);
#2098=PLANE('',#29124);
#2099=PLANE('',#29126);
#2100=PLANE('',#29127);
#2101=PLANE('',#29128);
#2102=PLANE('',#29130);
#2103=PLANE('',#29131);
#2104=PLANE('',#29132);
#2105=PLANE('',#29134);
#2106=PLANE('',#29135);
#2107=PLANE('',#29136);
#2108=PLANE('',#29138);
#2109=PLANE('',#29139);
#2110=PLANE('',#29140);
#2111=PLANE('',#29142);
#2112=PLANE('',#29143);
#2113=PLANE('',#29144);
#2114=PLANE('',#29146);
#2115=PLANE('',#29147);
#2116=PLANE('',#29148);
#2117=PLANE('',#29151);
#2118=PLANE('',#29152);
#2119=PLANE('',#29154);
#2120=PLANE('',#29156);
#2121=PLANE('',#29158);
#2122=PLANE('',#29160);
#2123=PLANE('',#29162);
#2124=PLANE('',#29165);
#2125=PLANE('',#29166);
#2126=PLANE('',#29167);
#2127=PLANE('',#29168);
#2128=PLANE('',#29169);
#2129=PLANE('',#29170);
#2330=CYLINDRICAL_SURFACE('',#28928,1.26999999999999);
#2331=CYLINDRICAL_SURFACE('',#28930,1.26999999999999);
#2332=CYLINDRICAL_SURFACE('',#28931,1.26999999999999);
#2333=CYLINDRICAL_SURFACE('',#28932,1.26999999999999);
#2334=CYLINDRICAL_SURFACE('',#28933,1.26999999999999);
#2335=CYLINDRICAL_SURFACE('',#28934,1.26999999999999);
#2336=CYLINDRICAL_SURFACE('',#28935,1.26999999999999);
#2337=CYLINDRICAL_SURFACE('',#28936,1.26999999999999);
#2338=CYLINDRICAL_SURFACE('',#28937,1.26999999999999);
#2339=CYLINDRICAL_SURFACE('',#28938,1.26999999999999);
#2340=CYLINDRICAL_SURFACE('',#28939,1.26999999999999);
#2341=CYLINDRICAL_SURFACE('',#28940,1.26999999999999);
#2342=CYLINDRICAL_SURFACE('',#28941,1.26999999999999);
#2343=CYLINDRICAL_SURFACE('',#28942,1.26999999999999);
#2344=CYLINDRICAL_SURFACE('',#28943,1.26999999999999);
#2345=CYLINDRICAL_SURFACE('',#28944,1.26999999999999);
#2346=CYLINDRICAL_SURFACE('',#28945,1.26999999999999);
#2347=CYLINDRICAL_SURFACE('',#28946,1.26999999999999);
#2348=CYLINDRICAL_SURFACE('',#28947,1.26999999999999);
#2349=CYLINDRICAL_SURFACE('',#28948,1.70434);
#2350=CYLINDRICAL_SURFACE('',#28951,1.26999999999999);
#2351=CYLINDRICAL_SURFACE('',#29150,2.8702);
#3561=FACE_OUTER_BOUND('',#5094,.T.);
#3562=FACE_OUTER_BOUND('',#5095,.T.);
#3563=FACE_OUTER_BOUND('',#5096,.T.);
#3564=FACE_OUTER_BOUND('',#5097,.T.);
#3565=FACE_OUTER_BOUND('',#5098,.T.);
#3566=FACE_OUTER_BOUND('',#5099,.T.);
#3567=FACE_OUTER_BOUND('',#5100,.T.);
#3568=FACE_OUTER_BOUND('',#5101,.T.);
#3569=FACE_OUTER_BOUND('',#5102,.T.);
#3570=FACE_OUTER_BOUND('',#5103,.T.);
#3571=FACE_OUTER_BOUND('',#5104,.T.);
#3572=FACE_OUTER_BOUND('',#5105,.T.);
#3573=FACE_OUTER_BOUND('',#5106,.T.);
#3574=FACE_OUTER_BOUND('',#5107,.T.);
#3575=FACE_OUTER_BOUND('',#5108,.T.);
#3576=FACE_OUTER_BOUND('',#5109,.T.);
#3577=FACE_OUTER_BOUND('',#5110,.T.);
#3578=FACE_OUTER_BOUND('',#5111,.T.);
#3579=FACE_OUTER_BOUND('',#5112,.T.);
#3580=FACE_OUTER_BOUND('',#5113,.T.);
#3581=FACE_OUTER_BOUND('',#5114,.T.);
#3582=FACE_OUTER_BOUND('',#5115,.T.);
#3583=FACE_OUTER_BOUND('',#5116,.T.);
#3584=FACE_OUTER_BOUND('',#5117,.T.);
#3585=FACE_OUTER_BOUND('',#5118,.T.);
#3586=FACE_OUTER_BOUND('',#5119,.T.);
#3587=FACE_OUTER_BOUND('',#5120,.T.);
#3588=FACE_OUTER_BOUND('',#5122,.T.);
#3589=FACE_OUTER_BOUND('',#5123,.T.);
#3590=FACE_OUTER_BOUND('',#5124,.T.);
#3591=FACE_OUTER_BOUND('',#5125,.T.);
#3592=FACE_OUTER_BOUND('',#5126,.T.);
#3593=FACE_OUTER_BOUND('',#5127,.T.);
#3594=FACE_OUTER_BOUND('',#5128,.T.);
#3595=FACE_OUTER_BOUND('',#5129,.T.);
#3596=FACE_OUTER_BOUND('',#5130,.T.);
#3597=FACE_OUTER_BOUND('',#5131,.T.);
#3598=FACE_OUTER_BOUND('',#5132,.T.);
#3599=FACE_OUTER_BOUND('',#5133,.T.);
#3600=FACE_OUTER_BOUND('',#5134,.T.);
#3601=FACE_OUTER_BOUND('',#5135,.T.);
#3602=FACE_OUTER_BOUND('',#5136,.T.);
#3603=FACE_OUTER_BOUND('',#5137,.T.);
#3604=FACE_OUTER_BOUND('',#5138,.T.);
#3605=FACE_OUTER_BOUND('',#5139,.T.);
#3606=FACE_OUTER_BOUND('',#5140,.T.);
#3607=FACE_OUTER_BOUND('',#5141,.T.);
#3608=FACE_OUTER_BOUND('',#5142,.T.);
#3609=FACE_OUTER_BOUND('',#5143,.T.);
#3610=FACE_OUTER_BOUND('',#5144,.T.);
#3611=FACE_OUTER_BOUND('',#5145,.T.);
#3612=FACE_OUTER_BOUND('',#5146,.T.);
#3613=FACE_OUTER_BOUND('',#5147,.T.);
#3614=FACE_OUTER_BOUND('',#5148,.T.);
#3615=FACE_OUTER_BOUND('',#5149,.T.);
#3616=FACE_OUTER_BOUND('',#5150,.T.);
#3617=FACE_OUTER_BOUND('',#5151,.T.);
#3618=FACE_OUTER_BOUND('',#5152,.T.);
#3619=FACE_OUTER_BOUND('',#5153,.T.);
#3620=FACE_OUTER_BOUND('',#5154,.T.);
#3621=FACE_OUTER_BOUND('',#5155,.T.);
#3622=FACE_OUTER_BOUND('',#5156,.T.);
#3623=FACE_OUTER_BOUND('',#5157,.T.);
#3624=FACE_OUTER_BOUND('',#5158,.T.);
#3625=FACE_OUTER_BOUND('',#5159,.T.);
#3626=FACE_OUTER_BOUND('',#5160,.T.);
#3627=FACE_OUTER_BOUND('',#5161,.T.);
#3628=FACE_OUTER_BOUND('',#5162,.T.);
#3629=FACE_OUTER_BOUND('',#5163,.T.);
#3630=FACE_OUTER_BOUND('',#5164,.T.);
#3631=FACE_OUTER_BOUND('',#5165,.T.);
#3632=FACE_OUTER_BOUND('',#5166,.T.);
#3633=FACE_OUTER_BOUND('',#5167,.T.);
#3634=FACE_OUTER_BOUND('',#5168,.T.);
#3635=FACE_OUTER_BOUND('',#5169,.T.);
#3636=FACE_OUTER_BOUND('',#5170,.T.);
#3637=FACE_OUTER_BOUND('',#5171,.T.);
#3638=FACE_OUTER_BOUND('',#5172,.T.);
#3639=FACE_OUTER_BOUND('',#5173,.T.);
#3640=FACE_OUTER_BOUND('',#5174,.T.);
#3641=FACE_OUTER_BOUND('',#5175,.T.);
#3642=FACE_OUTER_BOUND('',#5176,.T.);
#3643=FACE_OUTER_BOUND('',#5177,.T.);
#3644=FACE_OUTER_BOUND('',#5178,.T.);
#3645=FACE_OUTER_BOUND('',#5179,.T.);
#3646=FACE_OUTER_BOUND('',#5180,.T.);
#3647=FACE_OUTER_BOUND('',#5181,.T.);
#3648=FACE_OUTER_BOUND('',#5182,.T.);
#3649=FACE_OUTER_BOUND('',#5183,.T.);
#3650=FACE_OUTER_BOUND('',#5184,.T.);
#3651=FACE_OUTER_BOUND('',#5185,.T.);
#3652=FACE_OUTER_BOUND('',#5186,.T.);
#3653=FACE_OUTER_BOUND('',#5187,.T.);
#3654=FACE_OUTER_BOUND('',#5188,.T.);
#3655=FACE_OUTER_BOUND('',#5189,.T.);
#3656=FACE_OUTER_BOUND('',#5190,.T.);
#3657=FACE_OUTER_BOUND('',#5191,.T.);
#3658=FACE_OUTER_BOUND('',#5192,.T.);
#3659=FACE_OUTER_BOUND('',#5193,.T.);
#3660=FACE_OUTER_BOUND('',#5194,.T.);
#3661=FACE_OUTER_BOUND('',#5195,.T.);
#3662=FACE_OUTER_BOUND('',#5196,.T.);
#3663=FACE_OUTER_BOUND('',#5197,.T.);
#3664=FACE_OUTER_BOUND('',#5198,.T.);
#3665=FACE_OUTER_BOUND('',#5199,.T.);
#3666=FACE_OUTER_BOUND('',#5200,.T.);
#3667=FACE_OUTER_BOUND('',#5201,.T.);
#3668=FACE_OUTER_BOUND('',#5202,.T.);
#3669=FACE_OUTER_BOUND('',#5203,.T.);
#3670=FACE_OUTER_BOUND('',#5204,.T.);
#3671=FACE_OUTER_BOUND('',#5205,.T.);
#3672=FACE_OUTER_BOUND('',#5206,.T.);
#3673=FACE_OUTER_BOUND('',#5207,.T.);
#3674=FACE_OUTER_BOUND('',#5208,.T.);
#3675=FACE_OUTER_BOUND('',#5209,.T.);
#3676=FACE_OUTER_BOUND('',#5210,.T.);
#3677=FACE_OUTER_BOUND('',#5211,.T.);
#3678=FACE_OUTER_BOUND('',#5212,.T.);
#3679=FACE_OUTER_BOUND('',#5213,.T.);
#3680=FACE_OUTER_BOUND('',#5214,.T.);
#3681=FACE_OUTER_BOUND('',#5215,.T.);
#3682=FACE_OUTER_BOUND('',#5216,.T.);
#3683=FACE_OUTER_BOUND('',#5217,.T.);
#3684=FACE_OUTER_BOUND('',#5218,.T.);
#3685=FACE_OUTER_BOUND('',#5219,.T.);
#3686=FACE_OUTER_BOUND('',#5220,.T.);
#3687=FACE_OUTER_BOUND('',#5221,.T.);
#3688=FACE_OUTER_BOUND('',#5222,.T.);
#3689=FACE_OUTER_BOUND('',#5223,.T.);
#3690=FACE_OUTER_BOUND('',#5224,.T.);
#3691=FACE_OUTER_BOUND('',#5225,.T.);
#3692=FACE_OUTER_BOUND('',#5226,.T.);
#3693=FACE_OUTER_BOUND('',#5227,.T.);
#3694=FACE_OUTER_BOUND('',#5228,.T.);
#3695=FACE_OUTER_BOUND('',#5229,.T.);
#3696=FACE_OUTER_BOUND('',#5230,.T.);
#3697=FACE_OUTER_BOUND('',#5231,.T.);
#3698=FACE_OUTER_BOUND('',#5232,.T.);
#3699=FACE_OUTER_BOUND('',#5233,.T.);
#3700=FACE_OUTER_BOUND('',#5234,.T.);
#3701=FACE_OUTER_BOUND('',#5236,.T.);
#3702=FACE_OUTER_BOUND('',#5237,.T.);
#3703=FACE_OUTER_BOUND('',#5238,.T.);
#3704=FACE_OUTER_BOUND('',#5239,.T.);
#3705=FACE_OUTER_BOUND('',#5240,.T.);
#3706=FACE_OUTER_BOUND('',#5241,.T.);
#3707=FACE_OUTER_BOUND('',#5242,.T.);
#3708=FACE_OUTER_BOUND('',#5243,.T.);
#3709=FACE_OUTER_BOUND('',#5244,.T.);
#3710=FACE_OUTER_BOUND('',#5245,.T.);
#3711=FACE_OUTER_BOUND('',#5246,.T.);
#3712=FACE_OUTER_BOUND('',#5247,.T.);
#3713=FACE_OUTER_BOUND('',#5248,.T.);
#5094=EDGE_LOOP('',(#24372,#24373,#24374,#24375));
#5095=EDGE_LOOP('',(#24376,#24377,#24378,#24379));
#5096=EDGE_LOOP('',(#24380,#24381,#24382,#24383,#24384,#24385));
#5097=EDGE_LOOP('',(#24386,#24387,#24388,#24389,#24390));
#5098=EDGE_LOOP('',(#24391,#24392,#24393,#24394,#24395,#24396));
#5099=EDGE_LOOP('',(#24397,#24398,#24399,#24400));
#5100=EDGE_LOOP('',(#24401,#24402,#24403,#24404,#24405,#24406));
#5101=EDGE_LOOP('',(#24407,#24408,#24409,#24410));
#5102=EDGE_LOOP('',(#24411,#24412,#24413,#24414,#24415,#24416));
#5103=EDGE_LOOP('',(#24417,#24418,#24419,#24420,#24421));
#5104=EDGE_LOOP('',(#24422,#24423,#24424,#24425,#24426,#24427));
#5105=EDGE_LOOP('',(#24428,#24429,#24430,#24431,#24432));
#5106=EDGE_LOOP('',(#24433,#24434,#24435,#24436,#24437));
#5107=EDGE_LOOP('',(#24438,#24439,#24440,#24441,#24442));
#5108=EDGE_LOOP('',(#24443,#24444,#24445,#24446,#24447));
#5109=EDGE_LOOP('',(#24448,#24449,#24450,#24451));
#5110=EDGE_LOOP('',(#24452,#24453,#24454,#24455,#24456,#24457));
#5111=EDGE_LOOP('',(#24458,#24459,#24460,#24461,#24462));
#5112=EDGE_LOOP('',(#24463,#24464,#24465,#24466,#24467,#24468));
#5113=EDGE_LOOP('',(#24469,#24470,#24471,#24472,#24473,#24474,#24475,#24476,
#24477,#24478,#24479,#24480,#24481,#24482,#24483,#24484,#24485,#24486,#24487,
#24488,#24489,#24490,#24491,#24492,#24493,#24494,#24495,#24496,#24497,#24498,
#24499,#24500,#24501,#24502,#24503,#24504,#24505,#24506,#24507,#24508,#24509,
#24510,#24511,#24512));
#5114=EDGE_LOOP('',(#24513,#24514,#24515,#24516));
#5115=EDGE_LOOP('',(#24517,#24518,#24519,#24520,#24521,#24522));
#5116=EDGE_LOOP('',(#24523,#24524,#24525,#24526,#24527,#24528,#24529,#24530,
#24531,#24532,#24533,#24534,#24535,#24536,#24537,#24538,#24539,#24540,#24541,
#24542,#24543,#24544,#24545,#24546,#24547,#24548,#24549,#24550,#24551,#24552,
#24553,#24554,#24555,#24556,#24557,#24558,#24559,#24560,#24561,#24562,#24563,
#24564,#24565,#24566,#24567,#24568,#24569,#24570,#24571,#24572,#24573,#24574,
#24575,#24576,#24577,#24578));
#5117=EDGE_LOOP('',(#24579,#24580,#24581,#24582,#24583,#24584));
#5118=EDGE_LOOP('',(#24585,#24586,#24587,#24588,#24589,#24590,#24591,#24592,
#24593,#24594,#24595,#24596,#24597,#24598,#24599,#24600,#24601,#24602,#24603,
#24604,#24605,#24606,#24607,#24608,#24609,#24610,#24611,#24612,#24613,#24614,
#24615,#24616,#24617,#24618,#24619,#24620,#24621,#24622,#24623,#24624,#24625,
#24626,#24627,#24628,#24629,#24630,#24631,#24632,#24633,#24634,#24635,#24636,
#24637,#24638,#24639));
#5119=EDGE_LOOP('',(#24640,#24641,#24642,#24643,#24644,#24645,#24646));
#5120=EDGE_LOOP('',(#24647));
#5121=EDGE_LOOP('',(#24648));
#5122=EDGE_LOOP('',(#24649,#24650,#24651,#24652,#24653,#24654,#24655));
#5123=EDGE_LOOP('',(#24656));
#5124=EDGE_LOOP('',(#24657,#24658,#24659,#24660));
#5125=EDGE_LOOP('',(#24661,#24662,#24663,#24664));
#5126=EDGE_LOOP('',(#24665,#24666,#24667));
#5127=EDGE_LOOP('',(#24668,#24669,#24670,#24671,#24672,#24673,#24674,#24675,
#24676,#24677,#24678,#24679,#24680,#24681,#24682,#24683,#24684,#24685,#24686,
#24687,#24688,#24689,#24690,#24691,#24692,#24693,#24694,#24695,#24696,#24697,
#24698,#24699,#24700,#24701,#24702,#24703,#24704,#24705,#24706,#24707,#24708,
#24709,#24710,#24711,#24712,#24713,#24714,#24715,#24716,#24717,#24718,#24719,
#24720,#24721,#24722,#24723,#24724,#24725,#24726,#24727,#24728,#24729,#24730,
#24731,#24732,#24733,#24734,#24735,#24736,#24737,#24738,#24739,#24740,#24741,
#24742,#24743,#24744,#24745,#24746,#24747,#24748,#24749,#24750,#24751,#24752,
#24753,#24754,#24755,#24756,#24757,#24758,#24759,#24760,#24761,#24762,#24763,
#24764,#24765,#24766,#24767,#24768,#24769,#24770,#24771,#24772,#24773,#24774,
#24775,#24776,#24777,#24778));
#5128=EDGE_LOOP('',(#24779,#24780,#24781,#24782));
#5129=EDGE_LOOP('',(#24783,#24784,#24785,#24786));
#5130=EDGE_LOOP('',(#24787,#24788,#24789));
#5131=EDGE_LOOP('',(#24790,#24791,#24792,#24793));
#5132=EDGE_LOOP('',(#24794,#24795,#24796,#24797));
#5133=EDGE_LOOP('',(#24798,#24799,#24800));
#5134=EDGE_LOOP('',(#24801,#24802,#24803,#24804));
#5135=EDGE_LOOP('',(#24805,#24806,#24807,#24808));
#5136=EDGE_LOOP('',(#24809,#24810,#24811));
#5137=EDGE_LOOP('',(#24812,#24813,#24814,#24815));
#5138=EDGE_LOOP('',(#24816,#24817,#24818,#24819));
#5139=EDGE_LOOP('',(#24820,#24821,#24822));
#5140=EDGE_LOOP('',(#24823,#24824,#24825,#24826));
#5141=EDGE_LOOP('',(#24827,#24828,#24829,#24830));
#5142=EDGE_LOOP('',(#24831,#24832,#24833));
#5143=EDGE_LOOP('',(#24834,#24835,#24836,#24837));
#5144=EDGE_LOOP('',(#24838,#24839,#24840,#24841));
#5145=EDGE_LOOP('',(#24842,#24843,#24844));
#5146=EDGE_LOOP('',(#24845,#24846,#24847,#24848));
#5147=EDGE_LOOP('',(#24849,#24850,#24851,#24852));
#5148=EDGE_LOOP('',(#24853,#24854,#24855));
#5149=EDGE_LOOP('',(#24856,#24857,#24858,#24859));
#5150=EDGE_LOOP('',(#24860,#24861,#24862,#24863));
#5151=EDGE_LOOP('',(#24864,#24865,#24866));
#5152=EDGE_LOOP('',(#24867,#24868,#24869,#24870));
#5153=EDGE_LOOP('',(#24871,#24872,#24873,#24874));
#5154=EDGE_LOOP('',(#24875,#24876,#24877));
#5155=EDGE_LOOP('',(#24878,#24879,#24880,#24881));
#5156=EDGE_LOOP('',(#24882,#24883,#24884,#24885));
#5157=EDGE_LOOP('',(#24886,#24887,#24888));
#5158=EDGE_LOOP('',(#24889,#24890,#24891,#24892));
#5159=EDGE_LOOP('',(#24893,#24894,#24895,#24896));
#5160=EDGE_LOOP('',(#24897,#24898,#24899));
#5161=EDGE_LOOP('',(#24900,#24901,#24902,#24903));
#5162=EDGE_LOOP('',(#24904,#24905,#24906,#24907));
#5163=EDGE_LOOP('',(#24908,#24909,#24910));
#5164=EDGE_LOOP('',(#24911,#24912,#24913,#24914));
#5165=EDGE_LOOP('',(#24915,#24916,#24917,#24918));
#5166=EDGE_LOOP('',(#24919,#24920,#24921));
#5167=EDGE_LOOP('',(#24922,#24923,#24924,#24925));
#5168=EDGE_LOOP('',(#24926,#24927,#24928,#24929));
#5169=EDGE_LOOP('',(#24930,#24931,#24932));
#5170=EDGE_LOOP('',(#24933,#24934,#24935,#24936));
#5171=EDGE_LOOP('',(#24937,#24938,#24939,#24940));
#5172=EDGE_LOOP('',(#24941,#24942,#24943));
#5173=EDGE_LOOP('',(#24944,#24945,#24946,#24947));
#5174=EDGE_LOOP('',(#24948,#24949,#24950,#24951));
#5175=EDGE_LOOP('',(#24952,#24953,#24954));
#5176=EDGE_LOOP('',(#24955,#24956,#24957,#24958));
#5177=EDGE_LOOP('',(#24959,#24960,#24961,#24962));
#5178=EDGE_LOOP('',(#24963,#24964,#24965,#24966));
#5179=EDGE_LOOP('',(#24967,#24968,#24969,#24970));
#5180=EDGE_LOOP('',(#24971,#24972,#24973,#24974));
#5181=EDGE_LOOP('',(#24975,#24976,#24977));
#5182=EDGE_LOOP('',(#24978,#24979,#24980,#24981));
#5183=EDGE_LOOP('',(#24982,#24983,#24984,#24985));
#5184=EDGE_LOOP('',(#24986,#24987,#24988));
#5185=EDGE_LOOP('',(#24989,#24990,#24991,#24992));
#5186=EDGE_LOOP('',(#24993,#24994,#24995,#24996));
#5187=EDGE_LOOP('',(#24997,#24998,#24999));
#5188=EDGE_LOOP('',(#25000,#25001,#25002,#25003));
#5189=EDGE_LOOP('',(#25004,#25005,#25006,#25007));
#5190=EDGE_LOOP('',(#25008,#25009,#25010));
#5191=EDGE_LOOP('',(#25011,#25012,#25013,#25014));
#5192=EDGE_LOOP('',(#25015,#25016,#25017,#25018));
#5193=EDGE_LOOP('',(#25019,#25020,#25021));
#5194=EDGE_LOOP('',(#25022,#25023,#25024,#25025));
#5195=EDGE_LOOP('',(#25026,#25027,#25028,#25029));
#5196=EDGE_LOOP('',(#25030,#25031,#25032));
#5197=EDGE_LOOP('',(#25033,#25034,#25035,#25036));
#5198=EDGE_LOOP('',(#25037,#25038,#25039,#25040));
#5199=EDGE_LOOP('',(#25041,#25042,#25043));
#5200=EDGE_LOOP('',(#25044,#25045,#25046,#25047));
#5201=EDGE_LOOP('',(#25048,#25049,#25050,#25051));
#5202=EDGE_LOOP('',(#25052,#25053,#25054));
#5203=EDGE_LOOP('',(#25055,#25056,#25057,#25058));
#5204=EDGE_LOOP('',(#25059,#25060,#25061,#25062));
#5205=EDGE_LOOP('',(#25063,#25064,#25065));
#5206=EDGE_LOOP('',(#25066,#25067,#25068,#25069));
#5207=EDGE_LOOP('',(#25070,#25071,#25072,#25073));
#5208=EDGE_LOOP('',(#25074,#25075,#25076));
#5209=EDGE_LOOP('',(#25077,#25078,#25079,#25080));
#5210=EDGE_LOOP('',(#25081,#25082,#25083,#25084));
#5211=EDGE_LOOP('',(#25085,#25086,#25087));
#5212=EDGE_LOOP('',(#25088,#25089,#25090,#25091));
#5213=EDGE_LOOP('',(#25092,#25093,#25094,#25095));
#5214=EDGE_LOOP('',(#25096,#25097,#25098));
#5215=EDGE_LOOP('',(#25099,#25100,#25101,#25102));
#5216=EDGE_LOOP('',(#25103,#25104,#25105,#25106));
#5217=EDGE_LOOP('',(#25107,#25108,#25109));
#5218=EDGE_LOOP('',(#25110,#25111,#25112,#25113));
#5219=EDGE_LOOP('',(#25114,#25115,#25116,#25117));
#5220=EDGE_LOOP('',(#25118,#25119,#25120));
#5221=EDGE_LOOP('',(#25121,#25122,#25123,#25124));
#5222=EDGE_LOOP('',(#25125,#25126,#25127,#25128));
#5223=EDGE_LOOP('',(#25129,#25130,#25131));
#5224=EDGE_LOOP('',(#25132,#25133,#25134,#25135));
#5225=EDGE_LOOP('',(#25136,#25137,#25138,#25139));
#5226=EDGE_LOOP('',(#25140,#25141,#25142));
#5227=EDGE_LOOP('',(#25143,#25144,#25145,#25146));
#5228=EDGE_LOOP('',(#25147,#25148,#25149,#25150));
#5229=EDGE_LOOP('',(#25151,#25152,#25153));
#5230=EDGE_LOOP('',(#25154,#25155,#25156,#25157));
#5231=EDGE_LOOP('',(#25158,#25159,#25160,#25161));
#5232=EDGE_LOOP('',(#25162,#25163,#25164));
#5233=EDGE_LOOP('',(#25165,#25166,#25167,#25168,#25169,#25170,#25171,#25172,
#25173,#25174,#25175,#25176,#25177,#25178,#25179,#25180,#25181,#25182,#25183,
#25184,#25185,#25186,#25187,#25188,#25189,#25190,#25191,#25192,#25193,#25194,
#25195,#25196,#25197,#25198,#25199,#25200,#25201,#25202,#25203,#25204,#25205,
#25206,#25207,#25208,#25209,#25210,#25211,#25212,#25213,#25214,#25215,#25216,
#25217,#25218,#25219,#25220,#25221,#25222,#25223,#25224,#25225,#25226,#25227,
#25228,#25229,#25230,#25231,#25232,#25233,#25234,#25235,#25236,#25237,#25238,
#25239,#25240,#25241,#25242,#25243,#25244,#25245,#25246,#25247,#25248,#25249,
#25250,#25251,#25252,#25253,#25254,#25255,#25256,#25257,#25258,#25259,#25260,
#25261,#25262,#25263,#25264,#25265,#25266,#25267,#25268,#25269,#25270,#25271,
#25272,#25273,#25274,#25275,#25276,#25277,#25278,#25279,#25280,#25281,#25282,
#25283,#25284,#25285,#25286,#25287,#25288,#25289,#25290,#25291,#25292,#25293,
#25294,#25295,#25296,#25297,#25298,#25299,#25300,#25301,#25302,#25303,#25304,
#25305,#25306,#25307,#25308,#25309,#25310,#25311,#25312));
#5234=EDGE_LOOP('',(#25313));
#5235=EDGE_LOOP('',(#25314,#25315,#25316,#25317,#25318,#25319));
#5236=EDGE_LOOP('',(#25320,#25321));
#5237=EDGE_LOOP('',(#25322,#25323));
#5238=EDGE_LOOP('',(#25324,#25325));
#5239=EDGE_LOOP('',(#25326,#25327));
#5240=EDGE_LOOP('',(#25328,#25329));
#5241=EDGE_LOOP('',(#25330,#25331));
#5242=EDGE_LOOP('',(#25332,#25333,#25334,#25335,#25336,#25337,#25338,#25339));
#5243=EDGE_LOOP('',(#25340,#25341,#25342,#25343));
#5244=EDGE_LOOP('',(#25344,#25345,#25346,#25347));
#5245=EDGE_LOOP('',(#25348,#25349,#25350,#25351));
#5246=EDGE_LOOP('',(#25352,#25353,#25354,#25355));
#5247=EDGE_LOOP('',(#25356,#25357,#25358,#25359));
#5248=EDGE_LOOP('',(#25360,#25361,#25362,#25363));
#7545=LINE('',#66840,#10056);
#7546=LINE('',#67099,#10057);
#7547=LINE('',#67517,#10058);
#7548=LINE('',#67785,#10059);
#7549=LINE('',#68181,#10060);
#7550=LINE('',#68617,#10061);
#7551=LINE('',#69039,#10062);
#7552=LINE('',#69473,#10063);
#7553=LINE('',#69905,#10064);
#7554=LINE('',#70148,#10065);
#7555=LINE('',#70520,#10066);
#7556=LINE('',#70787,#10067);
#7557=LINE('',#71233,#10068);
#7558=LINE('',#71652,#10069);
#7559=LINE('',#72067,#10070);
#7560=LINE('',#72504,#10071);
#7561=LINE('',#72914,#10072);
#7562=LINE('',#73169,#10073);
#7563=LINE('',#73537,#10074);
#7564=LINE('',#82182,#10075);
#7565=LINE('',#82188,#10076);
#7566=LINE('',#82190,#10077);
#7567=LINE('',#82192,#10078);
#7568=LINE('',#82199,#10079);
#7569=LINE('',#82203,#10080);
#7570=LINE('',#82559,#10081);
#7571=LINE('',#82563,#10082);
#7572=LINE('',#82565,#10083);
#7573=LINE('',#82566,#10084);
#7574=LINE('',#82569,#10085);
#7575=LINE('',#82570,#10086);
#7576=LINE('',#82575,#10087);
#7577=LINE('',#82577,#10088);
#7578=LINE('',#82578,#10089);
#7579=LINE('',#82581,#10090);
#7580=LINE('',#82582,#10091);
#7581=LINE('',#82587,#10092);
#7582=LINE('',#82589,#10093);
#7583=LINE('',#82590,#10094);
#7584=LINE('',#82593,#10095);
#7585=LINE('',#82594,#10096);
#7586=LINE('',#82599,#10097);
#7587=LINE('',#82601,#10098);
#7588=LINE('',#82602,#10099);
#7589=LINE('',#82605,#10100);
#7590=LINE('',#82606,#10101);
#7591=LINE('',#82611,#10102);
#7592=LINE('',#82613,#10103);
#7593=LINE('',#82614,#10104);
#7594=LINE('',#82617,#10105);
#7595=LINE('',#82618,#10106);
#7596=LINE('',#82623,#10107);
#7597=LINE('',#82625,#10108);
#7598=LINE('',#82626,#10109);
#7599=LINE('',#82629,#10110);
#7600=LINE('',#82630,#10111);
#7601=LINE('',#82635,#10112);
#7602=LINE('',#82637,#10113);
#7603=LINE('',#82638,#10114);
#7604=LINE('',#82641,#10115);
#7605=LINE('',#82642,#10116);
#7606=LINE('',#82647,#10117);
#7607=LINE('',#82649,#10118);
#7608=LINE('',#82650,#10119);
#7609=LINE('',#82653,#10120);
#7610=LINE('',#82654,#10121);
#7611=LINE('',#82659,#10122);
#7612=LINE('',#82661,#10123);
#7613=LINE('',#82662,#10124);
#7614=LINE('',#82665,#10125);
#7615=LINE('',#82666,#10126);
#7616=LINE('',#82671,#10127);
#7617=LINE('',#82673,#10128);
#7618=LINE('',#82674,#10129);
#7619=LINE('',#82677,#10130);
#7620=LINE('',#82678,#10131);
#7621=LINE('',#82683,#10132);
#7622=LINE('',#82685,#10133);
#7623=LINE('',#82686,#10134);
#7624=LINE('',#82689,#10135);
#7625=LINE('',#82690,#10136);
#7626=LINE('',#82695,#10137);
#7627=LINE('',#82697,#10138);
#7628=LINE('',#82698,#10139);
#7629=LINE('',#82701,#10140);
#7630=LINE('',#82702,#10141);
#7631=LINE('',#82707,#10142);
#7632=LINE('',#82709,#10143);
#7633=LINE('',#82710,#10144);
#7634=LINE('',#82713,#10145);
#7635=LINE('',#82714,#10146);
#7636=LINE('',#82719,#10147);
#7637=LINE('',#82721,#10148);
#7638=LINE('',#82722,#10149);
#7639=LINE('',#82725,#10150);
#7640=LINE('',#82726,#10151);
#7641=LINE('',#82731,#10152);
#7642=LINE('',#82733,#10153);
#7643=LINE('',#82734,#10154);
#7644=LINE('',#82737,#10155);
#7645=LINE('',#82738,#10156);
#7646=LINE('',#82743,#10157);
#7647=LINE('',#82745,#10158);
#7648=LINE('',#82746,#10159);
#7649=LINE('',#82749,#10160);
#7650=LINE('',#82750,#10161);
#7651=LINE('',#82755,#10162);
#7652=LINE('',#82757,#10163);
#7653=LINE('',#82758,#10164);
#7654=LINE('',#82761,#10165);
#7655=LINE('',#82762,#10166);
#7656=LINE('',#82769,#10167);
#7657=LINE('',#82771,#10168);
#7658=LINE('',#82772,#10169);
#7659=LINE('',#82775,#10170);
#7660=LINE('',#82776,#10171);
#7661=LINE('',#82781,#10172);
#7662=LINE('',#82783,#10173);
#7663=LINE('',#82784,#10174);
#7664=LINE('',#82787,#10175);
#7665=LINE('',#82788,#10176);
#7666=LINE('',#82793,#10177);
#7667=LINE('',#82795,#10178);
#7668=LINE('',#82796,#10179);
#7669=LINE('',#82799,#10180);
#7670=LINE('',#82800,#10181);
#7671=LINE('',#82805,#10182);
#7672=LINE('',#82807,#10183);
#7673=LINE('',#82808,#10184);
#7674=LINE('',#82811,#10185);
#7675=LINE('',#82812,#10186);
#7676=LINE('',#82817,#10187);
#7677=LINE('',#82819,#10188);
#7678=LINE('',#82820,#10189);
#7679=LINE('',#82823,#10190);
#7680=LINE('',#82824,#10191);
#7681=LINE('',#82829,#10192);
#7682=LINE('',#82831,#10193);
#7683=LINE('',#82832,#10194);
#7684=LINE('',#82835,#10195);
#7685=LINE('',#82836,#10196);
#7686=LINE('',#82841,#10197);
#7687=LINE('',#82843,#10198);
#7688=LINE('',#82844,#10199);
#7689=LINE('',#82847,#10200);
#7690=LINE('',#82848,#10201);
#7691=LINE('',#82853,#10202);
#7692=LINE('',#82855,#10203);
#7693=LINE('',#82856,#10204);
#7694=LINE('',#82859,#10205);
#7695=LINE('',#82860,#10206);
#7696=LINE('',#82865,#10207);
#7697=LINE('',#82867,#10208);
#7698=LINE('',#82868,#10209);
#7699=LINE('',#82871,#10210);
#7700=LINE('',#82872,#10211);
#7701=LINE('',#82877,#10212);
#7702=LINE('',#82879,#10213);
#7703=LINE('',#82880,#10214);
#7704=LINE('',#82883,#10215);
#7705=LINE('',#82884,#10216);
#7706=LINE('',#82889,#10217);
#7707=LINE('',#82891,#10218);
#7708=LINE('',#82892,#10219);
#7709=LINE('',#82895,#10220);
#7710=LINE('',#82896,#10221);
#7711=LINE('',#82901,#10222);
#7712=LINE('',#82903,#10223);
#7713=LINE('',#82904,#10224);
#7714=LINE('',#82907,#10225);
#7715=LINE('',#82908,#10226);
#7716=LINE('',#82913,#10227);
#7717=LINE('',#82915,#10228);
#7718=LINE('',#82916,#10229);
#7719=LINE('',#82919,#10230);
#7720=LINE('',#82920,#10231);
#7721=LINE('',#82925,#10232);
#7722=LINE('',#82927,#10233);
#7723=LINE('',#82928,#10234);
#7724=LINE('',#82931,#10235);
#7725=LINE('',#82932,#10236);
#7726=LINE('',#82937,#10237);
#7727=LINE('',#82939,#10238);
#7728=LINE('',#82940,#10239);
#7729=LINE('',#82943,#10240);
#7730=LINE('',#82944,#10241);
#7731=LINE('',#82949,#10242);
#7732=LINE('',#82951,#10243);
#7733=LINE('',#82952,#10244);
#7734=LINE('',#82955,#10245);
#7735=LINE('',#82956,#10246);
#7736=LINE('',#82961,#10247);
#7737=LINE('',#82963,#10248);
#7738=LINE('',#82964,#10249);
#7739=LINE('',#82967,#10250);
#7740=LINE('',#82968,#10251);
#7741=LINE('',#82973,#10252);
#7742=LINE('',#82975,#10253);
#7743=LINE('',#82976,#10254);
#7744=LINE('',#82979,#10255);
#7745=LINE('',#82980,#10256);
#7746=LINE('',#82984,#10257);
#7747=LINE('',#82988,#10258);
#7748=LINE('',#82990,#10259);
#7749=LINE('',#82992,#10260);
#7750=LINE('',#82994,#10261);
#7751=LINE('',#82996,#10262);
#7752=LINE('',#82997,#10263);
#7753=LINE('',#83001,#10264);
#7754=LINE('',#83005,#10265);
#7755=LINE('',#83009,#10266);
#7756=LINE('',#83013,#10267);
#7757=LINE('',#83017,#10268);
#7758=LINE('',#83020,#10269);
#7759=LINE('',#83024,#10270);
#7760=LINE('',#83026,#10271);
#7761=LINE('',#83027,#10272);
#7762=LINE('',#83029,#10273);
#7763=LINE('',#83031,#10274);
#7764=LINE('',#83033,#10275);
#7765=LINE('',#83035,#10276);
#10056=VECTOR('',#35185,1.26999999999999);
#10057=VECTOR('',#35190,1.26999999999999);
#10058=VECTOR('',#35193,1.26999999999999);
#10059=VECTOR('',#35196,1.26999999999999);
#10060=VECTOR('',#35199,1.26999999999999);
#10061=VECTOR('',#35202,1.26999999999999);
#10062=VECTOR('',#35205,1.26999999999999);
#10063=VECTOR('',#35208,1.26999999999999);
#10064=VECTOR('',#35211,1.26999999999999);
#10065=VECTOR('',#35214,1.26999999999999);
#10066=VECTOR('',#35217,1.26999999999999);
#10067=VECTOR('',#35220,1.26999999999999);
#10068=VECTOR('',#35223,1.26999999999999);
#10069=VECTOR('',#35226,1.26999999999999);
#10070=VECTOR('',#35229,1.26999999999999);
#10071=VECTOR('',#35232,1.26999999999999);
#10072=VECTOR('',#35235,1.26999999999999);
#10073=VECTOR('',#35238,1.26999999999999);
#10074=VECTOR('',#35241,1.26999999999999);
#10075=VECTOR('',#35276,1.52934);
#10076=VECTOR('',#35283,10.);
#10077=VECTOR('',#35284,10.);
#10078=VECTOR('',#35285,10.);
#10079=VECTOR('',#35288,10.);
#10080=VECTOR('',#35289,10.);
#10081=VECTOR('',#35368,2.7202);
#10082=VECTOR('',#35373,10.);
#10083=VECTOR('',#35374,10.);
#10084=VECTOR('',#35375,10.);
#10085=VECTOR('',#35378,10.);
#10086=VECTOR('',#35379,10.);
#10087=VECTOR('',#35386,10.);
#10088=VECTOR('',#35387,10.);
#10089=VECTOR('',#35388,10.);
#10090=VECTOR('',#35391,10.);
#10091=VECTOR('',#35392,10.);
#10092=VECTOR('',#35399,10.);
#10093=VECTOR('',#35400,10.);
#10094=VECTOR('',#35401,10.);
#10095=VECTOR('',#35404,10.);
#10096=VECTOR('',#35405,10.);
#10097=VECTOR('',#35412,10.);
#10098=VECTOR('',#35413,10.);
#10099=VECTOR('',#35414,10.);
#10100=VECTOR('',#35417,10.);
#10101=VECTOR('',#35418,10.);
#10102=VECTOR('',#35425,10.);
#10103=VECTOR('',#35426,10.);
#10104=VECTOR('',#35427,10.);
#10105=VECTOR('',#35430,10.);
#10106=VECTOR('',#35431,10.);
#10107=VECTOR('',#35438,10.);
#10108=VECTOR('',#35439,10.);
#10109=VECTOR('',#35440,10.);
#10110=VECTOR('',#35443,10.);
#10111=VECTOR('',#35444,9.99999999999999);
#10112=VECTOR('',#35451,10.);
#10113=VECTOR('',#35452,10.);
#10114=VECTOR('',#35453,10.);
#10115=VECTOR('',#35456,10.);
#10116=VECTOR('',#35457,10.);
#10117=VECTOR('',#35464,10.);
#10118=VECTOR('',#35465,10.);
#10119=VECTOR('',#35466,10.);
#10120=VECTOR('',#35469,10.);
#10121=VECTOR('',#35470,10.);
#10122=VECTOR('',#35477,10.);
#10123=VECTOR('',#35478,10.);
#10124=VECTOR('',#35479,10.);
#10125=VECTOR('',#35482,10.);
#10126=VECTOR('',#35483,10.);
#10127=VECTOR('',#35490,10.);
#10128=VECTOR('',#35491,10.);
#10129=VECTOR('',#35492,10.);
#10130=VECTOR('',#35495,10.);
#10131=VECTOR('',#35496,10.);
#10132=VECTOR('',#35503,10.);
#10133=VECTOR('',#35504,10.);
#10134=VECTOR('',#35505,10.);
#10135=VECTOR('',#35508,10.);
#10136=VECTOR('',#35509,10.);
#10137=VECTOR('',#35516,10.);
#10138=VECTOR('',#35517,10.);
#10139=VECTOR('',#35518,10.);
#10140=VECTOR('',#35521,10.);
#10141=VECTOR('',#35522,10.);
#10142=VECTOR('',#35529,10.);
#10143=VECTOR('',#35530,10.);
#10144=VECTOR('',#35531,10.);
#10145=VECTOR('',#35534,10.);
#10146=VECTOR('',#35535,10.);
#10147=VECTOR('',#35542,10.);
#10148=VECTOR('',#35543,10.);
#10149=VECTOR('',#35544,10.);
#10150=VECTOR('',#35547,10.);
#10151=VECTOR('',#35548,10.);
#10152=VECTOR('',#35555,10.);
#10153=VECTOR('',#35556,10.);
#10154=VECTOR('',#35557,10.);
#10155=VECTOR('',#35560,10.);
#10156=VECTOR('',#35561,10.);
#10157=VECTOR('',#35568,10.);
#10158=VECTOR('',#35569,10.);
#10159=VECTOR('',#35570,10.);
#10160=VECTOR('',#35573,10.);
#10161=VECTOR('',#35574,10.);
#10162=VECTOR('',#35581,10.);
#10163=VECTOR('',#35582,10.);
#10164=VECTOR('',#35583,10.);
#10165=VECTOR('',#35586,10.);
#10166=VECTOR('',#35587,10.);
#10167=VECTOR('',#35596,10.);
#10168=VECTOR('',#35597,10.);
#10169=VECTOR('',#35598,10.);
#10170=VECTOR('',#35601,10.);
#10171=VECTOR('',#35602,10.);
#10172=VECTOR('',#35609,10.);
#10173=VECTOR('',#35610,10.);
#10174=VECTOR('',#35611,10.);
#10175=VECTOR('',#35614,10.);
#10176=VECTOR('',#35615,10.);
#10177=VECTOR('',#35622,10.);
#10178=VECTOR('',#35623,10.);
#10179=VECTOR('',#35624,10.);
#10180=VECTOR('',#35627,10.);
#10181=VECTOR('',#35628,10.);
#10182=VECTOR('',#35635,10.);
#10183=VECTOR('',#35636,10.);
#10184=VECTOR('',#35637,10.);
#10185=VECTOR('',#35640,10.);
#10186=VECTOR('',#35641,10.);
#10187=VECTOR('',#35648,10.);
#10188=VECTOR('',#35649,10.);
#10189=VECTOR('',#35650,10.);
#10190=VECTOR('',#35653,10.);
#10191=VECTOR('',#35654,10.);
#10192=VECTOR('',#35661,10.);
#10193=VECTOR('',#35662,10.);
#10194=VECTOR('',#35663,10.);
#10195=VECTOR('',#35666,10.);
#10196=VECTOR('',#35667,10.);
#10197=VECTOR('',#35674,10.);
#10198=VECTOR('',#35675,10.);
#10199=VECTOR('',#35676,10.);
#10200=VECTOR('',#35679,10.);
#10201=VECTOR('',#35680,10.);
#10202=VECTOR('',#35687,10.);
#10203=VECTOR('',#35688,10.);
#10204=VECTOR('',#35689,10.);
#10205=VECTOR('',#35692,10.);
#10206=VECTOR('',#35693,10.);
#10207=VECTOR('',#35700,10.);
#10208=VECTOR('',#35701,10.);
#10209=VECTOR('',#35702,10.);
#10210=VECTOR('',#35705,10.);
#10211=VECTOR('',#35706,10.);
#10212=VECTOR('',#35713,10.);
#10213=VECTOR('',#35714,10.);
#10214=VECTOR('',#35715,10.);
#10215=VECTOR('',#35718,10.);
#10216=VECTOR('',#35719,10.);
#10217=VECTOR('',#35726,10.);
#10218=VECTOR('',#35727,10.);
#10219=VECTOR('',#35728,10.);
#10220=VECTOR('',#35731,10.);
#10221=VECTOR('',#35732,10.);
#10222=VECTOR('',#35739,10.);
#10223=VECTOR('',#35740,10.);
#10224=VECTOR('',#35741,10.);
#10225=VECTOR('',#35744,10.);
#10226=VECTOR('',#35745,10.);
#10227=VECTOR('',#35752,10.);
#10228=VECTOR('',#35753,10.);
#10229=VECTOR('',#35754,10.);
#10230=VECTOR('',#35757,10.);
#10231=VECTOR('',#35758,10.);
#10232=VECTOR('',#35765,10.);
#10233=VECTOR('',#35766,10.);
#10234=VECTOR('',#35767,10.);
#10235=VECTOR('',#35770,10.);
#10236=VECTOR('',#35771,10.);
#10237=VECTOR('',#35778,10.);
#10238=VECTOR('',#35779,10.);
#10239=VECTOR('',#35780,10.);
#10240=VECTOR('',#35783,10.);
#10241=VECTOR('',#35784,10.);
#10242=VECTOR('',#35791,10.);
#10243=VECTOR('',#35792,10.);
#10244=VECTOR('',#35793,10.);
#10245=VECTOR('',#35796,10.);
#10246=VECTOR('',#35797,10.);
#10247=VECTOR('',#35804,10.);
#10248=VECTOR('',#35805,10.);
#10249=VECTOR('',#35806,10.);
#10250=VECTOR('',#35809,10.);
#10251=VECTOR('',#35810,10.);
#10252=VECTOR('',#35817,10.);
#10253=VECTOR('',#35818,10.);
#10254=VECTOR('',#35819,10.);
#10255=VECTOR('',#35822,10.);
#10256=VECTOR('',#35823,10.);
#10257=VECTOR('',#35830,2.8702);
#10258=VECTOR('',#35833,10.);
#10259=VECTOR('',#35834,10.);
#10260=VECTOR('',#35835,10.);
#10261=VECTOR('',#35836,10.);
#10262=VECTOR('',#35837,10.);
#10263=VECTOR('',#35838,10.);
#10264=VECTOR('',#35841,10.);
#10265=VECTOR('',#35846,10.);
#10266=VECTOR('',#35851,10.);
#10267=VECTOR('',#35856,10.);
#10268=VECTOR('',#35861,10.);
#10269=VECTOR('',#35866,10.);
#10270=VECTOR('',#35871,1.60395121659244);
#10271=VECTOR('',#35874,10.);
#10272=VECTOR('',#35875,10.);
#10273=VECTOR('',#35878,10.);
#10274=VECTOR('',#35881,10.);
#10275=VECTOR('',#35884,10.);
#10276=VECTOR('',#35887,10.);
#10944=CIRCLE('',#28929,1.26999999999999);
#10945=CIRCLE('',#28949,1.70434);
#10946=CIRCLE('',#28950,1.70434);
#10947=CIRCLE('',#28952,1.26999999999999);
#10948=CIRCLE('',#28954,1.70434);
#10949=CIRCLE('',#28955,1.70434);
#10950=CIRCLE('',#28957,1.70434);
#10951=CIRCLE('',#28958,1.70434);
#10952=CIRCLE('',#28960,1.85434);
#10953=CIRCLE('',#28961,0.15);
#10954=CIRCLE('',#28963,2.8702);
#10955=CIRCLE('',#28965,1.35434);
#10956=CIRCLE('',#28970,2.8702);
#10957=CIRCLE('',#28972,2.8702);
#10958=CIRCLE('',#28973,2.8702);
#10959=CIRCLE('',#28974,2.8702);
#10960=CIRCLE('',#28975,2.8702);
#10961=CIRCLE('',#28976,2.8702);
#10962=CIRCLE('',#28977,2.8702);
#10963=CIRCLE('',#28978,2.8702);
#10964=CIRCLE('',#28979,2.8702);
#10965=CIRCLE('',#28980,2.8702);
#10966=CIRCLE('',#28981,2.8702);
#10967=CIRCLE('',#28982,2.8702);
#10968=CIRCLE('',#28983,2.8702);
#10969=CIRCLE('',#28984,2.8702);
#10970=CIRCLE('',#28985,2.8702);
#10971=CIRCLE('',#28986,2.8702);
#10972=CIRCLE('',#28987,2.8702);
#10973=CIRCLE('',#28988,2.8702);
#10974=CIRCLE('',#28989,2.8702);
#10975=CIRCLE('',#28990,2.8702);
#10976=CIRCLE('',#28991,2.8702);
#10977=CIRCLE('',#28992,2.8702);
#10978=CIRCLE('',#28993,2.8702);
#10979=CIRCLE('',#28994,2.8702);
#10980=CIRCLE('',#28995,2.8702);
#10981=CIRCLE('',#28996,2.8702);
#10982=CIRCLE('',#28997,2.8702);
#10983=CIRCLE('',#28998,2.8702);
#10984=CIRCLE('',#28999,2.8702);
#10985=CIRCLE('',#29000,2.8702);
#10986=CIRCLE('',#29001,2.8702);
#10987=CIRCLE('',#29002,2.8702);
#10988=CIRCLE('',#29003,2.8702);
#10989=CIRCLE('',#29004,2.8702);
#10990=CIRCLE('',#29005,2.8702);
#10991=CIRCLE('',#29006,2.8702);
#10992=CIRCLE('',#29007,2.8702);
#10993=CIRCLE('',#29008,2.57020000000001);
#10994=CIRCLE('',#29012,2.8702);
#10995=CIRCLE('',#29016,2.8702);
#10996=CIRCLE('',#29020,2.8702);
#10997=CIRCLE('',#29024,2.8702);
#10998=CIRCLE('',#29028,2.8702);
#10999=CIRCLE('',#29032,2.8702);
#11000=CIRCLE('',#29036,2.8702);
#11001=CIRCLE('',#29040,2.8702);
#11002=CIRCLE('',#29044,2.8702);
#11003=CIRCLE('',#29048,2.8702);
#11004=CIRCLE('',#29052,2.8702);
#11005=CIRCLE('',#29056,2.8702);
#11006=CIRCLE('',#29060,2.8702);
#11007=CIRCLE('',#29064,2.8702);
#11008=CIRCLE('',#29068,2.8702);
#11009=CIRCLE('',#29072,2.8702);
#11010=CIRCLE('',#29076,2.8702);
#11011=CIRCLE('',#29077,2.8702);
#11012=CIRCLE('',#29081,2.8702);
#11013=CIRCLE('',#29085,2.8702);
#11014=CIRCLE('',#29089,2.8702);
#11015=CIRCLE('',#29093,2.8702);
#11016=CIRCLE('',#29097,2.8702);
#11017=CIRCLE('',#29101,2.8702);
#11018=CIRCLE('',#29105,2.8702);
#11019=CIRCLE('',#29109,2.8702);
#11020=CIRCLE('',#29113,2.8702);
#11021=CIRCLE('',#29117,2.8702);
#11022=CIRCLE('',#29121,2.8702);
#11023=CIRCLE('',#29125,2.8702);
#11024=CIRCLE('',#29129,2.8702);
#11025=CIRCLE('',#29133,2.8702);
#11026=CIRCLE('',#29137,2.8702);
#11027=CIRCLE('',#29141,2.8702);
#11028=CIRCLE('',#29145,2.8702);
#11029=CIRCLE('',#29149,2.8702);
#11030=CIRCLE('',#29153,1.60395121659244);
#11031=CIRCLE('',#29155,1.60395121659244);
#11032=CIRCLE('',#29157,1.60395121659244);
#11033=CIRCLE('',#29159,1.60395121659244);
#11034=CIRCLE('',#29161,1.60395121659244);
#11035=CIRCLE('',#29163,1.60395121659244);
#13280=VERTEX_POINT('',#66838);
#13281=VERTEX_POINT('',#66839);
#13282=VERTEX_POINT('',#66841);
#13283=VERTEX_POINT('',#66992);
#13284=VERTEX_POINT('',#67097);
#13285=VERTEX_POINT('',#67098);
#13286=VERTEX_POINT('',#67515);
#13287=VERTEX_POINT('',#67516);
#13288=VERTEX_POINT('',#67518);
#13289=VERTEX_POINT('',#67561);
#13290=VERTEX_POINT('',#67783);
#13291=VERTEX_POINT('',#67784);
#13292=VERTEX_POINT('',#67786);
#13293=VERTEX_POINT('',#68179);
#13294=VERTEX_POINT('',#68180);
#13295=VERTEX_POINT('',#68182);
#13296=VERTEX_POINT('',#68413);
#13297=VERTEX_POINT('',#68615);
#13298=VERTEX_POINT('',#68616);
#13299=VERTEX_POINT('',#69037);
#13300=VERTEX_POINT('',#69038);
#13301=VERTEX_POINT('',#69040);
#13302=VERTEX_POINT('',#69249);
#13303=VERTEX_POINT('',#69471);
#13304=VERTEX_POINT('',#69472);
#13305=VERTEX_POINT('',#69903);
#13306=VERTEX_POINT('',#69904);
#13307=VERTEX_POINT('',#69906);
#13308=VERTEX_POINT('',#69942);
#13309=VERTEX_POINT('',#70146);
#13310=VERTEX_POINT('',#70147);
#13311=VERTEX_POINT('',#70149);
#13312=VERTEX_POINT('',#70518);
#13313=VERTEX_POINT('',#70519);
#13314=VERTEX_POINT('',#70521);
#13315=VERTEX_POINT('',#70739);
#13316=VERTEX_POINT('',#70785);
#13317=VERTEX_POINT('',#70786);
#13318=VERTEX_POINT('',#70998);
#13319=VERTEX_POINT('',#71231);
#13320=VERTEX_POINT('',#71232);
#13321=VERTEX_POINT('',#71234);
#13322=VERTEX_POINT('',#71650);
#13323=VERTEX_POINT('',#71651);
#13324=VERTEX_POINT('',#71849);
#13325=VERTEX_POINT('',#72065);
#13326=VERTEX_POINT('',#72066);
#13327=VERTEX_POINT('',#72068);
#13328=VERTEX_POINT('',#72502);
#13329=VERTEX_POINT('',#72503);
#13330=VERTEX_POINT('',#72912);
#13331=VERTEX_POINT('',#72913);
#13332=VERTEX_POINT('',#72915);
#13333=VERTEX_POINT('',#73122);
#13334=VERTEX_POINT('',#73167);
#13335=VERTEX_POINT('',#73168);
#13336=VERTEX_POINT('',#73380);
#13337=VERTEX_POINT('',#73535);
#13338=VERTEX_POINT('',#73536);
#13339=VERTEX_POINT('',#73538);
#13340=VERTEX_POINT('',#73743);
#13341=VERTEX_POINT('',#73946);
#13342=VERTEX_POINT('',#73947);
#13343=VERTEX_POINT('',#74009);
#13344=VERTEX_POINT('',#74011);
#13345=VERTEX_POINT('',#74017);
#13346=VERTEX_POINT('',#74196);
#13347=VERTEX_POINT('',#74372);
#13348=VERTEX_POINT('',#74545);
#13349=VERTEX_POINT('',#74721);
#13350=VERTEX_POINT('',#74897);
#13351=VERTEX_POINT('',#75073);
#13352=VERTEX_POINT('',#75246);
#13353=VERTEX_POINT('',#75422);
#13354=VERTEX_POINT('',#75598);
#13355=VERTEX_POINT('',#75771);
#13356=VERTEX_POINT('',#75944);
#13357=VERTEX_POINT('',#76120);
#13358=VERTEX_POINT('',#76293);
#13359=VERTEX_POINT('',#76466);
#13360=VERTEX_POINT('',#76639);
#13361=VERTEX_POINT('',#76812);
#13362=VERTEX_POINT('',#76982);
#13363=VERTEX_POINT('',#77155);
#13364=VERTEX_POINT('',#77331);
#13365=VERTEX_POINT('',#77369);
#13366=VERTEX_POINT('',#77371);
#13367=VERTEX_POINT('',#77379);
#13368=VERTEX_POINT('',#77390);
#13369=VERTEX_POINT('',#77563);
#13370=VERTEX_POINT('',#77733);
#13371=VERTEX_POINT('',#77906);
#13372=VERTEX_POINT('',#78079);
#13373=VERTEX_POINT('',#78252);
#13374=VERTEX_POINT('',#78425);
#13375=VERTEX_POINT('',#78598);
#13376=VERTEX_POINT('',#78771);
#13377=VERTEX_POINT('',#78944);
#13378=VERTEX_POINT('',#79117);
#13379=VERTEX_POINT('',#79290);
#13380=VERTEX_POINT('',#79460);
#13381=VERTEX_POINT('',#79633);
#13382=VERTEX_POINT('',#79806);
#13383=VERTEX_POINT('',#79979);
#13384=VERTEX_POINT('',#80152);
#13385=VERTEX_POINT('',#80498);
#13386=VERTEX_POINT('',#80683);
#13387=VERTEX_POINT('',#80820);
#13388=VERTEX_POINT('',#80821);
#13389=VERTEX_POINT('',#80899);
#13390=VERTEX_POINT('',#81496);
#13391=VERTEX_POINT('',#81581);
#13392=VERTEX_POINT('',#81582);
#13393=VERTEX_POINT('',#82174);
#13394=VERTEX_POINT('',#82178);
#13395=VERTEX_POINT('',#82181);
#13396=VERTEX_POINT('',#82186);
#13397=VERTEX_POINT('',#82187);
#13398=VERTEX_POINT('',#82189);
#13399=VERTEX_POINT('',#82191);
#13400=VERTEX_POINT('',#82197);
#13401=VERTEX_POINT('',#82198);
#13402=VERTEX_POINT('',#82207);
#13403=VERTEX_POINT('',#82208);
#13404=VERTEX_POINT('',#82212);
#13405=VERTEX_POINT('',#82214);
#13406=VERTEX_POINT('',#82218);
#13407=VERTEX_POINT('',#82222);
#13408=VERTEX_POINT('',#82224);
#13409=VERTEX_POINT('',#82228);
#13410=VERTEX_POINT('',#82232);
#13411=VERTEX_POINT('',#82234);
#13412=VERTEX_POINT('',#82238);
#13413=VERTEX_POINT('',#82242);
#13414=VERTEX_POINT('',#82244);
#13415=VERTEX_POINT('',#82248);
#13416=VERTEX_POINT('',#82252);
#13417=VERTEX_POINT('',#82254);
#13418=VERTEX_POINT('',#82258);
#13419=VERTEX_POINT('',#82262);
#13420=VERTEX_POINT('',#82264);
#13421=VERTEX_POINT('',#82268);
#13422=VERTEX_POINT('',#82272);
#13423=VERTEX_POINT('',#82274);
#13424=VERTEX_POINT('',#82278);
#13425=VERTEX_POINT('',#82282);
#13426=VERTEX_POINT('',#82284);
#13427=VERTEX_POINT('',#82288);
#13428=VERTEX_POINT('',#82292);
#13429=VERTEX_POINT('',#82294);
#13430=VERTEX_POINT('',#82298);
#13431=VERTEX_POINT('',#82302);
#13432=VERTEX_POINT('',#82304);
#13433=VERTEX_POINT('',#82308);
#13434=VERTEX_POINT('',#82312);
#13435=VERTEX_POINT('',#82314);
#13436=VERTEX_POINT('',#82318);
#13437=VERTEX_POINT('',#82322);
#13438=VERTEX_POINT('',#82324);
#13439=VERTEX_POINT('',#82328);
#13440=VERTEX_POINT('',#82332);
#13441=VERTEX_POINT('',#82334);
#13442=VERTEX_POINT('',#82338);
#13443=VERTEX_POINT('',#82342);
#13444=VERTEX_POINT('',#82344);
#13445=VERTEX_POINT('',#82348);
#13446=VERTEX_POINT('',#82352);
#13447=VERTEX_POINT('',#82354);
#13448=VERTEX_POINT('',#82358);
#13449=VERTEX_POINT('',#82362);
#13450=VERTEX_POINT('',#82364);
#13451=VERTEX_POINT('',#82368);
#13452=VERTEX_POINT('',#82372);
#13453=VERTEX_POINT('',#82374);
#13454=VERTEX_POINT('',#82378);
#13455=VERTEX_POINT('',#82382);
#13456=VERTEX_POINT('',#82384);
#13457=VERTEX_POINT('',#82388);
#13458=VERTEX_POINT('',#82393);
#13459=VERTEX_POINT('',#82395);
#13460=VERTEX_POINT('',#82399);
#13461=VERTEX_POINT('',#82403);
#13462=VERTEX_POINT('',#82405);
#13463=VERTEX_POINT('',#82409);
#13464=VERTEX_POINT('',#82413);
#13465=VERTEX_POINT('',#82415);
#13466=VERTEX_POINT('',#82419);
#13467=VERTEX_POINT('',#82423);
#13468=VERTEX_POINT('',#82425);
#13469=VERTEX_POINT('',#82429);
#13470=VERTEX_POINT('',#82433);
#13471=VERTEX_POINT('',#82435);
#13472=VERTEX_POINT('',#82439);
#13473=VERTEX_POINT('',#82443);
#13474=VERTEX_POINT('',#82445);
#13475=VERTEX_POINT('',#82449);
#13476=VERTEX_POINT('',#82453);
#13477=VERTEX_POINT('',#82455);
#13478=VERTEX_POINT('',#82459);
#13479=VERTEX_POINT('',#82463);
#13480=VERTEX_POINT('',#82465);
#13481=VERTEX_POINT('',#82469);
#13482=VERTEX_POINT('',#82473);
#13483=VERTEX_POINT('',#82475);
#13484=VERTEX_POINT('',#82479);
#13485=VERTEX_POINT('',#82483);
#13486=VERTEX_POINT('',#82485);
#13487=VERTEX_POINT('',#82489);
#13488=VERTEX_POINT('',#82493);
#13489=VERTEX_POINT('',#82495);
#13490=VERTEX_POINT('',#82499);
#13491=VERTEX_POINT('',#82503);
#13492=VERTEX_POINT('',#82505);
#13493=VERTEX_POINT('',#82509);
#13494=VERTEX_POINT('',#82513);
#13495=VERTEX_POINT('',#82515);
#13496=VERTEX_POINT('',#82519);
#13497=VERTEX_POINT('',#82523);
#13498=VERTEX_POINT('',#82525);
#13499=VERTEX_POINT('',#82529);
#13500=VERTEX_POINT('',#82533);
#13501=VERTEX_POINT('',#82535);
#13502=VERTEX_POINT('',#82539);
#13503=VERTEX_POINT('',#82543);
#13504=VERTEX_POINT('',#82545);
#13505=VERTEX_POINT('',#82549);
#13506=VERTEX_POINT('',#82553);
#13507=VERTEX_POINT('',#82558);
#13508=VERTEX_POINT('',#82562);
#13509=VERTEX_POINT('',#82564);
#13510=VERTEX_POINT('',#82568);
#13511=VERTEX_POINT('',#82574);
#13512=VERTEX_POINT('',#82576);
#13513=VERTEX_POINT('',#82580);
#13514=VERTEX_POINT('',#82586);
#13515=VERTEX_POINT('',#82588);
#13516=VERTEX_POINT('',#82592);
#13517=VERTEX_POINT('',#82598);
#13518=VERTEX_POINT('',#82600);
#13519=VERTEX_POINT('',#82604);
#13520=VERTEX_POINT('',#82610);
#13521=VERTEX_POINT('',#82612);
#13522=VERTEX_POINT('',#82616);
#13523=VERTEX_POINT('',#82622);
#13524=VERTEX_POINT('',#82624);
#13525=VERTEX_POINT('',#82628);
#13526=VERTEX_POINT('',#82634);
#13527=VERTEX_POINT('',#82636);
#13528=VERTEX_POINT('',#82640);
#13529=VERTEX_POINT('',#82646);
#13530=VERTEX_POINT('',#82648);
#13531=VERTEX_POINT('',#82652);
#13532=VERTEX_POINT('',#82658);
#13533=VERTEX_POINT('',#82660);
#13534=VERTEX_POINT('',#82664);
#13535=VERTEX_POINT('',#82670);
#13536=VERTEX_POINT('',#82672);
#13537=VERTEX_POINT('',#82676);
#13538=VERTEX_POINT('',#82682);
#13539=VERTEX_POINT('',#82684);
#13540=VERTEX_POINT('',#82688);
#13541=VERTEX_POINT('',#82694);
#13542=VERTEX_POINT('',#82696);
#13543=VERTEX_POINT('',#82700);
#13544=VERTEX_POINT('',#82706);
#13545=VERTEX_POINT('',#82708);
#13546=VERTEX_POINT('',#82712);
#13547=VERTEX_POINT('',#82718);
#13548=VERTEX_POINT('',#82720);
#13549=VERTEX_POINT('',#82724);
#13550=VERTEX_POINT('',#82730);
#13551=VERTEX_POINT('',#82732);
#13552=VERTEX_POINT('',#82736);
#13553=VERTEX_POINT('',#82742);
#13554=VERTEX_POINT('',#82744);
#13555=VERTEX_POINT('',#82748);
#13556=VERTEX_POINT('',#82754);
#13557=VERTEX_POINT('',#82756);
#13558=VERTEX_POINT('',#82760);
#13559=VERTEX_POINT('',#82764);
#13560=VERTEX_POINT('',#82768);
#13561=VERTEX_POINT('',#82770);
#13562=VERTEX_POINT('',#82774);
#13563=VERTEX_POINT('',#82780);
#13564=VERTEX_POINT('',#82782);
#13565=VERTEX_POINT('',#82786);
#13566=VERTEX_POINT('',#82792);
#13567=VERTEX_POINT('',#82794);
#13568=VERTEX_POINT('',#82798);
#13569=VERTEX_POINT('',#82804);
#13570=VERTEX_POINT('',#82806);
#13571=VERTEX_POINT('',#82810);
#13572=VERTEX_POINT('',#82816);
#13573=VERTEX_POINT('',#82818);
#13574=VERTEX_POINT('',#82822);
#13575=VERTEX_POINT('',#82828);
#13576=VERTEX_POINT('',#82830);
#13577=VERTEX_POINT('',#82834);
#13578=VERTEX_POINT('',#82840);
#13579=VERTEX_POINT('',#82842);
#13580=VERTEX_POINT('',#82846);
#13581=VERTEX_POINT('',#82852);
#13582=VERTEX_POINT('',#82854);
#13583=VERTEX_POINT('',#82858);
#13584=VERTEX_POINT('',#82864);
#13585=VERTEX_POINT('',#82866);
#13586=VERTEX_POINT('',#82870);
#13587=VERTEX_POINT('',#82876);
#13588=VERTEX_POINT('',#82878);
#13589=VERTEX_POINT('',#82882);
#13590=VERTEX_POINT('',#82888);
#13591=VERTEX_POINT('',#82890);
#13592=VERTEX_POINT('',#82894);
#13593=VERTEX_POINT('',#82900);
#13594=VERTEX_POINT('',#82902);
#13595=VERTEX_POINT('',#82906);
#13596=VERTEX_POINT('',#82912);
#13597=VERTEX_POINT('',#82914);
#13598=VERTEX_POINT('',#82918);
#13599=VERTEX_POINT('',#82924);
#13600=VERTEX_POINT('',#82926);
#13601=VERTEX_POINT('',#82930);
#13602=VERTEX_POINT('',#82936);
#13603=VERTEX_POINT('',#82938);
#13604=VERTEX_POINT('',#82942);
#13605=VERTEX_POINT('',#82948);
#13606=VERTEX_POINT('',#82950);
#13607=VERTEX_POINT('',#82954);
#13608=VERTEX_POINT('',#82960);
#13609=VERTEX_POINT('',#82962);
#13610=VERTEX_POINT('',#82966);
#13611=VERTEX_POINT('',#82972);
#13612=VERTEX_POINT('',#82974);
#13613=VERTEX_POINT('',#82978);
#13614=VERTEX_POINT('',#82986);
#13615=VERTEX_POINT('',#82987);
#13616=VERTEX_POINT('',#82989);
#13617=VERTEX_POINT('',#82991);
#13618=VERTEX_POINT('',#82993);
#13619=VERTEX_POINT('',#82995);
#13620=VERTEX_POINT('',#82999);
#13621=VERTEX_POINT('',#83000);
#13622=VERTEX_POINT('',#83004);
#13623=VERTEX_POINT('',#83008);
#13624=VERTEX_POINT('',#83012);
#13625=VERTEX_POINT('',#83016);
#13626=VERTEX_POINT('',#83023);
#17047=EDGE_CURVE('',#13280,#13281,#7545,.T.);
#17048=EDGE_CURVE('',#13282,#13280,#754,.F.);
#17049=EDGE_CURVE('',#13283,#13282,#10944,.T.);
#17050=EDGE_CURVE('',#13283,#13281,#755,.T.);
#17051=EDGE_CURVE('',#13284,#13285,#7546,.T.);
#17052=EDGE_CURVE('',#13280,#13284,#756,.F.);
#17053=EDGE_CURVE('',#13281,#13285,#757,.T.);
#17054=EDGE_CURVE('',#13286,#13287,#7547,.T.);
#17055=EDGE_CURVE('',#13288,#13286,#758,.T.);
#17056=EDGE_CURVE('',#13284,#13288,#759,.F.);
#17057=EDGE_CURVE('',#13285,#13289,#760,.T.);
#17058=EDGE_CURVE('',#13289,#13287,#761,.T.);
#17059=EDGE_CURVE('',#13290,#13291,#7548,.T.);
#17060=EDGE_CURVE('',#13292,#13290,#762,.T.);
#17061=EDGE_CURVE('',#13286,#13292,#763,.T.);
#17062=EDGE_CURVE('',#13287,#13291,#764,.T.);
#17063=EDGE_CURVE('',#13293,#13294,#7549,.T.);
#17064=EDGE_CURVE('',#13295,#13293,#765,.F.);
#17065=EDGE_CURVE('',#13290,#13295,#766,.T.);
#17066=EDGE_CURVE('',#13291,#13296,#767,.T.);
#17067=EDGE_CURVE('',#13296,#13294,#768,.T.);
#17068=EDGE_CURVE('',#13297,#13298,#7550,.T.);
#17069=EDGE_CURVE('',#13293,#13297,#769,.F.);
#17070=EDGE_CURVE('',#13294,#13298,#770,.T.);
#17071=EDGE_CURVE('',#13299,#13300,#7551,.T.);
#17072=EDGE_CURVE('',#13301,#13299,#771,.F.);
#17073=EDGE_CURVE('',#13297,#13301,#772,.F.);
#17074=EDGE_CURVE('',#13298,#13302,#773,.T.);
#17075=EDGE_CURVE('',#13302,#13300,#774,.T.);
#17076=EDGE_CURVE('',#13303,#13304,#7552,.T.);
#17077=EDGE_CURVE('',#13299,#13303,#775,.F.);
#17078=EDGE_CURVE('',#13300,#13304,#776,.T.);
#17079=EDGE_CURVE('',#13305,#13306,#7553,.T.);
#17080=EDGE_CURVE('',#13307,#13305,#777,.T.);
#17081=EDGE_CURVE('',#13303,#13307,#778,.F.);
#17082=EDGE_CURVE('',#13304,#13308,#779,.T.);
#17083=EDGE_CURVE('',#13308,#13306,#780,.T.);
#17084=EDGE_CURVE('',#13309,#13310,#7554,.T.);
#17085=EDGE_CURVE('',#13311,#13309,#781,.T.);
#17086=EDGE_CURVE('',#13305,#13311,#782,.T.);
#17087=EDGE_CURVE('',#13306,#13310,#783,.T.);
#17088=EDGE_CURVE('',#13312,#13313,#7555,.T.);
#17089=EDGE_CURVE('',#13314,#13312,#784,.F.);
#17090=EDGE_CURVE('',#13309,#13314,#785,.T.);
#17091=EDGE_CURVE('',#13310,#13315,#786,.T.);
#17092=EDGE_CURVE('',#13315,#13313,#787,.T.);
#17093=EDGE_CURVE('',#13316,#13317,#7556,.T.);
#17094=EDGE_CURVE('',#13312,#13316,#788,.F.);
#17095=EDGE_CURVE('',#13313,#13318,#789,.T.);
#17096=EDGE_CURVE('',#13318,#13317,#790,.T.);
#17097=EDGE_CURVE('',#13319,#13320,#7557,.T.);
#17098=EDGE_CURVE('',#13321,#13319,#791,.F.);
#17099=EDGE_CURVE('',#13316,#13321,#792,.F.);
#17100=EDGE_CURVE('',#13317,#13320,#793,.T.);
#17101=EDGE_CURVE('',#13322,#13323,#7558,.T.);
#17102=EDGE_CURVE('',#13319,#13322,#794,.F.);
#17103=EDGE_CURVE('',#13320,#13324,#795,.T.);
#17104=EDGE_CURVE('',#13324,#13323,#796,.T.);
#17105=EDGE_CURVE('',#13325,#13326,#7559,.T.);
#17106=EDGE_CURVE('',#13327,#13325,#797,.F.);
#17107=EDGE_CURVE('',#13322,#13327,#798,.F.);
#17108=EDGE_CURVE('',#13323,#13326,#799,.T.);
#17109=EDGE_CURVE('',#13328,#13329,#7560,.T.);
#17110=EDGE_CURVE('',#13325,#13328,#800,.F.);
#17111=EDGE_CURVE('',#13326,#13329,#801,.T.);
#17112=EDGE_CURVE('',#13330,#13331,#7561,.T.);
#17113=EDGE_CURVE('',#13332,#13330,#802,.F.);
#17114=EDGE_CURVE('',#13328,#13332,#803,.F.);
#17115=EDGE_CURVE('',#13329,#13333,#804,.T.);
#17116=EDGE_CURVE('',#13333,#13331,#805,.T.);
#17117=EDGE_CURVE('',#13334,#13335,#7562,.T.);
#17118=EDGE_CURVE('',#13330,#13334,#806,.F.);
#17119=EDGE_CURVE('',#13331,#13336,#807,.T.);
#17120=EDGE_CURVE('',#13336,#13335,#808,.T.);
#17121=EDGE_CURVE('',#13337,#13338,#7563,.T.);
#17122=EDGE_CURVE('',#13339,#13337,#809,.F.);
#17123=EDGE_CURVE('',#13334,#13339,#810,.F.);
#17124=EDGE_CURVE('',#13335,#13340,#811,.T.);
#17125=EDGE_CURVE('',#13340,#13338,#812,.F.);
#17126=EDGE_CURVE('',#13341,#13342,#813,.T.);
#17127=EDGE_CURVE('',#13343,#13342,#10945,.T.);
#17128=EDGE_CURVE('',#13343,#13344,#814,.T.);
#17129=EDGE_CURVE('',#13344,#13345,#815,.T.);
#17130=EDGE_CURVE('',#13345,#13346,#816,.T.);
#17131=EDGE_CURVE('',#13346,#13347,#817,.T.);
#17132=EDGE_CURVE('',#13347,#13348,#818,.T.);
#17133=EDGE_CURVE('',#13348,#13349,#819,.T.);
#17134=EDGE_CURVE('',#13349,#13350,#820,.T.);
#17135=EDGE_CURVE('',#13350,#13351,#821,.T.);
#17136=EDGE_CURVE('',#13351,#13352,#822,.T.);
#17137=EDGE_CURVE('',#13352,#13353,#823,.T.);
#17138=EDGE_CURVE('',#13353,#13354,#824,.T.);
#17139=EDGE_CURVE('',#13354,#13355,#825,.T.);
#17140=EDGE_CURVE('',#13355,#13356,#826,.T.);
#17141=EDGE_CURVE('',#13356,#13357,#827,.T.);
#17142=EDGE_CURVE('',#13357,#13358,#828,.T.);
#17143=EDGE_CURVE('',#13358,#13359,#829,.T.);
#17144=EDGE_CURVE('',#13359,#13360,#830,.T.);
#17145=EDGE_CURVE('',#13360,#13361,#831,.T.);
#17146=EDGE_CURVE('',#13361,#13362,#832,.T.);
#17147=EDGE_CURVE('',#13362,#13363,#833,.T.);
#17148=EDGE_CURVE('',#13363,#13364,#834,.T.);
#17149=EDGE_CURVE('',#13365,#13364,#10946,.T.);
#17150=EDGE_CURVE('',#13365,#13366,#835,.T.);
#17151=EDGE_CURVE('',#13366,#13367,#836,.T.);
#17152=EDGE_CURVE('',#13367,#13368,#837,.T.);
#17153=EDGE_CURVE('',#13368,#13369,#838,.T.);
#17154=EDGE_CURVE('',#13369,#13370,#839,.T.);
#17155=EDGE_CURVE('',#13370,#13371,#840,.T.);
#17156=EDGE_CURVE('',#13371,#13372,#841,.T.);
#17157=EDGE_CURVE('',#13372,#13373,#842,.T.);
#17158=EDGE_CURVE('',#13373,#13374,#843,.T.);
#17159=EDGE_CURVE('',#13374,#13375,#844,.T.);
#17160=EDGE_CURVE('',#13375,#13376,#845,.T.);
#17161=EDGE_CURVE('',#13376,#13377,#846,.T.);
#17162=EDGE_CURVE('',#13377,#13378,#847,.T.);
#17163=EDGE_CURVE('',#13378,#13379,#848,.T.);
#17164=EDGE_CURVE('',#13379,#13380,#849,.T.);
#17165=EDGE_CURVE('',#13380,#13381,#850,.T.);
#17166=EDGE_CURVE('',#13381,#13382,#851,.T.);
#17167=EDGE_CURVE('',#13382,#13383,#852,.T.);
#17168=EDGE_CURVE('',#13383,#13384,#853,.T.);
#17169=EDGE_CURVE('',#13384,#13341,#854,.T.);
#17170=EDGE_CURVE('',#13338,#13385,#855,.F.);
#17171=EDGE_CURVE('',#13386,#13385,#10947,.T.);
#17172=EDGE_CURVE('',#13337,#13386,#856,.F.);
#17173=EDGE_CURVE('',#13387,#13388,#10948,.T.);
#17174=EDGE_CURVE('',#13387,#13386,#857,.T.);
#17175=EDGE_CURVE('',#13385,#13389,#858,.T.);
#17176=EDGE_CURVE('',#13389,#13365,#859,.T.);
#17177=EDGE_CURVE('',#13388,#13365,#10949,.T.);
#17178=EDGE_CURVE('',#13364,#13387,#860,.T.);
#17179=EDGE_CURVE('',#13390,#13343,#861,.T.);
#17180=EDGE_CURVE('',#13390,#13282,#862,.T.);
#17181=EDGE_CURVE('',#13391,#13392,#10950,.T.);
#17182=EDGE_CURVE('',#13391,#13283,#863,.T.);
#17183=EDGE_CURVE('',#13392,#13343,#10951,.T.);
#17184=EDGE_CURVE('',#13342,#13391,#864,.T.);
#17185=EDGE_CURVE('',#13393,#13393,#10952,.T.);
#17186=EDGE_CURVE('',#13393,#13392,#10953,.T.);
#17187=EDGE_CURVE('',#13394,#13394,#10954,.T.);
#17188=EDGE_CURVE('',#13388,#13395,#7564,.T.);
#17189=EDGE_CURVE('',#13395,#13395,#10955,.T.);
#17190=EDGE_CURVE('',#13396,#13397,#7565,.T.);
#17191=EDGE_CURVE('',#13396,#13398,#7566,.T.);
#17192=EDGE_CURVE('',#13399,#13398,#7567,.T.);
#17193=EDGE_CURVE('',#13397,#13399,#425,.T.);
#17194=EDGE_CURVE('',#13400,#13401,#7568,.T.);
#17195=EDGE_CURVE('',#13399,#13400,#426,.T.);
#17196=EDGE_CURVE('',#13398,#13401,#7569,.T.);
#17197=EDGE_CURVE('',#13401,#13396,#10956,.T.);
#17198=EDGE_CURVE('',#13402,#13403,#427,.T.);
#17199=EDGE_CURVE('',#13403,#13404,#10957,.T.);
#17200=EDGE_CURVE('',#13404,#13405,#428,.T.);
#17201=EDGE_CURVE('',#13405,#13406,#429,.T.);
#17202=EDGE_CURVE('',#13406,#13407,#10958,.T.);
#17203=EDGE_CURVE('',#13407,#13408,#430,.T.);
#17204=EDGE_CURVE('',#13408,#13409,#431,.T.);
#17205=EDGE_CURVE('',#13409,#13410,#10959,.T.);
#17206=EDGE_CURVE('',#13410,#13411,#432,.T.);
#17207=EDGE_CURVE('',#13411,#13412,#433,.T.);
#17208=EDGE_CURVE('',#13412,#13413,#10960,.T.);
#17209=EDGE_CURVE('',#13413,#13414,#434,.T.);
#17210=EDGE_CURVE('',#13414,#13415,#435,.T.);
#17211=EDGE_CURVE('',#13415,#13416,#10961,.T.);
#17212=EDGE_CURVE('',#13416,#13417,#436,.T.);
#17213=EDGE_CURVE('',#13417,#13418,#437,.T.);
#17214=EDGE_CURVE('',#13418,#13419,#10962,.T.);
#17215=EDGE_CURVE('',#13419,#13420,#438,.T.);
#17216=EDGE_CURVE('',#13420,#13421,#439,.T.);
#17217=EDGE_CURVE('',#13421,#13422,#10963,.T.);
#17218=EDGE_CURVE('',#13422,#13423,#440,.T.);
#17219=EDGE_CURVE('',#13423,#13424,#441,.T.);
#17220=EDGE_CURVE('',#13424,#13425,#10964,.T.);
#17221=EDGE_CURVE('',#13425,#13426,#442,.T.);
#17222=EDGE_CURVE('',#13426,#13427,#443,.T.);
#17223=EDGE_CURVE('',#13427,#13428,#10965,.T.);
#17224=EDGE_CURVE('',#13428,#13429,#444,.T.);
#17225=EDGE_CURVE('',#13429,#13430,#445,.T.);
#17226=EDGE_CURVE('',#13430,#13431,#10966,.T.);
#17227=EDGE_CURVE('',#13431,#13432,#446,.T.);
#17228=EDGE_CURVE('',#13432,#13433,#447,.T.);
#17229=EDGE_CURVE('',#13433,#13434,#10967,.T.);
#17230=EDGE_CURVE('',#13434,#13435,#448,.T.);
#17231=EDGE_CURVE('',#13435,#13436,#449,.T.);
#17232=EDGE_CURVE('',#13436,#13437,#10968,.T.);
#17233=EDGE_CURVE('',#13437,#13438,#450,.T.);
#17234=EDGE_CURVE('',#13438,#13439,#451,.T.);
#17235=EDGE_CURVE('',#13439,#13440,#10969,.T.);
#17236=EDGE_CURVE('',#13440,#13441,#452,.T.);
#17237=EDGE_CURVE('',#13441,#13442,#453,.T.);
#17238=EDGE_CURVE('',#13442,#13443,#10970,.T.);
#17239=EDGE_CURVE('',#13443,#13444,#454,.T.);
#17240=EDGE_CURVE('',#13444,#13445,#455,.T.);
#17241=EDGE_CURVE('',#13445,#13446,#10971,.T.);
#17242=EDGE_CURVE('',#13446,#13447,#456,.T.);
#17243=EDGE_CURVE('',#13447,#13448,#457,.T.);
#17244=EDGE_CURVE('',#13448,#13449,#10972,.T.);
#17245=EDGE_CURVE('',#13449,#13450,#458,.T.);
#17246=EDGE_CURVE('',#13450,#13451,#459,.T.);
#17247=EDGE_CURVE('',#13451,#13452,#10973,.T.);
#17248=EDGE_CURVE('',#13452,#13453,#460,.T.);
#17249=EDGE_CURVE('',#13453,#13454,#461,.T.);
#17250=EDGE_CURVE('',#13454,#13455,#10974,.T.);
#17251=EDGE_CURVE('',#13455,#13456,#462,.T.);
#17252=EDGE_CURVE('',#13456,#13457,#463,.T.);
#17253=EDGE_CURVE('',#13457,#13397,#10975,.T.);
#17254=EDGE_CURVE('',#13400,#13458,#10976,.T.);
#17255=EDGE_CURVE('',#13458,#13459,#464,.T.);
#17256=EDGE_CURVE('',#13459,#13460,#465,.T.);
#17257=EDGE_CURVE('',#13460,#13461,#10977,.T.);
#17258=EDGE_CURVE('',#13461,#13462,#466,.T.);
#17259=EDGE_CURVE('',#13462,#13463,#467,.T.);
#17260=EDGE_CURVE('',#13463,#13464,#10978,.T.);
#17261=EDGE_CURVE('',#13464,#13465,#468,.T.);
#17262=EDGE_CURVE('',#13465,#13466,#469,.T.);
#17263=EDGE_CURVE('',#13466,#13467,#10979,.T.);
#17264=EDGE_CURVE('',#13467,#13468,#470,.T.);
#17265=EDGE_CURVE('',#13468,#13469,#471,.T.);
#17266=EDGE_CURVE('',#13469,#13470,#10980,.T.);
#17267=EDGE_CURVE('',#13470,#13471,#472,.T.);
#17268=EDGE_CURVE('',#13471,#13472,#473,.T.);
#17269=EDGE_CURVE('',#13472,#13473,#10981,.T.);
#17270=EDGE_CURVE('',#13473,#13474,#474,.T.);
#17271=EDGE_CURVE('',#13474,#13475,#475,.T.);
#17272=EDGE_CURVE('',#13475,#13476,#10982,.T.);
#17273=EDGE_CURVE('',#13476,#13477,#476,.T.);
#17274=EDGE_CURVE('',#13477,#13478,#477,.T.);
#17275=EDGE_CURVE('',#13478,#13479,#10983,.T.);
#17276=EDGE_CURVE('',#13479,#13480,#478,.T.);
#17277=EDGE_CURVE('',#13480,#13481,#479,.T.);
#17278=EDGE_CURVE('',#13481,#13482,#10984,.T.);
#17279=EDGE_CURVE('',#13482,#13483,#480,.T.);
#17280=EDGE_CURVE('',#13483,#13484,#481,.T.);
#17281=EDGE_CURVE('',#13484,#13485,#10985,.T.);
#17282=EDGE_CURVE('',#13485,#13486,#482,.T.);
#17283=EDGE_CURVE('',#13486,#13487,#483,.T.);
#17284=EDGE_CURVE('',#13487,#13488,#10986,.T.);
#17285=EDGE_CURVE('',#13488,#13489,#484,.T.);
#17286=EDGE_CURVE('',#13489,#13490,#485,.T.);
#17287=EDGE_CURVE('',#13490,#13491,#10987,.T.);
#17288=EDGE_CURVE('',#13491,#13492,#486,.T.);
#17289=EDGE_CURVE('',#13492,#13493,#487,.T.);
#17290=EDGE_CURVE('',#13493,#13494,#10988,.T.);
#17291=EDGE_CURVE('',#13494,#13495,#488,.T.);
#17292=EDGE_CURVE('',#13495,#13496,#489,.T.);
#17293=EDGE_CURVE('',#13496,#13497,#10989,.T.);
#17294=EDGE_CURVE('',#13497,#13498,#490,.T.);
#17295=EDGE_CURVE('',#13498,#13499,#491,.T.);
#17296=EDGE_CURVE('',#13499,#13500,#10990,.T.);
#17297=EDGE_CURVE('',#13500,#13501,#492,.T.);
#17298=EDGE_CURVE('',#13501,#13502,#493,.T.);
#17299=EDGE_CURVE('',#13502,#13503,#10991,.T.);
#17300=EDGE_CURVE('',#13503,#13504,#494,.T.);
#17301=EDGE_CURVE('',#13504,#13505,#495,.T.);
#17302=EDGE_CURVE('',#13505,#13506,#10992,.T.);
#17303=EDGE_CURVE('',#13506,#13402,#496,.T.);
#17304=EDGE_CURVE('',#13402,#13507,#7570,.T.);
#17305=EDGE_CURVE('',#13507,#13507,#10993,.T.);
#17306=EDGE_CURVE('',#13508,#13458,#7571,.T.);
#17307=EDGE_CURVE('',#13508,#13509,#7572,.T.);
#17308=EDGE_CURVE('',#13459,#13509,#7573,.T.);
#17309=EDGE_CURVE('',#13460,#13510,#7574,.T.);
#17310=EDGE_CURVE('',#13509,#13510,#7575,.T.);
#17311=EDGE_CURVE('',#13510,#13508,#10994,.T.);
#17312=EDGE_CURVE('',#13511,#13461,#7576,.T.);
#17313=EDGE_CURVE('',#13511,#13512,#7577,.T.);
#17314=EDGE_CURVE('',#13462,#13512,#7578,.T.);
#17315=EDGE_CURVE('',#13463,#13513,#7579,.T.);
#17316=EDGE_CURVE('',#13512,#13513,#7580,.T.);
#17317=EDGE_CURVE('',#13513,#13511,#10995,.T.);
#17318=EDGE_CURVE('',#13514,#13464,#7581,.T.);
#17319=EDGE_CURVE('',#13514,#13515,#7582,.T.);
#17320=EDGE_CURVE('',#13465,#13515,#7583,.T.);
#17321=EDGE_CURVE('',#13466,#13516,#7584,.T.);
#17322=EDGE_CURVE('',#13515,#13516,#7585,.T.);
#17323=EDGE_CURVE('',#13516,#13514,#10996,.T.);
#17324=EDGE_CURVE('',#13517,#13467,#7586,.T.);
#17325=EDGE_CURVE('',#13517,#13518,#7587,.T.);
#17326=EDGE_CURVE('',#13468,#13518,#7588,.T.);
#17327=EDGE_CURVE('',#13469,#13519,#7589,.T.);
#17328=EDGE_CURVE('',#13518,#13519,#7590,.T.);
#17329=EDGE_CURVE('',#13519,#13517,#10997,.T.);
#17330=EDGE_CURVE('',#13520,#13470,#7591,.T.);
#17331=EDGE_CURVE('',#13520,#13521,#7592,.T.);
#17332=EDGE_CURVE('',#13471,#13521,#7593,.T.);
#17333=EDGE_CURVE('',#13472,#13522,#7594,.T.);
#17334=EDGE_CURVE('',#13521,#13522,#7595,.T.);
#17335=EDGE_CURVE('',#13522,#13520,#10998,.T.);
#17336=EDGE_CURVE('',#13523,#13473,#7596,.T.);
#17337=EDGE_CURVE('',#13523,#13524,#7597,.T.);
#17338=EDGE_CURVE('',#13474,#13524,#7598,.T.);
#17339=EDGE_CURVE('',#13475,#13525,#7599,.T.);
#17340=EDGE_CURVE('',#13524,#13525,#7600,.T.);
#17341=EDGE_CURVE('',#13525,#13523,#10999,.T.);
#17342=EDGE_CURVE('',#13526,#13476,#7601,.T.);
#17343=EDGE_CURVE('',#13526,#13527,#7602,.T.);
#17344=EDGE_CURVE('',#13477,#13527,#7603,.T.);
#17345=EDGE_CURVE('',#13478,#13528,#7604,.T.);
#17346=EDGE_CURVE('',#13527,#13528,#7605,.T.);
#17347=EDGE_CURVE('',#13528,#13526,#11000,.T.);
#17348=EDGE_CURVE('',#13529,#13479,#7606,.T.);
#17349=EDGE_CURVE('',#13529,#13530,#7607,.T.);
#17350=EDGE_CURVE('',#13480,#13530,#7608,.T.);
#17351=EDGE_CURVE('',#13481,#13531,#7609,.T.);
#17352=EDGE_CURVE('',#13530,#13531,#7610,.T.);
#17353=EDGE_CURVE('',#13531,#13529,#11001,.T.);
#17354=EDGE_CURVE('',#13532,#13482,#7611,.T.);
#17355=EDGE_CURVE('',#13532,#13533,#7612,.T.);
#17356=EDGE_CURVE('',#13483,#13533,#7613,.T.);
#17357=EDGE_CURVE('',#13484,#13534,#7614,.T.);
#17358=EDGE_CURVE('',#13533,#13534,#7615,.T.);
#17359=EDGE_CURVE('',#13534,#13532,#11002,.T.);
#17360=EDGE_CURVE('',#13535,#13485,#7616,.T.);
#17361=EDGE_CURVE('',#13535,#13536,#7617,.T.);
#17362=EDGE_CURVE('',#13486,#13536,#7618,.T.);
#17363=EDGE_CURVE('',#13487,#13537,#7619,.T.);
#17364=EDGE_CURVE('',#13536,#13537,#7620,.T.);
#17365=EDGE_CURVE('',#13537,#13535,#11003,.T.);
#17366=EDGE_CURVE('',#13538,#13488,#7621,.T.);
#17367=EDGE_CURVE('',#13538,#13539,#7622,.T.);
#17368=EDGE_CURVE('',#13489,#13539,#7623,.T.);
#17369=EDGE_CURVE('',#13490,#13540,#7624,.T.);
#17370=EDGE_CURVE('',#13539,#13540,#7625,.T.);
#17371=EDGE_CURVE('',#13540,#13538,#11004,.T.);
#17372=EDGE_CURVE('',#13541,#13491,#7626,.T.);
#17373=EDGE_CURVE('',#13541,#13542,#7627,.T.);
#17374=EDGE_CURVE('',#13492,#13542,#7628,.T.);
#17375=EDGE_CURVE('',#13493,#13543,#7629,.T.);
#17376=EDGE_CURVE('',#13542,#13543,#7630,.T.);
#17377=EDGE_CURVE('',#13543,#13541,#11005,.T.);
#17378=EDGE_CURVE('',#13544,#13494,#7631,.T.);
#17379=EDGE_CURVE('',#13544,#13545,#7632,.T.);
#17380=EDGE_CURVE('',#13495,#13545,#7633,.T.);
#17381=EDGE_CURVE('',#13496,#13546,#7634,.T.);
#17382=EDGE_CURVE('',#13545,#13546,#7635,.T.);
#17383=EDGE_CURVE('',#13546,#13544,#11006,.T.);
#17384=EDGE_CURVE('',#13547,#13497,#7636,.T.);
#17385=EDGE_CURVE('',#13547,#13548,#7637,.T.);
#17386=EDGE_CURVE('',#13498,#13548,#7638,.T.);
#17387=EDGE_CURVE('',#13499,#13549,#7639,.T.);
#17388=EDGE_CURVE('',#13548,#13549,#7640,.T.);
#17389=EDGE_CURVE('',#13549,#13547,#11007,.T.);
#17390=EDGE_CURVE('',#13550,#13500,#7641,.T.);
#17391=EDGE_CURVE('',#13550,#13551,#7642,.T.);
#17392=EDGE_CURVE('',#13501,#13551,#7643,.T.);
#17393=EDGE_CURVE('',#13502,#13552,#7644,.T.);
#17394=EDGE_CURVE('',#13551,#13552,#7645,.T.);
#17395=EDGE_CURVE('',#13552,#13550,#11008,.T.);
#17396=EDGE_CURVE('',#13553,#13503,#7646,.T.);
#17397=EDGE_CURVE('',#13553,#13554,#7647,.T.);
#17398=EDGE_CURVE('',#13504,#13554,#7648,.T.);
#17399=EDGE_CURVE('',#13505,#13555,#7649,.T.);
#17400=EDGE_CURVE('',#13554,#13555,#7650,.T.);
#17401=EDGE_CURVE('',#13555,#13553,#11009,.T.);
#17402=EDGE_CURVE('',#13556,#13506,#7651,.T.);
#17403=EDGE_CURVE('',#13556,#13557,#7652,.T.);
#17404=EDGE_CURVE('',#13402,#13557,#7653,.T.);
#17405=EDGE_CURVE('',#13403,#13558,#7654,.T.);
#17406=EDGE_CURVE('',#13557,#13558,#7655,.T.);
#17407=EDGE_CURVE('',#13558,#13559,#11010,.T.);
#17408=EDGE_CURVE('',#13559,#13556,#11011,.T.);
#17409=EDGE_CURVE('',#13560,#13404,#7656,.T.);
#17410=EDGE_CURVE('',#13560,#13561,#7657,.T.);
#17411=EDGE_CURVE('',#13405,#13561,#7658,.T.);
#17412=EDGE_CURVE('',#13406,#13562,#7659,.T.);
#17413=EDGE_CURVE('',#13561,#13562,#7660,.T.);
#17414=EDGE_CURVE('',#13562,#13560,#11012,.T.);
#17415=EDGE_CURVE('',#13563,#13407,#7661,.T.);
#17416=EDGE_CURVE('',#13563,#13564,#7662,.T.);
#17417=EDGE_CURVE('',#13408,#13564,#7663,.T.);
#17418=EDGE_CURVE('',#13409,#13565,#7664,.T.);
#17419=EDGE_CURVE('',#13564,#13565,#7665,.T.);
#17420=EDGE_CURVE('',#13565,#13563,#11013,.T.);
#17421=EDGE_CURVE('',#13566,#13410,#7666,.T.);
#17422=EDGE_CURVE('',#13566,#13567,#7667,.T.);
#17423=EDGE_CURVE('',#13411,#13567,#7668,.T.);
#17424=EDGE_CURVE('',#13412,#13568,#7669,.T.);
#17425=EDGE_CURVE('',#13567,#13568,#7670,.T.);
#17426=EDGE_CURVE('',#13568,#13566,#11014,.T.);
#17427=EDGE_CURVE('',#13569,#13413,#7671,.T.);
#17428=EDGE_CURVE('',#13569,#13570,#7672,.T.);
#17429=EDGE_CURVE('',#13414,#13570,#7673,.T.);
#17430=EDGE_CURVE('',#13415,#13571,#7674,.T.);
#17431=EDGE_CURVE('',#13570,#13571,#7675,.T.);
#17432=EDGE_CURVE('',#13571,#13569,#11015,.T.);
#17433=EDGE_CURVE('',#13572,#13416,#7676,.T.);
#17434=EDGE_CURVE('',#13572,#13573,#7677,.T.);
#17435=EDGE_CURVE('',#13417,#13573,#7678,.T.);
#17436=EDGE_CURVE('',#13418,#13574,#7679,.T.);
#17437=EDGE_CURVE('',#13573,#13574,#7680,.T.);
#17438=EDGE_CURVE('',#13574,#13572,#11016,.T.);
#17439=EDGE_CURVE('',#13575,#13419,#7681,.T.);
#17440=EDGE_CURVE('',#13575,#13576,#7682,.T.);
#17441=EDGE_CURVE('',#13420,#13576,#7683,.T.);
#17442=EDGE_CURVE('',#13421,#13577,#7684,.T.);
#17443=EDGE_CURVE('',#13576,#13577,#7685,.T.);
#17444=EDGE_CURVE('',#13577,#13575,#11017,.T.);
#17445=EDGE_CURVE('',#13578,#13422,#7686,.T.);
#17446=EDGE_CURVE('',#13578,#13579,#7687,.T.);
#17447=EDGE_CURVE('',#13423,#13579,#7688,.T.);
#17448=EDGE_CURVE('',#13424,#13580,#7689,.T.);
#17449=EDGE_CURVE('',#13579,#13580,#7690,.T.);
#17450=EDGE_CURVE('',#13580,#13578,#11018,.T.);
#17451=EDGE_CURVE('',#13581,#13425,#7691,.T.);
#17452=EDGE_CURVE('',#13581,#13582,#7692,.T.);
#17453=EDGE_CURVE('',#13426,#13582,#7693,.T.);
#17454=EDGE_CURVE('',#13427,#13583,#7694,.T.);
#17455=EDGE_CURVE('',#13582,#13583,#7695,.T.);
#17456=EDGE_CURVE('',#13583,#13581,#11019,.T.);
#17457=EDGE_CURVE('',#13584,#13428,#7696,.T.);
#17458=EDGE_CURVE('',#13584,#13585,#7697,.T.);
#17459=EDGE_CURVE('',#13429,#13585,#7698,.T.);
#17460=EDGE_CURVE('',#13430,#13586,#7699,.T.);
#17461=EDGE_CURVE('',#13585,#13586,#7700,.T.);
#17462=EDGE_CURVE('',#13586,#13584,#11020,.T.);
#17463=EDGE_CURVE('',#13587,#13431,#7701,.T.);
#17464=EDGE_CURVE('',#13587,#13588,#7702,.T.);
#17465=EDGE_CURVE('',#13432,#13588,#7703,.T.);
#17466=EDGE_CURVE('',#13433,#13589,#7704,.T.);
#17467=EDGE_CURVE('',#13588,#13589,#7705,.T.);
#17468=EDGE_CURVE('',#13589,#13587,#11021,.T.);
#17469=EDGE_CURVE('',#13590,#13434,#7706,.T.);
#17470=EDGE_CURVE('',#13590,#13591,#7707,.T.);
#17471=EDGE_CURVE('',#13435,#13591,#7708,.T.);
#17472=EDGE_CURVE('',#13436,#13592,#7709,.T.);
#17473=EDGE_CURVE('',#13591,#13592,#7710,.T.);
#17474=EDGE_CURVE('',#13592,#13590,#11022,.T.);
#17475=EDGE_CURVE('',#13593,#13437,#7711,.T.);
#17476=EDGE_CURVE('',#13593,#13594,#7712,.T.);
#17477=EDGE_CURVE('',#13438,#13594,#7713,.T.);
#17478=EDGE_CURVE('',#13439,#13595,#7714,.T.);
#17479=EDGE_CURVE('',#13594,#13595,#7715,.T.);
#17480=EDGE_CURVE('',#13595,#13593,#11023,.T.);
#17481=EDGE_CURVE('',#13596,#13440,#7716,.T.);
#17482=EDGE_CURVE('',#13596,#13597,#7717,.T.);
#17483=EDGE_CURVE('',#13441,#13597,#7718,.T.);
#17484=EDGE_CURVE('',#13442,#13598,#7719,.T.);
#17485=EDGE_CURVE('',#13597,#13598,#7720,.T.);
#17486=EDGE_CURVE('',#13598,#13596,#11024,.T.);
#17487=EDGE_CURVE('',#13599,#13443,#7721,.T.);
#17488=EDGE_CURVE('',#13599,#13600,#7722,.T.);
#17489=EDGE_CURVE('',#13444,#13600,#7723,.T.);
#17490=EDGE_CURVE('',#13445,#13601,#7724,.T.);
#17491=EDGE_CURVE('',#13600,#13601,#7725,.T.);
#17492=EDGE_CURVE('',#13601,#13599,#11025,.T.);
#17493=EDGE_CURVE('',#13602,#13446,#7726,.T.);
#17494=EDGE_CURVE('',#13602,#13603,#7727,.T.);
#17495=EDGE_CURVE('',#13447,#13603,#7728,.T.);
#17496=EDGE_CURVE('',#13448,#13604,#7729,.T.);
#17497=EDGE_CURVE('',#13603,#13604,#7730,.T.);
#17498=EDGE_CURVE('',#13604,#13602,#11026,.T.);
#17499=EDGE_CURVE('',#13605,#13449,#7731,.T.);
#17500=EDGE_CURVE('',#13605,#13606,#7732,.T.);
#17501=EDGE_CURVE('',#13450,#13606,#7733,.T.);
#17502=EDGE_CURVE('',#13451,#13607,#7734,.T.);
#17503=EDGE_CURVE('',#13606,#13607,#7735,.T.);
#17504=EDGE_CURVE('',#13607,#13605,#11027,.T.);
#17505=EDGE_CURVE('',#13608,#13452,#7736,.T.);
#17506=EDGE_CURVE('',#13608,#13609,#7737,.T.);
#17507=EDGE_CURVE('',#13453,#13609,#7738,.T.);
#17508=EDGE_CURVE('',#13454,#13610,#7739,.T.);
#17509=EDGE_CURVE('',#13609,#13610,#7740,.T.);
#17510=EDGE_CURVE('',#13610,#13608,#11028,.T.);
#17511=EDGE_CURVE('',#13611,#13455,#7741,.T.);
#17512=EDGE_CURVE('',#13611,#13612,#7742,.T.);
#17513=EDGE_CURVE('',#13456,#13612,#7743,.T.);
#17514=EDGE_CURVE('',#13457,#13613,#7744,.T.);
#17515=EDGE_CURVE('',#13612,#13613,#7745,.T.);
#17516=EDGE_CURVE('',#13613,#13611,#11029,.T.);
#17517=EDGE_CURVE('',#13559,#13394,#7746,.T.);
#17518=EDGE_CURVE('',#13614,#13615,#7747,.T.);
#17519=EDGE_CURVE('',#13615,#13616,#7748,.T.);
#17520=EDGE_CURVE('',#13616,#13617,#7749,.T.);
#17521=EDGE_CURVE('',#13617,#13618,#7750,.T.);
#17522=EDGE_CURVE('',#13618,#13619,#7751,.T.);
#17523=EDGE_CURVE('',#13619,#13614,#7752,.T.);
#17524=EDGE_CURVE('',#13620,#13621,#7753,.T.);
#17525=EDGE_CURVE('',#13620,#13621,#11030,.T.);
#17526=EDGE_CURVE('',#13621,#13622,#7754,.T.);
#17527=EDGE_CURVE('',#13621,#13622,#11031,.T.);
#17528=EDGE_CURVE('',#13622,#13623,#7755,.T.);
#17529=EDGE_CURVE('',#13622,#13623,#11032,.T.);
#17530=EDGE_CURVE('',#13623,#13624,#7756,.T.);
#17531=EDGE_CURVE('',#13623,#13624,#11033,.T.);
#17532=EDGE_CURVE('',#13624,#13625,#7757,.T.);
#17533=EDGE_CURVE('',#13624,#13625,#11034,.T.);
#17534=EDGE_CURVE('',#13625,#13620,#7758,.T.);
#17535=EDGE_CURVE('',#13625,#13620,#11035,.T.);
#17536=EDGE_CURVE('',#13626,#13620,#7759,.T.);
#17537=EDGE_CURVE('',#13614,#13620,#7760,.T.);
#17538=EDGE_CURVE('',#13615,#13621,#7761,.T.);
#17539=EDGE_CURVE('',#13619,#13625,#7762,.T.);
#17540=EDGE_CURVE('',#13618,#13624,#7763,.T.);
#17541=EDGE_CURVE('',#13617,#13623,#7764,.T.);
#17542=EDGE_CURVE('',#13616,#13622,#7765,.T.);
#24372=ORIENTED_EDGE('',*,*,#17047,.F.);
#24373=ORIENTED_EDGE('',*,*,#17048,.F.);
#24374=ORIENTED_EDGE('',*,*,#17049,.F.);
#24375=ORIENTED_EDGE('',*,*,#17050,.T.);
#24376=ORIENTED_EDGE('',*,*,#17051,.F.);
#24377=ORIENTED_EDGE('',*,*,#17052,.F.);
#24378=ORIENTED_EDGE('',*,*,#17047,.T.);
#24379=ORIENTED_EDGE('',*,*,#17053,.T.);
#24380=ORIENTED_EDGE('',*,*,#17054,.F.);
#24381=ORIENTED_EDGE('',*,*,#17055,.F.);
#24382=ORIENTED_EDGE('',*,*,#17056,.F.);
#24383=ORIENTED_EDGE('',*,*,#17051,.T.);
#24384=ORIENTED_EDGE('',*,*,#17057,.T.);
#24385=ORIENTED_EDGE('',*,*,#17058,.T.);
#24386=ORIENTED_EDGE('',*,*,#17059,.F.);
#24387=ORIENTED_EDGE('',*,*,#17060,.F.);
#24388=ORIENTED_EDGE('',*,*,#17061,.F.);
#24389=ORIENTED_EDGE('',*,*,#17054,.T.);
#24390=ORIENTED_EDGE('',*,*,#17062,.T.);
#24391=ORIENTED_EDGE('',*,*,#17063,.F.);
#24392=ORIENTED_EDGE('',*,*,#17064,.F.);
#24393=ORIENTED_EDGE('',*,*,#17065,.F.);
#24394=ORIENTED_EDGE('',*,*,#17059,.T.);
#24395=ORIENTED_EDGE('',*,*,#17066,.T.);
#24396=ORIENTED_EDGE('',*,*,#17067,.T.);
#24397=ORIENTED_EDGE('',*,*,#17068,.F.);
#24398=ORIENTED_EDGE('',*,*,#17069,.F.);
#24399=ORIENTED_EDGE('',*,*,#17063,.T.);
#24400=ORIENTED_EDGE('',*,*,#17070,.T.);
#24401=ORIENTED_EDGE('',*,*,#17071,.F.);
#24402=ORIENTED_EDGE('',*,*,#17072,.F.);
#24403=ORIENTED_EDGE('',*,*,#17073,.F.);
#24404=ORIENTED_EDGE('',*,*,#17068,.T.);
#24405=ORIENTED_EDGE('',*,*,#17074,.T.);
#24406=ORIENTED_EDGE('',*,*,#17075,.T.);
#24407=ORIENTED_EDGE('',*,*,#17076,.F.);
#24408=ORIENTED_EDGE('',*,*,#17077,.F.);
#24409=ORIENTED_EDGE('',*,*,#17071,.T.);
#24410=ORIENTED_EDGE('',*,*,#17078,.T.);
#24411=ORIENTED_EDGE('',*,*,#17079,.F.);
#24412=ORIENTED_EDGE('',*,*,#17080,.F.);
#24413=ORIENTED_EDGE('',*,*,#17081,.F.);
#24414=ORIENTED_EDGE('',*,*,#17076,.T.);
#24415=ORIENTED_EDGE('',*,*,#17082,.T.);
#24416=ORIENTED_EDGE('',*,*,#17083,.T.);
#24417=ORIENTED_EDGE('',*,*,#17084,.F.);
#24418=ORIENTED_EDGE('',*,*,#17085,.F.);
#24419=ORIENTED_EDGE('',*,*,#17086,.F.);
#24420=ORIENTED_EDGE('',*,*,#17079,.T.);
#24421=ORIENTED_EDGE('',*,*,#17087,.T.);
#24422=ORIENTED_EDGE('',*,*,#17088,.F.);
#24423=ORIENTED_EDGE('',*,*,#17089,.F.);
#24424=ORIENTED_EDGE('',*,*,#17090,.F.);
#24425=ORIENTED_EDGE('',*,*,#17084,.T.);
#24426=ORIENTED_EDGE('',*,*,#17091,.T.);
#24427=ORIENTED_EDGE('',*,*,#17092,.T.);
#24428=ORIENTED_EDGE('',*,*,#17093,.F.);
#24429=ORIENTED_EDGE('',*,*,#17094,.F.);
#24430=ORIENTED_EDGE('',*,*,#17088,.T.);
#24431=ORIENTED_EDGE('',*,*,#17095,.T.);
#24432=ORIENTED_EDGE('',*,*,#17096,.T.);
#24433=ORIENTED_EDGE('',*,*,#17097,.F.);
#24434=ORIENTED_EDGE('',*,*,#17098,.F.);
#24435=ORIENTED_EDGE('',*,*,#17099,.F.);
#24436=ORIENTED_EDGE('',*,*,#17093,.T.);
#24437=ORIENTED_EDGE('',*,*,#17100,.T.);
#24438=ORIENTED_EDGE('',*,*,#17101,.F.);
#24439=ORIENTED_EDGE('',*,*,#17102,.F.);
#24440=ORIENTED_EDGE('',*,*,#17097,.T.);
#24441=ORIENTED_EDGE('',*,*,#17103,.T.);
#24442=ORIENTED_EDGE('',*,*,#17104,.T.);
#24443=ORIENTED_EDGE('',*,*,#17105,.F.);
#24444=ORIENTED_EDGE('',*,*,#17106,.F.);
#24445=ORIENTED_EDGE('',*,*,#17107,.F.);
#24446=ORIENTED_EDGE('',*,*,#17101,.T.);
#24447=ORIENTED_EDGE('',*,*,#17108,.T.);
#24448=ORIENTED_EDGE('',*,*,#17109,.F.);
#24449=ORIENTED_EDGE('',*,*,#17110,.F.);
#24450=ORIENTED_EDGE('',*,*,#17105,.T.);
#24451=ORIENTED_EDGE('',*,*,#17111,.T.);
#24452=ORIENTED_EDGE('',*,*,#17112,.F.);
#24453=ORIENTED_EDGE('',*,*,#17113,.F.);
#24454=ORIENTED_EDGE('',*,*,#17114,.F.);
#24455=ORIENTED_EDGE('',*,*,#17109,.T.);
#24456=ORIENTED_EDGE('',*,*,#17115,.T.);
#24457=ORIENTED_EDGE('',*,*,#17116,.T.);
#24458=ORIENTED_EDGE('',*,*,#17117,.F.);
#24459=ORIENTED_EDGE('',*,*,#17118,.F.);
#24460=ORIENTED_EDGE('',*,*,#17112,.T.);
#24461=ORIENTED_EDGE('',*,*,#17119,.T.);
#24462=ORIENTED_EDGE('',*,*,#17120,.T.);
#24463=ORIENTED_EDGE('',*,*,#17121,.F.);
#24464=ORIENTED_EDGE('',*,*,#17122,.F.);
#24465=ORIENTED_EDGE('',*,*,#17123,.F.);
#24466=ORIENTED_EDGE('',*,*,#17117,.T.);
#24467=ORIENTED_EDGE('',*,*,#17124,.T.);
#24468=ORIENTED_EDGE('',*,*,#17125,.T.);
#24469=ORIENTED_EDGE('',*,*,#17126,.T.);
#24470=ORIENTED_EDGE('',*,*,#17127,.F.);
#24471=ORIENTED_EDGE('',*,*,#17128,.T.);
#24472=ORIENTED_EDGE('',*,*,#17129,.T.);
#24473=ORIENTED_EDGE('',*,*,#17130,.T.);
#24474=ORIENTED_EDGE('',*,*,#17131,.T.);
#24475=ORIENTED_EDGE('',*,*,#17132,.T.);
#24476=ORIENTED_EDGE('',*,*,#17133,.T.);
#24477=ORIENTED_EDGE('',*,*,#17134,.T.);
#24478=ORIENTED_EDGE('',*,*,#17135,.T.);
#24479=ORIENTED_EDGE('',*,*,#17136,.T.);
#24480=ORIENTED_EDGE('',*,*,#17137,.T.);
#24481=ORIENTED_EDGE('',*,*,#17138,.T.);
#24482=ORIENTED_EDGE('',*,*,#17139,.T.);
#24483=ORIENTED_EDGE('',*,*,#17140,.T.);
#24484=ORIENTED_EDGE('',*,*,#17141,.T.);
#24485=ORIENTED_EDGE('',*,*,#17142,.T.);
#24486=ORIENTED_EDGE('',*,*,#17143,.T.);
#24487=ORIENTED_EDGE('',*,*,#17144,.T.);
#24488=ORIENTED_EDGE('',*,*,#17145,.T.);
#24489=ORIENTED_EDGE('',*,*,#17146,.T.);
#24490=ORIENTED_EDGE('',*,*,#17147,.T.);
#24491=ORIENTED_EDGE('',*,*,#17148,.T.);
#24492=ORIENTED_EDGE('',*,*,#17149,.F.);
#24493=ORIENTED_EDGE('',*,*,#17150,.T.);
#24494=ORIENTED_EDGE('',*,*,#17151,.T.);
#24495=ORIENTED_EDGE('',*,*,#17152,.T.);
#24496=ORIENTED_EDGE('',*,*,#17153,.T.);
#24497=ORIENTED_EDGE('',*,*,#17154,.T.);
#24498=ORIENTED_EDGE('',*,*,#17155,.T.);
#24499=ORIENTED_EDGE('',*,*,#17156,.T.);
#24500=ORIENTED_EDGE('',*,*,#17157,.T.);
#24501=ORIENTED_EDGE('',*,*,#17158,.T.);
#24502=ORIENTED_EDGE('',*,*,#17159,.T.);
#24503=ORIENTED_EDGE('',*,*,#17160,.T.);
#24504=ORIENTED_EDGE('',*,*,#17161,.T.);
#24505=ORIENTED_EDGE('',*,*,#17162,.T.);
#24506=ORIENTED_EDGE('',*,*,#17163,.T.);
#24507=ORIENTED_EDGE('',*,*,#17164,.T.);
#24508=ORIENTED_EDGE('',*,*,#17165,.T.);
#24509=ORIENTED_EDGE('',*,*,#17166,.T.);
#24510=ORIENTED_EDGE('',*,*,#17167,.T.);
#24511=ORIENTED_EDGE('',*,*,#17168,.T.);
#24512=ORIENTED_EDGE('',*,*,#17169,.T.);
#24513=ORIENTED_EDGE('',*,*,#17121,.T.);
#24514=ORIENTED_EDGE('',*,*,#17170,.T.);
#24515=ORIENTED_EDGE('',*,*,#17171,.F.);
#24516=ORIENTED_EDGE('',*,*,#17172,.F.);
#24517=ORIENTED_EDGE('',*,*,#17173,.F.);
#24518=ORIENTED_EDGE('',*,*,#17174,.T.);
#24519=ORIENTED_EDGE('',*,*,#17171,.T.);
#24520=ORIENTED_EDGE('',*,*,#17175,.T.);
#24521=ORIENTED_EDGE('',*,*,#17176,.T.);
#24522=ORIENTED_EDGE('',*,*,#17177,.F.);
#24523=ORIENTED_EDGE('',*,*,#17174,.F.);
#24524=ORIENTED_EDGE('',*,*,#17178,.F.);
#24525=ORIENTED_EDGE('',*,*,#17148,.F.);
#24526=ORIENTED_EDGE('',*,*,#17147,.F.);
#24527=ORIENTED_EDGE('',*,*,#17146,.F.);
#24528=ORIENTED_EDGE('',*,*,#17145,.F.);
#24529=ORIENTED_EDGE('',*,*,#17144,.F.);
#24530=ORIENTED_EDGE('',*,*,#17143,.F.);
#24531=ORIENTED_EDGE('',*,*,#17142,.F.);
#24532=ORIENTED_EDGE('',*,*,#17141,.F.);
#24533=ORIENTED_EDGE('',*,*,#17140,.F.);
#24534=ORIENTED_EDGE('',*,*,#17139,.F.);
#24535=ORIENTED_EDGE('',*,*,#17138,.F.);
#24536=ORIENTED_EDGE('',*,*,#17137,.F.);
#24537=ORIENTED_EDGE('',*,*,#17136,.F.);
#24538=ORIENTED_EDGE('',*,*,#17135,.F.);
#24539=ORIENTED_EDGE('',*,*,#17134,.F.);
#24540=ORIENTED_EDGE('',*,*,#17133,.F.);
#24541=ORIENTED_EDGE('',*,*,#17132,.F.);
#24542=ORIENTED_EDGE('',*,*,#17131,.F.);
#24543=ORIENTED_EDGE('',*,*,#17130,.F.);
#24544=ORIENTED_EDGE('',*,*,#17129,.F.);
#24545=ORIENTED_EDGE('',*,*,#17128,.F.);
#24546=ORIENTED_EDGE('',*,*,#17179,.F.);
#24547=ORIENTED_EDGE('',*,*,#17180,.T.);
#24548=ORIENTED_EDGE('',*,*,#17048,.T.);
#24549=ORIENTED_EDGE('',*,*,#17052,.T.);
#24550=ORIENTED_EDGE('',*,*,#17056,.T.);
#24551=ORIENTED_EDGE('',*,*,#17055,.T.);
#24552=ORIENTED_EDGE('',*,*,#17061,.T.);
#24553=ORIENTED_EDGE('',*,*,#17060,.T.);
#24554=ORIENTED_EDGE('',*,*,#17065,.T.);
#24555=ORIENTED_EDGE('',*,*,#17064,.T.);
#24556=ORIENTED_EDGE('',*,*,#17069,.T.);
#24557=ORIENTED_EDGE('',*,*,#17073,.T.);
#24558=ORIENTED_EDGE('',*,*,#17072,.T.);
#24559=ORIENTED_EDGE('',*,*,#17077,.T.);
#24560=ORIENTED_EDGE('',*,*,#17081,.T.);
#24561=ORIENTED_EDGE('',*,*,#17080,.T.);
#24562=ORIENTED_EDGE('',*,*,#17086,.T.);
#24563=ORIENTED_EDGE('',*,*,#17085,.T.);
#24564=ORIENTED_EDGE('',*,*,#17090,.T.);
#24565=ORIENTED_EDGE('',*,*,#17089,.T.);
#24566=ORIENTED_EDGE('',*,*,#17094,.T.);
#24567=ORIENTED_EDGE('',*,*,#17099,.T.);
#24568=ORIENTED_EDGE('',*,*,#17098,.T.);
#24569=ORIENTED_EDGE('',*,*,#17102,.T.);
#24570=ORIENTED_EDGE('',*,*,#17107,.T.);
#24571=ORIENTED_EDGE('',*,*,#17106,.T.);
#24572=ORIENTED_EDGE('',*,*,#17110,.T.);
#24573=ORIENTED_EDGE('',*,*,#17114,.T.);
#24574=ORIENTED_EDGE('',*,*,#17113,.T.);
#24575=ORIENTED_EDGE('',*,*,#17118,.T.);
#24576=ORIENTED_EDGE('',*,*,#17123,.T.);
#24577=ORIENTED_EDGE('',*,*,#17122,.T.);
#24578=ORIENTED_EDGE('',*,*,#17172,.T.);
#24579=ORIENTED_EDGE('',*,*,#17181,.F.);
#24580=ORIENTED_EDGE('',*,*,#17182,.T.);
#24581=ORIENTED_EDGE('',*,*,#17049,.T.);
#24582=ORIENTED_EDGE('',*,*,#17180,.F.);
#24583=ORIENTED_EDGE('',*,*,#17179,.T.);
#24584=ORIENTED_EDGE('',*,*,#17183,.F.);
#24585=ORIENTED_EDGE('',*,*,#17176,.F.);
#24586=ORIENTED_EDGE('',*,*,#17175,.F.);
#24587=ORIENTED_EDGE('',*,*,#17170,.F.);
#24588=ORIENTED_EDGE('',*,*,#17125,.F.);
#24589=ORIENTED_EDGE('',*,*,#17124,.F.);
#24590=ORIENTED_EDGE('',*,*,#17120,.F.);
#24591=ORIENTED_EDGE('',*,*,#17119,.F.);
#24592=ORIENTED_EDGE('',*,*,#17116,.F.);
#24593=ORIENTED_EDGE('',*,*,#17115,.F.);
#24594=ORIENTED_EDGE('',*,*,#17111,.F.);
#24595=ORIENTED_EDGE('',*,*,#17108,.F.);
#24596=ORIENTED_EDGE('',*,*,#17104,.F.);
#24597=ORIENTED_EDGE('',*,*,#17103,.F.);
#24598=ORIENTED_EDGE('',*,*,#17100,.F.);
#24599=ORIENTED_EDGE('',*,*,#17096,.F.);
#24600=ORIENTED_EDGE('',*,*,#17095,.F.);
#24601=ORIENTED_EDGE('',*,*,#17092,.F.);
#24602=ORIENTED_EDGE('',*,*,#17091,.F.);
#24603=ORIENTED_EDGE('',*,*,#17087,.F.);
#24604=ORIENTED_EDGE('',*,*,#17083,.F.);
#24605=ORIENTED_EDGE('',*,*,#17082,.F.);
#24606=ORIENTED_EDGE('',*,*,#17078,.F.);
#24607=ORIENTED_EDGE('',*,*,#17075,.F.);
#24608=ORIENTED_EDGE('',*,*,#17074,.F.);
#24609=ORIENTED_EDGE('',*,*,#17070,.F.);
#24610=ORIENTED_EDGE('',*,*,#17067,.F.);
#24611=ORIENTED_EDGE('',*,*,#17066,.F.);
#24612=ORIENTED_EDGE('',*,*,#17062,.F.);
#24613=ORIENTED_EDGE('',*,*,#17058,.F.);
#24614=ORIENTED_EDGE('',*,*,#17057,.F.);
#24615=ORIENTED_EDGE('',*,*,#17053,.F.);
#24616=ORIENTED_EDGE('',*,*,#17050,.F.);
#24617=ORIENTED_EDGE('',*,*,#17182,.F.);
#24618=ORIENTED_EDGE('',*,*,#17184,.F.);
#24619=ORIENTED_EDGE('',*,*,#17126,.F.);
#24620=ORIENTED_EDGE('',*,*,#17169,.F.);
#24621=ORIENTED_EDGE('',*,*,#17168,.F.);
#24622=ORIENTED_EDGE('',*,*,#17167,.F.);
#24623=ORIENTED_EDGE('',*,*,#17166,.F.);
#24624=ORIENTED_EDGE('',*,*,#17165,.F.);
#24625=ORIENTED_EDGE('',*,*,#17164,.F.);
#24626=ORIENTED_EDGE('',*,*,#17163,.F.);
#24627=ORIENTED_EDGE('',*,*,#17162,.F.);
#24628=ORIENTED_EDGE('',*,*,#17161,.F.);
#24629=ORIENTED_EDGE('',*,*,#17160,.F.);
#24630=ORIENTED_EDGE('',*,*,#17159,.F.);
#24631=ORIENTED_EDGE('',*,*,#17158,.F.);
#24632=ORIENTED_EDGE('',*,*,#17157,.F.);
#24633=ORIENTED_EDGE('',*,*,#17156,.F.);
#24634=ORIENTED_EDGE('',*,*,#17155,.F.);
#24635=ORIENTED_EDGE('',*,*,#17154,.F.);
#24636=ORIENTED_EDGE('',*,*,#17153,.F.);
#24637=ORIENTED_EDGE('',*,*,#17152,.F.);
#24638=ORIENTED_EDGE('',*,*,#17151,.F.);
#24639=ORIENTED_EDGE('',*,*,#17150,.F.);
#24640=ORIENTED_EDGE('',*,*,#17185,.T.);
#24641=ORIENTED_EDGE('',*,*,#17186,.T.);
#24642=ORIENTED_EDGE('',*,*,#17183,.T.);
#24643=ORIENTED_EDGE('',*,*,#17127,.T.);
#24644=ORIENTED_EDGE('',*,*,#17184,.T.);
#24645=ORIENTED_EDGE('',*,*,#17181,.T.);
#24646=ORIENTED_EDGE('',*,*,#17186,.F.);
#24647=ORIENTED_EDGE('',*,*,#17187,.F.);
#24648=ORIENTED_EDGE('',*,*,#17185,.F.);
#24649=ORIENTED_EDGE('',*,*,#17173,.T.);
#24650=ORIENTED_EDGE('',*,*,#17188,.T.);
#24651=ORIENTED_EDGE('',*,*,#17189,.T.);
#24652=ORIENTED_EDGE('',*,*,#17188,.F.);
#24653=ORIENTED_EDGE('',*,*,#17177,.T.);
#24654=ORIENTED_EDGE('',*,*,#17149,.T.);
#24655=ORIENTED_EDGE('',*,*,#17178,.T.);
#24656=ORIENTED_EDGE('',*,*,#17189,.F.);
#24657=ORIENTED_EDGE('',*,*,#17190,.F.);
#24658=ORIENTED_EDGE('',*,*,#17191,.T.);
#24659=ORIENTED_EDGE('',*,*,#17192,.F.);
#24660=ORIENTED_EDGE('',*,*,#17193,.F.);
#24661=ORIENTED_EDGE('',*,*,#17194,.F.);
#24662=ORIENTED_EDGE('',*,*,#17195,.F.);
#24663=ORIENTED_EDGE('',*,*,#17192,.T.);
#24664=ORIENTED_EDGE('',*,*,#17196,.T.);
#24665=ORIENTED_EDGE('',*,*,#17197,.F.);
#24666=ORIENTED_EDGE('',*,*,#17196,.F.);
#24667=ORIENTED_EDGE('',*,*,#17191,.F.);
#24668=ORIENTED_EDGE('',*,*,#17198,.T.);
#24669=ORIENTED_EDGE('',*,*,#17199,.T.);
#24670=ORIENTED_EDGE('',*,*,#17200,.T.);
#24671=ORIENTED_EDGE('',*,*,#17201,.T.);
#24672=ORIENTED_EDGE('',*,*,#17202,.T.);
#24673=ORIENTED_EDGE('',*,*,#17203,.T.);
#24674=ORIENTED_EDGE('',*,*,#17204,.T.);
#24675=ORIENTED_EDGE('',*,*,#17205,.T.);
#24676=ORIENTED_EDGE('',*,*,#17206,.T.);
#24677=ORIENTED_EDGE('',*,*,#17207,.T.);
#24678=ORIENTED_EDGE('',*,*,#17208,.T.);
#24679=ORIENTED_EDGE('',*,*,#17209,.T.);
#24680=ORIENTED_EDGE('',*,*,#17210,.T.);
#24681=ORIENTED_EDGE('',*,*,#17211,.T.);
#24682=ORIENTED_EDGE('',*,*,#17212,.T.);
#24683=ORIENTED_EDGE('',*,*,#17213,.T.);
#24684=ORIENTED_EDGE('',*,*,#17214,.T.);
#24685=ORIENTED_EDGE('',*,*,#17215,.T.);
#24686=ORIENTED_EDGE('',*,*,#17216,.T.);
#24687=ORIENTED_EDGE('',*,*,#17217,.T.);
#24688=ORIENTED_EDGE('',*,*,#17218,.T.);
#24689=ORIENTED_EDGE('',*,*,#17219,.T.);
#24690=ORIENTED_EDGE('',*,*,#17220,.T.);
#24691=ORIENTED_EDGE('',*,*,#17221,.T.);
#24692=ORIENTED_EDGE('',*,*,#17222,.T.);
#24693=ORIENTED_EDGE('',*,*,#17223,.T.);
#24694=ORIENTED_EDGE('',*,*,#17224,.T.);
#24695=ORIENTED_EDGE('',*,*,#17225,.T.);
#24696=ORIENTED_EDGE('',*,*,#17226,.T.);
#24697=ORIENTED_EDGE('',*,*,#17227,.T.);
#24698=ORIENTED_EDGE('',*,*,#17228,.T.);
#24699=ORIENTED_EDGE('',*,*,#17229,.T.);
#24700=ORIENTED_EDGE('',*,*,#17230,.T.);
#24701=ORIENTED_EDGE('',*,*,#17231,.T.);
#24702=ORIENTED_EDGE('',*,*,#17232,.T.);
#24703=ORIENTED_EDGE('',*,*,#17233,.T.);
#24704=ORIENTED_EDGE('',*,*,#17234,.T.);
#24705=ORIENTED_EDGE('',*,*,#17235,.T.);
#24706=ORIENTED_EDGE('',*,*,#17236,.T.);
#24707=ORIENTED_EDGE('',*,*,#17237,.T.);
#24708=ORIENTED_EDGE('',*,*,#17238,.T.);
#24709=ORIENTED_EDGE('',*,*,#17239,.T.);
#24710=ORIENTED_EDGE('',*,*,#17240,.T.);
#24711=ORIENTED_EDGE('',*,*,#17241,.T.);
#24712=ORIENTED_EDGE('',*,*,#17242,.T.);
#24713=ORIENTED_EDGE('',*,*,#17243,.T.);
#24714=ORIENTED_EDGE('',*,*,#17244,.T.);
#24715=ORIENTED_EDGE('',*,*,#17245,.T.);
#24716=ORIENTED_EDGE('',*,*,#17246,.T.);
#24717=ORIENTED_EDGE('',*,*,#17247,.T.);
#24718=ORIENTED_EDGE('',*,*,#17248,.T.);
#24719=ORIENTED_EDGE('',*,*,#17249,.T.);
#24720=ORIENTED_EDGE('',*,*,#17250,.T.);
#24721=ORIENTED_EDGE('',*,*,#17251,.T.);
#24722=ORIENTED_EDGE('',*,*,#17252,.T.);
#24723=ORIENTED_EDGE('',*,*,#17253,.T.);
#24724=ORIENTED_EDGE('',*,*,#17193,.T.);
#24725=ORIENTED_EDGE('',*,*,#17195,.T.);
#24726=ORIENTED_EDGE('',*,*,#17254,.T.);
#24727=ORIENTED_EDGE('',*,*,#17255,.T.);
#24728=ORIENTED_EDGE('',*,*,#17256,.T.);
#24729=ORIENTED_EDGE('',*,*,#17257,.T.);
#24730=ORIENTED_EDGE('',*,*,#17258,.T.);
#24731=ORIENTED_EDGE('',*,*,#17259,.T.);
#24732=ORIENTED_EDGE('',*,*,#17260,.T.);
#24733=ORIENTED_EDGE('',*,*,#17261,.T.);
#24734=ORIENTED_EDGE('',*,*,#17262,.T.);
#24735=ORIENTED_EDGE('',*,*,#17263,.T.);
#24736=ORIENTED_EDGE('',*,*,#17264,.T.);
#24737=ORIENTED_EDGE('',*,*,#17265,.T.);
#24738=ORIENTED_EDGE('',*,*,#17266,.T.);
#24739=ORIENTED_EDGE('',*,*,#17267,.T.);
#24740=ORIENTED_EDGE('',*,*,#17268,.T.);
#24741=ORIENTED_EDGE('',*,*,#17269,.T.);
#24742=ORIENTED_EDGE('',*,*,#17270,.T.);
#24743=ORIENTED_EDGE('',*,*,#17271,.T.);
#24744=ORIENTED_EDGE('',*,*,#17272,.T.);
#24745=ORIENTED_EDGE('',*,*,#17273,.T.);
#24746=ORIENTED_EDGE('',*,*,#17274,.T.);
#24747=ORIENTED_EDGE('',*,*,#17275,.T.);
#24748=ORIENTED_EDGE('',*,*,#17276,.T.);
#24749=ORIENTED_EDGE('',*,*,#17277,.T.);
#24750=ORIENTED_EDGE('',*,*,#17278,.T.);
#24751=ORIENTED_EDGE('',*,*,#17279,.T.);
#24752=ORIENTED_EDGE('',*,*,#17280,.T.);
#24753=ORIENTED_EDGE('',*,*,#17281,.T.);
#24754=ORIENTED_EDGE('',*,*,#17282,.T.);
#24755=ORIENTED_EDGE('',*,*,#17283,.T.);
#24756=ORIENTED_EDGE('',*,*,#17284,.T.);
#24757=ORIENTED_EDGE('',*,*,#17285,.T.);
#24758=ORIENTED_EDGE('',*,*,#17286,.T.);
#24759=ORIENTED_EDGE('',*,*,#17287,.T.);
#24760=ORIENTED_EDGE('',*,*,#17288,.T.);
#24761=ORIENTED_EDGE('',*,*,#17289,.T.);
#24762=ORIENTED_EDGE('',*,*,#17290,.T.);
#24763=ORIENTED_EDGE('',*,*,#17291,.T.);
#24764=ORIENTED_EDGE('',*,*,#17292,.T.);
#24765=ORIENTED_EDGE('',*,*,#17293,.T.);
#24766=ORIENTED_EDGE('',*,*,#17294,.T.);
#24767=ORIENTED_EDGE('',*,*,#17295,.T.);
#24768=ORIENTED_EDGE('',*,*,#17296,.T.);
#24769=ORIENTED_EDGE('',*,*,#17297,.T.);
#24770=ORIENTED_EDGE('',*,*,#17298,.T.);
#24771=ORIENTED_EDGE('',*,*,#17299,.T.);
#24772=ORIENTED_EDGE('',*,*,#17300,.T.);
#24773=ORIENTED_EDGE('',*,*,#17301,.T.);
#24774=ORIENTED_EDGE('',*,*,#17302,.T.);
#24775=ORIENTED_EDGE('',*,*,#17303,.T.);
#24776=ORIENTED_EDGE('',*,*,#17304,.T.);
#24777=ORIENTED_EDGE('',*,*,#17305,.T.);
#24778=ORIENTED_EDGE('',*,*,#17304,.F.);
#24779=ORIENTED_EDGE('',*,*,#17306,.F.);
#24780=ORIENTED_EDGE('',*,*,#17307,.T.);
#24781=ORIENTED_EDGE('',*,*,#17308,.F.);
#24782=ORIENTED_EDGE('',*,*,#17255,.F.);
#24783=ORIENTED_EDGE('',*,*,#17309,.F.);
#24784=ORIENTED_EDGE('',*,*,#17256,.F.);
#24785=ORIENTED_EDGE('',*,*,#17308,.T.);
#24786=ORIENTED_EDGE('',*,*,#17310,.T.);
#24787=ORIENTED_EDGE('',*,*,#17311,.F.);
#24788=ORIENTED_EDGE('',*,*,#17310,.F.);
#24789=ORIENTED_EDGE('',*,*,#17307,.F.);
#24790=ORIENTED_EDGE('',*,*,#17312,.F.);
#24791=ORIENTED_EDGE('',*,*,#17313,.T.);
#24792=ORIENTED_EDGE('',*,*,#17314,.F.);
#24793=ORIENTED_EDGE('',*,*,#17258,.F.);
#24794=ORIENTED_EDGE('',*,*,#17315,.F.);
#24795=ORIENTED_EDGE('',*,*,#17259,.F.);
#24796=ORIENTED_EDGE('',*,*,#17314,.T.);
#24797=ORIENTED_EDGE('',*,*,#17316,.T.);
#24798=ORIENTED_EDGE('',*,*,#17317,.F.);
#24799=ORIENTED_EDGE('',*,*,#17316,.F.);
#24800=ORIENTED_EDGE('',*,*,#17313,.F.);
#24801=ORIENTED_EDGE('',*,*,#17318,.F.);
#24802=ORIENTED_EDGE('',*,*,#17319,.T.);
#24803=ORIENTED_EDGE('',*,*,#17320,.F.);
#24804=ORIENTED_EDGE('',*,*,#17261,.F.);
#24805=ORIENTED_EDGE('',*,*,#17321,.F.);
#24806=ORIENTED_EDGE('',*,*,#17262,.F.);
#24807=ORIENTED_EDGE('',*,*,#17320,.T.);
#24808=ORIENTED_EDGE('',*,*,#17322,.T.);
#24809=ORIENTED_EDGE('',*,*,#17323,.F.);
#24810=ORIENTED_EDGE('',*,*,#17322,.F.);
#24811=ORIENTED_EDGE('',*,*,#17319,.F.);
#24812=ORIENTED_EDGE('',*,*,#17324,.F.);
#24813=ORIENTED_EDGE('',*,*,#17325,.T.);
#24814=ORIENTED_EDGE('',*,*,#17326,.F.);
#24815=ORIENTED_EDGE('',*,*,#17264,.F.);
#24816=ORIENTED_EDGE('',*,*,#17327,.F.);
#24817=ORIENTED_EDGE('',*,*,#17265,.F.);
#24818=ORIENTED_EDGE('',*,*,#17326,.T.);
#24819=ORIENTED_EDGE('',*,*,#17328,.T.);
#24820=ORIENTED_EDGE('',*,*,#17329,.F.);
#24821=ORIENTED_EDGE('',*,*,#17328,.F.);
#24822=ORIENTED_EDGE('',*,*,#17325,.F.);
#24823=ORIENTED_EDGE('',*,*,#17330,.F.);
#24824=ORIENTED_EDGE('',*,*,#17331,.T.);
#24825=ORIENTED_EDGE('',*,*,#17332,.F.);
#24826=ORIENTED_EDGE('',*,*,#17267,.F.);
#24827=ORIENTED_EDGE('',*,*,#17333,.F.);
#24828=ORIENTED_EDGE('',*,*,#17268,.F.);
#24829=ORIENTED_EDGE('',*,*,#17332,.T.);
#24830=ORIENTED_EDGE('',*,*,#17334,.T.);
#24831=ORIENTED_EDGE('',*,*,#17335,.F.);
#24832=ORIENTED_EDGE('',*,*,#17334,.F.);
#24833=ORIENTED_EDGE('',*,*,#17331,.F.);
#24834=ORIENTED_EDGE('',*,*,#17336,.F.);
#24835=ORIENTED_EDGE('',*,*,#17337,.T.);
#24836=ORIENTED_EDGE('',*,*,#17338,.F.);
#24837=ORIENTED_EDGE('',*,*,#17270,.F.);
#24838=ORIENTED_EDGE('',*,*,#17339,.F.);
#24839=ORIENTED_EDGE('',*,*,#17271,.F.);
#24840=ORIENTED_EDGE('',*,*,#17338,.T.);
#24841=ORIENTED_EDGE('',*,*,#17340,.T.);
#24842=ORIENTED_EDGE('',*,*,#17341,.F.);
#24843=ORIENTED_EDGE('',*,*,#17340,.F.);
#24844=ORIENTED_EDGE('',*,*,#17337,.F.);
#24845=ORIENTED_EDGE('',*,*,#17342,.F.);
#24846=ORIENTED_EDGE('',*,*,#17343,.T.);
#24847=ORIENTED_EDGE('',*,*,#17344,.F.);
#24848=ORIENTED_EDGE('',*,*,#17273,.F.);
#24849=ORIENTED_EDGE('',*,*,#17345,.F.);
#24850=ORIENTED_EDGE('',*,*,#17274,.F.);
#24851=ORIENTED_EDGE('',*,*,#17344,.T.);
#24852=ORIENTED_EDGE('',*,*,#17346,.T.);
#24853=ORIENTED_EDGE('',*,*,#17347,.F.);
#24854=ORIENTED_EDGE('',*,*,#17346,.F.);
#24855=ORIENTED_EDGE('',*,*,#17343,.F.);
#24856=ORIENTED_EDGE('',*,*,#17348,.F.);
#24857=ORIENTED_EDGE('',*,*,#17349,.T.);
#24858=ORIENTED_EDGE('',*,*,#17350,.F.);
#24859=ORIENTED_EDGE('',*,*,#17276,.F.);
#24860=ORIENTED_EDGE('',*,*,#17351,.F.);
#24861=ORIENTED_EDGE('',*,*,#17277,.F.);
#24862=ORIENTED_EDGE('',*,*,#17350,.T.);
#24863=ORIENTED_EDGE('',*,*,#17352,.T.);
#24864=ORIENTED_EDGE('',*,*,#17353,.F.);
#24865=ORIENTED_EDGE('',*,*,#17352,.F.);
#24866=ORIENTED_EDGE('',*,*,#17349,.F.);
#24867=ORIENTED_EDGE('',*,*,#17354,.F.);
#24868=ORIENTED_EDGE('',*,*,#17355,.T.);
#24869=ORIENTED_EDGE('',*,*,#17356,.F.);
#24870=ORIENTED_EDGE('',*,*,#17279,.F.);
#24871=ORIENTED_EDGE('',*,*,#17357,.F.);
#24872=ORIENTED_EDGE('',*,*,#17280,.F.);
#24873=ORIENTED_EDGE('',*,*,#17356,.T.);
#24874=ORIENTED_EDGE('',*,*,#17358,.T.);
#24875=ORIENTED_EDGE('',*,*,#17359,.F.);
#24876=ORIENTED_EDGE('',*,*,#17358,.F.);
#24877=ORIENTED_EDGE('',*,*,#17355,.F.);
#24878=ORIENTED_EDGE('',*,*,#17360,.F.);
#24879=ORIENTED_EDGE('',*,*,#17361,.T.);
#24880=ORIENTED_EDGE('',*,*,#17362,.F.);
#24881=ORIENTED_EDGE('',*,*,#17282,.F.);
#24882=ORIENTED_EDGE('',*,*,#17363,.F.);
#24883=ORIENTED_EDGE('',*,*,#17283,.F.);
#24884=ORIENTED_EDGE('',*,*,#17362,.T.);
#24885=ORIENTED_EDGE('',*,*,#17364,.T.);
#24886=ORIENTED_EDGE('',*,*,#17365,.F.);
#24887=ORIENTED_EDGE('',*,*,#17364,.F.);
#24888=ORIENTED_EDGE('',*,*,#17361,.F.);
#24889=ORIENTED_EDGE('',*,*,#17366,.F.);
#24890=ORIENTED_EDGE('',*,*,#17367,.T.);
#24891=ORIENTED_EDGE('',*,*,#17368,.F.);
#24892=ORIENTED_EDGE('',*,*,#17285,.F.);
#24893=ORIENTED_EDGE('',*,*,#17369,.F.);
#24894=ORIENTED_EDGE('',*,*,#17286,.F.);
#24895=ORIENTED_EDGE('',*,*,#17368,.T.);
#24896=ORIENTED_EDGE('',*,*,#17370,.T.);
#24897=ORIENTED_EDGE('',*,*,#17371,.F.);
#24898=ORIENTED_EDGE('',*,*,#17370,.F.);
#24899=ORIENTED_EDGE('',*,*,#17367,.F.);
#24900=ORIENTED_EDGE('',*,*,#17372,.F.);
#24901=ORIENTED_EDGE('',*,*,#17373,.T.);
#24902=ORIENTED_EDGE('',*,*,#17374,.F.);
#24903=ORIENTED_EDGE('',*,*,#17288,.F.);
#24904=ORIENTED_EDGE('',*,*,#17375,.F.);
#24905=ORIENTED_EDGE('',*,*,#17289,.F.);
#24906=ORIENTED_EDGE('',*,*,#17374,.T.);
#24907=ORIENTED_EDGE('',*,*,#17376,.T.);
#24908=ORIENTED_EDGE('',*,*,#17377,.F.);
#24909=ORIENTED_EDGE('',*,*,#17376,.F.);
#24910=ORIENTED_EDGE('',*,*,#17373,.F.);
#24911=ORIENTED_EDGE('',*,*,#17378,.F.);
#24912=ORIENTED_EDGE('',*,*,#17379,.T.);
#24913=ORIENTED_EDGE('',*,*,#17380,.F.);
#24914=ORIENTED_EDGE('',*,*,#17291,.F.);
#24915=ORIENTED_EDGE('',*,*,#17381,.F.);
#24916=ORIENTED_EDGE('',*,*,#17292,.F.);
#24917=ORIENTED_EDGE('',*,*,#17380,.T.);
#24918=ORIENTED_EDGE('',*,*,#17382,.T.);
#24919=ORIENTED_EDGE('',*,*,#17383,.F.);
#24920=ORIENTED_EDGE('',*,*,#17382,.F.);
#24921=ORIENTED_EDGE('',*,*,#17379,.F.);
#24922=ORIENTED_EDGE('',*,*,#17384,.F.);
#24923=ORIENTED_EDGE('',*,*,#17385,.T.);
#24924=ORIENTED_EDGE('',*,*,#17386,.F.);
#24925=ORIENTED_EDGE('',*,*,#17294,.F.);
#24926=ORIENTED_EDGE('',*,*,#17387,.F.);
#24927=ORIENTED_EDGE('',*,*,#17295,.F.);
#24928=ORIENTED_EDGE('',*,*,#17386,.T.);
#24929=ORIENTED_EDGE('',*,*,#17388,.T.);
#24930=ORIENTED_EDGE('',*,*,#17389,.F.);
#24931=ORIENTED_EDGE('',*,*,#17388,.F.);
#24932=ORIENTED_EDGE('',*,*,#17385,.F.);
#24933=ORIENTED_EDGE('',*,*,#17390,.F.);
#24934=ORIENTED_EDGE('',*,*,#17391,.T.);
#24935=ORIENTED_EDGE('',*,*,#17392,.F.);
#24936=ORIENTED_EDGE('',*,*,#17297,.F.);
#24937=ORIENTED_EDGE('',*,*,#17393,.F.);
#24938=ORIENTED_EDGE('',*,*,#17298,.F.);
#24939=ORIENTED_EDGE('',*,*,#17392,.T.);
#24940=ORIENTED_EDGE('',*,*,#17394,.T.);
#24941=ORIENTED_EDGE('',*,*,#17395,.F.);
#24942=ORIENTED_EDGE('',*,*,#17394,.F.);
#24943=ORIENTED_EDGE('',*,*,#17391,.F.);
#24944=ORIENTED_EDGE('',*,*,#17396,.F.);
#24945=ORIENTED_EDGE('',*,*,#17397,.T.);
#24946=ORIENTED_EDGE('',*,*,#17398,.F.);
#24947=ORIENTED_EDGE('',*,*,#17300,.F.);
#24948=ORIENTED_EDGE('',*,*,#17399,.F.);
#24949=ORIENTED_EDGE('',*,*,#17301,.F.);
#24950=ORIENTED_EDGE('',*,*,#17398,.T.);
#24951=ORIENTED_EDGE('',*,*,#17400,.T.);
#24952=ORIENTED_EDGE('',*,*,#17401,.F.);
#24953=ORIENTED_EDGE('',*,*,#17400,.F.);
#24954=ORIENTED_EDGE('',*,*,#17397,.F.);
#24955=ORIENTED_EDGE('',*,*,#17402,.F.);
#24956=ORIENTED_EDGE('',*,*,#17403,.T.);
#24957=ORIENTED_EDGE('',*,*,#17404,.F.);
#24958=ORIENTED_EDGE('',*,*,#17303,.F.);
#24959=ORIENTED_EDGE('',*,*,#17405,.F.);
#24960=ORIENTED_EDGE('',*,*,#17198,.F.);
#24961=ORIENTED_EDGE('',*,*,#17404,.T.);
#24962=ORIENTED_EDGE('',*,*,#17406,.T.);
#24963=ORIENTED_EDGE('',*,*,#17407,.F.);
#24964=ORIENTED_EDGE('',*,*,#17406,.F.);
#24965=ORIENTED_EDGE('',*,*,#17403,.F.);
#24966=ORIENTED_EDGE('',*,*,#17408,.F.);
#24967=ORIENTED_EDGE('',*,*,#17409,.F.);
#24968=ORIENTED_EDGE('',*,*,#17410,.T.);
#24969=ORIENTED_EDGE('',*,*,#17411,.F.);
#24970=ORIENTED_EDGE('',*,*,#17200,.F.);
#24971=ORIENTED_EDGE('',*,*,#17412,.F.);
#24972=ORIENTED_EDGE('',*,*,#17201,.F.);
#24973=ORIENTED_EDGE('',*,*,#17411,.T.);
#24974=ORIENTED_EDGE('',*,*,#17413,.T.);
#24975=ORIENTED_EDGE('',*,*,#17414,.F.);
#24976=ORIENTED_EDGE('',*,*,#17413,.F.);
#24977=ORIENTED_EDGE('',*,*,#17410,.F.);
#24978=ORIENTED_EDGE('',*,*,#17415,.F.);
#24979=ORIENTED_EDGE('',*,*,#17416,.T.);
#24980=ORIENTED_EDGE('',*,*,#17417,.F.);
#24981=ORIENTED_EDGE('',*,*,#17203,.F.);
#24982=ORIENTED_EDGE('',*,*,#17418,.F.);
#24983=ORIENTED_EDGE('',*,*,#17204,.F.);
#24984=ORIENTED_EDGE('',*,*,#17417,.T.);
#24985=ORIENTED_EDGE('',*,*,#17419,.T.);
#24986=ORIENTED_EDGE('',*,*,#17420,.F.);
#24987=ORIENTED_EDGE('',*,*,#17419,.F.);
#24988=ORIENTED_EDGE('',*,*,#17416,.F.);
#24989=ORIENTED_EDGE('',*,*,#17421,.F.);
#24990=ORIENTED_EDGE('',*,*,#17422,.T.);
#24991=ORIENTED_EDGE('',*,*,#17423,.F.);
#24992=ORIENTED_EDGE('',*,*,#17206,.F.);
#24993=ORIENTED_EDGE('',*,*,#17424,.F.);
#24994=ORIENTED_EDGE('',*,*,#17207,.F.);
#24995=ORIENTED_EDGE('',*,*,#17423,.T.);
#24996=ORIENTED_EDGE('',*,*,#17425,.T.);
#24997=ORIENTED_EDGE('',*,*,#17426,.F.);
#24998=ORIENTED_EDGE('',*,*,#17425,.F.);
#24999=ORIENTED_EDGE('',*,*,#17422,.F.);
#25000=ORIENTED_EDGE('',*,*,#17427,.F.);
#25001=ORIENTED_EDGE('',*,*,#17428,.T.);
#25002=ORIENTED_EDGE('',*,*,#17429,.F.);
#25003=ORIENTED_EDGE('',*,*,#17209,.F.);
#25004=ORIENTED_EDGE('',*,*,#17430,.F.);
#25005=ORIENTED_EDGE('',*,*,#17210,.F.);
#25006=ORIENTED_EDGE('',*,*,#17429,.T.);
#25007=ORIENTED_EDGE('',*,*,#17431,.T.);
#25008=ORIENTED_EDGE('',*,*,#17432,.F.);
#25009=ORIENTED_EDGE('',*,*,#17431,.F.);
#25010=ORIENTED_EDGE('',*,*,#17428,.F.);
#25011=ORIENTED_EDGE('',*,*,#17433,.F.);
#25012=ORIENTED_EDGE('',*,*,#17434,.T.);
#25013=ORIENTED_EDGE('',*,*,#17435,.F.);
#25014=ORIENTED_EDGE('',*,*,#17212,.F.);
#25015=ORIENTED_EDGE('',*,*,#17436,.F.);
#25016=ORIENTED_EDGE('',*,*,#17213,.F.);
#25017=ORIENTED_EDGE('',*,*,#17435,.T.);
#25018=ORIENTED_EDGE('',*,*,#17437,.T.);
#25019=ORIENTED_EDGE('',*,*,#17438,.F.);
#25020=ORIENTED_EDGE('',*,*,#17437,.F.);
#25021=ORIENTED_EDGE('',*,*,#17434,.F.);
#25022=ORIENTED_EDGE('',*,*,#17439,.F.);
#25023=ORIENTED_EDGE('',*,*,#17440,.T.);
#25024=ORIENTED_EDGE('',*,*,#17441,.F.);
#25025=ORIENTED_EDGE('',*,*,#17215,.F.);
#25026=ORIENTED_EDGE('',*,*,#17442,.F.);
#25027=ORIENTED_EDGE('',*,*,#17216,.F.);
#25028=ORIENTED_EDGE('',*,*,#17441,.T.);
#25029=ORIENTED_EDGE('',*,*,#17443,.T.);
#25030=ORIENTED_EDGE('',*,*,#17444,.F.);
#25031=ORIENTED_EDGE('',*,*,#17443,.F.);
#25032=ORIENTED_EDGE('',*,*,#17440,.F.);
#25033=ORIENTED_EDGE('',*,*,#17445,.F.);
#25034=ORIENTED_EDGE('',*,*,#17446,.T.);
#25035=ORIENTED_EDGE('',*,*,#17447,.F.);
#25036=ORIENTED_EDGE('',*,*,#17218,.F.);
#25037=ORIENTED_EDGE('',*,*,#17448,.F.);
#25038=ORIENTED_EDGE('',*,*,#17219,.F.);
#25039=ORIENTED_EDGE('',*,*,#17447,.T.);
#25040=ORIENTED_EDGE('',*,*,#17449,.T.);
#25041=ORIENTED_EDGE('',*,*,#17450,.F.);
#25042=ORIENTED_EDGE('',*,*,#17449,.F.);
#25043=ORIENTED_EDGE('',*,*,#17446,.F.);
#25044=ORIENTED_EDGE('',*,*,#17451,.F.);
#25045=ORIENTED_EDGE('',*,*,#17452,.T.);
#25046=ORIENTED_EDGE('',*,*,#17453,.F.);
#25047=ORIENTED_EDGE('',*,*,#17221,.F.);
#25048=ORIENTED_EDGE('',*,*,#17454,.F.);
#25049=ORIENTED_EDGE('',*,*,#17222,.F.);
#25050=ORIENTED_EDGE('',*,*,#17453,.T.);
#25051=ORIENTED_EDGE('',*,*,#17455,.T.);
#25052=ORIENTED_EDGE('',*,*,#17456,.F.);
#25053=ORIENTED_EDGE('',*,*,#17455,.F.);
#25054=ORIENTED_EDGE('',*,*,#17452,.F.);
#25055=ORIENTED_EDGE('',*,*,#17457,.F.);
#25056=ORIENTED_EDGE('',*,*,#17458,.T.);
#25057=ORIENTED_EDGE('',*,*,#17459,.F.);
#25058=ORIENTED_EDGE('',*,*,#17224,.F.);
#25059=ORIENTED_EDGE('',*,*,#17460,.F.);
#25060=ORIENTED_EDGE('',*,*,#17225,.F.);
#25061=ORIENTED_EDGE('',*,*,#17459,.T.);
#25062=ORIENTED_EDGE('',*,*,#17461,.T.);
#25063=ORIENTED_EDGE('',*,*,#17462,.F.);
#25064=ORIENTED_EDGE('',*,*,#17461,.F.);
#25065=ORIENTED_EDGE('',*,*,#17458,.F.);
#25066=ORIENTED_EDGE('',*,*,#17463,.F.);
#25067=ORIENTED_EDGE('',*,*,#17464,.T.);
#25068=ORIENTED_EDGE('',*,*,#17465,.F.);
#25069=ORIENTED_EDGE('',*,*,#17227,.F.);
#25070=ORIENTED_EDGE('',*,*,#17466,.F.);
#25071=ORIENTED_EDGE('',*,*,#17228,.F.);
#25072=ORIENTED_EDGE('',*,*,#17465,.T.);
#25073=ORIENTED_EDGE('',*,*,#17467,.T.);
#25074=ORIENTED_EDGE('',*,*,#17468,.F.);
#25075=ORIENTED_EDGE('',*,*,#17467,.F.);
#25076=ORIENTED_EDGE('',*,*,#17464,.F.);
#25077=ORIENTED_EDGE('',*,*,#17469,.F.);
#25078=ORIENTED_EDGE('',*,*,#17470,.T.);
#25079=ORIENTED_EDGE('',*,*,#17471,.F.);
#25080=ORIENTED_EDGE('',*,*,#17230,.F.);
#25081=ORIENTED_EDGE('',*,*,#17472,.F.);
#25082=ORIENTED_EDGE('',*,*,#17231,.F.);
#25083=ORIENTED_EDGE('',*,*,#17471,.T.);
#25084=ORIENTED_EDGE('',*,*,#17473,.T.);
#25085=ORIENTED_EDGE('',*,*,#17474,.F.);
#25086=ORIENTED_EDGE('',*,*,#17473,.F.);
#25087=ORIENTED_EDGE('',*,*,#17470,.F.);
#25088=ORIENTED_EDGE('',*,*,#17475,.F.);
#25089=ORIENTED_EDGE('',*,*,#17476,.T.);
#25090=ORIENTED_EDGE('',*,*,#17477,.F.);
#25091=ORIENTED_EDGE('',*,*,#17233,.F.);
#25092=ORIENTED_EDGE('',*,*,#17478,.F.);
#25093=ORIENTED_EDGE('',*,*,#17234,.F.);
#25094=ORIENTED_EDGE('',*,*,#17477,.T.);
#25095=ORIENTED_EDGE('',*,*,#17479,.T.);
#25096=ORIENTED_EDGE('',*,*,#17480,.F.);
#25097=ORIENTED_EDGE('',*,*,#17479,.F.);
#25098=ORIENTED_EDGE('',*,*,#17476,.F.);
#25099=ORIENTED_EDGE('',*,*,#17481,.F.);
#25100=ORIENTED_EDGE('',*,*,#17482,.T.);
#25101=ORIENTED_EDGE('',*,*,#17483,.F.);
#25102=ORIENTED_EDGE('',*,*,#17236,.F.);
#25103=ORIENTED_EDGE('',*,*,#17484,.F.);
#25104=ORIENTED_EDGE('',*,*,#17237,.F.);
#25105=ORIENTED_EDGE('',*,*,#17483,.T.);
#25106=ORIENTED_EDGE('',*,*,#17485,.T.);
#25107=ORIENTED_EDGE('',*,*,#17486,.F.);
#25108=ORIENTED_EDGE('',*,*,#17485,.F.);
#25109=ORIENTED_EDGE('',*,*,#17482,.F.);
#25110=ORIENTED_EDGE('',*,*,#17487,.F.);
#25111=ORIENTED_EDGE('',*,*,#17488,.T.);
#25112=ORIENTED_EDGE('',*,*,#17489,.F.);
#25113=ORIENTED_EDGE('',*,*,#17239,.F.);
#25114=ORIENTED_EDGE('',*,*,#17490,.F.);
#25115=ORIENTED_EDGE('',*,*,#17240,.F.);
#25116=ORIENTED_EDGE('',*,*,#17489,.T.);
#25117=ORIENTED_EDGE('',*,*,#17491,.T.);
#25118=ORIENTED_EDGE('',*,*,#17492,.F.);
#25119=ORIENTED_EDGE('',*,*,#17491,.F.);
#25120=ORIENTED_EDGE('',*,*,#17488,.F.);
#25121=ORIENTED_EDGE('',*,*,#17493,.F.);
#25122=ORIENTED_EDGE('',*,*,#17494,.T.);
#25123=ORIENTED_EDGE('',*,*,#17495,.F.);
#25124=ORIENTED_EDGE('',*,*,#17242,.F.);
#25125=ORIENTED_EDGE('',*,*,#17496,.F.);
#25126=ORIENTED_EDGE('',*,*,#17243,.F.);
#25127=ORIENTED_EDGE('',*,*,#17495,.T.);
#25128=ORIENTED_EDGE('',*,*,#17497,.T.);
#25129=ORIENTED_EDGE('',*,*,#17498,.F.);
#25130=ORIENTED_EDGE('',*,*,#17497,.F.);
#25131=ORIENTED_EDGE('',*,*,#17494,.F.);
#25132=ORIENTED_EDGE('',*,*,#17499,.F.);
#25133=ORIENTED_EDGE('',*,*,#17500,.T.);
#25134=ORIENTED_EDGE('',*,*,#17501,.F.);
#25135=ORIENTED_EDGE('',*,*,#17245,.F.);
#25136=ORIENTED_EDGE('',*,*,#17502,.F.);
#25137=ORIENTED_EDGE('',*,*,#17246,.F.);
#25138=ORIENTED_EDGE('',*,*,#17501,.T.);
#25139=ORIENTED_EDGE('',*,*,#17503,.T.);
#25140=ORIENTED_EDGE('',*,*,#17504,.F.);
#25141=ORIENTED_EDGE('',*,*,#17503,.F.);
#25142=ORIENTED_EDGE('',*,*,#17500,.F.);
#25143=ORIENTED_EDGE('',*,*,#17505,.F.);
#25144=ORIENTED_EDGE('',*,*,#17506,.T.);
#25145=ORIENTED_EDGE('',*,*,#17507,.F.);
#25146=ORIENTED_EDGE('',*,*,#17248,.F.);
#25147=ORIENTED_EDGE('',*,*,#17508,.F.);
#25148=ORIENTED_EDGE('',*,*,#17249,.F.);
#25149=ORIENTED_EDGE('',*,*,#17507,.T.);
#25150=ORIENTED_EDGE('',*,*,#17509,.T.);
#25151=ORIENTED_EDGE('',*,*,#17510,.F.);
#25152=ORIENTED_EDGE('',*,*,#17509,.F.);
#25153=ORIENTED_EDGE('',*,*,#17506,.F.);
#25154=ORIENTED_EDGE('',*,*,#17511,.F.);
#25155=ORIENTED_EDGE('',*,*,#17512,.T.);
#25156=ORIENTED_EDGE('',*,*,#17513,.F.);
#25157=ORIENTED_EDGE('',*,*,#17251,.F.);
#25158=ORIENTED_EDGE('',*,*,#17514,.F.);
#25159=ORIENTED_EDGE('',*,*,#17252,.F.);
#25160=ORIENTED_EDGE('',*,*,#17513,.T.);
#25161=ORIENTED_EDGE('',*,*,#17515,.T.);
#25162=ORIENTED_EDGE('',*,*,#17516,.F.);
#25163=ORIENTED_EDGE('',*,*,#17515,.F.);
#25164=ORIENTED_EDGE('',*,*,#17512,.F.);
#25165=ORIENTED_EDGE('',*,*,#17407,.T.);
#25166=ORIENTED_EDGE('',*,*,#17517,.T.);
#25167=ORIENTED_EDGE('',*,*,#17187,.T.);
#25168=ORIENTED_EDGE('',*,*,#17517,.F.);
#25169=ORIENTED_EDGE('',*,*,#17408,.T.);
#25170=ORIENTED_EDGE('',*,*,#17402,.T.);
#25171=ORIENTED_EDGE('',*,*,#17302,.F.);
#25172=ORIENTED_EDGE('',*,*,#17399,.T.);
#25173=ORIENTED_EDGE('',*,*,#17401,.T.);
#25174=ORIENTED_EDGE('',*,*,#17396,.T.);
#25175=ORIENTED_EDGE('',*,*,#17299,.F.);
#25176=ORIENTED_EDGE('',*,*,#17393,.T.);
#25177=ORIENTED_EDGE('',*,*,#17395,.T.);
#25178=ORIENTED_EDGE('',*,*,#17390,.T.);
#25179=ORIENTED_EDGE('',*,*,#17296,.F.);
#25180=ORIENTED_EDGE('',*,*,#17387,.T.);
#25181=ORIENTED_EDGE('',*,*,#17389,.T.);
#25182=ORIENTED_EDGE('',*,*,#17384,.T.);
#25183=ORIENTED_EDGE('',*,*,#17293,.F.);
#25184=ORIENTED_EDGE('',*,*,#17381,.T.);
#25185=ORIENTED_EDGE('',*,*,#17383,.T.);
#25186=ORIENTED_EDGE('',*,*,#17378,.T.);
#25187=ORIENTED_EDGE('',*,*,#17290,.F.);
#25188=ORIENTED_EDGE('',*,*,#17375,.T.);
#25189=ORIENTED_EDGE('',*,*,#17377,.T.);
#25190=ORIENTED_EDGE('',*,*,#17372,.T.);
#25191=ORIENTED_EDGE('',*,*,#17287,.F.);
#25192=ORIENTED_EDGE('',*,*,#17369,.T.);
#25193=ORIENTED_EDGE('',*,*,#17371,.T.);
#25194=ORIENTED_EDGE('',*,*,#17366,.T.);
#25195=ORIENTED_EDGE('',*,*,#17284,.F.);
#25196=ORIENTED_EDGE('',*,*,#17363,.T.);
#25197=ORIENTED_EDGE('',*,*,#17365,.T.);
#25198=ORIENTED_EDGE('',*,*,#17360,.T.);
#25199=ORIENTED_EDGE('',*,*,#17281,.F.);
#25200=ORIENTED_EDGE('',*,*,#17357,.T.);
#25201=ORIENTED_EDGE('',*,*,#17359,.T.);
#25202=ORIENTED_EDGE('',*,*,#17354,.T.);
#25203=ORIENTED_EDGE('',*,*,#17278,.F.);
#25204=ORIENTED_EDGE('',*,*,#17351,.T.);
#25205=ORIENTED_EDGE('',*,*,#17353,.T.);
#25206=ORIENTED_EDGE('',*,*,#17348,.T.);
#25207=ORIENTED_EDGE('',*,*,#17275,.F.);
#25208=ORIENTED_EDGE('',*,*,#17345,.T.);
#25209=ORIENTED_EDGE('',*,*,#17347,.T.);
#25210=ORIENTED_EDGE('',*,*,#17342,.T.);
#25211=ORIENTED_EDGE('',*,*,#17272,.F.);
#25212=ORIENTED_EDGE('',*,*,#17339,.T.);
#25213=ORIENTED_EDGE('',*,*,#17341,.T.);
#25214=ORIENTED_EDGE('',*,*,#17336,.T.);
#25215=ORIENTED_EDGE('',*,*,#17269,.F.);
#25216=ORIENTED_EDGE('',*,*,#17333,.T.);
#25217=ORIENTED_EDGE('',*,*,#17335,.T.);
#25218=ORIENTED_EDGE('',*,*,#17330,.T.);
#25219=ORIENTED_EDGE('',*,*,#17266,.F.);
#25220=ORIENTED_EDGE('',*,*,#17327,.T.);
#25221=ORIENTED_EDGE('',*,*,#17329,.T.);
#25222=ORIENTED_EDGE('',*,*,#17324,.T.);
#25223=ORIENTED_EDGE('',*,*,#17263,.F.);
#25224=ORIENTED_EDGE('',*,*,#17321,.T.);
#25225=ORIENTED_EDGE('',*,*,#17323,.T.);
#25226=ORIENTED_EDGE('',*,*,#17318,.T.);
#25227=ORIENTED_EDGE('',*,*,#17260,.F.);
#25228=ORIENTED_EDGE('',*,*,#17315,.T.);
#25229=ORIENTED_EDGE('',*,*,#17317,.T.);
#25230=ORIENTED_EDGE('',*,*,#17312,.T.);
#25231=ORIENTED_EDGE('',*,*,#17257,.F.);
#25232=ORIENTED_EDGE('',*,*,#17309,.T.);
#25233=ORIENTED_EDGE('',*,*,#17311,.T.);
#25234=ORIENTED_EDGE('',*,*,#17306,.T.);
#25235=ORIENTED_EDGE('',*,*,#17254,.F.);
#25236=ORIENTED_EDGE('',*,*,#17194,.T.);
#25237=ORIENTED_EDGE('',*,*,#17197,.T.);
#25238=ORIENTED_EDGE('',*,*,#17190,.T.);
#25239=ORIENTED_EDGE('',*,*,#17253,.F.);
#25240=ORIENTED_EDGE('',*,*,#17514,.T.);
#25241=ORIENTED_EDGE('',*,*,#17516,.T.);
#25242=ORIENTED_EDGE('',*,*,#17511,.T.);
#25243=ORIENTED_EDGE('',*,*,#17250,.F.);
#25244=ORIENTED_EDGE('',*,*,#17508,.T.);
#25245=ORIENTED_EDGE('',*,*,#17510,.T.);
#25246=ORIENTED_EDGE('',*,*,#17505,.T.);
#25247=ORIENTED_EDGE('',*,*,#17247,.F.);
#25248=ORIENTED_EDGE('',*,*,#17502,.T.);
#25249=ORIENTED_EDGE('',*,*,#17504,.T.);
#25250=ORIENTED_EDGE('',*,*,#17499,.T.);
#25251=ORIENTED_EDGE('',*,*,#17244,.F.);
#25252=ORIENTED_EDGE('',*,*,#17496,.T.);
#25253=ORIENTED_EDGE('',*,*,#17498,.T.);
#25254=ORIENTED_EDGE('',*,*,#17493,.T.);
#25255=ORIENTED_EDGE('',*,*,#17241,.F.);
#25256=ORIENTED_EDGE('',*,*,#17490,.T.);
#25257=ORIENTED_EDGE('',*,*,#17492,.T.);
#25258=ORIENTED_EDGE('',*,*,#17487,.T.);
#25259=ORIENTED_EDGE('',*,*,#17238,.F.);
#25260=ORIENTED_EDGE('',*,*,#17484,.T.);
#25261=ORIENTED_EDGE('',*,*,#17486,.T.);
#25262=ORIENTED_EDGE('',*,*,#17481,.T.);
#25263=ORIENTED_EDGE('',*,*,#17235,.F.);
#25264=ORIENTED_EDGE('',*,*,#17478,.T.);
#25265=ORIENTED_EDGE('',*,*,#17480,.T.);
#25266=ORIENTED_EDGE('',*,*,#17475,.T.);
#25267=ORIENTED_EDGE('',*,*,#17232,.F.);
#25268=ORIENTED_EDGE('',*,*,#17472,.T.);
#25269=ORIENTED_EDGE('',*,*,#17474,.T.);
#25270=ORIENTED_EDGE('',*,*,#17469,.T.);
#25271=ORIENTED_EDGE('',*,*,#17229,.F.);
#25272=ORIENTED_EDGE('',*,*,#17466,.T.);
#25273=ORIENTED_EDGE('',*,*,#17468,.T.);
#25274=ORIENTED_EDGE('',*,*,#17463,.T.);
#25275=ORIENTED_EDGE('',*,*,#17226,.F.);
#25276=ORIENTED_EDGE('',*,*,#17460,.T.);
#25277=ORIENTED_EDGE('',*,*,#17462,.T.);
#25278=ORIENTED_EDGE('',*,*,#17457,.T.);
#25279=ORIENTED_EDGE('',*,*,#17223,.F.);
#25280=ORIENTED_EDGE('',*,*,#17454,.T.);
#25281=ORIENTED_EDGE('',*,*,#17456,.T.);
#25282=ORIENTED_EDGE('',*,*,#17451,.T.);
#25283=ORIENTED_EDGE('',*,*,#17220,.F.);
#25284=ORIENTED_EDGE('',*,*,#17448,.T.);
#25285=ORIENTED_EDGE('',*,*,#17450,.T.);
#25286=ORIENTED_EDGE('',*,*,#17445,.T.);
#25287=ORIENTED_EDGE('',*,*,#17217,.F.);
#25288=ORIENTED_EDGE('',*,*,#17442,.T.);
#25289=ORIENTED_EDGE('',*,*,#17444,.T.);
#25290=ORIENTED_EDGE('',*,*,#17439,.T.);
#25291=ORIENTED_EDGE('',*,*,#17214,.F.);
#25292=ORIENTED_EDGE('',*,*,#17436,.T.);
#25293=ORIENTED_EDGE('',*,*,#17438,.T.);
#25294=ORIENTED_EDGE('',*,*,#17433,.T.);
#25295=ORIENTED_EDGE('',*,*,#17211,.F.);
#25296=ORIENTED_EDGE('',*,*,#17430,.T.);
#25297=ORIENTED_EDGE('',*,*,#17432,.T.);
#25298=ORIENTED_EDGE('',*,*,#17427,.T.);
#25299=ORIENTED_EDGE('',*,*,#17208,.F.);
#25300=ORIENTED_EDGE('',*,*,#17424,.T.);
#25301=ORIENTED_EDGE('',*,*,#17426,.T.);
#25302=ORIENTED_EDGE('',*,*,#17421,.T.);
#25303=ORIENTED_EDGE('',*,*,#17205,.F.);
#25304=ORIENTED_EDGE('',*,*,#17418,.T.);
#25305=ORIENTED_EDGE('',*,*,#17420,.T.);
#25306=ORIENTED_EDGE('',*,*,#17415,.T.);
#25307=ORIENTED_EDGE('',*,*,#17202,.F.);
#25308=ORIENTED_EDGE('',*,*,#17412,.T.);
#25309=ORIENTED_EDGE('',*,*,#17414,.T.);
#25310=ORIENTED_EDGE('',*,*,#17409,.T.);
#25311=ORIENTED_EDGE('',*,*,#17199,.F.);
#25312=ORIENTED_EDGE('',*,*,#17405,.T.);
#25313=ORIENTED_EDGE('',*,*,#17305,.F.);
#25314=ORIENTED_EDGE('',*,*,#17518,.T.);
#25315=ORIENTED_EDGE('',*,*,#17519,.T.);
#25316=ORIENTED_EDGE('',*,*,#17520,.T.);
#25317=ORIENTED_EDGE('',*,*,#17521,.T.);
#25318=ORIENTED_EDGE('',*,*,#17522,.T.);
#25319=ORIENTED_EDGE('',*,*,#17523,.T.);
#25320=ORIENTED_EDGE('',*,*,#17524,.F.);
#25321=ORIENTED_EDGE('',*,*,#17525,.T.);
#25322=ORIENTED_EDGE('',*,*,#17526,.F.);
#25323=ORIENTED_EDGE('',*,*,#17527,.T.);
#25324=ORIENTED_EDGE('',*,*,#17528,.F.);
#25325=ORIENTED_EDGE('',*,*,#17529,.T.);
#25326=ORIENTED_EDGE('',*,*,#17530,.F.);
#25327=ORIENTED_EDGE('',*,*,#17531,.T.);
#25328=ORIENTED_EDGE('',*,*,#17532,.F.);
#25329=ORIENTED_EDGE('',*,*,#17533,.T.);
#25330=ORIENTED_EDGE('',*,*,#17534,.F.);
#25331=ORIENTED_EDGE('',*,*,#17535,.T.);
#25332=ORIENTED_EDGE('',*,*,#17536,.T.);
#25333=ORIENTED_EDGE('',*,*,#17535,.F.);
#25334=ORIENTED_EDGE('',*,*,#17533,.F.);
#25335=ORIENTED_EDGE('',*,*,#17531,.F.);
#25336=ORIENTED_EDGE('',*,*,#17529,.F.);
#25337=ORIENTED_EDGE('',*,*,#17527,.F.);
#25338=ORIENTED_EDGE('',*,*,#17525,.F.);
#25339=ORIENTED_EDGE('',*,*,#17536,.F.);
#25340=ORIENTED_EDGE('',*,*,#17518,.F.);
#25341=ORIENTED_EDGE('',*,*,#17537,.T.);
#25342=ORIENTED_EDGE('',*,*,#17524,.T.);
#25343=ORIENTED_EDGE('',*,*,#17538,.F.);
#25344=ORIENTED_EDGE('',*,*,#17523,.F.);
#25345=ORIENTED_EDGE('',*,*,#17539,.T.);
#25346=ORIENTED_EDGE('',*,*,#17534,.T.);
#25347=ORIENTED_EDGE('',*,*,#17537,.F.);
#25348=ORIENTED_EDGE('',*,*,#17522,.F.);
#25349=ORIENTED_EDGE('',*,*,#17540,.T.);
#25350=ORIENTED_EDGE('',*,*,#17532,.T.);
#25351=ORIENTED_EDGE('',*,*,#17539,.F.);
#25352=ORIENTED_EDGE('',*,*,#17521,.F.);
#25353=ORIENTED_EDGE('',*,*,#17541,.T.);
#25354=ORIENTED_EDGE('',*,*,#17530,.T.);
#25355=ORIENTED_EDGE('',*,*,#17540,.F.);
#25356=ORIENTED_EDGE('',*,*,#17520,.F.);
#25357=ORIENTED_EDGE('',*,*,#17542,.T.);
#25358=ORIENTED_EDGE('',*,*,#17528,.T.);
#25359=ORIENTED_EDGE('',*,*,#17541,.F.);
#25360=ORIENTED_EDGE('',*,*,#17519,.F.);
#25361=ORIENTED_EDGE('',*,*,#17538,.T.);
#25362=ORIENTED_EDGE('',*,*,#17526,.T.);
#25363=ORIENTED_EDGE('',*,*,#17542,.F.);
#25542=CONICAL_SURFACE('',#28964,1.52934,0.785398163397448);
#25543=CONICAL_SURFACE('',#28971,2.7202,0.785398163397434);
#25544=CONICAL_SURFACE('',#29164,1.60395121659244,1.02974425867666);
#26754=ADVANCED_FACE('',(#3561),#2330,.T.);
#26755=ADVANCED_FACE('',(#3562),#2331,.T.);
#26756=ADVANCED_FACE('',(#3563),#2332,.T.);
#26757=ADVANCED_FACE('',(#3564),#2333,.T.);
#26758=ADVANCED_FACE('',(#3565),#2334,.T.);
#26759=ADVANCED_FACE('',(#3566),#2335,.T.);
#26760=ADVANCED_FACE('',(#3567),#2336,.T.);
#26761=ADVANCED_FACE('',(#3568),#2337,.T.);
#26762=ADVANCED_FACE('',(#3569),#2338,.T.);
#26763=ADVANCED_FACE('',(#3570),#2339,.T.);
#26764=ADVANCED_FACE('',(#3571),#2340,.T.);
#26765=ADVANCED_FACE('',(#3572),#2341,.T.);
#26766=ADVANCED_FACE('',(#3573),#2342,.T.);
#26767=ADVANCED_FACE('',(#3574),#2343,.T.);
#26768=ADVANCED_FACE('',(#3575),#2344,.T.);
#26769=ADVANCED_FACE('',(#3576),#2345,.T.);
#26770=ADVANCED_FACE('',(#3577),#2346,.T.);
#26771=ADVANCED_FACE('',(#3578),#2347,.T.);
#26772=ADVANCED_FACE('',(#3579),#2348,.T.);
#26773=ADVANCED_FACE('',(#3580),#2349,.T.);
#26774=ADVANCED_FACE('',(#3581),#2350,.T.);
#26775=ADVANCED_FACE('',(#3582),#2005,.T.);
#26776=ADVANCED_FACE('',(#3583),#903,.F.);
#26777=ADVANCED_FACE('',(#3584),#2006,.F.);
#26778=ADVANCED_FACE('',(#3585),#904,.F.);
#26779=ADVANCED_FACE('',(#3586),#507,.F.);
#26780=ADVANCED_FACE('',(#3587,#1115),#2007,.F.);
#26781=ADVANCED_FACE('',(#3588),#25542,.T.);
#26782=ADVANCED_FACE('',(#3589),#2008,.F.);
#26783=ADVANCED_FACE('',(#3590),#2009,.F.);
#26784=ADVANCED_FACE('',(#3591),#2010,.F.);
#26785=ADVANCED_FACE('',(#3592),#2011,.F.);
#26786=ADVANCED_FACE('',(#3593),#25543,.T.);
#26787=ADVANCED_FACE('',(#3594),#2012,.F.);
#26788=ADVANCED_FACE('',(#3595),#2013,.F.);
#26789=ADVANCED_FACE('',(#3596),#2014,.F.);
#26790=ADVANCED_FACE('',(#3597),#2015,.F.);
#26791=ADVANCED_FACE('',(#3598),#2016,.F.);
#26792=ADVANCED_FACE('',(#3599),#2017,.F.);
#26793=ADVANCED_FACE('',(#3600),#2018,.F.);
#26794=ADVANCED_FACE('',(#3601),#2019,.F.);
#26795=ADVANCED_FACE('',(#3602),#2020,.F.);
#26796=ADVANCED_FACE('',(#3603),#2021,.F.);
#26797=ADVANCED_FACE('',(#3604),#2022,.F.);
#26798=ADVANCED_FACE('',(#3605),#2023,.F.);
#26799=ADVANCED_FACE('',(#3606),#2024,.F.);
#26800=ADVANCED_FACE('',(#3607),#2025,.F.);
#26801=ADVANCED_FACE('',(#3608),#2026,.F.);
#26802=ADVANCED_FACE('',(#3609),#2027,.F.);
#26803=ADVANCED_FACE('',(#3610),#2028,.F.);
#26804=ADVANCED_FACE('',(#3611),#2029,.F.);
#26805=ADVANCED_FACE('',(#3612),#2030,.F.);
#26806=ADVANCED_FACE('',(#3613),#2031,.F.);
#26807=ADVANCED_FACE('',(#3614),#2032,.F.);
#26808=ADVANCED_FACE('',(#3615),#2033,.F.);
#26809=ADVANCED_FACE('',(#3616),#2034,.F.);
#26810=ADVANCED_FACE('',(#3617),#2035,.F.);
#26811=ADVANCED_FACE('',(#3618),#2036,.F.);
#26812=ADVANCED_FACE('',(#3619),#2037,.F.);
#26813=ADVANCED_FACE('',(#3620),#2038,.F.);
#26814=ADVANCED_FACE('',(#3621),#2039,.F.);
#26815=ADVANCED_FACE('',(#3622),#2040,.F.);
#26816=ADVANCED_FACE('',(#3623),#2041,.F.);
#26817=ADVANCED_FACE('',(#3624),#2042,.F.);
#26818=ADVANCED_FACE('',(#3625),#2043,.F.);
#26819=ADVANCED_FACE('',(#3626),#2044,.F.);
#26820=ADVANCED_FACE('',(#3627),#2045,.F.);
#26821=ADVANCED_FACE('',(#3628),#2046,.F.);
#26822=ADVANCED_FACE('',(#3629),#2047,.F.);
#26823=ADVANCED_FACE('',(#3630),#2048,.F.);
#26824=ADVANCED_FACE('',(#3631),#2049,.F.);
#26825=ADVANCED_FACE('',(#3632),#2050,.F.);
#26826=ADVANCED_FACE('',(#3633),#2051,.F.);
#26827=ADVANCED_FACE('',(#3634),#2052,.F.);
#26828=ADVANCED_FACE('',(#3635),#2053,.F.);
#26829=ADVANCED_FACE('',(#3636),#2054,.F.);
#26830=ADVANCED_FACE('',(#3637),#2055,.F.);
#26831=ADVANCED_FACE('',(#3638),#2056,.F.);
#26832=ADVANCED_FACE('',(#3639),#2057,.F.);
#26833=ADVANCED_FACE('',(#3640),#2058,.F.);
#26834=ADVANCED_FACE('',(#3641),#2059,.F.);
#26835=ADVANCED_FACE('',(#3642),#2060,.F.);
#26836=ADVANCED_FACE('',(#3643),#2061,.F.);
#26837=ADVANCED_FACE('',(#3644),#2062,.F.);
#26838=ADVANCED_FACE('',(#3645),#2063,.F.);
#26839=ADVANCED_FACE('',(#3646),#2064,.F.);
#26840=ADVANCED_FACE('',(#3647),#2065,.F.);
#26841=ADVANCED_FACE('',(#3648),#2066,.F.);
#26842=ADVANCED_FACE('',(#3649),#2067,.F.);
#26843=ADVANCED_FACE('',(#3650),#2068,.F.);
#26844=ADVANCED_FACE('',(#3651),#2069,.F.);
#26845=ADVANCED_FACE('',(#3652),#2070,.F.);
#26846=ADVANCED_FACE('',(#3653),#2071,.F.);
#26847=ADVANCED_FACE('',(#3654),#2072,.F.);
#26848=ADVANCED_FACE('',(#3655),#2073,.F.);
#26849=ADVANCED_FACE('',(#3656),#2074,.F.);
#26850=ADVANCED_FACE('',(#3657),#2075,.F.);
#26851=ADVANCED_FACE('',(#3658),#2076,.F.);
#26852=ADVANCED_FACE('',(#3659),#2077,.F.);
#26853=ADVANCED_FACE('',(#3660),#2078,.F.);
#26854=ADVANCED_FACE('',(#3661),#2079,.F.);
#26855=ADVANCED_FACE('',(#3662),#2080,.F.);
#26856=ADVANCED_FACE('',(#3663),#2081,.F.);
#26857=ADVANCED_FACE('',(#3664),#2082,.F.);
#26858=ADVANCED_FACE('',(#3665),#2083,.F.);
#26859=ADVANCED_FACE('',(#3666),#2084,.F.);
#26860=ADVANCED_FACE('',(#3667),#2085,.F.);
#26861=ADVANCED_FACE('',(#3668),#2086,.F.);
#26862=ADVANCED_FACE('',(#3669),#2087,.F.);
#26863=ADVANCED_FACE('',(#3670),#2088,.F.);
#26864=ADVANCED_FACE('',(#3671),#2089,.F.);
#26865=ADVANCED_FACE('',(#3672),#2090,.F.);
#26866=ADVANCED_FACE('',(#3673),#2091,.F.);
#26867=ADVANCED_FACE('',(#3674),#2092,.F.);
#26868=ADVANCED_FACE('',(#3675),#2093,.F.);
#26869=ADVANCED_FACE('',(#3676),#2094,.F.);
#26870=ADVANCED_FACE('',(#3677),#2095,.F.);
#26871=ADVANCED_FACE('',(#3678),#2096,.F.);
#26872=ADVANCED_FACE('',(#3679),#2097,.F.);
#26873=ADVANCED_FACE('',(#3680),#2098,.F.);
#26874=ADVANCED_FACE('',(#3681),#2099,.F.);
#26875=ADVANCED_FACE('',(#3682),#2100,.F.);
#26876=ADVANCED_FACE('',(#3683),#2101,.F.);
#26877=ADVANCED_FACE('',(#3684),#2102,.F.);
#26878=ADVANCED_FACE('',(#3685),#2103,.F.);
#26879=ADVANCED_FACE('',(#3686),#2104,.F.);
#26880=ADVANCED_FACE('',(#3687),#2105,.F.);
#26881=ADVANCED_FACE('',(#3688),#2106,.F.);
#26882=ADVANCED_FACE('',(#3689),#2107,.F.);
#26883=ADVANCED_FACE('',(#3690),#2108,.F.);
#26884=ADVANCED_FACE('',(#3691),#2109,.F.);
#26885=ADVANCED_FACE('',(#3692),#2110,.F.);
#26886=ADVANCED_FACE('',(#3693),#2111,.F.);
#26887=ADVANCED_FACE('',(#3694),#2112,.F.);
#26888=ADVANCED_FACE('',(#3695),#2113,.F.);
#26889=ADVANCED_FACE('',(#3696),#2114,.F.);
#26890=ADVANCED_FACE('',(#3697),#2115,.F.);
#26891=ADVANCED_FACE('',(#3698),#2116,.F.);
#26892=ADVANCED_FACE('',(#3699),#2351,.T.);
#26893=ADVANCED_FACE('',(#3700,#1116),#2117,.T.);
#26894=ADVANCED_FACE('',(#3701),#2118,.F.);
#26895=ADVANCED_FACE('',(#3702),#2119,.F.);
#26896=ADVANCED_FACE('',(#3703),#2120,.F.);
#26897=ADVANCED_FACE('',(#3704),#2121,.F.);
#26898=ADVANCED_FACE('',(#3705),#2122,.F.);
#26899=ADVANCED_FACE('',(#3706),#2123,.F.);
#26900=ADVANCED_FACE('',(#3707),#25544,.F.);
#26901=ADVANCED_FACE('',(#3708),#2124,.F.);
#26902=ADVANCED_FACE('',(#3709),#2125,.F.);
#26903=ADVANCED_FACE('',(#3710),#2126,.F.);
#26904=ADVANCED_FACE('',(#3711),#2127,.F.);
#26905=ADVANCED_FACE('',(#3712),#2128,.F.);
#26906=ADVANCED_FACE('',(#3713),#2129,.F.);
#26940=CLOSED_SHELL('',(#26754,#26755,#26756,#26757,#26758,#26759,#26760,
#26761,#26762,#26763,#26764,#26765,#26766,#26767,#26768,#26769,#26770,#26771,
#26772,#26773,#26774,#26775,#26776,#26777,#26778,#26779,#26780,#26781,#26782,
#26783,#26784,#26785,#26786,#26787,#26788,#26789,#26790,#26791,#26792,#26793,
#26794,#26795,#26796,#26797,#26798,#26799,#26800,#26801,#26802,#26803,#26804,
#26805,#26806,#26807,#26808,#26809,#26810,#26811,#26812,#26813,#26814,#26815,
#26816,#26817,#26818,#26819,#26820,#26821,#26822,#26823,#26824,#26825,#26826,
#26827,#26828,#26829,#26830,#26831,#26832,#26833,#26834,#26835,#26836,#26837,
#26838,#26839,#26840,#26841,#26842,#26843,#26844,#26845,#26846,#26847,#26848,
#26849,#26850,#26851,#26852,#26853,#26854,#26855,#26856,#26857,#26858,#26859,
#26860,#26861,#26862,#26863,#26864,#26865,#26866,#26867,#26868,#26869,#26870,
#26871,#26872,#26873,#26874,#26875,#26876,#26877,#26878,#26879,#26880,#26881,
#26882,#26883,#26884,#26885,#26886,#26887,#26888,#26889,#26890,#26891,#26892,
#26893,#26894,#26895,#26896,#26897,#26898,#26899,#26900,#26901,#26902,#26903,
#26904,#26905,#26906));
#28927=AXIS2_PLACEMENT_3D('',#66836,#35181,#35182);
#28928=AXIS2_PLACEMENT_3D('',#66837,#35183,#35184);
#28929=AXIS2_PLACEMENT_3D('',#66993,#35186,#35187);
#28930=AXIS2_PLACEMENT_3D('',#67096,#35188,#35189);
#28931=AXIS2_PLACEMENT_3D('',#67514,#35191,#35192);
#28932=AXIS2_PLACEMENT_3D('',#67782,#35194,#35195);
#28933=AXIS2_PLACEMENT_3D('',#68178,#35197,#35198);
#28934=AXIS2_PLACEMENT_3D('',#68614,#35200,#35201);
#28935=AXIS2_PLACEMENT_3D('',#69036,#35203,#35204);
#28936=AXIS2_PLACEMENT_3D('',#69470,#35206,#35207);
#28937=AXIS2_PLACEMENT_3D('',#69902,#35209,#35210);
#28938=AXIS2_PLACEMENT_3D('',#70145,#35212,#35213);
#28939=AXIS2_PLACEMENT_3D('',#70517,#35215,#35216);
#28940=AXIS2_PLACEMENT_3D('',#70784,#35218,#35219);
#28941=AXIS2_PLACEMENT_3D('',#71230,#35221,#35222);
#28942=AXIS2_PLACEMENT_3D('',#71649,#35224,#35225);
#28943=AXIS2_PLACEMENT_3D('',#72064,#35227,#35228);
#28944=AXIS2_PLACEMENT_3D('',#72501,#35230,#35231);
#28945=AXIS2_PLACEMENT_3D('',#72911,#35233,#35234);
#28946=AXIS2_PLACEMENT_3D('',#73166,#35236,#35237);
#28947=AXIS2_PLACEMENT_3D('',#73534,#35239,#35240);
#28948=AXIS2_PLACEMENT_3D('',#73945,#35242,#35243);
#28949=AXIS2_PLACEMENT_3D('',#74010,#35244,#35245);
#28950=AXIS2_PLACEMENT_3D('',#77370,#35246,#35247);
#28951=AXIS2_PLACEMENT_3D('',#80497,#35248,#35249);
#28952=AXIS2_PLACEMENT_3D('',#80684,#35250,#35251);
#28953=AXIS2_PLACEMENT_3D('',#80819,#35252,#35253);
#28954=AXIS2_PLACEMENT_3D('',#80822,#35254,#35255);
#28955=AXIS2_PLACEMENT_3D('',#80983,#35256,#35257);
#28956=AXIS2_PLACEMENT_3D('',#81580,#35258,#35259);
#28957=AXIS2_PLACEMENT_3D('',#81583,#35260,#35261);
#28958=AXIS2_PLACEMENT_3D('',#81660,#35262,#35263);
#28959=AXIS2_PLACEMENT_3D('',#82173,#35264,#35265);
#28960=AXIS2_PLACEMENT_3D('',#82175,#35266,#35267);
#28961=AXIS2_PLACEMENT_3D('',#82176,#35268,#35269);
#28962=AXIS2_PLACEMENT_3D('',#82177,#35270,#35271);
#28963=AXIS2_PLACEMENT_3D('',#82179,#35272,#35273);
#28964=AXIS2_PLACEMENT_3D('',#82180,#35274,#35275);
#28965=AXIS2_PLACEMENT_3D('',#82183,#35277,#35278);
#28966=AXIS2_PLACEMENT_3D('',#82184,#35279,#35280);
#28967=AXIS2_PLACEMENT_3D('',#82185,#35281,#35282);
#28968=AXIS2_PLACEMENT_3D('',#82196,#35286,#35287);
#28969=AXIS2_PLACEMENT_3D('',#82204,#35290,#35291);
#28970=AXIS2_PLACEMENT_3D('',#82205,#35292,#35293);
#28971=AXIS2_PLACEMENT_3D('',#82206,#35294,#35295);
#28972=AXIS2_PLACEMENT_3D('',#82213,#35296,#35297);
#28973=AXIS2_PLACEMENT_3D('',#82223,#35298,#35299);
#28974=AXIS2_PLACEMENT_3D('',#82233,#35300,#35301);
#28975=AXIS2_PLACEMENT_3D('',#82243,#35302,#35303);
#28976=AXIS2_PLACEMENT_3D('',#82253,#35304,#35305);
#28977=AXIS2_PLACEMENT_3D('',#82263,#35306,#35307);
#28978=AXIS2_PLACEMENT_3D('',#82273,#35308,#35309);
#28979=AXIS2_PLACEMENT_3D('',#82283,#35310,#35311);
#28980=AXIS2_PLACEMENT_3D('',#82293,#35312,#35313);
#28981=AXIS2_PLACEMENT_3D('',#82303,#35314,#35315);
#28982=AXIS2_PLACEMENT_3D('',#82313,#35316,#35317);
#28983=AXIS2_PLACEMENT_3D('',#82323,#35318,#35319);
#28984=AXIS2_PLACEMENT_3D('',#82333,#35320,#35321);
#28985=AXIS2_PLACEMENT_3D('',#82343,#35322,#35323);
#28986=AXIS2_PLACEMENT_3D('',#82353,#35324,#35325);
#28987=AXIS2_PLACEMENT_3D('',#82363,#35326,#35327);
#28988=AXIS2_PLACEMENT_3D('',#82373,#35328,#35329);
#28989=AXIS2_PLACEMENT_3D('',#82383,#35330,#35331);
#28990=AXIS2_PLACEMENT_3D('',#82392,#35332,#35333);
#28991=AXIS2_PLACEMENT_3D('',#82394,#35334,#35335);
#28992=AXIS2_PLACEMENT_3D('',#82404,#35336,#35337);
#28993=AXIS2_PLACEMENT_3D('',#82414,#35338,#35339);
#28994=AXIS2_PLACEMENT_3D('',#82424,#35340,#35341);
#28995=AXIS2_PLACEMENT_3D('',#82434,#35342,#35343);
#28996=AXIS2_PLACEMENT_3D('',#82444,#35344,#35345);
#28997=AXIS2_PLACEMENT_3D('',#82454,#35346,#35347);
#28998=AXIS2_PLACEMENT_3D('',#82464,#35348,#35349);
#28999=AXIS2_PLACEMENT_3D('',#82474,#35350,#35351);
#29000=AXIS2_PLACEMENT_3D('',#82484,#35352,#35353);
#29001=AXIS2_PLACEMENT_3D('',#82494,#35354,#35355);
#29002=AXIS2_PLACEMENT_3D('',#82504,#35356,#35357);
#29003=AXIS2_PLACEMENT_3D('',#82514,#35358,#35359);
#29004=AXIS2_PLACEMENT_3D('',#82524,#35360,#35361);
#29005=AXIS2_PLACEMENT_3D('',#82534,#35362,#35363);
#29006=AXIS2_PLACEMENT_3D('',#82544,#35364,#35365);
#29007=AXIS2_PLACEMENT_3D('',#82554,#35366,#35367);
#29008=AXIS2_PLACEMENT_3D('',#82560,#35369,#35370);
#29009=AXIS2_PLACEMENT_3D('',#82561,#35371,#35372);
#29010=AXIS2_PLACEMENT_3D('',#82567,#35376,#35377);
#29011=AXIS2_PLACEMENT_3D('',#82571,#35380,#35381);
#29012=AXIS2_PLACEMENT_3D('',#82572,#35382,#35383);
#29013=AXIS2_PLACEMENT_3D('',#82573,#35384,#35385);
#29014=AXIS2_PLACEMENT_3D('',#82579,#35389,#35390);
#29015=AXIS2_PLACEMENT_3D('',#82583,#35393,#35394);
#29016=AXIS2_PLACEMENT_3D('',#82584,#35395,#35396);
#29017=AXIS2_PLACEMENT_3D('',#82585,#35397,#35398);
#29018=AXIS2_PLACEMENT_3D('',#82591,#35402,#35403);
#29019=AXIS2_PLACEMENT_3D('',#82595,#35406,#35407);
#29020=AXIS2_PLACEMENT_3D('',#82596,#35408,#35409);
#29021=AXIS2_PLACEMENT_3D('',#82597,#35410,#35411);
#29022=AXIS2_PLACEMENT_3D('',#82603,#35415,#35416);
#29023=AXIS2_PLACEMENT_3D('',#82607,#35419,#35420);
#29024=AXIS2_PLACEMENT_3D('',#82608,#35421,#35422);
#29025=AXIS2_PLACEMENT_3D('',#82609,#35423,#35424);
#29026=AXIS2_PLACEMENT_3D('',#82615,#35428,#35429);
#29027=AXIS2_PLACEMENT_3D('',#82619,#35432,#35433);
#29028=AXIS2_PLACEMENT_3D('',#82620,#35434,#35435);
#29029=AXIS2_PLACEMENT_3D('',#82621,#35436,#35437);
#29030=AXIS2_PLACEMENT_3D('',#82627,#35441,#35442);
#29031=AXIS2_PLACEMENT_3D('',#82631,#35445,#35446);
#29032=AXIS2_PLACEMENT_3D('',#82632,#35447,#35448);
#29033=AXIS2_PLACEMENT_3D('',#82633,#35449,#35450);
#29034=AXIS2_PLACEMENT_3D('',#82639,#35454,#35455);
#29035=AXIS2_PLACEMENT_3D('',#82643,#35458,#35459);
#29036=AXIS2_PLACEMENT_3D('',#82644,#35460,#35461);
#29037=AXIS2_PLACEMENT_3D('',#82645,#35462,#35463);
#29038=AXIS2_PLACEMENT_3D('',#82651,#35467,#35468);
#29039=AXIS2_PLACEMENT_3D('',#82655,#35471,#35472);
#29040=AXIS2_PLACEMENT_3D('',#82656,#35473,#35474);
#29041=AXIS2_PLACEMENT_3D('',#82657,#35475,#35476);
#29042=AXIS2_PLACEMENT_3D('',#82663,#35480,#35481);
#29043=AXIS2_PLACEMENT_3D('',#82667,#35484,#35485);
#29044=AXIS2_PLACEMENT_3D('',#82668,#35486,#35487);
#29045=AXIS2_PLACEMENT_3D('',#82669,#35488,#35489);
#29046=AXIS2_PLACEMENT_3D('',#82675,#35493,#35494);
#29047=AXIS2_PLACEMENT_3D('',#82679,#35497,#35498);
#29048=AXIS2_PLACEMENT_3D('',#82680,#35499,#35500);
#29049=AXIS2_PLACEMENT_3D('',#82681,#35501,#35502);
#29050=AXIS2_PLACEMENT_3D('',#82687,#35506,#35507);
#29051=AXIS2_PLACEMENT_3D('',#82691,#35510,#35511);
#29052=AXIS2_PLACEMENT_3D('',#82692,#35512,#35513);
#29053=AXIS2_PLACEMENT_3D('',#82693,#35514,#35515);
#29054=AXIS2_PLACEMENT_3D('',#82699,#35519,#35520);
#29055=AXIS2_PLACEMENT_3D('',#82703,#35523,#35524);
#29056=AXIS2_PLACEMENT_3D('',#82704,#35525,#35526);
#29057=AXIS2_PLACEMENT_3D('',#82705,#35527,#35528);
#29058=AXIS2_PLACEMENT_3D('',#82711,#35532,#35533);
#29059=AXIS2_PLACEMENT_3D('',#82715,#35536,#35537);
#29060=AXIS2_PLACEMENT_3D('',#82716,#35538,#35539);
#29061=AXIS2_PLACEMENT_3D('',#82717,#35540,#35541);
#29062=AXIS2_PLACEMENT_3D('',#82723,#35545,#35546);
#29063=AXIS2_PLACEMENT_3D('',#82727,#35549,#35550);
#29064=AXIS2_PLACEMENT_3D('',#82728,#35551,#35552);
#29065=AXIS2_PLACEMENT_3D('',#82729,#35553,#35554);
#29066=AXIS2_PLACEMENT_3D('',#82735,#35558,#35559);
#29067=AXIS2_PLACEMENT_3D('',#82739,#35562,#35563);
#29068=AXIS2_PLACEMENT_3D('',#82740,#35564,#35565);
#29069=AXIS2_PLACEMENT_3D('',#82741,#35566,#35567);
#29070=AXIS2_PLACEMENT_3D('',#82747,#35571,#35572);
#29071=AXIS2_PLACEMENT_3D('',#82751,#35575,#35576);
#29072=AXIS2_PLACEMENT_3D('',#82752,#35577,#35578);
#29073=AXIS2_PLACEMENT_3D('',#82753,#35579,#35580);
#29074=AXIS2_PLACEMENT_3D('',#82759,#35584,#35585);
#29075=AXIS2_PLACEMENT_3D('',#82763,#35588,#35589);
#29076=AXIS2_PLACEMENT_3D('',#82765,#35590,#35591);
#29077=AXIS2_PLACEMENT_3D('',#82766,#35592,#35593);
#29078=AXIS2_PLACEMENT_3D('',#82767,#35594,#35595);
#29079=AXIS2_PLACEMENT_3D('',#82773,#35599,#35600);
#29080=AXIS2_PLACEMENT_3D('',#82777,#35603,#35604);
#29081=AXIS2_PLACEMENT_3D('',#82778,#35605,#35606);
#29082=AXIS2_PLACEMENT_3D('',#82779,#35607,#35608);
#29083=AXIS2_PLACEMENT_3D('',#82785,#35612,#35613);
#29084=AXIS2_PLACEMENT_3D('',#82789,#35616,#35617);
#29085=AXIS2_PLACEMENT_3D('',#82790,#35618,#35619);
#29086=AXIS2_PLACEMENT_3D('',#82791,#35620,#35621);
#29087=AXIS2_PLACEMENT_3D('',#82797,#35625,#35626);
#29088=AXIS2_PLACEMENT_3D('',#82801,#35629,#35630);
#29089=AXIS2_PLACEMENT_3D('',#82802,#35631,#35632);
#29090=AXIS2_PLACEMENT_3D('',#82803,#35633,#35634);
#29091=AXIS2_PLACEMENT_3D('',#82809,#35638,#35639);
#29092=AXIS2_PLACEMENT_3D('',#82813,#35642,#35643);
#29093=AXIS2_PLACEMENT_3D('',#82814,#35644,#35645);
#29094=AXIS2_PLACEMENT_3D('',#82815,#35646,#35647);
#29095=AXIS2_PLACEMENT_3D('',#82821,#35651,#35652);
#29096=AXIS2_PLACEMENT_3D('',#82825,#35655,#35656);
#29097=AXIS2_PLACEMENT_3D('',#82826,#35657,#35658);
#29098=AXIS2_PLACEMENT_3D('',#82827,#35659,#35660);
#29099=AXIS2_PLACEMENT_3D('',#82833,#35664,#35665);
#29100=AXIS2_PLACEMENT_3D('',#82837,#35668,#35669);
#29101=AXIS2_PLACEMENT_3D('',#82838,#35670,#35671);
#29102=AXIS2_PLACEMENT_3D('',#82839,#35672,#35673);
#29103=AXIS2_PLACEMENT_3D('',#82845,#35677,#35678);
#29104=AXIS2_PLACEMENT_3D('',#82849,#35681,#35682);
#29105=AXIS2_PLACEMENT_3D('',#82850,#35683,#35684);
#29106=AXIS2_PLACEMENT_3D('',#82851,#35685,#35686);
#29107=AXIS2_PLACEMENT_3D('',#82857,#35690,#35691);
#29108=AXIS2_PLACEMENT_3D('',#82861,#35694,#35695);
#29109=AXIS2_PLACEMENT_3D('',#82862,#35696,#35697);
#29110=AXIS2_PLACEMENT_3D('',#82863,#35698,#35699);
#29111=AXIS2_PLACEMENT_3D('',#82869,#35703,#35704);
#29112=AXIS2_PLACEMENT_3D('',#82873,#35707,#35708);
#29113=AXIS2_PLACEMENT_3D('',#82874,#35709,#35710);
#29114=AXIS2_PLACEMENT_3D('',#82875,#35711,#35712);
#29115=AXIS2_PLACEMENT_3D('',#82881,#35716,#35717);
#29116=AXIS2_PLACEMENT_3D('',#82885,#35720,#35721);
#29117=AXIS2_PLACEMENT_3D('',#82886,#35722,#35723);
#29118=AXIS2_PLACEMENT_3D('',#82887,#35724,#35725);
#29119=AXIS2_PLACEMENT_3D('',#82893,#35729,#35730);
#29120=AXIS2_PLACEMENT_3D('',#82897,#35733,#35734);
#29121=AXIS2_PLACEMENT_3D('',#82898,#35735,#35736);
#29122=AXIS2_PLACEMENT_3D('',#82899,#35737,#35738);
#29123=AXIS2_PLACEMENT_3D('',#82905,#35742,#35743);
#29124=AXIS2_PLACEMENT_3D('',#82909,#35746,#35747);
#29125=AXIS2_PLACEMENT_3D('',#82910,#35748,#35749);
#29126=AXIS2_PLACEMENT_3D('',#82911,#35750,#35751);
#29127=AXIS2_PLACEMENT_3D('',#82917,#35755,#35756);
#29128=AXIS2_PLACEMENT_3D('',#82921,#35759,#35760);
#29129=AXIS2_PLACEMENT_3D('',#82922,#35761,#35762);
#29130=AXIS2_PLACEMENT_3D('',#82923,#35763,#35764);
#29131=AXIS2_PLACEMENT_3D('',#82929,#35768,#35769);
#29132=AXIS2_PLACEMENT_3D('',#82933,#35772,#35773);
#29133=AXIS2_PLACEMENT_3D('',#82934,#35774,#35775);
#29134=AXIS2_PLACEMENT_3D('',#82935,#35776,#35777);
#29135=AXIS2_PLACEMENT_3D('',#82941,#35781,#35782);
#29136=AXIS2_PLACEMENT_3D('',#82945,#35785,#35786);
#29137=AXIS2_PLACEMENT_3D('',#82946,#35787,#35788);
#29138=AXIS2_PLACEMENT_3D('',#82947,#35789,#35790);
#29139=AXIS2_PLACEMENT_3D('',#82953,#35794,#35795);
#29140=AXIS2_PLACEMENT_3D('',#82957,#35798,#35799);
#29141=AXIS2_PLACEMENT_3D('',#82958,#35800,#35801);
#29142=AXIS2_PLACEMENT_3D('',#82959,#35802,#35803);
#29143=AXIS2_PLACEMENT_3D('',#82965,#35807,#35808);
#29144=AXIS2_PLACEMENT_3D('',#82969,#35811,#35812);
#29145=AXIS2_PLACEMENT_3D('',#82970,#35813,#35814);
#29146=AXIS2_PLACEMENT_3D('',#82971,#35815,#35816);
#29147=AXIS2_PLACEMENT_3D('',#82977,#35820,#35821);
#29148=AXIS2_PLACEMENT_3D('',#82981,#35824,#35825);
#29149=AXIS2_PLACEMENT_3D('',#82982,#35826,#35827);
#29150=AXIS2_PLACEMENT_3D('',#82983,#35828,#35829);
#29151=AXIS2_PLACEMENT_3D('',#82985,#35831,#35832);
#29152=AXIS2_PLACEMENT_3D('',#82998,#35839,#35840);
#29153=AXIS2_PLACEMENT_3D('',#83002,#35842,#35843);
#29154=AXIS2_PLACEMENT_3D('',#83003,#35844,#35845);
#29155=AXIS2_PLACEMENT_3D('',#83006,#35847,#35848);
#29156=AXIS2_PLACEMENT_3D('',#83007,#35849,#35850);
#29157=AXIS2_PLACEMENT_3D('',#83010,#35852,#35853);
#29158=AXIS2_PLACEMENT_3D('',#83011,#35854,#35855);
#29159=AXIS2_PLACEMENT_3D('',#83014,#35857,#35858);
#29160=AXIS2_PLACEMENT_3D('',#83015,#35859,#35860);
#29161=AXIS2_PLACEMENT_3D('',#83018,#35862,#35863);
#29162=AXIS2_PLACEMENT_3D('',#83019,#35864,#35865);
#29163=AXIS2_PLACEMENT_3D('',#83021,#35867,#35868);
#29164=AXIS2_PLACEMENT_3D('',#83022,#35869,#35870);
#29165=AXIS2_PLACEMENT_3D('',#83025,#35872,#35873);
#29166=AXIS2_PLACEMENT_3D('',#83028,#35876,#35877);
#29167=AXIS2_PLACEMENT_3D('',#83030,#35879,#35880);
#29168=AXIS2_PLACEMENT_3D('',#83032,#35882,#35883);
#29169=AXIS2_PLACEMENT_3D('',#83034,#35885,#35886);
#29170=AXIS2_PLACEMENT_3D('',#83036,#35888,#35889);
#35181=DIRECTION('axis',(0.,0.,1.));
#35182=DIRECTION('refdir',(1.,0.,0.));
#35183=DIRECTION('center_axis',(0.,-1.,0.));
#35184=DIRECTION('ref_axis',(0.653824539037156,0.,-0.756646200117896));
#35185=DIRECTION('',(0.,1.,0.));
#35186=DIRECTION('center_axis',(0.,1.,0.));
#35187=DIRECTION('ref_axis',(1.,0.,1.17141641968325E-13));
#35188=DIRECTION('center_axis',(0.,-1.,0.));
#35189=DIRECTION('ref_axis',(0.653824539037156,0.,-0.756646200117896));
#35190=DIRECTION('',(0.,1.,0.));
#35191=DIRECTION('center_axis',(0.,-1.,0.));
#35192=DIRECTION('ref_axis',(0.653824539037156,0.,-0.756646200117896));
#35193=DIRECTION('',(0.,1.,0.));
#35194=DIRECTION('center_axis',(0.,-1.,0.));
#35195=DIRECTION('ref_axis',(0.653824539037156,0.,-0.756646200117896));
#35196=DIRECTION('',(0.,1.,0.));
#35197=DIRECTION('center_axis',(0.,-1.,0.));
#35198=DIRECTION('ref_axis',(0.653824539037156,0.,-0.756646200117896));
#35199=DIRECTION('',(0.,1.,0.));
#35200=DIRECTION('center_axis',(0.,-1.,0.));
#35201=DIRECTION('ref_axis',(0.653824539037156,0.,-0.756646200117896));
#35202=DIRECTION('',(0.,1.,0.));
#35203=DIRECTION('center_axis',(0.,-1.,0.));
#35204=DIRECTION('ref_axis',(0.653824539037156,0.,-0.756646200117896));
#35205=DIRECTION('',(0.,1.,0.));
#35206=DIRECTION('center_axis',(0.,-1.,0.));
#35207=DIRECTION('ref_axis',(0.653824539037156,0.,-0.756646200117896));
#35208=DIRECTION('',(0.,1.,0.));
#35209=DIRECTION('center_axis',(0.,-1.,0.));
#35210=DIRECTION('ref_axis',(0.653824539037156,0.,-0.756646200117896));
#35211=DIRECTION('',(0.,1.,0.));
#35212=DIRECTION('center_axis',(0.,-1.,0.));
#35213=DIRECTION('ref_axis',(0.653824539037156,0.,-0.756646200117896));
#35214=DIRECTION('',(0.,1.,0.));
#35215=DIRECTION('center_axis',(0.,-1.,0.));
#35216=DIRECTION('ref_axis',(0.653824539037156,0.,-0.756646200117896));
#35217=DIRECTION('',(0.,1.,0.));
#35218=DIRECTION('center_axis',(0.,-1.,0.));
#35219=DIRECTION('ref_axis',(0.653824539037156,0.,-0.756646200117896));
#35220=DIRECTION('',(0.,1.,0.));
#35221=DIRECTION('center_axis',(0.,-1.,0.));
#35222=DIRECTION('ref_axis',(0.653824539037156,0.,-0.756646200117896));
#35223=DIRECTION('',(0.,1.,0.));
#35224=DIRECTION('center_axis',(0.,-1.,0.));
#35225=DIRECTION('ref_axis',(0.653824539037156,0.,-0.756646200117896));
#35226=DIRECTION('',(0.,1.,0.));
#35227=DIRECTION('center_axis',(0.,-1.,0.));
#35228=DIRECTION('ref_axis',(0.653824539037156,0.,-0.756646200117896));
#35229=DIRECTION('',(0.,1.,0.));
#35230=DIRECTION('center_axis',(0.,-1.,0.));
#35231=DIRECTION('ref_axis',(0.653824539037156,0.,-0.756646200117896));
#35232=DIRECTION('',(0.,1.,0.));
#35233=DIRECTION('center_axis',(0.,-1.,0.));
#35234=DIRECTION('ref_axis',(0.653824539037156,0.,-0.756646200117896));
#35235=DIRECTION('',(0.,1.,0.));
#35236=DIRECTION('center_axis',(0.,-1.,0.));
#35237=DIRECTION('ref_axis',(0.653824539037156,0.,-0.756646200117896));
#35238=DIRECTION('',(0.,1.,0.));
#35239=DIRECTION('center_axis',(0.,-1.,0.));
#35240=DIRECTION('ref_axis',(0.653824539037156,0.,-0.756646200117896));
#35241=DIRECTION('',(0.,1.,0.));
#35242=DIRECTION('center_axis',(0.,-1.,0.));
#35243=DIRECTION('ref_axis',(1.,0.,0.));
#35244=DIRECTION('center_axis',(0.,1.,0.));
#35245=DIRECTION('ref_axis',(1.,0.,0.));
#35246=DIRECTION('center_axis',(0.,-1.,0.));
#35247=DIRECTION('ref_axis',(1.,0.,0.));
#35248=DIRECTION('center_axis',(0.,-1.,0.));
#35249=DIRECTION('ref_axis',(0.653824539037156,0.,-0.756646200117896));
#35250=DIRECTION('center_axis',(0.,-1.,0.));
#35251=DIRECTION('ref_axis',(1.,0.,1.17141641968325E-13));
#35252=DIRECTION('center_axis',(0.,1.,0.));
#35253=DIRECTION('ref_axis',(0.,0.,1.));
#35254=DIRECTION('center_axis',(0.,-1.,0.));
#35255=DIRECTION('ref_axis',(1.,0.,0.));
#35256=DIRECTION('center_axis',(0.,-1.,0.));
#35257=DIRECTION('ref_axis',(1.,0.,0.));
#35258=DIRECTION('center_axis',(0.,1.,0.));
#35259=DIRECTION('ref_axis',(0.,0.,1.));
#35260=DIRECTION('center_axis',(0.,1.,0.));
#35261=DIRECTION('ref_axis',(1.,0.,0.));
#35262=DIRECTION('center_axis',(0.,1.,0.));
#35263=DIRECTION('ref_axis',(1.,0.,0.));
#35264=DIRECTION('center_axis',(0.,1.,0.));
#35265=DIRECTION('ref_axis',(0.,0.,1.));
#35266=DIRECTION('center_axis',(0.,-1.,0.));
#35267=DIRECTION('ref_axis',(1.,0.,0.));
#35268=DIRECTION('center_axis',(1.,0.,0.));
#35269=DIRECTION('ref_axis',(0.,0.,-1.));
#35270=DIRECTION('center_axis',(0.,1.,0.));
#35271=DIRECTION('ref_axis',(1.,0.,0.));
#35272=DIRECTION('center_axis',(0.,1.,0.));
#35273=DIRECTION('ref_axis',(1.,0.,0.));
#35274=DIRECTION('center_axis',(0.,1.,0.));
#35275=DIRECTION('ref_axis',(1.,0.,0.));
#35276=DIRECTION('',(0.707106781186547,-0.707106781186548,-8.65956056235493E-17));
#35277=DIRECTION('center_axis',(0.,1.,0.));
#35278=DIRECTION('ref_axis',(1.,0.,0.));
#35279=DIRECTION('center_axis',(0.,1.,0.));
#35280=DIRECTION('ref_axis',(1.,0.,0.));
#35281=DIRECTION('center_axis',(-0.188314866426199,0.,0.982108706347155));
#35282=DIRECTION('ref_axis',(-0.982108706347155,0.,-0.188314866426199));
#35283=DIRECTION('',(0.,1.,0.));
#35284=DIRECTION('',(-0.982108706347155,0.,-0.188314866426199));
#35285=DIRECTION('',(0.,-1.,0.));
#35286=DIRECTION('center_axis',(-0.512859050871225,0.,-0.858472826558573));
#35287=DIRECTION('ref_axis',(0.858472826558573,0.,-0.512859050871225));
#35288=DIRECTION('',(0.,-1.,0.));
#35289=DIRECTION('',(0.858472826558573,0.,-0.512859050871225));
#35290=DIRECTION('center_axis',(0.,-1.,0.));
#35291=DIRECTION('ref_axis',(-0.17364817766693,0.,-0.984807753012208));
#35292=DIRECTION('center_axis',(0.,-1.,0.));
#35293=DIRECTION('ref_axis',(1.,0.,0.));
#35294=DIRECTION('center_axis',(0.,-1.,0.));
#35295=DIRECTION('ref_axis',(1.,0.,0.));
#35296=DIRECTION('center_axis',(0.,1.,0.));
#35297=DIRECTION('ref_axis',(1.,0.,0.));
#35298=DIRECTION('center_axis',(0.,1.,0.));
#35299=DIRECTION('ref_axis',(1.,0.,0.));
#35300=DIRECTION('center_axis',(0.,1.,0.));
#35301=DIRECTION('ref_axis',(1.,0.,0.));
#35302=DIRECTION('center_axis',(0.,1.,0.));
#35303=DIRECTION('ref_axis',(1.,0.,0.));
#35304=DIRECTION('center_axis',(0.,1.,0.));
#35305=DIRECTION('ref_axis',(1.,0.,0.));
#35306=DIRECTION('center_axis',(0.,1.,0.));
#35307=DIRECTION('ref_axis',(1.,0.,0.));
#35308=DIRECTION('center_axis',(0.,1.,0.));
#35309=DIRECTION('ref_axis',(1.,0.,0.));
#35310=DIRECTION('center_axis',(0.,1.,0.));
#35311=DIRECTION('ref_axis',(1.,0.,0.));
#35312=DIRECTION('center_axis',(0.,1.,0.));
#35313=DIRECTION('ref_axis',(1.,0.,0.));
#35314=DIRECTION('center_axis',(0.,1.,0.));
#35315=DIRECTION('ref_axis',(1.,0.,0.));
#35316=DIRECTION('center_axis',(0.,1.,0.));
#35317=DIRECTION('ref_axis',(1.,0.,0.));
#35318=DIRECTION('center_axis',(0.,1.,0.));
#35319=DIRECTION('ref_axis',(1.,0.,0.));
#35320=DIRECTION('center_axis',(0.,1.,0.));
#35321=DIRECTION('ref_axis',(1.,0.,0.));
#35322=DIRECTION('center_axis',(0.,1.,0.));
#35323=DIRECTION('ref_axis',(1.,0.,0.));
#35324=DIRECTION('center_axis',(0.,1.,0.));
#35325=DIRECTION('ref_axis',(1.,0.,0.));
#35326=DIRECTION('center_axis',(0.,1.,0.));
#35327=DIRECTION('ref_axis',(1.,0.,0.));
#35328=DIRECTION('center_axis',(0.,1.,0.));
#35329=DIRECTION('ref_axis',(1.,0.,0.));
#35330=DIRECTION('center_axis',(0.,1.,0.));
#35331=DIRECTION('ref_axis',(1.,0.,0.));
#35332=DIRECTION('center_axis',(0.,1.,0.));
#35333=DIRECTION('ref_axis',(1.,0.,0.));
#35334=DIRECTION('center_axis',(0.,1.,0.));
#35335=DIRECTION('ref_axis',(1.,0.,0.));
#35336=DIRECTION('center_axis',(0.,1.,0.));
#35337=DIRECTION('ref_axis',(1.,0.,0.));
#35338=DIRECTION('center_axis',(0.,1.,0.));
#35339=DIRECTION('ref_axis',(1.,0.,0.));
#35340=DIRECTION('center_axis',(0.,1.,0.));
#35341=DIRECTION('ref_axis',(1.,0.,0.));
#35342=DIRECTION('center_axis',(0.,1.,0.));
#35343=DIRECTION('ref_axis',(1.,0.,0.));
#35344=DIRECTION('center_axis',(0.,1.,0.));
#35345=DIRECTION('ref_axis',(1.,0.,0.));
#35346=DIRECTION('center_axis',(0.,1.,0.));
#35347=DIRECTION('ref_axis',(1.,0.,0.));
#35348=DIRECTION('center_axis',(0.,1.,0.));
#35349=DIRECTION('ref_axis',(1.,0.,0.));
#35350=DIRECTION('center_axis',(0.,1.,0.));
#35351=DIRECTION('ref_axis',(1.,0.,0.));
#35352=DIRECTION('center_axis',(0.,1.,0.));
#35353=DIRECTION('ref_axis',(1.,0.,0.));
#35354=DIRECTION('center_axis',(0.,1.,0.));
#35355=DIRECTION('ref_axis',(1.,0.,0.));
#35356=DIRECTION('center_axis',(0.,1.,0.));
#35357=DIRECTION('ref_axis',(1.,0.,0.));
#35358=DIRECTION('center_axis',(0.,1.,0.));
#35359=DIRECTION('ref_axis',(1.,0.,0.));
#35360=DIRECTION('center_axis',(0.,1.,0.));
#35361=DIRECTION('ref_axis',(1.,0.,0.));
#35362=DIRECTION('center_axis',(0.,1.,0.));
#35363=DIRECTION('ref_axis',(1.,0.,0.));
#35364=DIRECTION('center_axis',(0.,1.,0.));
#35365=DIRECTION('ref_axis',(1.,0.,0.));
#35366=DIRECTION('center_axis',(0.,1.,0.));
#35367=DIRECTION('ref_axis',(1.,0.,0.));
#35368=DIRECTION('',(0.707106781186537,0.707106781186558,8.65956056235481E-17));
#35369=DIRECTION('center_axis',(0.,-1.,0.));
#35370=DIRECTION('ref_axis',(1.,0.,0.));
#35371=DIRECTION('center_axis',(-0.0149125533359689,0.,0.999888801693969));
#35372=DIRECTION('ref_axis',(-0.999888801693969,0.,-0.0149125533359689));
#35373=DIRECTION('',(0.,1.,0.));
#35374=DIRECTION('',(-0.999888801693969,0.,-0.0149125533359689));
#35375=DIRECTION('',(0.,-1.,0.));
#35376=DIRECTION('center_axis',(-0.65413981140894,0.,-0.756373655761408));
#35377=DIRECTION('ref_axis',(0.756373655761408,0.,-0.65413981140894));
#35378=DIRECTION('',(0.,-1.,0.));
#35379=DIRECTION('',(0.756373655761408,0.,-0.65413981140894));
#35380=DIRECTION('center_axis',(0.,-1.,0.));
#35381=DIRECTION('ref_axis',(-0.342020143325669,0.,-0.939692620785908));
#35382=DIRECTION('center_axis',(0.,-1.,0.));
#35383=DIRECTION('ref_axis',(1.,0.,0.));
#35384=DIRECTION('center_axis',(0.158942870141258,0.,0.987287781769459));
#35385=DIRECTION('ref_axis',(-0.987287781769459,0.,0.158942870141258));
#35386=DIRECTION('',(0.,1.,0.));
#35387=DIRECTION('',(-0.987287781769459,0.,0.158942870141258));
#35388=DIRECTION('',(0.,-1.,0.));
#35389=DIRECTION('center_axis',(-0.77554486478771,0.,-0.631292454177469));
#35390=DIRECTION('ref_axis',(0.631292454177469,0.,-0.77554486478771));
#35391=DIRECTION('',(0.,-1.,0.));
#35392=DIRECTION('',(0.631292454177469,0.,-0.77554486478771));
#35393=DIRECTION('center_axis',(0.,-1.,0.));
#35394=DIRECTION('ref_axis',(-0.5,0.,-0.866025403784438));
#35395=DIRECTION('center_axis',(0.,-1.,0.));
#35396=DIRECTION('ref_axis',(1.,0.,0.));
#35397=DIRECTION('center_axis',(0.327968894938216,0.,0.944688522187607));
#35398=DIRECTION('ref_axis',(-0.944688522187607,0.,0.327968894938216));
#35399=DIRECTION('',(0.,1.,0.));
#35400=DIRECTION('',(-0.944688522187607,0.,0.327968894938216));
#35401=DIRECTION('',(0.,-1.,0.));
#35402=DIRECTION('center_axis',(-0.873385379894543,0.,-0.487029750822744));
#35403=DIRECTION('ref_axis',(0.487029750822744,0.,-0.873385379894543));
#35404=DIRECTION('',(0.,-1.,0.));
#35405=DIRECTION('',(0.487029750822744,0.,-0.873385379894543));
#35406=DIRECTION('center_axis',(0.,-1.,0.));
#35407=DIRECTION('ref_axis',(-0.64278760968654,0.,-0.766044443118978));
#35408=DIRECTION('center_axis',(0.,-1.,0.));
#35409=DIRECTION('ref_axis',(1.,0.,0.));
#35410=DIRECTION('center_axis',(0.487029750822745,0.,0.873385379894543));
#35411=DIRECTION('ref_axis',(-0.873385379894543,0.,0.487029750822745));
#35412=DIRECTION('',(0.,1.,0.));
#35413=DIRECTION('',(-0.873385379894543,0.,0.487029750822745));
#35414=DIRECTION('',(0.,-1.,0.));
#35415=DIRECTION('center_axis',(-0.944688522187607,0.,-0.327968894938216));
#35416=DIRECTION('ref_axis',(0.327968894938216,0.,-0.944688522187607));
#35417=DIRECTION('',(0.,-1.,0.));
#35418=DIRECTION('',(0.327968894938216,0.,-0.944688522187607));
#35419=DIRECTION('center_axis',(0.,-1.,0.));
#35420=DIRECTION('ref_axis',(-0.766044443118978,0.,-0.642787609686539));
#35421=DIRECTION('center_axis',(0.,-1.,0.));
#35422=DIRECTION('ref_axis',(1.,0.,0.));
#35423=DIRECTION('center_axis',(0.63129245417747,0.,0.77554486478771));
#35424=DIRECTION('ref_axis',(-0.77554486478771,0.,0.63129245417747));
#35425=DIRECTION('',(0.,1.,0.));
#35426=DIRECTION('',(-0.77554486478771,0.,0.63129245417747));
#35427=DIRECTION('',(0.,-1.,0.));
#35428=DIRECTION('center_axis',(-0.987287781769459,0.,-0.158942870141258));
#35429=DIRECTION('ref_axis',(0.158942870141258,0.,-0.987287781769459));
#35430=DIRECTION('',(0.,-1.,0.));
#35431=DIRECTION('',(0.158942870141258,0.,-0.987287781769459));
#35432=DIRECTION('center_axis',(0.,-1.,0.));
#35433=DIRECTION('ref_axis',(-0.866025403784439,0.,-0.5));
#35434=DIRECTION('center_axis',(0.,-1.,0.));
#35435=DIRECTION('ref_axis',(1.,0.,0.));
#35436=DIRECTION('center_axis',(0.756373655761408,0.,0.654139811408939));
#35437=DIRECTION('ref_axis',(-0.654139811408939,0.,0.756373655761408));
#35438=DIRECTION('',(0.,1.,0.));
#35439=DIRECTION('',(-0.654139811408939,0.,0.756373655761408));
#35440=DIRECTION('',(0.,-1.,0.));
#35441=DIRECTION('center_axis',(-0.999888801693969,0.,0.0149125533359702));
#35442=DIRECTION('ref_axis',(-0.0149125533359702,0.,-0.999888801693969));
#35443=DIRECTION('',(0.,-1.,0.));
#35444=DIRECTION('',(-0.0149125533359701,0.,-0.999888801693969));
#35445=DIRECTION('center_axis',(0.,-1.,0.));
#35446=DIRECTION('ref_axis',(-0.939692620785909,0.,-0.342020143325668));
#35447=DIRECTION('center_axis',(0.,-1.,0.));
#35448=DIRECTION('ref_axis',(1.,0.,0.));
#35449=DIRECTION('center_axis',(0.858472826558574,0.,0.512859050871224));
#35450=DIRECTION('ref_axis',(-0.512859050871224,0.,0.858472826558574));
#35451=DIRECTION('',(0.,1.,0.));
#35452=DIRECTION('',(-0.512859050871224,0.,0.858472826558574));
#35453=DIRECTION('',(0.,-1.,0.));
#35454=DIRECTION('center_axis',(-0.982108706347155,0.,0.1883148664262));
#35455=DIRECTION('ref_axis',(-0.1883148664262,0.,-0.982108706347155));
#35456=DIRECTION('',(0.,-1.,0.));
#35457=DIRECTION('',(-0.1883148664262,0.,-0.982108706347155));
#35458=DIRECTION('center_axis',(0.,-1.,0.));
#35459=DIRECTION('ref_axis',(-0.984807753012208,0.,-0.17364817766693));
#35460=DIRECTION('center_axis',(0.,-1.,0.));
#35461=DIRECTION('ref_axis',(1.,0.,0.));
#35462=DIRECTION('center_axis',(0.934487734928968,0.,0.355995327591989));
#35463=DIRECTION('ref_axis',(-0.355995327591989,0.,0.934487734928968));
#35464=DIRECTION('',(0.,1.,0.));
#35465=DIRECTION('',(-0.355995327591989,0.,0.934487734928968));
#35466=DIRECTION('',(0.,-1.,0.));
#35467=DIRECTION('center_axis',(-0.934487734928967,0.,0.35599532759199));
#35468=DIRECTION('ref_axis',(-0.35599532759199,0.,-0.934487734928967));
#35469=DIRECTION('',(0.,-1.,0.));
#35470=DIRECTION('',(-0.35599532759199,0.,-0.934487734928967));
#35471=DIRECTION('center_axis',(0.,-1.,0.));
#35472=DIRECTION('ref_axis',(-1.,0.,1.83697019872103E-16));
#35473=DIRECTION('center_axis',(0.,-1.,0.));
#35474=DIRECTION('ref_axis',(1.,0.,0.));
#35475=DIRECTION('center_axis',(0.982108706347155,0.,0.188314866426199));
#35476=DIRECTION('ref_axis',(-0.188314866426199,0.,0.982108706347155));
#35477=DIRECTION('',(0.,1.,0.));
#35478=DIRECTION('',(-0.188314866426199,0.,0.982108706347155));
#35479=DIRECTION('',(0.,-1.,0.));
#35480=DIRECTION('center_axis',(-0.858472826558574,0.,0.512859050871225));
#35481=DIRECTION('ref_axis',(-0.512859050871225,0.,-0.858472826558573));
#35482=DIRECTION('',(0.,-1.,0.));
#35483=DIRECTION('',(-0.512859050871225,0.,-0.858472826558573));
#35484=DIRECTION('center_axis',(0.,-1.,0.));
#35485=DIRECTION('ref_axis',(-0.984807753012208,0.,0.17364817766693));
#35486=DIRECTION('center_axis',(0.,-1.,0.));
#35487=DIRECTION('ref_axis',(1.,0.,0.));
#35488=DIRECTION('center_axis',(0.999888801693969,0.,0.0149125533359689));
#35489=DIRECTION('ref_axis',(-0.0149125533359689,0.,0.999888801693969));
#35490=DIRECTION('',(0.,1.,0.));
#35491=DIRECTION('',(-0.0149125533359689,0.,0.999888801693969));
#35492=DIRECTION('',(0.,-1.,0.));
#35493=DIRECTION('center_axis',(-0.756373655761408,0.,0.65413981140894));
#35494=DIRECTION('ref_axis',(-0.65413981140894,0.,-0.756373655761408));
#35495=DIRECTION('',(0.,-1.,0.));
#35496=DIRECTION('',(-0.65413981140894,0.,-0.756373655761408));
#35497=DIRECTION('center_axis',(0.,-1.,0.));
#35498=DIRECTION('ref_axis',(-0.939692620785908,0.,0.342020143325669));
#35499=DIRECTION('center_axis',(0.,-1.,0.));
#35500=DIRECTION('ref_axis',(1.,0.,0.));
#35501=DIRECTION('center_axis',(0.987287781769459,0.,-0.158942870141258));
#35502=DIRECTION('ref_axis',(0.158942870141258,0.,0.987287781769459));
#35503=DIRECTION('',(0.,1.,0.));
#35504=DIRECTION('',(0.158942870141258,0.,0.987287781769459));
#35505=DIRECTION('',(0.,-1.,0.));
#35506=DIRECTION('center_axis',(-0.631292454177469,0.,0.77554486478771));
#35507=DIRECTION('ref_axis',(-0.77554486478771,0.,-0.631292454177469));
#35508=DIRECTION('',(0.,-1.,0.));
#35509=DIRECTION('',(-0.77554486478771,0.,-0.631292454177469));
#35510=DIRECTION('center_axis',(0.,-1.,0.));
#35511=DIRECTION('ref_axis',(-0.866025403784438,0.,0.5));
#35512=DIRECTION('center_axis',(0.,-1.,0.));
#35513=DIRECTION('ref_axis',(1.,0.,0.));
#35514=DIRECTION('center_axis',(0.944688522187607,0.,-0.327968894938216));
#35515=DIRECTION('ref_axis',(0.327968894938216,0.,0.944688522187607));
#35516=DIRECTION('',(0.,1.,0.));
#35517=DIRECTION('',(0.327968894938216,0.,0.944688522187607));
#35518=DIRECTION('',(0.,-1.,0.));
#35519=DIRECTION('center_axis',(-0.487029750822744,0.,0.873385379894543));
#35520=DIRECTION('ref_axis',(-0.873385379894543,0.,-0.487029750822744));
#35521=DIRECTION('',(0.,-1.,0.));
#35522=DIRECTION('',(-0.873385379894543,0.,-0.487029750822744));
#35523=DIRECTION('center_axis',(0.,-1.,0.));
#35524=DIRECTION('ref_axis',(-0.766044443118978,0.,0.642787609686539));
#35525=DIRECTION('center_axis',(0.,-1.,0.));
#35526=DIRECTION('ref_axis',(1.,0.,0.));
#35527=DIRECTION('center_axis',(0.873385379894543,0.,-0.487029750822745));
#35528=DIRECTION('ref_axis',(0.487029750822745,0.,0.873385379894543));
#35529=DIRECTION('',(0.,1.,0.));
#35530=DIRECTION('',(0.487029750822745,0.,0.873385379894543));
#35531=DIRECTION('',(0.,-1.,0.));
#35532=DIRECTION('center_axis',(-0.327968894938216,0.,0.944688522187607));
#35533=DIRECTION('ref_axis',(-0.944688522187607,0.,-0.327968894938216));
#35534=DIRECTION('',(0.,-1.,0.));
#35535=DIRECTION('',(-0.944688522187607,0.,-0.327968894938216));
#35536=DIRECTION('center_axis',(0.,-1.,0.));
#35537=DIRECTION('ref_axis',(-0.642787609686539,0.,0.766044443118978));
#35538=DIRECTION('center_axis',(0.,-1.,0.));
#35539=DIRECTION('ref_axis',(1.,0.,0.));
#35540=DIRECTION('center_axis',(0.77554486478771,0.,-0.63129245417747));
#35541=DIRECTION('ref_axis',(0.63129245417747,0.,0.77554486478771));
#35542=DIRECTION('',(0.,1.,0.));
#35543=DIRECTION('',(0.63129245417747,0.,0.77554486478771));
#35544=DIRECTION('',(0.,-1.,0.));
#35545=DIRECTION('center_axis',(-0.158942870141257,0.,0.987287781769459));
#35546=DIRECTION('ref_axis',(-0.987287781769459,0.,-0.158942870141257));
#35547=DIRECTION('',(0.,-1.,0.));
#35548=DIRECTION('',(-0.987287781769459,0.,-0.158942870141257));
#35549=DIRECTION('center_axis',(0.,-1.,0.));
#35550=DIRECTION('ref_axis',(-0.5,0.,0.866025403784439));
#35551=DIRECTION('center_axis',(0.,-1.,0.));
#35552=DIRECTION('ref_axis',(1.,0.,0.));
#35553=DIRECTION('center_axis',(0.65413981140894,0.,-0.756373655761408));
#35554=DIRECTION('ref_axis',(0.756373655761408,0.,0.65413981140894));
#35555=DIRECTION('',(0.,1.,0.));
#35556=DIRECTION('',(0.756373655761408,0.,0.65413981140894));
#35557=DIRECTION('',(0.,-1.,0.));
#35558=DIRECTION('center_axis',(0.0149125533359697,0.,0.999888801693969));
#35559=DIRECTION('ref_axis',(-0.999888801693969,0.,0.0149125533359697));
#35560=DIRECTION('',(0.,-1.,0.));
#35561=DIRECTION('',(-0.999888801693969,0.,0.0149125533359697));
#35562=DIRECTION('center_axis',(0.,-1.,0.));
#35563=DIRECTION('ref_axis',(-0.342020143325669,0.,0.939692620785908));
#35564=DIRECTION('center_axis',(0.,-1.,0.));
#35565=DIRECTION('ref_axis',(1.,0.,0.));
#35566=DIRECTION('center_axis',(0.512859050871225,0.,-0.858472826558573));
#35567=DIRECTION('ref_axis',(0.858472826558573,0.,0.512859050871225));
#35568=DIRECTION('',(0.,1.,0.));
#35569=DIRECTION('',(0.858472826558574,0.,0.512859050871224));
#35570=DIRECTION('',(0.,-1.,0.));
#35571=DIRECTION('center_axis',(0.1883148664262,0.,0.982108706347155));
#35572=DIRECTION('ref_axis',(-0.982108706347155,0.,0.1883148664262));
#35573=DIRECTION('',(0.,-1.,0.));
#35574=DIRECTION('',(-0.982108706347155,0.,0.1883148664262));
#35575=DIRECTION('center_axis',(0.,-1.,0.));
#35576=DIRECTION('ref_axis',(-0.17364817766693,0.,0.984807753012208));
#35577=DIRECTION('center_axis',(0.,-1.,0.));
#35578=DIRECTION('ref_axis',(1.,0.,0.));
#35579=DIRECTION('center_axis',(0.355995327591989,0.,-0.934487734928968));
#35580=DIRECTION('ref_axis',(0.934487734928968,0.,0.355995327591989));
#35581=DIRECTION('',(0.,1.,0.));
#35582=DIRECTION('',(0.934487734928968,0.,0.355995327591989));
#35583=DIRECTION('',(0.,-1.,0.));
#35584=DIRECTION('center_axis',(0.35599532759199,0.,0.934487734928967));
#35585=DIRECTION('ref_axis',(-0.934487734928967,0.,0.35599532759199));
#35586=DIRECTION('',(0.,-1.,0.));
#35587=DIRECTION('',(-0.934487734928967,0.,0.35599532759199));
#35588=DIRECTION('center_axis',(0.,-1.,0.));
#35589=DIRECTION('ref_axis',(1.22464679914735E-16,0.,1.));
#35590=DIRECTION('center_axis',(0.,-1.,0.));
#35591=DIRECTION('ref_axis',(1.,0.,0.));
#35592=DIRECTION('center_axis',(0.,-1.,0.));
#35593=DIRECTION('ref_axis',(1.,0.,0.));
#35594=DIRECTION('center_axis',(0.188314866426199,0.,-0.982108706347155));
#35595=DIRECTION('ref_axis',(0.982108706347155,0.,0.188314866426199));
#35596=DIRECTION('',(0.,1.,0.));
#35597=DIRECTION('',(0.982108706347155,0.,0.188314866426199));
#35598=DIRECTION('',(0.,-1.,0.));
#35599=DIRECTION('center_axis',(0.512859050871225,0.,0.858472826558573));
#35600=DIRECTION('ref_axis',(-0.858472826558573,0.,0.512859050871225));
#35601=DIRECTION('',(0.,-1.,0.));
#35602=DIRECTION('',(-0.858472826558573,0.,0.512859050871225));
#35603=DIRECTION('center_axis',(0.,-1.,0.));
#35604=DIRECTION('ref_axis',(0.173648177666931,0.,0.984807753012208));
#35605=DIRECTION('center_axis',(0.,-1.,0.));
#35606=DIRECTION('ref_axis',(1.,0.,0.));
#35607=DIRECTION('center_axis',(0.0149125533359694,0.,-0.999888801693969));
#35608=DIRECTION('ref_axis',(0.999888801693969,0.,0.0149125533359694));
#35609=DIRECTION('',(0.,1.,0.));
#35610=DIRECTION('',(0.999888801693969,0.,0.0149125533359694));
#35611=DIRECTION('',(0.,-1.,0.));
#35612=DIRECTION('center_axis',(0.65413981140894,0.,0.756373655761408));
#35613=DIRECTION('ref_axis',(-0.756373655761408,0.,0.65413981140894));
#35614=DIRECTION('',(0.,-1.,0.));
#35615=DIRECTION('',(-0.756373655761408,0.,0.65413981140894));
#35616=DIRECTION('center_axis',(0.,-1.,0.));
#35617=DIRECTION('ref_axis',(0.342020143325669,0.,0.939692620785908));
#35618=DIRECTION('center_axis',(0.,-1.,0.));
#35619=DIRECTION('ref_axis',(1.,0.,0.));
#35620=DIRECTION('center_axis',(-0.158942870141257,0.,-0.987287781769459));
#35621=DIRECTION('ref_axis',(0.987287781769459,0.,-0.158942870141257));
#35622=DIRECTION('',(0.,1.,0.));
#35623=DIRECTION('',(0.987287781769459,0.,-0.158942870141257));
#35624=DIRECTION('',(0.,-1.,0.));
#35625=DIRECTION('center_axis',(0.77554486478771,0.,0.63129245417747));
#35626=DIRECTION('ref_axis',(-0.63129245417747,0.,0.77554486478771));
#35627=DIRECTION('',(0.,-1.,0.));
#35628=DIRECTION('',(-0.63129245417747,0.,0.77554486478771));
#35629=DIRECTION('center_axis',(0.,-1.,0.));
#35630=DIRECTION('ref_axis',(0.5,0.,0.866025403784439));
#35631=DIRECTION('center_axis',(0.,-1.,0.));
#35632=DIRECTION('ref_axis',(1.,0.,0.));
#35633=DIRECTION('center_axis',(-0.327968894938216,0.,-0.944688522187607));
#35634=DIRECTION('ref_axis',(0.944688522187607,0.,-0.327968894938216));
#35635=DIRECTION('',(0.,1.,0.));
#35636=DIRECTION('',(0.944688522187607,0.,-0.327968894938216));
#35637=DIRECTION('',(0.,-1.,0.));
#35638=DIRECTION('center_axis',(0.873385379894543,0.,0.487029750822744));
#35639=DIRECTION('ref_axis',(-0.487029750822744,0.,0.873385379894543));
#35640=DIRECTION('',(0.,-1.,0.));
#35641=DIRECTION('',(-0.487029750822744,0.,0.873385379894543));
#35642=DIRECTION('center_axis',(0.,-1.,0.));
#35643=DIRECTION('ref_axis',(0.642787609686539,0.,0.766044443118978));
#35644=DIRECTION('center_axis',(0.,-1.,0.));
#35645=DIRECTION('ref_axis',(1.,0.,0.));
#35646=DIRECTION('center_axis',(-0.487029750822745,0.,-0.873385379894543));
#35647=DIRECTION('ref_axis',(0.873385379894543,0.,-0.487029750822745));
#35648=DIRECTION('',(0.,1.,0.));
#35649=DIRECTION('',(0.873385379894543,0.,-0.487029750822745));
#35650=DIRECTION('',(0.,-1.,0.));
#35651=DIRECTION('center_axis',(0.944688522187607,0.,0.327968894938216));
#35652=DIRECTION('ref_axis',(-0.327968894938216,0.,0.944688522187607));
#35653=DIRECTION('',(0.,-1.,0.));
#35654=DIRECTION('',(-0.327968894938216,0.,0.944688522187607));
#35655=DIRECTION('center_axis',(0.,-1.,0.));
#35656=DIRECTION('ref_axis',(0.766044443118978,0.,0.642787609686539));
#35657=DIRECTION('center_axis',(0.,-1.,0.));
#35658=DIRECTION('ref_axis',(1.,0.,0.));
#35659=DIRECTION('center_axis',(-0.63129245417747,0.,-0.77554486478771));
#35660=DIRECTION('ref_axis',(0.77554486478771,0.,-0.63129245417747));
#35661=DIRECTION('',(0.,1.,0.));
#35662=DIRECTION('',(0.77554486478771,0.,-0.63129245417747));
#35663=DIRECTION('',(0.,-1.,0.));
#35664=DIRECTION('center_axis',(0.987287781769459,0.,0.158942870141257));
#35665=DIRECTION('ref_axis',(-0.158942870141257,0.,0.987287781769459));
#35666=DIRECTION('',(0.,-1.,0.));
#35667=DIRECTION('',(-0.158942870141257,0.,0.987287781769459));
#35668=DIRECTION('center_axis',(0.,-1.,0.));
#35669=DIRECTION('ref_axis',(0.866025403784439,0.,0.5));
#35670=DIRECTION('center_axis',(0.,-1.,0.));
#35671=DIRECTION('ref_axis',(1.,0.,0.));
#35672=DIRECTION('center_axis',(-0.756373655761408,0.,-0.65413981140894));
#35673=DIRECTION('ref_axis',(0.65413981140894,0.,-0.756373655761408));
#35674=DIRECTION('',(0.,1.,0.));
#35675=DIRECTION('',(0.65413981140894,0.,-0.756373655761408));
#35676=DIRECTION('',(0.,-1.,0.));
#35677=DIRECTION('center_axis',(0.999888801693969,0.,-0.0149125533359696));
#35678=DIRECTION('ref_axis',(0.0149125533359696,0.,0.999888801693969));
#35679=DIRECTION('',(0.,-1.,0.));
#35680=DIRECTION('',(0.0149125533359696,0.,0.999888801693969));
#35681=DIRECTION('center_axis',(0.,-1.,0.));
#35682=DIRECTION('ref_axis',(0.939692620785908,0.,0.342020143325669));
#35683=DIRECTION('center_axis',(0.,-1.,0.));
#35684=DIRECTION('ref_axis',(1.,0.,0.));
#35685=DIRECTION('center_axis',(-0.858472826558574,0.,-0.512859050871225));
#35686=DIRECTION('ref_axis',(0.512859050871225,0.,-0.858472826558573));
#35687=DIRECTION('',(0.,1.,0.));
#35688=DIRECTION('',(0.512859050871225,0.,-0.858472826558573));
#35689=DIRECTION('',(0.,-1.,0.));
#35690=DIRECTION('center_axis',(0.982108706347155,0.,-0.188314866426199));
#35691=DIRECTION('ref_axis',(0.188314866426199,0.,0.982108706347155));
#35692=DIRECTION('',(0.,-1.,0.));
#35693=DIRECTION('',(0.188314866426199,0.,0.982108706347155));
#35694=DIRECTION('center_axis',(0.,-1.,0.));
#35695=DIRECTION('ref_axis',(0.984807753012208,0.,0.17364817766693));
#35696=DIRECTION('center_axis',(0.,-1.,0.));
#35697=DIRECTION('ref_axis',(1.,0.,0.));
#35698=DIRECTION('center_axis',(-0.934487734928968,0.,-0.355995327591989));
#35699=DIRECTION('ref_axis',(0.355995327591989,0.,-0.934487734928968));
#35700=DIRECTION('',(0.,1.,0.));
#35701=DIRECTION('',(0.355995327591989,0.,-0.934487734928968));
#35702=DIRECTION('',(0.,-1.,0.));
#35703=DIRECTION('center_axis',(0.934487734928967,0.,-0.35599532759199));
#35704=DIRECTION('ref_axis',(0.35599532759199,0.,0.934487734928967));
#35705=DIRECTION('',(0.,-1.,0.));
#35706=DIRECTION('',(0.355995327591989,0.,0.934487734928968));
#35707=DIRECTION('center_axis',(0.,-1.,0.));
#35708=DIRECTION('ref_axis',(1.,0.,-6.12323399573677E-17));
#35709=DIRECTION('center_axis',(0.,-1.,0.));
#35710=DIRECTION('ref_axis',(1.,0.,0.));
#35711=DIRECTION('center_axis',(-0.982108706347155,0.,-0.188314866426199));
#35712=DIRECTION('ref_axis',(0.188314866426199,0.,-0.982108706347155));
#35713=DIRECTION('',(0.,1.,0.));
#35714=DIRECTION('',(0.188314866426199,0.,-0.982108706347155));
#35715=DIRECTION('',(0.,-1.,0.));
#35716=DIRECTION('center_axis',(0.858472826558573,0.,-0.512859050871225));
#35717=DIRECTION('ref_axis',(0.512859050871225,0.,0.858472826558573));
#35718=DIRECTION('',(0.,-1.,0.));
#35719=DIRECTION('',(0.512859050871225,0.,0.858472826558573));
#35720=DIRECTION('center_axis',(0.,-1.,0.));
#35721=DIRECTION('ref_axis',(0.984807753012208,0.,-0.17364817766693));
#35722=DIRECTION('center_axis',(0.,-1.,0.));
#35723=DIRECTION('ref_axis',(1.,0.,0.));
#35724=DIRECTION('center_axis',(-0.999888801693969,0.,-0.0149125533359695));
#35725=DIRECTION('ref_axis',(0.0149125533359695,0.,-0.999888801693969));
#35726=DIRECTION('',(0.,1.,0.));
#35727=DIRECTION('',(0.0149125533359695,0.,-0.999888801693969));
#35728=DIRECTION('',(0.,-1.,0.));
#35729=DIRECTION('center_axis',(0.756373655761408,0.,-0.65413981140894));
#35730=DIRECTION('ref_axis',(0.65413981140894,0.,0.756373655761408));
#35731=DIRECTION('',(0.,-1.,0.));
#35732=DIRECTION('',(0.65413981140894,0.,0.756373655761408));
#35733=DIRECTION('center_axis',(0.,-1.,0.));
#35734=DIRECTION('ref_axis',(0.939692620785908,0.,-0.342020143325669));
#35735=DIRECTION('center_axis',(0.,-1.,0.));
#35736=DIRECTION('ref_axis',(1.,0.,0.));
#35737=DIRECTION('center_axis',(-0.987287781769459,0.,0.158942870141258));
#35738=DIRECTION('ref_axis',(-0.158942870141258,0.,-0.987287781769459));
#35739=DIRECTION('',(0.,1.,0.));
#35740=DIRECTION('',(-0.158942870141258,0.,-0.987287781769459));
#35741=DIRECTION('',(0.,-1.,0.));
#35742=DIRECTION('center_axis',(0.63129245417747,0.,-0.77554486478771));
#35743=DIRECTION('ref_axis',(0.77554486478771,0.,0.63129245417747));
#35744=DIRECTION('',(0.,-1.,0.));
#35745=DIRECTION('',(0.77554486478771,0.,0.63129245417747));
#35746=DIRECTION('center_axis',(0.,-1.,0.));
#35747=DIRECTION('ref_axis',(0.866025403784439,0.,-0.5));
#35748=DIRECTION('center_axis',(0.,-1.,0.));
#35749=DIRECTION('ref_axis',(1.,0.,0.));
#35750=DIRECTION('center_axis',(-0.944688522187607,0.,0.327968894938216));
#35751=DIRECTION('ref_axis',(-0.327968894938216,0.,-0.944688522187607));
#35752=DIRECTION('',(0.,1.,0.));
#35753=DIRECTION('',(-0.327968894938216,0.,-0.944688522187607));
#35754=DIRECTION('',(0.,-1.,0.));
#35755=DIRECTION('center_axis',(0.487029750822745,0.,-0.873385379894543));
#35756=DIRECTION('ref_axis',(0.873385379894543,0.,0.487029750822745));
#35757=DIRECTION('',(0.,-1.,0.));
#35758=DIRECTION('',(0.873385379894543,0.,0.487029750822745));
#35759=DIRECTION('center_axis',(0.,-1.,0.));
#35760=DIRECTION('ref_axis',(0.766044443118978,0.,-0.642787609686539));
#35761=DIRECTION('center_axis',(0.,-1.,0.));
#35762=DIRECTION('ref_axis',(1.,0.,0.));
#35763=DIRECTION('center_axis',(-0.873385379894543,0.,0.487029750822745));
#35764=DIRECTION('ref_axis',(-0.487029750822745,0.,-0.873385379894543));
#35765=DIRECTION('',(0.,1.,0.));
#35766=DIRECTION('',(-0.487029750822745,0.,-0.873385379894543));
#35767=DIRECTION('',(0.,-1.,0.));
#35768=DIRECTION('center_axis',(0.327968894938216,0.,-0.944688522187607));
#35769=DIRECTION('ref_axis',(0.944688522187607,0.,0.327968894938216));
#35770=DIRECTION('',(0.,-1.,0.));
#35771=DIRECTION('',(0.944688522187607,0.,0.327968894938216));
#35772=DIRECTION('center_axis',(0.,-1.,0.));
#35773=DIRECTION('ref_axis',(0.642787609686539,0.,-0.766044443118978));
#35774=DIRECTION('center_axis',(0.,-1.,0.));
#35775=DIRECTION('ref_axis',(1.,0.,0.));
#35776=DIRECTION('center_axis',(-0.77554486478771,0.,0.63129245417747));
#35777=DIRECTION('ref_axis',(-0.63129245417747,0.,-0.77554486478771));
#35778=DIRECTION('',(0.,1.,0.));
#35779=DIRECTION('',(-0.63129245417747,0.,-0.77554486478771));
#35780=DIRECTION('',(0.,-1.,0.));
#35781=DIRECTION('center_axis',(0.158942870141257,0.,-0.987287781769459));
#35782=DIRECTION('ref_axis',(0.987287781769459,0.,0.158942870141257));
#35783=DIRECTION('',(0.,-1.,0.));
#35784=DIRECTION('',(0.987287781769459,0.,0.158942870141257));
#35785=DIRECTION('center_axis',(0.,-1.,0.));
#35786=DIRECTION('ref_axis',(0.5,0.,-0.866025403784439));
#35787=DIRECTION('center_axis',(0.,-1.,0.));
#35788=DIRECTION('ref_axis',(1.,0.,0.));
#35789=DIRECTION('center_axis',(-0.65413981140894,0.,0.756373655761408));
#35790=DIRECTION('ref_axis',(-0.756373655761408,0.,-0.65413981140894));
#35791=DIRECTION('',(0.,1.,0.));
#35792=DIRECTION('',(-0.756373655761408,0.,-0.65413981140894));
#35793=DIRECTION('',(0.,-1.,0.));
#35794=DIRECTION('center_axis',(-0.0149125533359696,0.,-0.999888801693969));
#35795=DIRECTION('ref_axis',(0.999888801693969,0.,-0.0149125533359696));
#35796=DIRECTION('',(0.,-1.,0.));
#35797=DIRECTION('',(0.999888801693969,0.,-0.0149125533359696));
#35798=DIRECTION('center_axis',(0.,-1.,0.));
#35799=DIRECTION('ref_axis',(0.342020143325669,0.,-0.939692620785908));
#35800=DIRECTION('center_axis',(0.,-1.,0.));
#35801=DIRECTION('ref_axis',(1.,0.,0.));
#35802=DIRECTION('center_axis',(-0.512859050871225,0.,0.858472826558573));
#35803=DIRECTION('ref_axis',(-0.858472826558573,0.,-0.512859050871225));
#35804=DIRECTION('',(0.,1.,0.));
#35805=DIRECTION('',(-0.858472826558573,0.,-0.512859050871225));
#35806=DIRECTION('',(0.,-1.,0.));
#35807=DIRECTION('center_axis',(-0.188314866426199,0.,-0.982108706347155));
#35808=DIRECTION('ref_axis',(0.982108706347155,0.,-0.188314866426199));
#35809=DIRECTION('',(0.,-1.,0.));
#35810=DIRECTION('',(0.982108706347155,0.,-0.188314866426199));
#35811=DIRECTION('center_axis',(0.,-1.,0.));
#35812=DIRECTION('ref_axis',(0.17364817766693,0.,-0.984807753012208));
#35813=DIRECTION('center_axis',(0.,-1.,0.));
#35814=DIRECTION('ref_axis',(1.,0.,0.));
#35815=DIRECTION('center_axis',(-0.355995327591989,0.,0.934487734928968));
#35816=DIRECTION('ref_axis',(-0.934487734928968,0.,-0.355995327591989));
#35817=DIRECTION('',(0.,1.,0.));
#35818=DIRECTION('',(-0.934487734928968,0.,-0.355995327591989));
#35819=DIRECTION('',(0.,-1.,0.));
#35820=DIRECTION('center_axis',(-0.355995327591989,0.,-0.934487734928968));
#35821=DIRECTION('ref_axis',(0.934487734928968,0.,-0.355995327591989));
#35822=DIRECTION('',(0.,-1.,0.));
#35823=DIRECTION('',(0.934487734928968,0.,-0.355995327591989));
#35824=DIRECTION('center_axis',(0.,-1.,0.));
#35825=DIRECTION('ref_axis',(0.,0.,-1.));
#35826=DIRECTION('center_axis',(0.,-1.,0.));
#35827=DIRECTION('ref_axis',(1.,0.,0.));
#35828=DIRECTION('center_axis',(0.,1.,0.));
#35829=DIRECTION('ref_axis',(1.,0.,0.));
#35830=DIRECTION('',(0.,-1.,0.));
#35831=DIRECTION('center_axis',(0.,1.,0.));
#35832=DIRECTION('ref_axis',(1.,0.,0.));
#35833=DIRECTION('',(0.499999999999998,0.,-0.86602540378444));
#35834=DIRECTION('',(1.,0.,0.));
#35835=DIRECTION('',(0.500000000000006,0.,0.866025403784435));
#35836=DIRECTION('',(-0.500000000000006,0.,0.866025403784435));
#35837=DIRECTION('',(-1.,0.,0.));
#35838=DIRECTION('',(-0.499999999999998,0.,-0.86602540378444));
#35839=DIRECTION('center_axis',(0.,1.,0.));
#35840=DIRECTION('ref_axis',(0.,0.,1.));
#35841=DIRECTION('',(0.499999999999998,0.,-0.86602540378444));
#35842=DIRECTION('center_axis',(0.,-1.,0.));
#35843=DIRECTION('ref_axis',(1.,0.,0.));
#35844=DIRECTION('center_axis',(0.,1.,0.));
#35845=DIRECTION('ref_axis',(0.,0.,1.));
#35846=DIRECTION('',(1.,0.,0.));
#35847=DIRECTION('center_axis',(0.,-1.,0.));
#35848=DIRECTION('ref_axis',(1.,0.,0.));
#35849=DIRECTION('center_axis',(0.,1.,0.));
#35850=DIRECTION('ref_axis',(0.,0.,1.));
#35851=DIRECTION('',(0.500000000000006,0.,0.866025403784435));
#35852=DIRECTION('center_axis',(0.,-1.,0.));
#35853=DIRECTION('ref_axis',(1.,0.,0.));
#35854=DIRECTION('center_axis',(0.,1.,0.));
#35855=DIRECTION('ref_axis',(0.,0.,1.));
#35856=DIRECTION('',(-0.500000000000006,0.,0.866025403784435));
#35857=DIRECTION('center_axis',(0.,-1.,0.));
#35858=DIRECTION('ref_axis',(1.,0.,0.));
#35859=DIRECTION('center_axis',(0.,1.,0.));
#35860=DIRECTION('ref_axis',(0.,0.,1.));
#35861=DIRECTION('',(-1.,0.,0.));
#35862=DIRECTION('center_axis',(0.,-1.,0.));
#35863=DIRECTION('ref_axis',(1.,0.,0.));
#35864=DIRECTION('center_axis',(0.,1.,0.));
#35865=DIRECTION('ref_axis',(0.,0.,1.));
#35866=DIRECTION('',(-0.499999999999998,0.,-0.86602540378444));
#35867=DIRECTION('center_axis',(0.,-1.,0.));
#35868=DIRECTION('ref_axis',(1.,0.,0.));
#35869=DIRECTION('center_axis',(0.,1.,0.));
#35870=DIRECTION('ref_axis',(1.,0.,0.));
#35871=DIRECTION('',(-0.857167300702115,0.515038074910049,1.04972719113862E-16));
#35872=DIRECTION('center_axis',(-0.86602540378444,0.,-0.499999999999998));
#35873=DIRECTION('ref_axis',(0.499999999999998,0.,-0.86602540378444));
#35874=DIRECTION('',(0.,-1.,0.));
#35875=DIRECTION('',(0.,-1.,0.));
#35876=DIRECTION('center_axis',(-0.86602540378444,0.,0.499999999999998));
#35877=DIRECTION('ref_axis',(-0.499999999999998,0.,-0.86602540378444));
#35878=DIRECTION('',(0.,-1.,0.));
#35879=DIRECTION('center_axis',(0.,0.,1.));
#35880=DIRECTION('ref_axis',(-1.,0.,0.));
#35881=DIRECTION('',(0.,-1.,0.));
#35882=DIRECTION('center_axis',(0.866025403784435,0.,0.500000000000006));
#35883=DIRECTION('ref_axis',(-0.500000000000006,0.,0.866025403784435));
#35884=DIRECTION('',(0.,-1.,0.));
#35885=DIRECTION('center_axis',(0.866025403784435,0.,-0.500000000000006));
#35886=DIRECTION('ref_axis',(0.500000000000006,0.,0.866025403784435));
#35887=DIRECTION('',(0.,-1.,0.));
#35888=DIRECTION('center_axis',(0.,0.,-1.));
#35889=DIRECTION('ref_axis',(1.,0.,0.));
#66836=CARTESIAN_POINT('',(0.,0.,0.));
#66837=CARTESIAN_POINT('Origin',(88.011,66.41344859951,12.066));
#66838=CARTESIAN_POINT('',(87.1806428355035,64.3667534988952,13.0269406742195));
#66839=CARTESIAN_POINT('',(87.1806426736235,64.5371153383989,13.0269405343375));
#66840=CARTESIAN_POINT('',(87.1806428354228,66.41344859951,13.0269406741497));
#66841=CARTESIAN_POINT('',(87.2317863635668,64.9396,11.0631410324494));
#66842=CARTESIAN_POINT('Ctrl Pts',(87.1806428355035,64.3667534988952,13.0269406742195));
#66843=CARTESIAN_POINT('Ctrl Pts',(87.1852854866371,64.3673553924107,13.0309524292991));
#66844=CARTESIAN_POINT('Ctrl Pts',(87.1899570974136,64.3679586289739,13.0349304406614));
#66845=CARTESIAN_POINT('Ctrl Pts',(87.2014060533446,64.3694313833721,13.0445373041855));
#66846=CARTESIAN_POINT('Ctrl Pts',(87.2082133282221,64.3703023144596,13.0501296478996));
#66847=CARTESIAN_POINT('Ctrl Pts',(87.2230030283886,64.3721849081683,13.0620241974872));
#66848=CARTESIAN_POINT('Ctrl Pts',(87.2310040091184,64.3731974606554,13.0683021839868));
#66849=CARTESIAN_POINT('Ctrl Pts',(87.2535051205216,64.3760296076747,13.0855251537965));
#66850=CARTESIAN_POINT('Ctrl Pts',(87.2681652799829,64.3778573401527,13.0962555618629));
#66851=CARTESIAN_POINT('Ctrl Pts',(87.3514985479614,64.3881574257102,13.1545474817563));
#66852=CARTESIAN_POINT('Ctrl Pts',(87.4244878535983,64.3968669982924,13.195546313156));
#66853=CARTESIAN_POINT('Ctrl Pts',(87.569344206767,64.4135313761296,13.2590704050229));
#66854=CARTESIAN_POINT('Ctrl Pts',(87.6402549801509,64.421433039703,13.2829747600588));
#66855=CARTESIAN_POINT('Ctrl Pts',(87.7250878854589,64.4303806930004,13.3034620886454));
#66856=CARTESIAN_POINT('Ctrl Pts',(87.7373565607569,64.4316624541041,13.3062328287028));
#66857=CARTESIAN_POINT('Ctrl Pts',(87.7557049422675,64.4335593748953,13.3100910436916));
#66858=CARTESIAN_POINT('Ctrl Pts',(87.761754101863,64.4341815353569,13.3113170598695));
#66859=CARTESIAN_POINT('Ctrl Pts',(87.7726933367175,64.4353005652632,13.3134512682679));
#66860=CARTESIAN_POINT('Ctrl Pts',(87.7775799980215,64.4357982376748,13.3143748788322));
#66861=CARTESIAN_POINT('Ctrl Pts',(87.7886766903221,64.4369234303532,13.3164047859502));
#66862=CARTESIAN_POINT('Ctrl Pts',(87.7948897037884,64.4375499693954,13.3174935592502));
#66863=CARTESIAN_POINT('Ctrl Pts',(87.8141792544465,64.4394852644231,13.3207259357762));
#66864=CARTESIAN_POINT('Ctrl Pts',(87.8272821105822,64.4407857551994,13.3227113302234));
#66865=CARTESIAN_POINT('Ctrl Pts',(87.8585697877915,64.4438631434926,13.3269522980635));
#66866=CARTESIAN_POINT('Ctrl Pts',(87.8767775526825,64.4456316233368,13.3290202322757));
#66867=CARTESIAN_POINT('Ctrl Pts',(87.9482150465085,64.4525065353792,13.3355711924903));
#66868=CARTESIAN_POINT('Ctrl Pts',(88.0016654145285,64.4575140393961,13.3370889092384));
#66869=CARTESIAN_POINT('Ctrl Pts',(88.138142665675,64.4703121658286,13.3323515329334));
#66870=CARTESIAN_POINT('Ctrl Pts',(88.2207313937079,64.4780807532932,13.3213171577363));
#66871=CARTESIAN_POINT('Ctrl Pts',(88.318488572518,64.4877786842529,13.2983352841671));
#66872=CARTESIAN_POINT('Ctrl Pts',(88.3352509548554,64.4894592769705,13.2940312397134));
#66873=CARTESIAN_POINT('Ctrl Pts',(88.36249774422,64.492223952646,13.2864384172987));
#66874=CARTESIAN_POINT('Ctrl Pts',(88.3730371411727,64.4933015117071,13.2833535577206));
#66875=CARTESIAN_POINT('Ctrl Pts',(88.3919711725778,64.495253014305,13.2775439894654));
#66876=CARTESIAN_POINT('Ctrl Pts',(88.4003800499037,64.4961253358192,13.2748676683435));
#66877=CARTESIAN_POINT('Ctrl Pts',(88.4184027938903,64.4980076240898,13.2689239618665));
#66878=CARTESIAN_POINT('Ctrl Pts',(88.4280066465741,64.4990184575209,13.2656284991102));
#66879=CARTESIAN_POINT('Ctrl Pts',(88.4545673556663,64.5018366555625,13.2561569916632));
#66880=CARTESIAN_POINT('Ctrl Pts',(88.4714328152699,64.503652005156,13.2497344299144));
#66881=CARTESIAN_POINT('Ctrl Pts',(88.5418197392397,64.511343116927,13.2211985531459));
#66882=CARTESIAN_POINT('Ctrl Pts',(88.5939235281691,64.5173244337867,13.1958013353278));
#66883=CARTESIAN_POINT('Ctrl Pts',(88.7136434776234,64.5317787459712,13.1269556319073));
#66884=CARTESIAN_POINT('Ctrl Pts',(88.7792349925987,64.540299077164,13.0804700611733));
#66885=CARTESIAN_POINT('Ctrl Pts',(88.8608747796471,64.5515234701443,13.0101249335553));
#66886=CARTESIAN_POINT('Ctrl Pts',(88.8811579420215,64.5543691432288,12.9914645033955));
#66887=CARTESIAN_POINT('Ctrl Pts',(88.906899172118,64.5580419360455,12.9661873482062));
#66888=CARTESIAN_POINT('Ctrl Pts',(88.9129182727707,64.5589053581524,12.9601566038432));
#66889=CARTESIAN_POINT('Ctrl Pts',(88.9225985753985,64.5603009134007,12.9502603517882));
#66890=CARTESIAN_POINT('Ctrl Pts',(88.9262968019798,64.5608357509062,12.9464317694061));
#66891=CARTESIAN_POINT('Ctrl Pts',(88.9335423951454,64.5618867649839,12.9388357822443));
#66892=CARTESIAN_POINT('Ctrl Pts',(88.9370908974795,64.5624029988859,12.9350698623594));
#66893=CARTESIAN_POINT('Ctrl Pts',(88.9460186071812,64.5637059630603,12.9254783718742));
#66894=CARTESIAN_POINT('Ctrl Pts',(88.9513665502599,64.5644903675441,12.9196238226746));
#66895=CARTESIAN_POINT('Ctrl Pts',(88.9731797724281,64.5677080677679,12.8952904349869));
#66896=CARTESIAN_POINT('Ctrl Pts',(88.9891597101199,64.5701089328065,12.8763804110166));
#66897=CARTESIAN_POINT('Ctrl Pts',(89.0331340280854,64.5768876028051,12.8211450009424));
#66898=CARTESIAN_POINT('Ctrl Pts',(89.0597295593094,64.5812022014698,12.7837528607944));
#66899=CARTESIAN_POINT('Ctrl Pts',(89.1356278363609,64.5945113116869,12.6637859247197));
#66900=CARTESIAN_POINT('Ctrl Pts',(89.177617514863,64.6034321586965,12.57701446151));
#66901=CARTESIAN_POINT('Ctrl Pts',(89.2149210778998,64.6143217509405,12.4706607475849));
#66902=CARTESIAN_POINT('Ctrl Pts',(89.2201137877058,64.6159365806313,12.4548702484375));
#66903=CARTESIAN_POINT('Ctrl Pts',(89.2281487666283,64.6186112724524,12.4287178052946));
#66904=CARTESIAN_POINT('Ctrl Pts',(89.2311722262133,64.6196651987894,12.4184131768855));
#66905=CARTESIAN_POINT('Ctrl Pts',(89.2364203523027,64.621585300348,12.3996487061065));
#66906=CARTESIAN_POINT('Ctrl Pts',(89.2386890144655,64.6224499850216,12.3912017419092));
#66907=CARTESIAN_POINT('Ctrl Pts',(89.2434119023822,64.6243284828954,12.3728627872661));
#66908=CARTESIAN_POINT('Ctrl Pts',(89.2458346333304,64.6253432506614,12.362963432144));
#66909=CARTESIAN_POINT('Ctrl Pts',(89.252311789645,64.6282079154989,12.3350466364236));
#66910=CARTESIAN_POINT('Ctrl Pts',(89.2560925171016,64.6300663908075,12.3169692867603));
#66911=CARTESIAN_POINT('Ctrl Pts',(89.2708742965482,64.6382363565111,12.2377022700086));
#66912=CARTESIAN_POINT('Ctrl Pts',(89.2777659347643,64.6446716250192,12.175845641126));
#66913=CARTESIAN_POINT('Ctrl Pts',(89.2837002742137,64.6612263211449,12.0181045687151));
#66914=CARTESIAN_POINT('Ctrl Pts',(89.2764761922883,64.6714249825564,11.9223609554739));
#66915=CARTESIAN_POINT('Ctrl Pts',(89.2562308114717,64.6825175433449,11.8160888547564));
#66916=CARTESIAN_POINT('Ctrl Pts',(89.2537179987655,64.6837880113829,11.8038790886222));
#66917=CARTESIAN_POINT('Ctrl Pts',(89.249701790301,64.6856695553526,11.7857225540153));
#66918=CARTESIAN_POINT('Ctrl Pts',(89.2483345662003,64.6862875366826,11.7797470540538));
#66919=CARTESIAN_POINT('Ctrl Pts',(89.2457828826171,64.6874011236585,11.768954832619));
#66920=CARTESIAN_POINT('Ctrl Pts',(89.2446134402925,64.6878975073301,11.7641349950594));
#66921=CARTESIAN_POINT('Ctrl Pts',(89.2418926014574,64.6890215212784,11.753201043222));
#66922=CARTESIAN_POINT('Ctrl Pts',(89.24032385375,64.6896481597839,11.7470914668708));
#66923=CARTESIAN_POINT('Ctrl Pts',(89.2353181202467,64.6915839388708,11.728182341041));
#66924=CARTESIAN_POINT('Ctrl Pts',(89.2317260841949,64.6928848140655,11.7154240335023));
#66925=CARTESIAN_POINT('Ctrl Pts',(89.222695434177,64.695962359248,11.6851723985457));
#66926=CARTESIAN_POINT('Ctrl Pts',(89.2170766641268,64.697730617066,11.6677354239861));
#66927=CARTESIAN_POINT('Ctrl Pts',(89.1936494975032,64.7045926066705,11.6000833509232));
#66928=CARTESIAN_POINT('Ctrl Pts',(89.1730645993851,64.7095876745403,11.5508833007178));
#66929=CARTESIAN_POINT('Ctrl Pts',(89.1120723102569,64.7224834710716,11.4275245023046));
#66930=CARTESIAN_POINT('Ctrl Pts',(89.067266964979,64.730360227484,11.3558534227431));
#66931=CARTESIAN_POINT('Ctrl Pts',(89.0050631185615,64.7401820398604,11.2754048581576));
#66932=CARTESIAN_POINT('Ctrl Pts',(88.9941496821539,64.7418704040926,11.2618738928168));
#66933=CARTESIAN_POINT('Ctrl Pts',(88.9758654161854,64.7446474986935,11.2401329926345));
#66934=CARTESIAN_POINT('Ctrl Pts',(88.9686589069861,64.7457296563503,11.2317872067827));
#66935=CARTESIAN_POINT('Ctrl Pts',(88.9554689062131,64.7476892246248,11.2169081620566));
#66936=CARTESIAN_POINT('Ctrl Pts',(88.9495238973119,64.7485650029243,11.2103415703415));
#66937=CARTESIAN_POINT('Ctrl Pts',(88.9365933639396,64.7504545244626,11.1963559601061));
#66938=CARTESIAN_POINT('Ctrl Pts',(88.9295863220642,64.751469135291,11.188957820299));
#66939=CARTESIAN_POINT('Ctrl Pts',(88.9098812166861,64.7542976910521,11.1686480657552));
#66940=CARTESIAN_POINT('Ctrl Pts',(88.8969954767106,64.7561196327396,11.1559231545613));
#66941=CARTESIAN_POINT('Ctrl Pts',(88.8410142582401,64.7639246987715,11.10295655043));
#66942=CARTESIAN_POINT('Ctrl Pts',(88.7954240824389,64.770016804994,11.0654737760627));
#66943=CARTESIAN_POINT('Ctrl Pts',(88.6777175811957,64.7851394260122,10.9817012552498));
#66944=CARTESIAN_POINT('Ctrl Pts',(88.6031993351915,64.7942286054061,10.9392718022762));
#66945=CARTESIAN_POINT('Ctrl Pts',(88.5050363255195,64.8053521666606,10.8958274437958));
#66946=CARTESIAN_POINT('Ctrl Pts',(88.484865580124,64.8075947035554,10.8875148254209));
#66947=CARTESIAN_POINT('Ctrl Pts',(88.4572636547063,64.8105975405033,10.8769631709453));
#66948=CARTESIAN_POINT('Ctrl Pts',(88.4500131648125,64.8113802684468,10.8742671094635));
#66949=CARTESIAN_POINT('Ctrl Pts',(88.4380428888494,64.8126621184818,10.8699400945722));
#66950=CARTESIAN_POINT('Ctrl Pts',(88.4333374545993,64.813163377797,10.8682704791849));
#66951=CARTESIAN_POINT('Ctrl Pts',(88.4236492171154,64.8141899110996,10.8648970272056));
#66952=CARTESIAN_POINT('Ctrl Pts',(88.4186654683518,64.8147150036664,10.8631963596466));
#66953=CARTESIAN_POINT('Ctrl Pts',(88.4057209130096,64.8160715520812,10.8588688261711));
#66954=CARTESIAN_POINT('Ctrl Pts',(88.3977442002758,64.8169003621621,10.8562896184672));
#66955=CARTESIAN_POINT('Ctrl Pts',(88.3631872209157,64.8204628278205,10.8454926618706));
#66956=CARTESIAN_POINT('Ctrl Pts',(88.3363635255105,64.8231565930429,10.8380696441756));
#66957=CARTESIAN_POINT('Ctrl Pts',(88.2545472012226,64.8312232903121,10.8182983677254));
#66958=CARTESIAN_POINT('Ctrl Pts',(88.1989545792285,64.8365051180142,10.8087216265665));
#66959=CARTESIAN_POINT('Ctrl Pts',(88.0677429999102,64.8488929218288,10.7950196148503));
#66960=CARTESIAN_POINT('Ctrl Pts',(87.992041432188,64.8559874194276,10.7938958494005));
#66961=CARTESIAN_POINT('Ctrl Pts',(87.8994704204392,64.8649562475728,10.8007887443804));
#66962=CARTESIAN_POINT('Ctrl Pts',(87.8822737119054,64.866634320773,10.802422600144));
#66963=CARTESIAN_POINT('Ctrl Pts',(87.8541600005214,64.8694012170085,10.8056735078812));
#66964=CARTESIAN_POINT('Ctrl Pts',(87.8432208019436,64.8704836923715,10.8070830947309));
#66965=CARTESIAN_POINT('Ctrl Pts',(87.8234756450992,64.8724491168913,10.8098893002345));
#66966=CARTESIAN_POINT('Ctrl Pts',(87.8146632701996,64.8733304823305,10.8112365353676));
#66967=CARTESIAN_POINT('Ctrl Pts',(87.7956818226743,64.875238468276,10.8143432658307));
#66968=CARTESIAN_POINT('Ctrl Pts',(87.78551864641,64.8762660082169,10.8161341508317));
#66969=CARTESIAN_POINT('Ctrl Pts',(87.7571709613859,64.8791496491295,10.8214863750839));
#66970=CARTESIAN_POINT('Ctrl Pts',(87.7390418183201,64.8810141666138,10.8253219601202));
#66971=CARTESIAN_POINT('Ctrl Pts',(87.657840884435,64.8894635397951,10.8443667844751));
#66972=CARTESIAN_POINT('Ctrl Pts',(87.5959188389235,64.8961827836235,10.8639960705532));
#66973=CARTESIAN_POINT('Ctrl Pts',(87.4758157700362,64.9097733715291,10.9124581914677));
#66974=CARTESIAN_POINT('Ctrl Pts',(87.4177898419301,64.9166247214548,10.9411966759536));
#66975=CARTESIAN_POINT('Ctrl Pts',(87.361856214396,64.9234340157367,10.9744357508572));
#66976=CARTESIAN_POINT('Ctrl Pts',(87.3615077575042,64.9234764445663,10.9746430504489));
#66977=CARTESIAN_POINT('Ctrl Pts',(87.3608474851119,64.9235568559819,10.9750362796211));
#66978=CARTESIAN_POINT('Ctrl Pts',(87.360535650008,64.9235948393556,10.9752221760651));
#66979=CARTESIAN_POINT('Ctrl Pts',(87.3599449971576,64.9236667966063,10.9755746294431));
#66980=CARTESIAN_POINT('Ctrl Pts',(87.359666163549,64.923700771128,10.9757411596439));
#66981=CARTESIAN_POINT('Ctrl Pts',(87.3436980245512,64.9256467060782,10.9852862610969));
#66982=CARTESIAN_POINT('Ctrl Pts',(87.3282119847719,64.9275502272988,10.9950029322982));
#66983=CARTESIAN_POINT('Ctrl Pts',(87.2968854250589,64.9314282561891,11.0156144920826));
#66984=CARTESIAN_POINT('Ctrl Pts',(87.2810709406688,64.9334009634589,11.0265419450587));
#66985=CARTESIAN_POINT('Ctrl Pts',(87.259586424246,64.9360962148432,11.042119558274));
#66986=CARTESIAN_POINT('Ctrl Pts',(87.2537006150598,64.9368362177496,11.0464652179827));
#66987=CARTESIAN_POINT('Ctrl Pts',(87.2438435312091,64.9380778590066,11.053875449143));
#66988=CARTESIAN_POINT('Ctrl Pts',(87.2398523847873,64.9385812585839,11.0569130300643));
#66989=CARTESIAN_POINT('Ctrl Pts',(87.2345127837759,64.9392555174034,11.0610270757134));
#66990=CARTESIAN_POINT('Ctrl Pts',(87.2331485041146,64.9394278609354,11.0620826598129));
#66991=CARTESIAN_POINT('Ctrl Pts',(87.2317863635668,64.9396,11.0631410324494));
#66992=CARTESIAN_POINT('',(88.8007982854172,64.9396,11.0714555473222));
#66993=CARTESIAN_POINT('Origin',(88.011,64.9396,12.066));
#66994=CARTESIAN_POINT('Ctrl Pts',(88.8007982854172,64.9395999999999,11.0714555473223));
#66995=CARTESIAN_POINT('Ctrl Pts',(88.8039625986033,64.9391980619403,11.0739684255774));
#66996=CARTESIAN_POINT('Ctrl Pts',(88.807114965516,64.9387969694434,11.0764964424272));
#66997=CARTESIAN_POINT('Ctrl Pts',(88.8140395431263,64.9379143035852,11.0821040683382));
#66998=CARTESIAN_POINT('Ctrl Pts',(88.8178062392383,64.9374331007555,11.0851904330235));
#66999=CARTESIAN_POINT('Ctrl Pts',(88.8300347641081,64.9358670524407,11.0953283879135));
#67000=CARTESIAN_POINT('Ctrl Pts',(88.8384229311932,64.9347867845429,11.1024686622547));
#67001=CARTESIAN_POINT('Ctrl Pts',(88.888433394735,64.9283022879217,11.1461739696863));
#67002=CARTESIAN_POINT('Ctrl Pts',(88.9277244303466,64.9230205582054,11.1853257428775));
#67003=CARTESIAN_POINT('Ctrl Pts',(88.9966091156371,64.9131116344935,11.2635907108737));
#67004=CARTESIAN_POINT('Ctrl Pts',(89.0267385508018,64.9084894206371,11.3020883485947));
#67005=CARTESIAN_POINT('Ctrl Pts',(89.0788693959558,64.899751525597,11.3772532037377));
#67006=CARTESIAN_POINT('Ctrl Pts',(89.1013819878381,64.8956521897241,11.4134790096461));
#67007=CARTESIAN_POINT('Ctrl Pts',(89.1275212597907,64.8903904022928,11.460682883441));
#67008=CARTESIAN_POINT('Ctrl Pts',(89.1328802420769,64.8892811253686,11.4706738370152));
#67009=CARTESIAN_POINT('Ctrl Pts',(89.1431190956893,64.8870991070607,11.4903918383416));
#67010=CARTESIAN_POINT('Ctrl Pts',(89.1480091230171,64.8860267819946,11.5001125196342));
#67011=CARTESIAN_POINT('Ctrl Pts',(89.1571032641745,64.8839724046135,11.5187842450845));
#67012=CARTESIAN_POINT('Ctrl Pts',(89.1613289357173,64.8829911132916,11.5277239542659));
#67013=CARTESIAN_POINT('Ctrl Pts',(89.1707618003447,64.8807371473299,11.5482983169384));
#67014=CARTESIAN_POINT('Ctrl Pts',(89.1758989774433,64.8794623851442,11.5599636275386));
#67015=CARTESIAN_POINT('Ctrl Pts',(89.1920641457929,64.8752897819886,11.5982220136997));
#67016=CARTESIAN_POINT('Ctrl Pts',(89.2023627202778,64.8723697190078,11.6251107815787));
#67017=CARTESIAN_POINT('Ctrl Pts',(89.2438264385035,64.8593312699377,11.745463462886));
#67018=CARTESIAN_POINT('Ctrl Pts',(89.2649621009981,64.8489203306577,11.8420015420369));
#67019=CARTESIAN_POINT('Ctrl Pts',(89.2791066873026,64.8338201746025,11.9838497602535));
#67020=CARTESIAN_POINT('Ctrl Pts',(89.2811942927401,64.8291623636649,12.0279162525263));
#67021=CARTESIAN_POINT('Ctrl Pts',(89.2809071201598,64.8228380985561,12.0886438597775));
#67022=CARTESIAN_POINT('Ctrl Pts',(89.2805014705874,64.8211154897322,12.1052802182264));
#67023=CARTESIAN_POINT('Ctrl Pts',(89.2792396040871,64.8181713908366,12.133918399802));
#67024=CARTESIAN_POINT('Ctrl Pts',(89.2785396304068,64.8169435713111,12.1459245040709));
#67025=CARTESIAN_POINT('Ctrl Pts',(89.2773022474209,64.8152103426091,12.1629758640275));
#67026=CARTESIAN_POINT('Ctrl Pts',(89.2769050443221,64.8146979220926,12.1680300055463));
#67027=CARTESIAN_POINT('Ctrl Pts',(89.2760520860028,64.8136787199122,12.178110147181));
#67028=CARTESIAN_POINT('Ctrl Pts',(89.2755966175181,64.8131719310478,12.1831360907898));
#67029=CARTESIAN_POINT('Ctrl Pts',(89.2745854028635,64.8121198285345,12.1936001913951));
#67030=CARTESIAN_POINT('Ctrl Pts',(89.2740244867495,64.81157485627,12.199037693705));
#67031=CARTESIAN_POINT('Ctrl Pts',(89.2723699609018,64.8100674305017,12.214121806448));
#67032=CARTESIAN_POINT('Ctrl Pts',(89.2712007769097,64.8091091899186,12.2237601718485));
#67033=CARTESIAN_POINT('Ctrl Pts',(89.2625600995788,64.8026753318308,12.288747761552));
#67034=CARTESIAN_POINT('Ctrl Pts',(89.2515535359822,64.797379371364,12.3435764336325));
#67035=CARTESIAN_POINT('Ctrl Pts',(89.2173790373507,64.7850756757847,12.4699576146926));
#67036=CARTESIAN_POINT('Ctrl Pts',(89.1914071549365,64.778123376064,12.5405215551405));
#67037=CARTESIAN_POINT('Ctrl Pts',(89.1479534032458,64.7684804319102,12.6325245258898));
#67038=CARTESIAN_POINT('Ctrl Pts',(89.1357912896725,64.7659331657174,12.6563028289485));
#67039=CARTESIAN_POINT('Ctrl Pts',(89.1130760809626,64.7614061004957,12.6974592401371));
#67040=CARTESIAN_POINT('Ctrl Pts',(89.10283809079,64.7594371464347,12.7150007176854));
#67041=CARTESIAN_POINT('Ctrl Pts',(89.0867791158788,64.7564459019296,12.7410595924762));
#67042=CARTESIAN_POINT('Ctrl Pts',(89.0812672557742,64.7554351946831,12.7497646852751));
#67043=CARTESIAN_POINT('Ctrl Pts',(89.0710750047924,64.7535938658215,12.7654364943452));
#67044=CARTESIAN_POINT('Ctrl Pts',(89.0664302414056,64.7527646555366,12.7724258078832));
#67045=CARTESIAN_POINT('Ctrl Pts',(89.0562308865529,64.7509644846309,12.7874483867613));
#67046=CARTESIAN_POINT('Ctrl Pts',(89.0506522631417,64.7499926196978,12.7954645559896));
#67047=CARTESIAN_POINT('Ctrl Pts',(89.0350375505561,64.7473061063133,12.8173590448606));
#67048=CARTESIAN_POINT('Ctrl Pts',(89.0248127905045,64.7455840077606,12.8310992535981));
#67049=CARTESIAN_POINT('Ctrl Pts',(88.947793396566,64.7328681192317,12.9303439136694));
#67050=CARTESIAN_POINT('Ctrl Pts',(88.8705809318035,64.7214245208296,13.007158332812));
#67051=CARTESIAN_POINT('Ctrl Pts',(88.7508671219386,64.7054423492614,13.0991040290845));
#67052=CARTESIAN_POINT('Ctrl Pts',(88.7158695065866,64.7009527455055,13.123292259264));
#67053=CARTESIAN_POINT('Ctrl Pts',(88.6597216871977,64.6940815401407,13.1580685007915));
#67054=CARTESIAN_POINT('Ctrl Pts',(88.6393791246303,64.6916556127317,13.1698991679731));
#67055=CARTESIAN_POINT('Ctrl Pts',(88.6120799267297,64.6884931444257,13.1847761435283));
#67056=CARTESIAN_POINT('Ctrl Pts',(88.605410101818,64.6877276437395,13.1883340765922));
#67057=CARTESIAN_POINT('Ctrl Pts',(88.5942810453438,64.6864626619759,13.1941436820083));
#67058=CARTESIAN_POINT('Ctrl Pts',(88.5898399292759,64.6859611099252,13.1964288056608));
#67059=CARTESIAN_POINT('Ctrl Pts',(88.5812408133145,64.6849961785841,13.2007894108011));
#67060=CARTESIAN_POINT('Ctrl Pts',(88.5770848653467,64.6845325773918,13.2028682948642));
#67061=CARTESIAN_POINT('Ctrl Pts',(88.567090758041,64.6834240593559,13.2077991433247));
#67062=CARTESIAN_POINT('Ctrl Pts',(88.5612418369229,64.6827804651764,13.2106292598123));
#67063=CARTESIAN_POINT('Ctrl Pts',(88.5394775038795,64.6804036119533,13.2209549763501));
#67064=CARTESIAN_POINT('Ctrl Pts',(88.5234273868804,64.6786862845017,13.2281651149287));
#67065=CARTESIAN_POINT('Ctrl Pts',(88.4042655311097,64.6661549432488,13.278746641844));
#67066=CARTESIAN_POINT('Ctrl Pts',(88.2959622948081,64.6559211468479,13.3086651245138));
#67067=CARTESIAN_POINT('Ctrl Pts',(88.1383241793907,64.6408773546819,13.3304844380366));
#67068=CARTESIAN_POINT('Ctrl Pts',(88.0912041650722,64.6363679741724,13.3343448052624));
#67069=CARTESIAN_POINT('Ctrl Pts',(88.0296166877627,64.6303811616122,13.3359448715109));
#67070=CARTESIAN_POINT('Ctrl Pts',(88.0152448407508,64.6289776846651,13.3360742099973));
#67071=CARTESIAN_POINT('Ctrl Pts',(87.9914222153296,64.6266386624352,13.3358842715739));
#67072=CARTESIAN_POINT('Ctrl Pts',(87.9819713117008,64.6257074331782,13.3357033811669));
#67073=CARTESIAN_POINT('Ctrl Pts',(87.9634625971441,64.6238766820813,13.3351423769161));
#67074=CARTESIAN_POINT('Ctrl Pts',(87.9544050775975,64.6229774769138,13.3347707364097));
#67075=CARTESIAN_POINT('Ctrl Pts',(87.9325271369293,64.6207969824826,13.3336383329156));
#67076=CARTESIAN_POINT('Ctrl Pts',(87.9197130917095,64.6195127721846,13.3327800136501));
#67077=CARTESIAN_POINT('Ctrl Pts',(87.8757942410094,64.6150852001708,13.3291684148847));
#67078=CARTESIAN_POINT('Ctrl Pts',(87.8447821908518,64.6119134679753,13.3254626873137));
#67079=CARTESIAN_POINT('Ctrl Pts',(87.711696870125,64.5980897811447,13.304559434578));
#67080=CARTESIAN_POINT('Ctrl Pts',(87.6118094170502,64.5871259828709,13.2760627817375));
#67081=CARTESIAN_POINT('Ctrl Pts',(87.4832054966514,64.5725363818701,13.2216990499138));
#67082=CARTESIAN_POINT('Ctrl Pts',(87.4505136322956,64.5687878865604,13.2062030772724));
#67083=CARTESIAN_POINT('Ctrl Pts',(87.4105048195553,64.564181695724,13.1851013047375));
#67084=CARTESIAN_POINT('Ctrl Pts',(87.4025309523575,64.5632627367182,13.1807859107637));
#67085=CARTESIAN_POINT('Ctrl Pts',(87.3897790350741,64.5617923480321,13.1737070739876));
#67086=CARTESIAN_POINT('Ctrl Pts',(87.3849718258394,64.5612378623138,13.1709973657771));
#67087=CARTESIAN_POINT('Ctrl Pts',(87.3757019500532,64.5601684873268,13.165692245785));
#67088=CARTESIAN_POINT('Ctrl Pts',(87.3712373837137,64.5596534163888,13.1631009272378));
#67089=CARTESIAN_POINT('Ctrl Pts',(87.3600673889788,64.5583643680578,13.1565262763514));
#67090=CARTESIAN_POINT('Ctrl Pts',(87.3533825560524,64.5575925569061,13.1525082292144));
#67091=CARTESIAN_POINT('Ctrl Pts',(87.3286813955454,64.5547375332339,13.1373496137561));
#67092=CARTESIAN_POINT('Ctrl Pts',(87.3109060796185,64.5526768222063,13.1258194935782));
#67093=CARTESIAN_POINT('Ctrl Pts',(87.2542136235734,64.5460535434991,13.0869961045621));
#67094=CARTESIAN_POINT('Ctrl Pts',(87.2165618611432,64.5415736954848,13.0579786261327));
#67095=CARTESIAN_POINT('Ctrl Pts',(87.1806426736235,64.5371153383989,13.0269405343375));
#67096=CARTESIAN_POINT('Origin',(88.011,66.41344859951,12.066));
#67097=CARTESIAN_POINT('',(87.1806430603713,63.5747053956106,13.0269408685296));
#67098=CARTESIAN_POINT('',(87.1806428353965,63.7449175370261,13.026940674127));
#67099=CARTESIAN_POINT('',(87.1806428354228,66.41344859951,13.0269406741497));
#67100=CARTESIAN_POINT('Ctrl Pts',(87.1806430603713,63.5747053956106,13.0269408685296));
#67101=CARTESIAN_POINT('Ctrl Pts',(87.2131406687874,63.5787450234789,13.0550223203165));
#67102=CARTESIAN_POINT('Ctrl Pts',(87.2470702450564,63.5827579522435,13.0814617222632));
#67103=CARTESIAN_POINT('Ctrl Pts',(87.3191685061318,63.5910193312261,13.1319712231246));
#67104=CARTESIAN_POINT('Ctrl Pts',(87.3573716279986,63.5952604067966,13.1558141030443));
#67105=CARTESIAN_POINT('Ctrl Pts',(87.4145618027948,63.6015073096007,13.1874166523558));
#67106=CARTESIAN_POINT('Ctrl Pts',(87.4325997569936,63.6034634380922,13.196825756598));
#67107=CARTESIAN_POINT('Ctrl Pts',(87.4617680786992,63.606611329425,13.2111603204942));
#67108=CARTESIAN_POINT('Ctrl Pts',(87.472757328571,63.6077939158658,13.2163663181297));
#67109=CARTESIAN_POINT('Ctrl Pts',(87.4938073175145,63.6100542870305,13.2259708015726));
#67110=CARTESIAN_POINT('Ctrl Pts',(87.5038537162376,63.6111310013651,13.2303981963543));
#67111=CARTESIAN_POINT('Ctrl Pts',(87.5142063701444,63.6122389457791,13.2348011650559));
#67112=CARTESIAN_POINT('Ctrl Pts',(87.5144569053705,63.612265757187,13.2349076222169));
#67113=CARTESIAN_POINT('Ctrl Pts',(87.5149878586663,63.6123225759548,13.2351330328213));
#67114=CARTESIAN_POINT('Ctrl Pts',(87.515268285302,63.6123525839926,13.235251965928));
#67115=CARTESIAN_POINT('Ctrl Pts',(87.5158627988254,63.6124161995113,13.2355038556333));
#67116=CARTESIAN_POINT('Ctrl Pts',(87.5161768965165,63.61244980785,13.235636786608));
#67117=CARTESIAN_POINT('Ctrl Pts',(87.5168430341345,63.6125210812403,13.2359183899411));
#67118=CARTESIAN_POINT('Ctrl Pts',(87.5171950875685,63.6125587473646,13.2360670299148));
#67119=CARTESIAN_POINT('Ctrl Pts',(87.5177264607698,63.6126155961416,13.2362910976934));
#67120=CARTESIAN_POINT('Ctrl Pts',(87.5179057312002,63.6126347748571,13.2363666433736));
#67121=CARTESIAN_POINT('Ctrl Pts',(87.5184222444489,63.6126900311517,13.2365841655457));
#67122=CARTESIAN_POINT('Ctrl Pts',(87.5187595310051,63.6127261122261,13.2367260373687));
#67123=CARTESIAN_POINT('Ctrl Pts',(87.5197258433452,63.6128294783682,13.237132002988));
#67124=CARTESIAN_POINT('Ctrl Pts',(87.5203550195716,63.6128967754866,13.2373957352643));
#67125=CARTESIAN_POINT('Ctrl Pts',(87.5261534965033,63.6135169332949,13.2398207959798));
#67126=CARTESIAN_POINT('Ctrl Pts',(87.5313367300346,63.614070915077,13.2419483568284));
#67127=CARTESIAN_POINT('Ctrl Pts',(87.5455210975899,63.6155860740318,13.2476612314488));
#67128=CARTESIAN_POINT('Ctrl Pts',(87.5545492293514,63.6165495119586,13.2511778580204));
#67129=CARTESIAN_POINT('Ctrl Pts',(87.5784760483602,63.6191011038844,13.2601838735489));
#67130=CARTESIAN_POINT('Ctrl Pts',(87.5934383831394,63.6206949429883,13.2654975322845));
#67131=CARTESIAN_POINT('Ctrl Pts',(87.6760588885035,63.6294912798135,13.2931059347143));
#67132=CARTESIAN_POINT('Ctrl Pts',(87.7453860665709,63.6368661139339,13.3099531291621));
#67133=CARTESIAN_POINT('Ctrl Pts',(87.8727567295861,63.650400179432,13.3297712955638));
#67134=CARTESIAN_POINT('Ctrl Pts',(87.9303064327199,63.6565068025264,13.3347464607807));
#67135=CARTESIAN_POINT('Ctrl Pts',(88.0145442374373,63.6653388672667,13.3362726264008));
#67136=CARTESIAN_POINT('Ctrl Pts',(88.0411046007869,63.6681074788489,13.3359208867717));
#67137=CARTESIAN_POINT('Ctrl Pts',(88.0849473249219,63.67263481569,13.3339637432382));
#67138=CARTESIAN_POINT('Ctrl Pts',(88.1022420391561,63.6744096520455,13.3328367125123));
#67139=CARTESIAN_POINT('Ctrl Pts',(88.1264742161432,63.6768765519549,13.3307586987851));
#67140=CARTESIAN_POINT('Ctrl Pts',(88.1334339497509,63.677582760264,13.3301039502309));
#67141=CARTESIAN_POINT('Ctrl Pts',(88.1453886095671,63.6787914641302,13.3288796331493));
#67142=CARTESIAN_POINT('Ctrl Pts',(88.1503860853758,63.6792954282006,13.3283378272539));
#67143=CARTESIAN_POINT('Ctrl Pts',(88.1610247368387,63.6803653614817,13.3271204751063));
#67144=CARTESIAN_POINT('Ctrl Pts',(88.1666647672518,63.6809308743539,13.3264367335511));
#67145=CARTESIAN_POINT('Ctrl Pts',(88.1821320602516,63.6824775553295,13.3244562240559));
#67146=CARTESIAN_POINT('Ctrl Pts',(88.1919493816631,63.6834546075764,13.3230821745321));
#67147=CARTESIAN_POINT('Ctrl Pts',(88.2637504602322,63.6905734878149,13.3121741296016));
#67148=CARTESIAN_POINT('Ctrl Pts',(88.3249808159283,63.6964983989757,13.2981736686667));
#67149=CARTESIAN_POINT('Ctrl Pts',(88.4319229477739,63.7070055514274,13.2652252342958));
#67150=CARTESIAN_POINT('Ctrl Pts',(88.4780285434595,63.7115915937569,13.2480328108368));
#67151=CARTESIAN_POINT('Ctrl Pts',(88.5575036850467,63.7197682114682,13.2130194248616));
#67152=CARTESIAN_POINT('Ctrl Pts',(88.5912901466401,63.7233364198879,13.1963020546574));
#67153=CARTESIAN_POINT('Ctrl Pts',(88.6473480786777,63.7294743352627,13.1653884758522));
#67154=CARTESIAN_POINT('Ctrl Pts',(88.6700117397826,63.7320197742271,13.1519545101977));
#67155=CARTESIAN_POINT('Ctrl Pts',(88.7021055914414,63.7357311203229,13.1315560617776));
#67156=CARTESIAN_POINT('Ctrl Pts',(88.7118841132616,63.7368767353092,13.1251497046399));
#67157=CARTESIAN_POINT('Ctrl Pts',(88.7289375286381,63.7389020713695,13.1136376612935));
#67158=CARTESIAN_POINT('Ctrl Pts',(88.7362500123025,63.7397796181008,13.1085887846743));
#67159=CARTESIAN_POINT('Ctrl Pts',(88.7514421101462,63.7416224181797,13.0978622956034));
#67160=CARTESIAN_POINT('Ctrl Pts',(88.759310737603,63.7425881794204,13.0921702305799));
#67161=CARTESIAN_POINT('Ctrl Pts',(88.7799557338921,63.7451528968482,13.0768721867402));
#67162=CARTESIAN_POINT('Ctrl Pts',(88.7926168405301,63.746757644709,13.067114655407));
#67163=CARTESIAN_POINT('Ctrl Pts',(88.8614207666623,63.7556615716778,13.0119887216614));
#67164=CARTESIAN_POINT('Ctrl Pts',(88.9137883536432,63.7631378547537,12.9621466423837));
#67165=CARTESIAN_POINT('Ctrl Pts',(88.9967866777995,63.7762839455562,12.8684558517146));
#67166=CARTESIAN_POINT('Ctrl Pts',(89.0294222183898,63.7818916109602,12.8266095438839));
#67167=CARTESIAN_POINT('Ctrl Pts',(89.0833411475737,63.7919186993168,12.747756198595));
#67168=CARTESIAN_POINT('Ctrl Pts',(89.1055621633078,63.7963467421912,12.7114779573518));
#67169=CARTESIAN_POINT('Ctrl Pts',(89.1303948830462,63.8016349441104,12.6659518835218));
#67170=CARTESIAN_POINT('Ctrl Pts',(89.1347753651175,63.8025823922271,12.6577061046064));
#67171=CARTESIAN_POINT('Ctrl Pts',(89.141591311496,63.8040795125435,12.6445270399634));
#67172=CARTESIAN_POINT('Ctrl Pts',(89.1440862110694,63.8046326243585,12.6396252192228));
#67173=CARTESIAN_POINT('Ctrl Pts',(89.148804906487,63.8056884558851,12.6302033033459));
#67174=CARTESIAN_POINT('Ctrl Pts',(89.1510336968047,63.8061914410068,12.6256861128039));
#67175=CARTESIAN_POINT('Ctrl Pts',(89.1564553745613,63.8074259352643,12.6145309802248));
#67176=CARTESIAN_POINT('Ctrl Pts',(89.1596175336583,63.8081555802353,12.6078782357836));
#67177=CARTESIAN_POINT('Ctrl Pts',(89.1705303452844,63.8107095262049,12.5843943637716));
#67178=CARTESIAN_POINT('Ctrl Pts',(89.1779709683628,63.8125166856189,12.5674202086316));
#67179=CARTESIAN_POINT('Ctrl Pts',(89.2149290597154,63.8218875464834,12.4778242807444));
#67180=CARTESIAN_POINT('Ctrl Pts',(89.2380517197679,63.8291784619634,12.4027377156281));
#67181=CARTESIAN_POINT('Ctrl Pts',(89.2687239892374,63.8432210895852,12.2560815713231));
#67182=CARTESIAN_POINT('Ctrl Pts',(89.2774195744954,63.8499382387509,12.1850778192762));
#67183=CARTESIAN_POINT('Ctrl Pts',(89.280773403647,63.858569533237,12.095897521019));
#67184=CARTESIAN_POINT('Ctrl Pts',(89.2810680787087,63.8603053854848,12.0780564740048));
#67185=CARTESIAN_POINT('Ctrl Pts',(89.2809408342881,63.8630419787497,12.0501167382223));
#67186=CARTESIAN_POINT('Ctrl Pts',(89.2807743705657,63.8640347674062,12.0400185860298));
#67187=CARTESIAN_POINT('Ctrl Pts',(89.2802372105144,63.8659007814367,12.0211164042517));
#67188=CARTESIAN_POINT('Ctrl Pts',(89.2798952802257,63.8667730560387,12.0123120906722));
#67189=CARTESIAN_POINT('Ctrl Pts',(89.2789201780326,63.8687416255734,11.992518109279));
#67190=CARTESIAN_POINT('Ctrl Pts',(89.2782356841114,63.8698394569732,11.981531855538));
#67191=CARTESIAN_POINT('Ctrl Pts',(89.2760985109865,63.8726875656997,11.9531744583774));
#67192=CARTESIAN_POINT('Ctrl Pts',(89.274430884886,63.8744443594351,11.9358225549148));
#67193=CARTESIAN_POINT('Ctrl Pts',(89.2642929771692,63.883298432387,11.8491172907055));
#67194=CARTESIAN_POINT('Ctrl Pts',(89.2504684527016,63.8905557788021,11.7805259593325));
#67195=CARTESIAN_POINT('Ctrl Pts',(89.2133710063105,63.9046046375526,11.6521482022126));
#67196=CARTESIAN_POINT('Ctrl Pts',(89.1910692512142,63.9113611225054,11.5922845371013));
#67197=CARTESIAN_POINT('Ctrl Pts',(89.1580831977303,63.9195780806291,11.5207246663503));
#67198=CARTESIAN_POINT('Ctrl Pts',(89.1515618710104,63.9211358260342,11.5072122768603));
#67199=CARTESIAN_POINT('Ctrl Pts',(89.1367915154864,63.9245195491915,11.4779442115678));
#67200=CARTESIAN_POINT('Ctrl Pts',(89.1284475334855,63.9263414857828,11.4622390629724));
#67201=CARTESIAN_POINT('Ctrl Pts',(89.1163336786624,63.9288617477336,11.4405503338875));
#67202=CARTESIAN_POINT('Ctrl Pts',(89.1128401677556,63.9295750147433,11.4344162135768));
#67203=CARTESIAN_POINT('Ctrl Pts',(89.1067666915956,63.9307917735312,11.4239558249729));
#67204=CARTESIAN_POINT('Ctrl Pts',(89.1042118665007,63.9312967883145,11.419615296589));
#67205=CARTESIAN_POINT('Ctrl Pts',(89.0987379192445,63.9323644014166,11.4104406170507));
#67206=CARTESIAN_POINT('Ctrl Pts',(89.0958122914753,63.9329265752029,11.4056105827813));
#67207=CARTESIAN_POINT('Ctrl Pts',(89.087606889162,63.9344806576538,11.3922656465326));
#67208=CARTESIAN_POINT('Ctrl Pts',(89.0822582334137,63.9354682880542,11.3837931448105));
#67209=CARTESIAN_POINT('Ctrl Pts',(89.0428437867525,63.9425731688896,11.3229658324481));
#67210=CARTESIAN_POINT('Ctrl Pts',(89.005050149669,63.9484753419939,11.273113632677));
#67211=CARTESIAN_POINT('Ctrl Pts',(88.9314862158845,63.95892212194,11.1896533973522));
#67212=CARTESIAN_POINT('Ctrl Pts',(88.8971597717507,63.9634710757743,11.1549571645173));
#67213=CARTESIAN_POINT('Ctrl Pts',(88.8326231080811,63.9716464978133,11.0968322885665));
#67214=CARTESIAN_POINT('Ctrl Pts',(88.8031929807521,63.9752520849876,11.0726317874674));
#67215=CARTESIAN_POINT('Ctrl Pts',(88.7514854356052,63.9814468660623,11.033873201625));
#67216=CARTESIAN_POINT('Ctrl Pts',(88.729756612073,63.9840111564482,11.0186256116557));
#67217=CARTESIAN_POINT('Ctrl Pts',(88.6977655029417,63.9877448704223,10.9976411777459));
#67218=CARTESIAN_POINT('Ctrl Pts',(88.6878749852476,63.9888936480539,10.9913476557364));
#67219=CARTESIAN_POINT('Ctrl Pts',(88.6703329490658,63.9909225798765,10.98052355803));
#67220=CARTESIAN_POINT('Ctrl Pts',(88.6627181664685,63.991800534376,10.9759346509671));
#67221=CARTESIAN_POINT('Ctrl Pts',(88.6466989888236,63.993642208575,10.9665088372009));
#67222=CARTESIAN_POINT('Ctrl Pts',(88.6382861651878,63.9946064225003,10.9616875102278));
#67223=CARTESIAN_POINT('Ctrl Pts',(88.6159236146856,63.9971623295577,10.9492096769612));
#67224=CARTESIAN_POINT('Ctrl Pts',(88.6018843224834,63.9987597422808,10.9417185123187));
#67225=CARTESIAN_POINT('Ctrl Pts',(88.5239249681155,64.007595907638,10.9019840113731));
#67226=CARTESIAN_POINT('Ctrl Pts',(88.4575215763254,64.015008778335,10.874933546742));
#67227=CARTESIAN_POINT('Ctrl Pts',(88.3353996434419,64.0284418570183,10.8368368536491));
#67228=CARTESIAN_POINT('Ctrl Pts',(88.2805336713743,64.0344064140802,10.8236519364154));
#67229=CARTESIAN_POINT('Ctrl Pts',(88.1854269851198,64.0445245098215,10.8073956730959));
#67230=CARTESIAN_POINT('Ctrl Pts',(88.1455763343356,64.0486982698697,10.8025128534222));
#67231=CARTESIAN_POINT('Ctrl Pts',(88.0963745849009,64.0537282366461,10.7988394152524));
#67232=CARTESIAN_POINT('Ctrl Pts',(88.087185548408,64.0546623572592,10.7982537527102));
#67233=CARTESIAN_POINT('Ctrl Pts',(88.0725258385121,64.0561434130099,10.7974793983722));
#67234=CARTESIAN_POINT('Ctrl Pts',(88.067059202746,64.0566936664489,10.7972260581442));
#67235=CARTESIAN_POINT('Ctrl Pts',(88.0565415215797,64.0577482282593,10.7968067496772));
#67236=CARTESIAN_POINT('Ctrl Pts',(88.0514910246063,64.0582527749808,10.7966355858726));
#67237=CARTESIAN_POINT('Ctrl Pts',(88.0389941399391,64.0594969468888,10.796286724085));
#67238=CARTESIAN_POINT('Ctrl Pts',(88.031546874037,64.0602346430776,10.7961443740158));
#67239=CARTESIAN_POINT('Ctrl Pts',(88.0050686975203,64.062845624223,10.7958712703927));
#67240=CARTESIAN_POINT('Ctrl Pts',(87.9860351083321,64.0647007693153,10.7961027353957));
#67241=CARTESIAN_POINT('Ctrl Pts',(87.8891426289245,64.074068813907,10.7994607298161));
#67242=CARTESIAN_POINT('Ctrl Pts',(87.8116747596349,64.0813162683423,10.8093202252663));
#67243=CARTESIAN_POINT('Ctrl Pts',(87.6661522397116,64.0952888852786,10.8416473049455));
#67244=CARTESIAN_POINT('Ctrl Pts',(87.59814434867,64.1019799919406,10.8628760819618));
#67245=CARTESIAN_POINT('Ctrl Pts',(87.515752326902,64.1105834245303,10.8964068828306));
#67246=CARTESIAN_POINT('Ctrl Pts',(87.4993715215902,64.1123191892338,10.9034792292961));
#67247=CARTESIAN_POINT('Ctrl Pts',(87.4739584275012,64.1150558899876,10.9150923627463));
#67248=CARTESIAN_POINT('Ctrl Pts',(87.4648215510081,64.116048880045,10.9194001886641));
#67249=CARTESIAN_POINT('Ctrl Pts',(87.4478100985854,64.1179154340813,10.9276701585964));
#67250=CARTESIAN_POINT('Ctrl Pts',(87.4399234375693,64.1187880483147,10.9316062223438));
#67251=CARTESIAN_POINT('Ctrl Pts',(87.4222754515723,64.1207576157007,10.940644626871));
#67252=CARTESIAN_POINT('Ctrl Pts',(87.4125384038292,64.1218561077368,10.945792426369));
#67253=CARTESIAN_POINT('Ctrl Pts',(87.3875535185791,64.1247064478936,10.9594201928604));
#67254=CARTESIAN_POINT('Ctrl Pts',(87.3724118997576,64.1264648241931,10.9680885529502));
#67255=CARTESIAN_POINT('Ctrl Pts',(87.2923526703218,64.1359352558347,11.0161376721976));
#67256=CARTESIAN_POINT('Ctrl Pts',(87.2309004700675,64.1438392951705,11.0609603375917));
#67257=CARTESIAN_POINT('Ctrl Pts',(87.1195558350058,64.159426540112,11.1585659985002));
#67258=CARTESIAN_POINT('Ctrl Pts',(87.0694328550914,64.1670722357002,11.2106859659522));
#67259=CARTESIAN_POINT('Ctrl Pts',(87.0125524887848,64.1764055149449,11.2809306849819));
#67260=CARTESIAN_POINT('Ctrl Pts',(87.0014031373127,64.1782711863826,11.2953213660597));
#67261=CARTESIAN_POINT('Ctrl Pts',(86.9863260827417,64.1808409420637,11.3156706794672));
#67262=CARTESIAN_POINT('Ctrl Pts',(86.9821341402639,64.1815607220895,11.3214291320676));
#67263=CARTESIAN_POINT('Ctrl Pts',(86.9750555275098,64.1827849341244,11.3313269372816));
#67264=CARTESIAN_POINT('Ctrl Pts',(86.9721447422379,64.1832909401244,11.335448689416));
#67265=CARTESIAN_POINT('Ctrl Pts',(86.9660479020776,64.1843562240845,11.3441921175065));
#67266=CARTESIAN_POINT('Ctrl Pts',(86.9628678130022,64.1849151079535,11.3488177154556));
#67267=CARTESIAN_POINT('Ctrl Pts',(86.9541786192119,64.1864516885805,11.3616378325616));
#67268=CARTESIAN_POINT('Ctrl Pts',(86.9487340464657,64.1874252545805,11.3698760455567));
#67269=CARTESIAN_POINT('Ctrl Pts',(86.9154367951051,64.1934534272418,11.4215588742874));
#67270=CARTESIAN_POINT('Ctrl Pts',(86.89015264914,64.1983627543781,11.4666117561619));
#67271=CARTESIAN_POINT('Ctrl Pts',(86.8197882194496,64.2135934603464,11.612112384576));
#67272=CARTESIAN_POINT('Ctrl Pts',(86.7849715252741,64.2237299871624,11.7169283300702));
#67273=CARTESIAN_POINT('Ctrl Pts',(86.7608576378158,64.2359998639838,11.8416464581302));
#67274=CARTESIAN_POINT('Ctrl Pts',(86.7579598015079,64.2376551876887,11.8584412525019));
#67275=CARTESIAN_POINT('Ctrl Pts',(86.7537654420734,64.2403855686736,11.8860558945803));
#67276=CARTESIAN_POINT('Ctrl Pts',(86.7522686104747,64.2414543339038,11.8968436060929));
#67277=CARTESIAN_POINT('Ctrl Pts',(86.7498137999967,64.2433943952547,11.9163779122075));
#67278=CARTESIAN_POINT('Ctrl Pts',(86.7488076146665,64.2442641204557,11.9251178762813));
#67279=CARTESIAN_POINT('Ctrl Pts',(86.7468339819988,64.2461457436484,11.9439845973359));
#67280=CARTESIAN_POINT('Ctrl Pts',(86.7458972562207,64.2471585426138,11.9541138445864));
#67281=CARTESIAN_POINT('Ctrl Pts',(86.7436229538902,64.2499958695721,11.9824102664751));
#67282=CARTESIAN_POINT('Ctrl Pts',(86.7425544914341,64.2518286100351,12.0005956892039));
#67283=CARTESIAN_POINT('Ctrl Pts',(86.741416161925,64.254930706385,12.0312011137534));
#67284=CARTESIAN_POINT('Ctrl Pts',(86.7411367015634,64.2561934210007,12.0436111484597));
#67285=CARTESIAN_POINT('Ctrl Pts',(86.7407470209236,64.261260659823,12.0932119099433));
#67286=CARTESIAN_POINT('Ctrl Pts',(86.7420885633283,64.2651054950066,12.1303914859789));
#67287=CARTESIAN_POINT('Ctrl Pts',(86.7490159633792,64.2741522994197,12.2168309390463));
#67288=CARTESIAN_POINT('Ctrl Pts',(86.7558582180125,64.2793744861255,12.2659303845996));
#67289=CARTESIAN_POINT('Ctrl Pts',(86.7770006061972,64.2907660866966,12.371892813843));
#67290=CARTESIAN_POINT('Ctrl Pts',(86.7924066335504,64.2969235381556,12.4284319860954));
#67291=CARTESIAN_POINT('Ctrl Pts',(86.8158911199343,64.3042476902289,12.495860700432));
#67292=CARTESIAN_POINT('Ctrl Pts',(86.8203064715159,64.3055592229958,12.5079439152556));
#67293=CARTESIAN_POINT('Ctrl Pts',(86.8271285147874,64.3074905933901,12.5257684228813));
#67294=CARTESIAN_POINT('Ctrl Pts',(86.8293948049736,64.3081178129633,12.5315618812203));
#67295=CARTESIAN_POINT('Ctrl Pts',(86.8335444677901,64.3092406340744,12.5419443989946));
#67296=CARTESIAN_POINT('Ctrl Pts',(86.8354122331139,64.3097370899307,12.5465392874675));
#67297=CARTESIAN_POINT('Ctrl Pts',(86.8396839252235,64.3108527292287,12.5568740906869));
#67298=CARTESIAN_POINT('Ctrl Pts',(86.8421031763912,64.3114709899404,12.562607432181));
#67299=CARTESIAN_POINT('Ctrl Pts',(86.8496508074487,64.3133596780019,12.5801336546242));
#67300=CARTESIAN_POINT('Ctrl Pts',(86.8549164975763,64.3146223560553,12.5918672303559));
#67301=CARTESIAN_POINT('Ctrl Pts',(86.8678122273157,64.3175938133118,12.6194724442524));
#67302=CARTESIAN_POINT('Ctrl Pts',(86.8755960979228,64.319294897505,12.6352697992552));
#67303=CARTESIAN_POINT('Ctrl Pts',(86.9066028202,64.3257530716487,12.6950297471398));
#67304=CARTESIAN_POINT('Ctrl Pts',(86.9320729482213,64.3304228446853,12.7377804872196));
#67305=CARTESIAN_POINT('Ctrl Pts',(87.0100279385388,64.3434392160269,12.8527027482771));
#67306=CARTESIAN_POINT('Ctrl Pts',(87.0676889060196,64.3517446021911,12.920989561554));
#67307=CARTESIAN_POINT('Ctrl Pts',(87.1443847984837,64.3620077360665,12.9945320065046));
#67308=CARTESIAN_POINT('Ctrl Pts',(87.1569903905394,64.3636719752522,13.0061388811433));
#67309=CARTESIAN_POINT('Ctrl Pts',(87.1734140123514,64.3658148539388,13.0206583922605));
#67310=CARTESIAN_POINT('Ctrl Pts',(87.1770196048446,64.3662837674904,13.0238098092067));
#67311=CARTESIAN_POINT('Ctrl Pts',(87.1806428355035,64.3667534988952,13.0269406742195));
#67312=CARTESIAN_POINT('Ctrl Pts',(87.1806426736235,64.5371153383989,13.0269405343375));
#67313=CARTESIAN_POINT('Ctrl Pts',(87.1514263005812,64.5334889472477,13.0016944045938));
#67314=CARTESIAN_POINT('Ctrl Pts',(87.1233561873418,64.5298768299862,12.9751114426022));
#67315=CARTESIAN_POINT('Ctrl Pts',(87.0555201547087,64.520689310057,12.9047193089426));
#67316=CARTESIAN_POINT('Ctrl Pts',(87.0175412458783,64.5150997030018,12.8593661369084));
#67317=CARTESIAN_POINT('Ctrl Pts',(86.9722199431844,64.5076327208031,12.7968656124822));
#67318=CARTESIAN_POINT('Ctrl Pts',(86.9618953341684,64.5058692079263,12.7819663901448));
#67319=CARTESIAN_POINT('Ctrl Pts',(86.9462692331873,64.5030954847935,12.7583527064121));
#67320=CARTESIAN_POINT('Ctrl Pts',(86.940747507997,64.5020934835451,12.7497861247048));
#67321=CARTESIAN_POINT('Ctrl Pts',(86.9306218333549,64.500213673722,12.7336536829499));
#67322=CARTESIAN_POINT('Ctrl Pts',(86.9259927259231,64.4993368519204,12.7261042557688));
#67323=CARTESIAN_POINT('Ctrl Pts',(86.9157821177259,64.4973625108793,12.7090545781324));
#67324=CARTESIAN_POINT('Ctrl Pts',(86.9102446307748,64.4962634838933,12.699529003006));
#67325=CARTESIAN_POINT('Ctrl Pts',(86.8963042190765,64.4934213174479,12.6748141086086));
#67326=CARTESIAN_POINT('Ctrl Pts',(86.8880878587672,64.4916717900589,12.6595229986332));
#67327=CARTESIAN_POINT('Ctrl Pts',(86.8414170612262,64.4812720287656,12.5682261513557));
#67328=CARTESIAN_POINT('Ctrl Pts',(86.8103837221789,64.4723754689405,12.4886929163256));
#67329=CARTESIAN_POINT('Ctrl Pts',(86.7734118987346,64.4578459449939,12.3559167338631));
#67330=CARTESIAN_POINT('Ctrl Pts',(86.7624499871806,64.4522803861895,12.3043265477575));
#67331=CARTESIAN_POINT('Ctrl Pts',(86.750783559761,64.4439984807312,12.2256148972025));
#67332=CARTESIAN_POINT('Ctrl Pts',(86.7476874389326,64.4412245571559,12.198906378796));
#67333=CARTESIAN_POINT('Ctrl Pts',(86.7447559369753,64.437655009817,12.1639449816109));
#67334=CARTESIAN_POINT('Ctrl Pts',(86.7441498706048,64.4368243646672,12.1557664147302));
#67335=CARTESIAN_POINT('Ctrl Pts',(86.7432849708381,64.4354674845392,12.1423302170906));
#67336=CARTESIAN_POINT('Ctrl Pts',(86.742979536059,64.4349388244294,12.1370760437235));
#67337=CARTESIAN_POINT('Ctrl Pts',(86.7424668449186,64.4339486386881,12.1271969304457));
#67338=CARTESIAN_POINT('Ctrl Pts',(86.7422521997091,64.4334867148656,12.1225725299884));
#67339=CARTESIAN_POINT('Ctrl Pts',(86.7417993822429,64.432385373132,12.1115113038061));
#67340=CARTESIAN_POINT('Ctrl Pts',(86.7415848767882,64.4317472441949,12.1050734993737));
#67341=CARTESIAN_POINT('Ctrl Pts',(86.7409779219114,64.4294162429925,12.081460824189));
#67342=CARTESIAN_POINT('Ctrl Pts',(86.7408849428629,64.4277385608864,12.06427883881));
#67343=CARTESIAN_POINT('Ctrl Pts',(86.7423247799866,64.4183688303657,11.9675449801144));
#67344=CARTESIAN_POINT('Ctrl Pts',(86.7509822654883,64.4109701511084,11.8882651688358));
#67345=CARTESIAN_POINT('Ctrl Pts',(86.7772020010118,64.3987688622362,11.7607016800924));
#67346=CARTESIAN_POINT('Ctrl Pts',(86.7903547609049,64.3940139219809,11.711755732834));
#67347=CARTESIAN_POINT('Ctrl Pts',(86.8133028262411,64.3871017878831,11.6430373958035));
#67348=CARTESIAN_POINT('Ctrl Pts',(86.8207441553494,64.3850079878521,11.6225287045076));
#67349=CARTESIAN_POINT('Ctrl Pts',(86.8351245368275,64.3811989508431,11.5858692952538));
#67350=CARTESIAN_POINT('Ctrl Pts',(86.841877851755,64.3794897971484,11.5696514040103));
#67351=CARTESIAN_POINT('Ctrl Pts',(86.8530016746293,64.3767894878367,11.544425486218));
#67352=CARTESIAN_POINT('Ctrl Pts',(86.8571462798581,64.3758060336757,11.5353196128981));
#67353=CARTESIAN_POINT('Ctrl Pts',(86.8651212212295,64.3739543670005,11.5183335140868));
#67354=CARTESIAN_POINT('Ctrl Pts',(86.868926397684,64.3730870707836,11.510442052974));
#67355=CARTESIAN_POINT('Ctrl Pts',(86.8776864510072,64.3711256887929,11.4927451794826));
#67356=CARTESIAN_POINT('Ctrl Pts',(86.8826874526101,64.3700300422996,11.4829635814334));
#67357=CARTESIAN_POINT('Ctrl Pts',(86.8959700102513,64.3671798752017,11.4577948970307));
#67358=CARTESIAN_POINT('Ctrl Pts',(86.9044430240218,64.365418727724,11.4425123048997));
#67359=CARTESIAN_POINT('Ctrl Pts',(86.9482963189253,64.3565721187751,11.3671260004022));
#67360=CARTESIAN_POINT('Ctrl Pts',(86.9882629789643,64.3493262275239,11.3098458963732));
#67361=CARTESIAN_POINT('Ctrl Pts',(87.0737872774044,64.3352207541863,11.2065349647267));
#67362=CARTESIAN_POINT('Ctrl Pts',(87.1185710934398,64.3283950668457,11.1601198158045));
#67363=CARTESIAN_POINT('Ctrl Pts',(87.1779501565983,64.3201025460595,11.107274056901));
#67364=CARTESIAN_POINT('Ctrl Pts',(87.1893950954753,64.3185358901248,11.0974480361107));
#67365=CARTESIAN_POINT('Ctrl Pts',(87.2147417733791,64.3151383816756,11.0764594226154));
#67366=CARTESIAN_POINT('Ctrl Pts',(87.228709638359,64.3133115679607,11.0653803809104));
#67367=CARTESIAN_POINT('Ctrl Pts',(87.2485109415623,64.3107888646646,11.0503426042845));
#67368=CARTESIAN_POINT('Ctrl Pts',(87.2541500286295,64.3100778106454,11.046133519007));
#67369=CARTESIAN_POINT('Ctrl Pts',(87.2638668210019,64.3088655030661,11.0390057685277));
#67370=CARTESIAN_POINT('Ctrl Pts',(87.2679272365382,64.3083627275558,11.0360640741105));
#67371=CARTESIAN_POINT('Ctrl Pts',(87.2765830441093,64.307299088083,11.0298709445926));
#67372=CARTESIAN_POINT('Ctrl Pts',(87.2811827549543,64.3067386508385,11.0266259201193));
#67373=CARTESIAN_POINT('Ctrl Pts',(87.2939613869813,64.3051943522894,11.0177374546552));
#67374=CARTESIAN_POINT('Ctrl Pts',(87.3021854954923,64.3042146820836,11.0121590455435));
#67375=CARTESIAN_POINT('Ctrl Pts',(87.3577438948443,64.2976844325905,10.9754185235902));
#67376=CARTESIAN_POINT('Ctrl Pts',(87.4070617320362,64.2923099975984,10.947352367846));
#67377=CARTESIAN_POINT('Ctrl Pts',(87.5449283615138,64.2779050190931,10.8806816027452));
#67378=CARTESIAN_POINT('Ctrl Pts',(87.6362494195677,64.2689811858377,10.8487233620262));
#67379=CARTESIAN_POINT('Ctrl Pts',(87.7538994904113,64.2573918041214,10.8220608064475));
#67380=CARTESIAN_POINT('Ctrl Pts',(87.7776420349127,64.2550501793617,10.8173890634394));
#67381=CARTESIAN_POINT('Ctrl Pts',(87.8126797724498,64.2515805649232,10.8115289837774));
#67382=CARTESIAN_POINT('Ctrl Pts',(87.8238818593748,64.2504692202658,10.8098092404708));
#67383=CARTESIAN_POINT('Ctrl Pts',(87.8438741424197,64.2484811519999,10.8070133642217));
#67384=CARTESIAN_POINT('Ctrl Pts',(87.852655559775,64.24760631994,10.8058788036133));
#67385=CARTESIAN_POINT('Ctrl Pts',(87.8713008731174,64.2457449509016,10.803667792833));
#67386=CARTESIAN_POINT('Ctrl Pts',(87.8811668882946,64.2447577357528,10.8026149454319));
#67387=CARTESIAN_POINT('Ctrl Pts',(87.9079082817935,64.24207499275,10.8000777803914));
#67388=CARTESIAN_POINT('Ctrl Pts',(87.9248019299921,64.2403727035484,10.7988154080409));
#67389=CARTESIAN_POINT('Ctrl Pts',(87.9624560215783,64.2365595105638,10.7967581133915));
#67390=CARTESIAN_POINT('Ctrl Pts',(87.9832204017704,64.2344438891176,10.7961340017414));
#67391=CARTESIAN_POINT('Ctrl Pts',(88.0505643823638,64.2275374953974,10.7957622405441));
#67392=CARTESIAN_POINT('Ctrl Pts',(88.0971121437529,64.2226925271662,10.7980674618984));
#67393=CARTESIAN_POINT('Ctrl Pts',(88.212385563456,64.2105326762894,10.810152861959));
#67394=CARTESIAN_POINT('Ctrl Pts',(88.2806403414343,64.203183458623,10.8230187250191));
#67395=CARTESIAN_POINT('Ctrl Pts',(88.3762349272313,64.192843860975,10.8492867123143));
#67396=CARTESIAN_POINT('Ctrl Pts',(88.4046824910195,64.1897621955934,10.8581911115611));
#67397=CARTESIAN_POINT('Ctrl Pts',(88.4410479720605,64.1858357329378,10.870995681333));
#67398=CARTESIAN_POINT('Ctrl Pts',(88.4492723947148,64.1849486128141,10.8739874566524));
#67399=CARTESIAN_POINT('Ctrl Pts',(88.4625046643305,64.1835234340543,10.8789563991309));
#67400=CARTESIAN_POINT('Ctrl Pts',(88.4675317771834,64.1829824859203,10.8808807179496));
#67401=CARTESIAN_POINT('Ctrl Pts',(88.4773747750737,64.1819244884297,10.8847204280945));
#67402=CARTESIAN_POINT('Ctrl Pts',(88.4821914062006,64.1814073319472,10.8866334246328));
#67403=CARTESIAN_POINT('Ctrl Pts',(88.4942658639066,64.1801120120324,10.8915147561668));
#67404=CARTESIAN_POINT('Ctrl Pts',(88.5015083794349,64.1793360539418,10.8945210098232));
#67405=CARTESIAN_POINT('Ctrl Pts',(88.5304822005445,64.1762339300989,10.9068634135562));
#67406=CARTESIAN_POINT('Ctrl Pts',(88.5519807807032,64.1739369425836,10.9167396158973));
#67407=CARTESIAN_POINT('Ctrl Pts',(88.639162269327,64.164588055302,10.9597790894026));
#67408=CARTESIAN_POINT('Ctrl Pts',(88.7021849870034,64.1577428061385,10.9980212617296));
#67409=CARTESIAN_POINT('Ctrl Pts',(88.8209621084332,64.1439391681884,11.0850381822837));
#67410=CARTESIAN_POINT('Ctrl Pts',(88.8764673917627,64.137005077584,11.1336438677674));
#67411=CARTESIAN_POINT('Ctrl Pts',(88.9384203134823,64.1283279890282,11.1982195158716));
#67412=CARTESIAN_POINT('Ctrl Pts',(88.9491814588237,64.1267823269317,11.2098651372503));
#67413=CARTESIAN_POINT('Ctrl Pts',(88.9661605086323,64.1242776274631,11.2289443127793));
#67414=CARTESIAN_POINT('Ctrl Pts',(88.9725165843419,64.1233244051715,11.2362532519637));
#67415=CARTESIAN_POINT('Ctrl Pts',(88.9845492098895,64.1214889329676,11.250413652914));
#67416=CARTESIAN_POINT('Ctrl Pts',(88.9902386054785,64.1206072768338,11.2572535026833));
#67417=CARTESIAN_POINT('Ctrl Pts',(89.0032769455921,64.1185538724829,11.2732676179831));
#67418=CARTESIAN_POINT('Ctrl Pts',(89.0105711658079,64.1173800261024,11.2824850819217));
#67419=CARTESIAN_POINT('Ctrl Pts',(89.034024988014,64.113520732952,11.3129834961945));
#67420=CARTESIAN_POINT('Ctrl Pts',(89.0496396985808,64.110814688494,11.3346715622391));
#67421=CARTESIAN_POINT('Ctrl Pts',(89.086027981821,64.104153523494,11.3887310349992));
#67422=CARTESIAN_POINT('Ctrl Pts',(89.106036224985,64.1001747616221,11.4215828975474));
#67423=CARTESIAN_POINT('Ctrl Pts',(89.1478112650182,64.0911031729747,11.4977520270928));
#67424=CARTESIAN_POINT('Ctrl Pts',(89.1686513517111,64.0859957755468,11.5415112865018));
#67425=CARTESIAN_POINT('Ctrl Pts',(89.2104674788678,64.0743234168536,11.6440305099637));
#67426=CARTESIAN_POINT('Ctrl Pts',(89.2297223071949,64.0677728430725,11.7033723539282));
#67427=CARTESIAN_POINT('Ctrl Pts',(89.2469263903564,64.0603882417334,11.7736198134119));
#67428=CARTESIAN_POINT('Ctrl Pts',(89.2491928113738,64.0593712872739,11.7833716211018));
#67429=CARTESIAN_POINT('Ctrl Pts',(89.2525565287029,64.057790402386,11.7986626682724));
#67430=CARTESIAN_POINT('Ctrl Pts',(89.2537325319229,64.057222374955,11.8041838019497));
#67431=CARTESIAN_POINT('Ctrl Pts',(89.2558875652958,64.0561517678565,11.8146431029454));
#67432=CARTESIAN_POINT('Ctrl Pts',(89.2568740644978,64.0556488265479,11.8195793083298));
#67433=CARTESIAN_POINT('Ctrl Pts',(89.2591727792289,64.0544448631296,11.831448314691));
#67434=CARTESIAN_POINT('Ctrl Pts',(89.2604566248935,64.0537454275362,11.8383864438066));
#67435=CARTESIAN_POINT('Ctrl Pts',(89.26477182315,64.0512939027927,11.8628440998175));
#67436=CARTESIAN_POINT('Ctrl Pts',(89.2674932823561,64.0495577445784,11.8804175352169));
#67437=CARTESIAN_POINT('Ctrl Pts',(89.2718292319115,64.0463832981692,11.9129158422528));
#67438=CARTESIAN_POINT('Ctrl Pts',(89.2735498741069,64.04494113111,11.9278226503319));
#67439=CARTESIAN_POINT('Ctrl Pts',(89.2811985731855,64.0374073224708,12.0062695105088));
#67440=CARTESIAN_POINT('Ctrl Pts',(89.2825959978206,64.0314586250321,12.0701642807362));
#67441=CARTESIAN_POINT('Ctrl Pts',(89.2754483935195,64.0189303066367,12.2036642181091));
#67442=CARTESIAN_POINT('Ctrl Pts',(89.2659633980586,64.0123635226596,12.2729920673909));
#67443=CARTESIAN_POINT('Ctrl Pts',(89.2470553414833,64.0039384684211,12.3581822357299));
#67444=CARTESIAN_POINT('Ctrl Pts',(89.2429329344428,64.0022476046765,12.3751026403264));
#67445=CARTESIAN_POINT('Ctrl Pts',(89.2356416927185,63.9994710390202,12.402561551866));
#67446=CARTESIAN_POINT('Ctrl Pts',(89.2326813562891,63.998392004269,12.4131535665589));
#67447=CARTESIAN_POINT('Ctrl Pts',(89.2271043923316,63.9964411675885,12.4321524376983));
#67448=CARTESIAN_POINT('Ctrl Pts',(89.2245371501587,63.995571018517,12.4405731917736));
#67449=CARTESIAN_POINT('Ctrl Pts',(89.2188397980792,63.9936972333885,12.458587373693));
#67450=CARTESIAN_POINT('Ctrl Pts',(89.2156824987669,63.9926927606254,12.4681714632859));
#67451=CARTESIAN_POINT('Ctrl Pts',(89.2066325511026,63.9899032026671,12.4945797054699));
#67452=CARTESIAN_POINT('Ctrl Pts',(89.2004996484263,63.9881103511096,12.5113181611129));
#67453=CARTESIAN_POINT('Ctrl Pts',(89.1896312321367,63.9850851977706,12.5391530546905));
#67454=CARTESIAN_POINT('Ctrl Pts',(89.1850859926142,63.9838593386643,12.5503216407021));
#67455=CARTESIAN_POINT('Ctrl Pts',(89.1727458331034,63.9806299811763,12.5794489880605));
#67456=CARTESIAN_POINT('Ctrl Pts',(89.1646937922239,63.9786187057474,12.5972944380734));
#67457=CARTESIAN_POINT('Ctrl Pts',(89.1240535654536,63.9689024317577,12.6820797693294));
#67458=CARTESIAN_POINT('Ctrl Pts',(89.0860369561961,63.9610479965126,12.7462464655865));
#67459=CARTESIAN_POINT('Ctrl Pts',(89.0092613097242,63.9471774561566,12.8531767326428));
#67460=CARTESIAN_POINT('Ctrl Pts',(88.9727879642447,63.941174782896,12.8973475802332));
#67461=CARTESIAN_POINT('Ctrl Pts',(88.926626713661,63.9343183923013,12.9461286217911));
#67462=CARTESIAN_POINT('Ctrl Pts',(88.9197144473054,63.9333094337404,12.9532636278205));
#67463=CARTESIAN_POINT('Ctrl Pts',(88.9087577170494,63.9317384973029,12.9643110387754));
#67464=CARTESIAN_POINT('Ctrl Pts',(88.9047700162786,63.9311724952946,12.9682786728214));
#67465=CARTESIAN_POINT('Ctrl Pts',(88.8971594450982,63.9301032999136,12.9757509778697));
#67466=CARTESIAN_POINT('Ctrl Pts',(88.8935420313433,63.9295997617446,12.9792606247455));
#67467=CARTESIAN_POINT('Ctrl Pts',(88.8847846003723,63.9283916656196,12.9876565313533));
#67468=CARTESIAN_POINT('Ctrl Pts',(88.8796243546938,63.927688721315,12.9925214669654));
#67469=CARTESIAN_POINT('Ctrl Pts',(88.8612230594843,63.925212086356,13.0095808175414));
#67470=CARTESIAN_POINT('Ctrl Pts',(88.8477628096726,63.9234547410478,13.0215376130314));
#67471=CARTESIAN_POINT('Ctrl Pts',(88.8224231326715,63.9202341145056,13.0431006298191));
#67472=CARTESIAN_POINT('Ctrl Pts',(88.8106164088786,63.9187669975777,13.052786093961));
#67473=CARTESIAN_POINT('Ctrl Pts',(88.7469704637981,63.9110150096771,13.1031043569611));
#67474=CARTESIAN_POINT('Ctrl Pts',(88.6921995914175,63.9048808839701,13.1398746330204));
#67475=CARTESIAN_POINT('Ctrl Pts',(88.570800145194,63.8918157099872,13.2083333263439));
#67476=CARTESIAN_POINT('Ctrl Pts',(88.5037799042016,63.8848962314556,13.2388029095509));
#67477=CARTESIAN_POINT('Ctrl Pts',(88.4195586494435,63.8762343506057,13.2685935873224));
#67478=CARTESIAN_POINT('Ctrl Pts',(88.4045105475992,63.8746884308345,13.2736013007533));
#67479=CARTESIAN_POINT('Ctrl Pts',(88.3801278952293,63.8721835678532,13.2812112586279));
#67480=CARTESIAN_POINT('Ctrl Pts',(88.3708499972099,63.8712304458611,13.2839908754675));
#67481=CARTESIAN_POINT('Ctrl Pts',(88.3529927141046,63.8693953435514,13.2891190018694));
#67482=CARTESIAN_POINT('Ctrl Pts',(88.3444186257631,63.8685139581952,13.2914840345707));
#67483=CARTESIAN_POINT('Ctrl Pts',(88.3244629813498,63.8664614495658,13.2967635782903));
#67484=CARTESIAN_POINT('Ctrl Pts',(88.3130646401807,63.8652882312671,13.2996105364436));
#67485=CARTESIAN_POINT('Ctrl Pts',(88.2756418075873,63.8614321516787,13.308407889798));
#67486=CARTESIAN_POINT('Ctrl Pts',(88.2494711694235,63.858728735124,13.3136954273214));
#67487=CARTESIAN_POINT('Ctrl Pts',(88.1852859641988,63.8520745933887,13.3245704977946));
#67488=CARTESIAN_POINT('Ctrl Pts',(88.1471491657478,63.8481002872882,13.3292648279829));
#67489=CARTESIAN_POINT('Ctrl Pts',(88.0606165737377,63.8390379911835,13.3359526659121));
#67490=CARTESIAN_POINT('Ctrl Pts',(88.0121996398267,63.8339354444197,13.3369207655648));
#67491=CARTESIAN_POINT('Ctrl Pts',(87.9016608098566,63.822275129154,13.3328139660754));
#67492=CARTESIAN_POINT('Ctrl Pts',(87.8397169563649,63.8157317057502,13.3259353877943));
#67493=CARTESIAN_POINT('Ctrl Pts',(87.7687925704164,63.8083657652721,13.312729096893));
#67494=CARTESIAN_POINT('Ctrl Pts',(87.7590872561698,63.8073607064224,13.3108043506762));
#67495=CARTESIAN_POINT('Ctrl Pts',(87.7438492447954,63.8057882010956,13.3075968374524));
#67496=CARTESIAN_POINT('Ctrl Pts',(87.7383013018057,63.805216829394,13.3063901230714));
#67497=CARTESIAN_POINT('Ctrl Pts',(87.7278556634671,63.8041434526552,13.3040446537746));
#67498=CARTESIAN_POINT('Ctrl Pts',(87.7229565760114,63.803641059109,13.3029140099103));
#67499=CARTESIAN_POINT('Ctrl Pts',(87.7112540187223,63.8024432242681,13.3001399147128));
#67500=CARTESIAN_POINT('Ctrl Pts',(87.7044571699791,63.8017493215497,13.2984692629455));
#67501=CARTESIAN_POINT('Ctrl Pts',(87.6808244473056,63.799341708248,13.2924527791167));
#67502=CARTESIAN_POINT('Ctrl Pts',(87.6640630560064,63.7976431602856,13.2878171632395));
#67503=CARTESIAN_POINT('Ctrl Pts',(87.6218336721022,63.7933735247816,13.2751987448215));
#67504=CARTESIAN_POINT('Ctrl Pts',(87.5965113144636,63.7908223617457,13.2667545277613));
#67505=CARTESIAN_POINT('Ctrl Pts',(87.4769298164312,63.7787299554461,13.2226431690182));
#67506=CARTESIAN_POINT('Ctrl Pts',(87.3868753899381,63.7694599997669,13.1766411877438));
#67507=CARTESIAN_POINT('Ctrl Pts',(87.2751706148619,63.7566423927022,13.1016616172297));
#67508=CARTESIAN_POINT('Ctrl Pts',(87.2479025986241,63.7533972341194,13.0817370620718));
#67509=CARTESIAN_POINT('Ctrl Pts',(87.211192502205,63.7488346316453,13.0526001736404));
#67510=CARTESIAN_POINT('Ctrl Pts',(87.2010492700679,63.7475523062412,13.0442902024588));
#67511=CARTESIAN_POINT('Ctrl Pts',(87.1875562592843,63.7458157261342,13.0328821963127));
#67512=CARTESIAN_POINT('Ctrl Pts',(87.1840915006016,63.7453670099197,13.0299206956189));
#67513=CARTESIAN_POINT('Ctrl Pts',(87.1806428353965,63.7449175370261,13.0269406741269));
#67514=CARTESIAN_POINT('Origin',(88.011,66.41344859951,12.066));
#67515=CARTESIAN_POINT('',(87.1797597215505,62.780326894738,13.0279488901568));
#67516=CARTESIAN_POINT('',(87.1806428339316,62.9499311262155,13.0269406728612));
#67517=CARTESIAN_POINT('',(87.1806428354228,66.41344859951,13.0269406741497));
#67518=CARTESIAN_POINT('',(86.7419560246514,63.4657506420021,12.0649467613062));
#67519=CARTESIAN_POINT('Ctrl Pts',(86.7419560246514,63.4657506420021,12.0649467613062));
#67520=CARTESIAN_POINT('Ctrl Pts',(86.7409244756087,63.4525560590529,11.9320771572024));
#67521=CARTESIAN_POINT('Ctrl Pts',(86.8212857002323,63.3973567279427,11.37743698812));
#67522=CARTESIAN_POINT('Ctrl Pts',(87.6251828593756,63.3001526486715,10.6153602361256));
#67523=CARTESIAN_POINT('Ctrl Pts',(89.0204464687028,63.1741384041882,10.9550414954645));
#67524=CARTESIAN_POINT('Ctrl Pts',(89.4918622599116,63.0481241597051,12.3114749020928));
#67525=CARTESIAN_POINT('Ctrl Pts',(88.6079892037427,62.9221099152218,13.443248983286));
#67526=CARTESIAN_POINT('Ctrl Pts',(87.5948389254085,62.8328441602328,13.3520895155867));
#67527=CARTESIAN_POINT('Ctrl Pts',(87.2193328732881,62.7855831534049,13.062732661936));
#67528=CARTESIAN_POINT('Ctrl Pts',(87.1797597215505,62.780326894738,13.0279488901567));
#67529=CARTESIAN_POINT('Ctrl Pts',(86.7410003896142,63.4652041016888,12.0650052036116));
#67530=CARTESIAN_POINT('Ctrl Pts',(86.7409713236518,63.4687020212302,12.1021120541925));
#67531=CARTESIAN_POINT('Ctrl Pts',(86.7425685365845,63.4722221260772,12.1391996150127));
#67532=CARTESIAN_POINT('Ctrl Pts',(86.7476703066644,63.4778718902256,12.1977936676512));
#67533=CARTESIAN_POINT('Ctrl Pts',(86.750108113238,63.4799715403944,12.2193721184907));
#67534=CARTESIAN_POINT('Ctrl Pts',(86.7544144072352,63.4830201377987,12.2503477553927));
#67535=CARTESIAN_POINT('Ctrl Pts',(86.7558380734332,63.4839554676294,12.2598039548382));
#67536=CARTESIAN_POINT('Ctrl Pts',(86.7586878084231,63.485703446774,12.2773815359158));
#67537=CARTESIAN_POINT('Ctrl Pts',(86.7600864601472,63.4865152030011,12.2855069172544));
#67538=CARTESIAN_POINT('Ctrl Pts',(86.7631563847018,63.4882069175507,12.3023582919543));
#67539=CARTESIAN_POINT('Ctrl Pts',(86.7648403033542,63.4890872318153,12.3110814776042));
#67540=CARTESIAN_POINT('Ctrl Pts',(86.7689097559293,63.4911119410671,12.3310351531677));
#67541=CARTESIAN_POINT('Ctrl Pts',(86.7713562966672,63.4922582120445,12.342252191584));
#67542=CARTESIAN_POINT('Ctrl Pts',(86.7798019162478,63.4960002128208,12.3786000626144));
#67543=CARTESIAN_POINT('Ctrl Pts',(86.7864153797502,63.4986151269625,12.4035792948837));
#67544=CARTESIAN_POINT('Ctrl Pts',(86.8150619224439,63.5088697567477,12.4998128233256));
#67545=CARTESIAN_POINT('Ctrl Pts',(86.8425886954972,63.5166728019777,12.5692617160998));
#67546=CARTESIAN_POINT('Ctrl Pts',(86.9082538467012,63.5320964874793,12.7000383366934));
#67547=CARTESIAN_POINT('Ctrl Pts',(86.9458532142023,63.539684769947,12.7613549836031));
#67548=CARTESIAN_POINT('Ctrl Pts',(86.9955183424985,63.5482693734341,12.8287840674081));
#67549=CARTESIAN_POINT('Ctrl Pts',(87.0027341681018,63.5494862787891,12.8382969502422));
#67550=CARTESIAN_POINT('Ctrl Pts',(87.0139651411797,63.5513332201002,12.852677353808));
#67551=CARTESIAN_POINT('Ctrl Pts',(87.0178838616202,63.5519692151185,12.8576186648877));
#67552=CARTESIAN_POINT('Ctrl Pts',(87.0249516937241,63.553101075651,12.8663957535368));
#67553=CARTESIAN_POINT('Ctrl Pts',(87.0280866399815,63.5535978647649,12.8702424726002));
#67554=CARTESIAN_POINT('Ctrl Pts',(87.0351536752969,63.554706127321,12.8788109877208));
#67555=CARTESIAN_POINT('Ctrl Pts',(87.039097580909,63.5553167430409,12.8835227487692));
#67556=CARTESIAN_POINT('Ctrl Pts',(87.0511383886331,63.5571580349622,12.8976975326192));
#67557=CARTESIAN_POINT('Ctrl Pts',(87.0593408319984,63.558381511451,12.9070707279191));
#67558=CARTESIAN_POINT('Ctrl Pts',(87.103024587476,63.5647485768805,12.9555320454869));
#67559=CARTESIAN_POINT('Ctrl Pts',(87.1407551420657,63.5697471123937,12.9924733889405));
#67560=CARTESIAN_POINT('Ctrl Pts',(87.1806430603713,63.5747053956106,13.0269408685296));
#67561=CARTESIAN_POINT('',(86.7410002780733,63.6360809738954,12.0668404202127));
#67562=CARTESIAN_POINT('Ctrl Pts',(87.1806428353965,63.7449175370261,13.0269406741269));
#67563=CARTESIAN_POINT('Ctrl Pts',(87.1778788344965,63.7445572980906,13.0245522769948));
#67564=CARTESIAN_POINT('Ctrl Pts',(87.1751251713004,63.7441965731412,13.0221519829543));
#67565=CARTESIAN_POINT('Ctrl Pts',(87.1659580280572,63.7429894889965,13.014091365608));
#67566=CARTESIAN_POINT('Ctrl Pts',(87.1595915709135,63.7421409630232,13.0083782943341));
#67567=CARTESIAN_POINT('Ctrl Pts',(87.1529095443805,63.741239248717,13.0022590598248));
#67568=CARTESIAN_POINT('Ctrl Pts',(87.1525357886098,63.7411887745264,13.0019163717393));
#67569=CARTESIAN_POINT('Ctrl Pts',(87.1518123142576,63.7410909999996,13.0012522367258));
#67570=CARTESIAN_POINT('Ctrl Pts',(87.1514625704879,63.7410437008327,13.0009308171722));
#67571=CARTESIAN_POINT('Ctrl Pts',(87.1507806068307,63.7409514084119,13.0003033766582));
#67572=CARTESIAN_POINT('Ctrl Pts',(87.1504483696968,63.7409064159682,12.9999973745148));
#67573=CARTESIAN_POINT('Ctrl Pts',(87.1497962050958,63.7408180397169,12.999396064489));
#67574=CARTESIAN_POINT('Ctrl Pts',(87.1494762660274,63.7407746564444,12.9991007691357));
#67575=CARTESIAN_POINT('Ctrl Pts',(87.1488443509107,63.7406889150047,12.9985169260302));
#67576=CARTESIAN_POINT('Ctrl Pts',(87.1485323676797,63.7406465571727,12.9982283860665));
#67577=CARTESIAN_POINT('Ctrl Pts',(87.1479125877201,63.740562357434,12.9976546006264));
#67578=CARTESIAN_POINT('Ctrl Pts',(87.1476047874424,63.7405205157009,12.9973693590814));
#67579=CARTESIAN_POINT('Ctrl Pts',(87.1469899506854,63.7404368845232,12.9967990171017));
#67580=CARTESIAN_POINT('Ctrl Pts',(87.1466829137761,63.7403950951006,12.9965139171525));
#67581=CARTESIAN_POINT('Ctrl Pts',(87.1357377501743,63.7389044792801,12.9863406648321));
#67582=CARTESIAN_POINT('Ctrl Pts',(87.1252704729314,63.7374479672294,12.9762714458703));
#67583=CARTESIAN_POINT('Ctrl Pts',(87.102570979154,63.7342183613692,12.9536729414441));
#67584=CARTESIAN_POINT('Ctrl Pts',(87.0904208160166,63.7324420838182,12.9410659553854));
#67585=CARTESIAN_POINT('Ctrl Pts',(87.0544416730841,63.7270326830765,12.9021552974288));
#67586=CARTESIAN_POINT('Ctrl Pts',(87.0314531185552,63.7233684024862,12.8751025100768));
#67587=CARTESIAN_POINT('Ctrl Pts',(86.9780054478688,63.7143148678151,12.8065848418268));
#67588=CARTESIAN_POINT('Ctrl Pts',(86.9488746554184,63.7088963998614,12.7641637642627));
#67589=CARTESIAN_POINT('Ctrl Pts',(86.8917177396462,63.697196099985,12.6690385322688));
#67590=CARTESIAN_POINT('Ctrl Pts',(86.8646645435672,63.690926387005,12.6158773931494));
#67591=CARTESIAN_POINT('Ctrl Pts',(86.8364194656174,63.6834929624039,12.5491423666132));
#67592=CARTESIAN_POINT('Ctrl Pts',(86.8315784424978,63.68217936296,12.5372014580475));
#67593=CARTESIAN_POINT('Ctrl Pts',(86.8246685914241,63.6802454217344,12.5193834476938));
#67594=CARTESIAN_POINT('Ctrl Pts',(86.8224601543705,63.6796176759507,12.5135620660421));
#67595=CARTESIAN_POINT('Ctrl Pts',(86.8185693728157,63.6784943314309,12.5030741367298));
#67596=CARTESIAN_POINT('Ctrl Pts',(86.8168714706041,63.6779978737666,12.4984137603813));
#67597=CARTESIAN_POINT('Ctrl Pts',(86.8131066870418,63.6768827325442,12.4878889297532));
#67598=CARTESIAN_POINT('Ctrl Pts',(86.811055510164,63.6762649676082,12.4820190928084));
#67599=CARTESIAN_POINT('Ctrl Pts',(86.8068366330882,63.6749719576557,12.4696551152142));
#67600=CARTESIAN_POINT('Ctrl Pts',(86.8046781557314,63.6742972303955,12.4631580058806));
#67601=CARTESIAN_POINT('Ctrl Pts',(86.7990370416351,63.6724967885898,12.4457076226712));
#67602=CARTESIAN_POINT('Ctrl Pts',(86.795650251061,63.6713758818327,12.4347236219992));
#67603=CARTESIAN_POINT('Ctrl Pts',(86.7583954637183,63.6585482493522,12.3078046967755));
#67604=CARTESIAN_POINT('Ctrl Pts',(86.7410802204873,63.647543432149,12.1876452771149));
#67605=CARTESIAN_POINT('Ctrl Pts',(86.7410002780733,63.6360809738954,12.0668404202127));
#67606=CARTESIAN_POINT('Ctrl Pts',(86.7410002770608,63.636080828584,12.0668388887506));
#67607=CARTESIAN_POINT('Ctrl Pts',(86.740974721301,63.6324098526892,12.0281498399178));
#67608=CARTESIAN_POINT('Ctrl Pts',(86.7427170789926,63.6287054753803,11.9894835192214));
#67609=CARTESIAN_POINT('Ctrl Pts',(86.7472007747758,63.6238967995667,11.9401886312309));
#67610=CARTESIAN_POINT('Ctrl Pts',(86.7483180247715,63.6228421524889,11.9294306236973));
#67611=CARTESIAN_POINT('Ctrl Pts',(86.7505582519984,63.620951283067,11.9102475602277));
#67612=CARTESIAN_POINT('Ctrl Pts',(86.7516286790657,63.6201167157255,11.9018169011103));
#67613=CARTESIAN_POINT('Ctrl Pts',(86.753964519267,63.6184234482191,11.8847893451752));
#67614=CARTESIAN_POINT('Ctrl Pts',(86.7552337148474,63.6175646738771,11.8761934436443));
#67615=CARTESIAN_POINT('Ctrl Pts',(86.7581571400063,63.6157089053529,11.8577086470707));
#67616=CARTESIAN_POINT('Ctrl Pts',(86.7598404591185,63.6147110479245,11.8478250518197));
#67617=CARTESIAN_POINT('Ctrl Pts',(86.7647003723756,63.612006910065,11.8211987908639));
#67618=CARTESIAN_POINT('Ctrl Pts',(86.7680970918383,63.6102938089331,11.8044991736362));
#67619=CARTESIAN_POINT('Ctrl Pts',(86.7852454194015,63.6023723622384,11.7280959774561));
#67620=CARTESIAN_POINT('Ctrl Pts',(86.8029673952892,63.5960422064472,11.6693795107205));
#67621=CARTESIAN_POINT('Ctrl Pts',(86.848504660637,63.5826946719617,11.5503585883345));
#67622=CARTESIAN_POINT('Ctrl Pts',(86.8769539359867,63.5756819554171,11.4904822905562));
#67623=CARTESIAN_POINT('Ctrl Pts',(86.9263682775954,63.5652919173396,11.4045162151344));
#67624=CARTESIAN_POINT('Ctrl Pts',(86.9439055312159,63.5618616976349,11.3765823693931));
#67625=CARTESIAN_POINT('Ctrl Pts',(86.969119568661,63.5572826287202,11.3396927115061));
#67626=CARTESIAN_POINT('Ctrl Pts',(86.9758608092795,63.5560893402348,11.3301168562208));
#67627=CARTESIAN_POINT('Ctrl Pts',(86.9864181605426,63.5542686928016,11.3155524937501));
#67628=CARTESIAN_POINT('Ctrl Pts',(86.9901401357136,63.5536356603764,11.3104971548669));
#67629=CARTESIAN_POINT('Ctrl Pts',(86.9968701658313,63.5525069531342,11.3014967061526));
#67630=CARTESIAN_POINT('Ctrl Pts',(86.9998639960061,63.5520103774356,11.29754141839));
#67631=CARTESIAN_POINT('Ctrl Pts',(87.0066323639656,63.5508999997015,11.2887074587019));
#67632=CARTESIAN_POINT('Ctrl Pts',(87.0104193614826,63.5502870756844,11.2838386133593));
#67633=CARTESIAN_POINT('Ctrl Pts',(87.0220374601805,63.5484311197828,11.2691240059134));
#67634=CARTESIAN_POINT('Ctrl Pts',(87.0299799035996,63.5471954573424,11.2593663350289));
#67635=CARTESIAN_POINT('Ctrl Pts',(87.0859781184939,63.5386948477733,11.1926208017888));
#67636=CARTESIAN_POINT('Ctrl Pts',(87.1388341623373,63.5317192327556,11.1398316765309));
#67637=CARTESIAN_POINT('Ctrl Pts',(87.2411061227295,63.5192270717127,11.0542598194228));
#67638=CARTESIAN_POINT('Ctrl Pts',(87.2887456790517,63.5137304606804,11.0197196343669));
#67639=CARTESIAN_POINT('Ctrl Pts',(87.3587933606617,63.5058685016279,10.9760032382588));
#67640=CARTESIAN_POINT('Ctrl Pts',(87.3793327625204,63.5035883119976,10.9639733246264));
#67641=CARTESIAN_POINT('Ctrl Pts',(87.4165491533752,63.4994874586822,10.9435579924292));
#67642=CARTESIAN_POINT('Ctrl Pts',(87.433096205729,63.4976745975404,10.9349496082414));
#67643=CARTESIAN_POINT('Ctrl Pts',(87.4589139148312,63.4948575063346,10.9222327216637));
#67644=CARTESIAN_POINT('Ctrl Pts',(87.4680549216134,63.4938622631665,10.9178653129466));
#67645=CARTESIAN_POINT('Ctrl Pts',(87.4830235823059,63.4922354082331,10.910932282714));
#67646=CARTESIAN_POINT('Ctrl Pts',(87.4888201910716,63.4916061059377,10.908300223472));
#67647=CARTESIAN_POINT('Ctrl Pts',(87.5035065002921,63.4900132391179,10.9017643653714));
#67648=CARTESIAN_POINT('Ctrl Pts',(87.5124214427587,63.4890477384642,10.8979188067478));
#67649=CARTESIAN_POINT('Ctrl Pts',(87.5361223890301,63.4864838919034,10.8880158913315));
#67650=CARTESIAN_POINT('Ctrl Pts',(87.5509795352429,63.4848797594324,10.8821349663878));
#67651=CARTESIAN_POINT('Ctrl Pts',(87.6330632860795,63.476028650612,10.8514219985663));
#67652=CARTESIAN_POINT('Ctrl Pts',(87.7021732161494,63.4686072973881,10.8320399275856));
#67653=CARTESIAN_POINT('Ctrl Pts',(87.8384575622074,63.4540365493605,10.8059865229269));
#67654=CARTESIAN_POINT('Ctrl Pts',(87.9052774317555,63.4469232689498,10.798629548326));
#67655=CARTESIAN_POINT('Ctrl Pts',(87.9877845416672,63.4383111584455,10.7961185188733));
#67656=CARTESIAN_POINT('Ctrl Pts',(88.0032106377316,63.436708687352,10.7959301940393));
#67657=CARTESIAN_POINT('Ctrl Pts',(88.0274280404582,63.4342081562478,10.7960758282989));
#67658=CARTESIAN_POINT('Ctrl Pts',(88.0362184949775,63.4333036562283,10.796219970864));
#67659=CARTESIAN_POINT('Ctrl Pts',(88.0570943431383,63.4311640237176,10.796779168949));
#67660=CARTESIAN_POINT('Ctrl Pts',(88.0691771630497,63.4299323075439,10.7972755764752));
#67661=CARTESIAN_POINT('Ctrl Pts',(88.0873153298456,63.4280949804343,10.7982804532267));
#67662=CARTESIAN_POINT('Ctrl Pts',(88.09337657037,63.4274829608338,10.7986598779004));
#67663=CARTESIAN_POINT('Ctrl Pts',(88.1043873265174,63.4263749970188,10.7994284657178));
#67664=CARTESIAN_POINT('Ctrl Pts',(88.1093374504023,63.4258783210353,10.7998031776724));
#67665=CARTESIAN_POINT('Ctrl Pts',(88.1206493612484,63.4247465164422,10.8007262016051));
#67666=CARTESIAN_POINT('Ctrl Pts',(88.1270093857434,63.4241124409511,10.8012934742789));
#67667=CARTESIAN_POINT('Ctrl Pts',(88.1465567868154,63.422169818513,10.8031856793412));
#67668=CARTESIAN_POINT('Ctrl Pts',(88.1597286159383,63.4208694842112,10.8046691550774));
#67669=CARTESIAN_POINT('Ctrl Pts',(88.2556597223201,63.4114456100984,10.8169972037597));
#67670=CARTESIAN_POINT('Ctrl Pts',(88.3372097345119,63.4036796444376,10.8357728125829));
#67671=CARTESIAN_POINT('Ctrl Pts',(88.4655506297708,63.3909903389589,10.878995316022));
#67672=CARTESIAN_POINT('Ctrl Pts',(88.5136946194585,63.3861167990531,10.8985696051021));
#67673=CARTESIAN_POINT('Ctrl Pts',(88.5804897238031,63.3790492965879,10.9306265072419));
#67674=CARTESIAN_POINT('Ctrl Pts',(88.6002212043818,63.3769217009862,10.9407401356802));
#67675=CARTESIAN_POINT('Ctrl Pts',(88.6353048853998,63.3730553897976,10.9598985206803));
#67676=CARTESIAN_POINT('Ctrl Pts',(88.6507508934359,63.3713229815764,10.9687599205163));
#67677=CARTESIAN_POINT('Ctrl Pts',(88.674650222375,63.3685906635285,10.9831471861076));
#67678=CARTESIAN_POINT('Ctrl Pts',(88.6832331625781,63.3675986646713,10.9884544581321));
#67679=CARTESIAN_POINT('Ctrl Pts',(88.6991896284926,63.3657334651901,10.9985859926686));
#67680=CARTESIAN_POINT('Ctrl Pts',(88.7065780201813,63.364861209331,11.0033858481464));
#67681=CARTESIAN_POINT('Ctrl Pts',(88.7230905723576,63.362891790435,11.0143592003217));
#67682=CARTESIAN_POINT('Ctrl Pts',(88.732185403177,63.3617930839797,11.0205752301688));
#67683=CARTESIAN_POINT('Ctrl Pts',(88.7554859699839,63.3589408438276,11.0369491727886));
#67684=CARTESIAN_POINT('Ctrl Pts',(88.769564513932,63.357180761172,11.0472827845639));
#67685=CARTESIAN_POINT('Ctrl Pts',(88.8386572720735,63.3483519730182,11.1002230628853));
#67686=CARTESIAN_POINT('Ctrl Pts',(88.8903065736056,63.3411247217809,11.1470017822481));
#67687=CARTESIAN_POINT('Ctrl Pts',(88.9815908506844,63.3270878005585,11.2444492537588));
#67688=CARTESIAN_POINT('Ctrl Pts',(89.0217352194448,63.3203121268649,11.2943738164153));
#67689=CARTESIAN_POINT('Ctrl Pts',(89.066452752112,63.3120738872346,11.3594978866205));
#67690=CARTESIAN_POINT('Ctrl Pts',(89.0747376630095,63.3105136989364,11.3720345961342));
#67691=CARTESIAN_POINT('Ctrl Pts',(89.0923468274495,63.307125599561,11.3997374023389));
#67692=CARTESIAN_POINT('Ctrl Pts',(89.1015791064942,63.3053017272696,11.4149591905281));
#67693=CARTESIAN_POINT('Ctrl Pts',(89.1140230828377,63.3027793325172,11.4364843635714));
#67694=CARTESIAN_POINT('Ctrl Pts',(89.117506189909,63.3020658353789,11.4426269832534));
#67695=CARTESIAN_POINT('Ctrl Pts',(89.1233854997704,63.3008488742855,11.4531999818722));
#67696=CARTESIAN_POINT('Ctrl Pts',(89.1258068557812,63.3003438851715,11.4576160411502));
#67697=CARTESIAN_POINT('Ctrl Pts',(89.1308860462559,63.2992765674508,11.4670116042895));
#67698=CARTESIAN_POINT('Ctrl Pts',(89.133537043653,63.2987146615583,11.4719945749487));
#67699=CARTESIAN_POINT('Ctrl Pts',(89.1407968601497,63.2971617872738,11.4858627438029));
#67700=CARTESIAN_POINT('Ctrl Pts',(89.1453341689594,63.2961750874136,11.4947853316033));
#67701=CARTESIAN_POINT('Ctrl Pts',(89.1773106872067,63.2890947249251,11.559550980414));
#67702=CARTESIAN_POINT('Ctrl Pts',(89.2007242013001,63.2832144724285,11.6173011677033));
#67703=CARTESIAN_POINT('Ctrl Pts',(89.2346374149941,63.2728292436425,11.7225632016002));
#67704=CARTESIAN_POINT('Ctrl Pts',(89.2468232308826,63.2683193639547,11.7693887082757));
#67705=CARTESIAN_POINT('Ctrl Pts',(89.2638600710811,63.2601484879769,11.8545238882428));
#67706=CARTESIAN_POINT('Ctrl Pts',(89.2696910935403,63.256506910786,11.892573461));
#67707=CARTESIAN_POINT('Ctrl Pts',(89.2766307282201,63.2502576874316,11.9574030926379));
#67708=CARTESIAN_POINT('Ctrl Pts',(89.2786356637877,63.2476755652195,11.9840608989241));
#67709=CARTESIAN_POINT('Ctrl Pts',(89.2803092410926,63.2439208875251,12.0225009981682));
#67710=CARTESIAN_POINT('Ctrl Pts',(89.2806573961418,63.2427693165201,12.0342480471408));
#67711=CARTESIAN_POINT('Ctrl Pts',(89.2809825347437,63.2407373898654,12.0548894792292));
#67712=CARTESIAN_POINT('Ctrl Pts',(89.2810291938153,63.2398592575688,12.0637821299032));
#67713=CARTESIAN_POINT('Ctrl Pts',(89.2809315937911,63.2380191318709,12.0823535359837));
#67714=CARTESIAN_POINT('Ctrl Pts',(89.2807700718168,63.2370566576788,12.0920315669013));
#67715=CARTESIAN_POINT('Ctrl Pts',(89.2800526317046,63.2345099097434,12.1175392356436));
#67716=CARTESIAN_POINT('Ctrl Pts',(89.2793111871343,63.2329199880404,12.1333613324134));
#67717=CARTESIAN_POINT('Ctrl Pts',(89.273640825396,63.2241765755638,12.2197671933302));
#67718=CARTESIAN_POINT('Ctrl Pts',(89.2631167562541,63.2168531806329,12.2898426582664));
#67719=CARTESIAN_POINT('Ctrl Pts',(89.2311345598257,63.202283925184,12.4248927202992));
#67720=CARTESIAN_POINT('Ctrl Pts',(89.2101518089455,63.1950694746176,12.4897540328759));
#67721=CARTESIAN_POINT('Ctrl Pts',(89.1781175456923,63.1863457211623,12.5669772062672));
#67722=CARTESIAN_POINT('Ctrl Pts',(89.1718993658539,63.1847309801808,12.5812225175145));
#67723=CARTESIAN_POINT('Ctrl Pts',(89.1578257297474,63.1812443265186,12.6119146374463));
#67724=CARTESIAN_POINT('Ctrl Pts',(89.1498742233914,63.1793764102443,12.6283145644598));
#67725=CARTESIAN_POINT('Ctrl Pts',(89.1383263850097,63.176804243065,12.6508811640239));
#67726=CARTESIAN_POINT('Ctrl Pts',(89.1350275555832,63.1760842551329,12.6571960904888));
#67727=CARTESIAN_POINT('Ctrl Pts',(89.1293017132122,63.1748598108925,12.6679358268252));
#67728=CARTESIAN_POINT('Ctrl Pts',(89.1269012079024,63.1743537796587,12.6723744391024));
#67729=CARTESIAN_POINT('Ctrl Pts',(89.1217737075779,63.1732882761929,12.6817217698689));
#67730=CARTESIAN_POINT('Ctrl Pts',(89.1190405308374,63.1727291988858,12.6866268716887));
#67731=CARTESIAN_POINT('Ctrl Pts',(89.1114121067439,63.1711925109648,12.7001061973528));
#67732=CARTESIAN_POINT('Ctrl Pts',(89.1064490951487,63.1702190251029,12.7086420281));
#67733=CARTESIAN_POINT('Ctrl Pts',(89.0750072113904,63.1642057379163,12.7612956636711));
#67734=CARTESIAN_POINT('Ctrl Pts',(89.0459624246218,63.159310196051,12.8038361059621));
#67735=CARTESIAN_POINT('Ctrl Pts',(88.9674603394924,63.1472403727625,12.9050172090907));
#67736=CARTESIAN_POINT('Ctrl Pts',(88.9151333661631,63.1401388838155,12.9611586597914));
#67737=CARTESIAN_POINT('Ctrl Pts',(88.8260415889831,63.1288094857315,13.0409127104838));
#67738=CARTESIAN_POINT('Ctrl Pts',(88.7925850252321,63.1246978942121,13.0679339198044));
#67739=CARTESIAN_POINT('Ctrl Pts',(88.7466167636479,63.1191716667531,13.1013550478156));
#67740=CARTESIAN_POINT('Ctrl Pts',(88.7352744079717,63.1178175435534,13.1093209686171));
#67741=CARTESIAN_POINT('Ctrl Pts',(88.7161332721881,63.115546074811,13.122301557047));
#67742=CARTESIAN_POINT('Ctrl Pts',(88.7084055926599,63.1146326762375,13.1274194924266));
#67743=CARTESIAN_POINT('Ctrl Pts',(88.693067454899,63.1128263003296,13.1373379209636));
#67744=CARTESIAN_POINT('Ctrl Pts',(88.6854606161328,63.111933558945,13.1421430297959));
#67745=CARTESIAN_POINT('Ctrl Pts',(88.6668008790737,63.109750644741,13.1536545135305));
#67746=CARTESIAN_POINT('Ctrl Pts',(88.6556956824345,63.1084573857454,13.1602735394108));
#67747=CARTESIAN_POINT('Ctrl Pts',(88.616380980306,63.1038975407184,13.1829001016026));
#67748=CARTESIAN_POINT('Ctrl Pts',(88.5876640577248,63.1005994501151,13.1979938393671));
#67749=CARTESIAN_POINT('Ctrl Pts',(88.4794661495387,63.0882746394056,13.2496775315404));
#67750=CARTESIAN_POINT('Ctrl Pts',(88.3968547200154,63.0790388568864,13.2791216559667));
#67751=CARTESIAN_POINT('Ctrl Pts',(88.2641322189051,63.064654316586,13.3114881361545));
#67752=CARTESIAN_POINT('Ctrl Pts',(88.2157300598901,63.0595035031374,13.3203538319252));
#67753=CARTESIAN_POINT('Ctrl Pts',(88.1547180398456,63.053202723132,13.3279019494363));
#67754=CARTESIAN_POINT('Ctrl Pts',(88.142484322706,63.0519489755785,13.3292352585699));
#67755=CARTESIAN_POINT('Ctrl Pts',(88.1241449180876,63.0500856002784,13.3309646690371));
#67756=CARTESIAN_POINT('Ctrl Pts',(88.1180531830252,63.0494693019542,13.3314947681054));
#67757=CARTESIAN_POINT('Ctrl Pts',(88.1075050201404,63.0484069847799,13.3323359478733));
#67758=CARTESIAN_POINT('Ctrl Pts',(88.1030505749248,63.0479598808253,13.3326675356406));
#67759=CARTESIAN_POINT('Ctrl Pts',(88.0925318053475,63.0469076111327,13.3333947660591));
#67760=CARTESIAN_POINT('Ctrl Pts',(88.0864662489153,63.0463035582571,13.3337703968814));
#67761=CARTESIAN_POINT('Ctrl Pts',(88.0683028681735,63.0445022121795,13.3347644035184));
#67762=CARTESIAN_POINT('Ctrl Pts',(88.0561980720637,63.0433116704835,13.3352532860217));
#67763=CARTESIAN_POINT('Ctrl Pts',(87.9465910620129,63.032605431056,13.3381098484464));
#67764=CARTESIAN_POINT('Ctrl Pts',(87.8491062050064,63.0235961835048,13.3294121332167));
#67765=CARTESIAN_POINT('Ctrl Pts',(87.6930982747609,63.0086411893832,13.2971178019581));
#67766=CARTESIAN_POINT('Ctrl Pts',(87.6336365895338,63.0028095373435,13.2802106558396));
#67767=CARTESIAN_POINT('Ctrl Pts',(87.5587237698494,62.9950984732415,13.2528743482221));
#67768=CARTESIAN_POINT('Ctrl Pts',(87.5419355399343,62.9933462132126,13.2463401890123));
#67769=CARTESIAN_POINT('Ctrl Pts',(87.5159291872691,62.990589694004,13.2355758169293));
#67770=CARTESIAN_POINT('Ctrl Pts',(87.5066125217897,62.9895935839611,13.2315882455934));
#67771=CARTESIAN_POINT('Ctrl Pts',(87.4892910978402,62.9877247563071,13.223928050818));
#67772=CARTESIAN_POINT('Ctrl Pts',(87.481274819796,62.9868530182226,13.2202827959413));
#67773=CARTESIAN_POINT('Ctrl Pts',(87.4633719291289,62.984890206739,13.2119160206114));
#67774=CARTESIAN_POINT('Ctrl Pts',(87.4535073561872,62.983797635278,13.2071494043554));
#67775=CARTESIAN_POINT('Ctrl Pts',(87.428268049815,62.9809726494415,13.1945482777152));
#67776=CARTESIAN_POINT('Ctrl Pts',(87.4129897234114,62.9792338961734,13.1865272754547));
#67777=CARTESIAN_POINT('Ctrl Pts',(87.3226930091744,62.9687784660065,13.1367495580658));
#67778=CARTESIAN_POINT('Ctrl Pts',(87.2519201410562,62.9598099227285,13.0877935866203));
#67779=CARTESIAN_POINT('Ctrl Pts',(87.1846354640199,62.9504866605631,13.0303799027871));
#67780=CARTESIAN_POINT('Ctrl Pts',(87.1826364289937,62.9502088975538,13.0286633556373));
#67781=CARTESIAN_POINT('Ctrl Pts',(87.1806428339316,62.9499311262155,13.0269406728612));
#67782=CARTESIAN_POINT('Origin',(88.011,66.41344859951,12.066));
#67783=CARTESIAN_POINT('',(87.1806428354228,61.9866340346925,13.0269406741497));
#67784=CARTESIAN_POINT('',(87.180642835277,62.1551929346177,13.0269406740237));
#67785=CARTESIAN_POINT('',(87.1806428354228,66.41344859951,13.0269406741497));
#67786=CARTESIAN_POINT('',(86.7407830691985,62.6720014274556,12.065881049187));
#67787=CARTESIAN_POINT('Ctrl Pts',(86.741000005594,62.67200140049,12.0658807996838));
#67788=CARTESIAN_POINT('Ctrl Pts',(86.7410006057567,62.6713614090784,12.0594864653682));
#67789=CARTESIAN_POINT('Ctrl Pts',(86.7410494978638,62.6707214176669,12.0530923928506));
#67790=CARTESIAN_POINT('Ctrl Pts',(86.7411466724212,62.6700814262553,12.0466990560575));
#67791=CARTESIAN_POINT('Ctrl Pts',(86.7418979703423,62.6651333798744,11.9972694443311));
#67792=CARTESIAN_POINT('Ctrl Pts',(86.7455413478563,62.6601853334935,11.9477745076525));
#67793=CARTESIAN_POINT('Ctrl Pts',(86.7520835395843,62.6552372871125,11.8985803306225));
#67794=CARTESIAN_POINT('Ctrl Pts',(86.7586136938254,62.6502983450267,11.8494766697819));
#67795=CARTESIAN_POINT('Ctrl Pts',(86.7680320119969,62.6453594029408,11.8006732098016));
#67796=CARTESIAN_POINT('Ctrl Pts',(86.7802932726123,62.6404204608549,11.7525339712782));
#67797=CARTESIAN_POINT('Ctrl Pts',(86.7925420837303,62.6354865335345,11.7044436110343));
#67798=CARTESIAN_POINT('Ctrl Pts',(86.8076279882371,62.6305526062142,11.6570166655944));
#67799=CARTESIAN_POINT('Ctrl Pts',(86.8254545663108,62.6256186788938,11.6106078342146));
#67800=CARTESIAN_POINT('Ctrl Pts',(86.8432706298085,62.6206876617311,11.564226375962));
#67801=CARTESIAN_POINT('Ctrl Pts',(86.8638239683567,62.6157566445685,11.5188623527093));
#67802=CARTESIAN_POINT('Ctrl Pts',(86.8869688672123,62.6108256274059,11.4748536454278));
#67803=CARTESIAN_POINT('Ctrl Pts',(86.9101099627559,62.6058954205383,11.4308521699275));
#67804=CARTESIAN_POINT('Ctrl Pts',(86.9358415173653,62.6009652136707,11.3882060525231));
#67805=CARTESIAN_POINT('Ctrl Pts',(86.9639715443507,62.5960350068031,11.3472292346925));
#67806=CARTESIAN_POINT('Ctrl Pts',(86.992129055113,62.5910999829936,11.3062123814323));
#67807=CARTESIAN_POINT('Ctrl Pts',(87.022689405474,62.5861649591841,11.2668685361716));
#67808=CARTESIAN_POINT('Ctrl Pts',(87.0554178905788,62.5812299353746,11.2294817203706));
#67809=CARTESIAN_POINT('Ctrl Pts',(87.088163989134,62.5762922556892,11.192074784151));
#67810=CARTESIAN_POINT('Ctrl Pts',(87.1230801610023,62.5713545760037,11.1566273654471));
#67811=CARTESIAN_POINT('Ctrl Pts',(87.159894543864,62.5664168963183,11.1233868754703));
#67812=CARTESIAN_POINT('Ctrl Pts',(87.1967776730886,62.5614699961192,11.0900843129392));
#67813=CARTESIAN_POINT('Ctrl Pts',(87.235565660193,62.5565230959201,11.0589972473201));
#67814=CARTESIAN_POINT('Ctrl Pts',(87.2759545580742,62.551576195721,11.0303320038236));
#67815=CARTESIAN_POINT('Ctrl Pts',(87.2963903047281,62.5490731910714,11.015828125664));
#67816=CARTESIAN_POINT('Ctrl Pts',(87.3172354577096,62.5465701864218,11.0019435539194));
#67817=CARTESIAN_POINT('Ctrl Pts',(87.3384482567997,62.5440671817721,10.9887005278391));
#67818=CARTESIAN_POINT('Ctrl Pts',(87.3803826224638,62.5391191354633,10.9625211492575));
#67819=CARTESIAN_POINT('Ctrl Pts',(87.4239405293717,62.5341710891545,10.9387360357047));
#67820=CARTESIAN_POINT('Ctrl Pts',(87.468818074963,62.5292230428457,10.9175494089151));
#67821=CARTESIAN_POINT('Ctrl Pts',(87.5136130468598,62.524284100833,10.8964017650517));
#67822=CARTESIAN_POINT('Ctrl Pts',(87.5597223501887,62.5193451588204,10.8778433573357));
#67823=CARTESIAN_POINT('Ctrl Pts',(87.6068156354732,62.5144062168077,10.8620336385629));
#67824=CARTESIAN_POINT('Ctrl Pts',(87.6538611044828,62.5094722895611,10.8462399722243));
#67825=CARTESIAN_POINT('Ctrl Pts',(87.7018880606137,62.5045383623145,10.8331896433857));
#67826=CARTESIAN_POINT('Ctrl Pts',(87.7505462155302,62.4996044350679,10.8229940361546));
#67827=CARTESIAN_POINT('Ctrl Pts',(87.7991756706055,62.4946734179794,10.8128044425569));
#67828=CARTESIAN_POINT('Ctrl Pts',(87.848435051608,62.489742400891,10.8054663470793));
#67829=CARTESIAN_POINT('Ctrl Pts',(87.897961462094,62.4848113838026,10.8010405979052));
#67830=CARTESIAN_POINT('Ctrl Pts',(87.9474797340928,62.4798811770095,10.7966155759977));
#67831=CARTESIAN_POINT('Ctrl Pts',(87.9972644028728,62.4749509702165,10.7951019980655));
#67832=CARTESIAN_POINT('Ctrl Pts',(88.0469475862184,62.4700207634234,10.7965088534988));
#67833=CARTESIAN_POINT('Ctrl Pts',(88.0966793113441,62.4650857396883,10.7979170834669));
#67834=CARTESIAN_POINT('Ctrl Pts',(88.1463088042846,62.4601507159532,10.8022514272422));
#67835=CARTESIAN_POINT('Ctrl Pts',(88.1954701489838,62.4552156922181,10.8094687571995));
#67836=CARTESIAN_POINT('Ctrl Pts',(88.2446579507863,62.4502780126071,10.8166899712987));
#67837=CARTESIAN_POINT('Ctrl Pts',(88.2933765655566,62.4453403329961,10.8267971497315));
#67838=CARTESIAN_POINT('Ctrl Pts',(88.3412706801208,62.440402653385,10.8396960907457));
#67839=CARTESIAN_POINT('Ctrl Pts',(88.3892542311027,62.4354557532595,10.852619118959));
#67840=CARTESIAN_POINT('Ctrl Pts',(88.4364096888277,62.4305088531341,10.8683441413176));
#67841=CARTESIAN_POINT('Ctrl Pts',(88.4823988545942,62.4255619530086,10.8867277159675));
#67842=CARTESIAN_POINT('Ctrl Pts',(88.5056681990265,62.4230589477687,10.8960293356707));
#67843=CARTESIAN_POINT('Ctrl Pts',(88.5286393123781,62.4205559425288,10.906010817654));
#67844=CARTESIAN_POINT('Ctrl Pts',(88.5512708602641,62.4180529372889,10.9166491407975));
#67845=CARTESIAN_POINT('Ctrl Pts',(88.5960098583555,62.4131048909947,10.937679426539));
#67846=CARTESIAN_POINT('Ctrl Pts',(88.6396179904876,62.4081568447004,10.9613723300261));
#67847=CARTESIAN_POINT('Ctrl Pts',(88.6817588492855,62.4032087984061,10.9875833059039));
#67848=CARTESIAN_POINT('Ctrl Pts',(88.7238221698255,62.3982698564088,11.0137460541597));
#67849=CARTESIAN_POINT('Ctrl Pts',(88.7644231100233,62.3933309144115,11.0424173985487));
#67850=CARTESIAN_POINT('Ctrl Pts',(88.8032485290623,62.3883919724141,11.0734062924849));
#67851=CARTESIAN_POINT('Ctrl Pts',(88.8420345266195,62.3834580451833,11.1043637217737));
#67852=CARTESIAN_POINT('Ctrl Pts',(88.8790481456838,62.3785241179525,11.1376337020299));
#67853=CARTESIAN_POINT('Ctrl Pts',(88.9140058141485,62.3735901907217,11.1729823632122));
#67854=CARTESIAN_POINT('Ctrl Pts',(88.9489428636708,62.3686591736495,11.2083101748345));
#67855=CARTESIAN_POINT('Ctrl Pts',(88.981825980317,62.3637281565774,11.2457138496118));
#67856=CARTESIAN_POINT('Ctrl Pts',(89.0124072096571,62.3587971395052,11.2849215145411));
#67857=CARTESIAN_POINT('Ctrl Pts',(89.0429834136973,62.3538669327288,11.3241227366203));
#67858=CARTESIAN_POINT('Ctrl Pts',(89.07125814532,62.3489367259524,11.3651269278832));
#67859=CARTESIAN_POINT('Ctrl Pts',(89.0970243134888,62.344006519176,11.4076298985288));
#67860=CARTESIAN_POINT('Ctrl Pts',(89.1228156558807,62.339071495458,11.4501743956931));
#67861=CARTESIAN_POINT('Ctrl Pts',(89.1460932575231,62.3341364717401,11.4942201259434));
#67862=CARTESIAN_POINT('Ctrl Pts',(89.1666948784301,62.3292014480221,11.539436283086));
#67863=CARTESIAN_POINT('Ctrl Pts',(89.187307586486,62.3242637684286,11.5846767741521));
#67864=CARTESIAN_POINT('Ctrl Pts',(89.2052412483597,62.319326088835,11.6310884347458));
#67865=CARTESIAN_POINT('Ctrl Pts',(89.2203822835105,62.3143884092415,11.678321663836));
#67866=CARTESIAN_POINT('Ctrl Pts',(89.235551592697,62.3094415091337,11.7256430952184));
#67867=CARTESIAN_POINT('Ctrl Pts',(89.2479177305411,62.304494609026,11.7737886260868));
#67868=CARTESIAN_POINT('Ctrl Pts',(89.2574177670228,62.2995477089182,11.8223963258696));
#67869=CARTESIAN_POINT('Ctrl Pts',(89.2622245433512,62.2970447035474,11.8469905830755));
#67870=CARTESIAN_POINT('Ctrl Pts',(89.2662983927379,62.2945416981765,11.8717030465113));
#67871=CARTESIAN_POINT('Ctrl Pts',(89.2696362359932,62.2920386928057,11.8964865036503));
#67872=CARTESIAN_POINT('Ctrl Pts',(89.2762346249657,62.2870906464855,11.9454794843787));
#67873=CARTESIAN_POINT('Ctrl Pts',(89.2799827120667,62.2821426001653,11.9949666012378));
#67874=CARTESIAN_POINT('Ctrl Pts',(89.2808194659684,62.2771945538451,12.0445868300438));
#67875=CARTESIAN_POINT('Ctrl Pts',(89.2816546802615,62.2722556118212,12.094115758722));
#67876=CARTESIAN_POINT('Ctrl Pts',(89.2795891765119,62.2673166697972,12.1437767701432));
#67877=CARTESIAN_POINT('Ctrl Pts',(89.2746136098131,62.2623777277733,12.1932031646421));
#67878=CARTESIAN_POINT('Ctrl Pts',(89.2696430950675,62.2574438005155,12.2425793739378));
#67879=CARTESIAN_POINT('Ctrl Pts',(89.2617684213628,62.2525098732577,12.291720895308));
#67880=CARTESIAN_POINT('Ctrl Pts',(89.2510322587157,62.2475759459999,12.3402626429981));
#67881=CARTESIAN_POINT('Ctrl Pts',(89.2403024285359,62.2426449289003,12.3887757595062));
#67882=CARTESIAN_POINT('Ctrl Pts',(89.2267145710931,62.2377139118008,12.4366892691107));
#67883=CARTESIAN_POINT('Ctrl Pts',(89.2103626024801,62.2327828947013,12.4836473964628));
#67884=CARTESIAN_POINT('Ctrl Pts',(89.1940133209245,62.2278526878972,12.5305978073627));
#67885=CARTESIAN_POINT('Ctrl Pts',(89.1749010109705,62.2229224810932,12.5765926307948));
#67886=CARTESIAN_POINT('Ctrl Pts',(89.1531689029913,62.2179922742891,12.6212928930209));
#67887=CARTESIAN_POINT('Ctrl Pts',(89.1314155621709,62.2130572505433,12.6660368285792));
#67888=CARTESIAN_POINT('Ctrl Pts',(89.1070375537581,62.2081222267974,12.7094831842614));
#67889=CARTESIAN_POINT('Ctrl Pts',(89.0802247962751,62.2031872030516,12.7513162299482));
#67890=CARTESIAN_POINT('Ctrl Pts',(89.0533976090026,62.19824952343,12.7931717888749));
#67891=CARTESIAN_POINT('Ctrl Pts',(89.0241333860616,62.1933118438083,12.8334118652639));
#67892=CARTESIAN_POINT('Ctrl Pts',(88.9926642287378,62.1883741641867,12.8717514145297));
#67893=CARTESIAN_POINT('Ctrl Pts',(88.9611363066031,62.1834272640509,12.9101625582249));
#67894=CARTESIAN_POINT('Ctrl Pts',(88.9273956043593,62.1784803639152,12.9466656888443));
#67895=CARTESIAN_POINT('Ctrl Pts',(88.8917120543797,62.1735334637794,12.9810116268498));
#67896=CARTESIAN_POINT('Ctrl Pts',(88.8736570892498,62.1710304586271,12.9983897944759));
#67897=CARTESIAN_POINT('Ctrl Pts',(88.8551052779863,62.1685274534748,13.0152163296696));
#67898=CARTESIAN_POINT('Ctrl Pts',(88.8360946146734,62.1660244483225,13.0314630375301));
#67899=CARTESIAN_POINT('Ctrl Pts',(88.7985135324435,62.1610764020127,13.0635802158748));
#67900=CARTESIAN_POINT('Ctrl Pts',(88.758971315785,62.156128355703,13.0935708141126));
#67901=CARTESIAN_POINT('Ctrl Pts',(88.7177381654394,62.1511803093933,13.1211877394622));
#67902=CARTESIAN_POINT('Ctrl Pts',(88.6765808831835,62.1462413673799,13.1487538502766));
#67903=CARTESIAN_POINT('Ctrl Pts',(88.6337392895444,62.1413024253665,13.1739546479818));
#67904=CARTESIAN_POINT('Ctrl Pts',(88.5895163880066,62.1363634833532,13.196583384279));
#67905=CARTESIAN_POINT('Ctrl Pts',(88.5453383882945,62.1314295561061,13.2191891444363));
#67906=CARTESIAN_POINT('Ctrl Pts',(88.4997823426521,62.126495628859,13.2392277647408));
#67907=CARTESIAN_POINT('Ctrl Pts',(88.4531781115136,62.1215617016119,13.2565370711147));
#67908=CARTESIAN_POINT('Ctrl Pts',(88.4066013687604,62.1166306845231,13.2738361680103));
#67909=CARTESIAN_POINT('Ctrl Pts',(88.3589781780092,62.1116996674344,13.2884089496651));
#67910=CARTESIAN_POINT('Ctrl Pts',(88.310658373634,62.1067686503456,13.3001413448674));
#67911=CARTESIAN_POINT('Ctrl Pts',(88.2623465094706,62.1018384435524,13.3118718121292));
#67912=CARTESIAN_POINT('Ctrl Pts',(88.213338791383,62.0969082367592,13.3207626912895));
#67913=CARTESIAN_POINT('Ctrl Pts',(88.1639976863608,62.091978029966,13.3267504542804));
#67914=CARTESIAN_POINT('Ctrl Pts',(88.1146083737807,62.087043006231,13.3327440674733));
#67915=CARTESIAN_POINT('Ctrl Pts',(88.0648855690676,62.082107982496,13.3358288361475));
#67916=CARTESIAN_POINT('Ctrl Pts',(88.015197535349,62.077172958761,13.3359930632476));
#67917=CARTESIAN_POINT('Ctrl Pts',(87.965482761081,62.0722352791502,13.3361573787296));
#67918=CARTESIAN_POINT('Ctrl Pts',(87.9158033427583,62.0672975995394,13.3333980532336));
#67919=CARTESIAN_POINT('Ctrl Pts',(87.8665246438208,62.0623599199287,13.3277554721327));
#67920=CARTESIAN_POINT('Ctrl Pts',(87.8171539229256,62.0574130198037,13.3221023542001));
#67921=CARTESIAN_POINT('Ctrl Pts',(87.7681859550106,62.0524661196787,13.3135553289302));
#67922=CARTESIAN_POINT('Ctrl Pts',(87.7199764920651,62.0475192195537,13.302206017551));
#67923=CARTESIAN_POINT('Ctrl Pts',(87.6955837339273,62.0450162143155,13.2964635555821));
#67924=CARTESIAN_POINT('Ctrl Pts',(87.6713849251587,62.0425132090774,13.2900044778591));
#67925=CARTESIAN_POINT('Ctrl Pts',(87.6474243608414,62.0400102038392,13.2828454111391));
#67926=CARTESIAN_POINT('Ctrl Pts',(87.6000738932191,62.0350638066293,13.2686977828762));
#67927=CARTESIAN_POINT('Ctrl Pts',(87.5534458113065,62.0301174094194,13.2517509792419));
#67928=CARTESIAN_POINT('Ctrl Pts',(87.5078939073899,62.0251710122095,13.2320978773579));
#67929=CARTESIAN_POINT('Ctrl Pts',(87.4624076610314,62.0202317446326,13.2124731030424));
#67930=CARTESIAN_POINT('Ctrl Pts',(87.417995021762,62.0152924770558,13.1901499645511));
#67931=CARTESIAN_POINT('Ctrl Pts',(87.3749941041958,62.010353209479,13.1652708949583));
#67932=CARTESIAN_POINT('Ctrl Pts',(87.3320398447943,62.0054193012567,13.1404188204109));
#67933=CARTESIAN_POINT('Ctrl Pts',(87.2904947446986,62.0004853930343,13.1130165818873));
#67934=CARTESIAN_POINT('Ctrl Pts',(87.2506739689398,61.995551484812,13.0832533246405));
#67935=CARTESIAN_POINT('Ctrl Pts',(87.2266835360991,61.9925790014388,13.0653221464931));
#67936=CARTESIAN_POINT('Ctrl Pts',(87.2033185036515,61.9896065180656,13.0465349155861));
#67937=CARTESIAN_POINT('Ctrl Pts',(87.1806428354228,61.9866340346925,13.0269406741497));
#67938=CARTESIAN_POINT('Ctrl Pts',(87.1797597215505,62.780326894738,13.0279488901567));
#67939=CARTESIAN_POINT('Ctrl Pts',(86.9079078714374,62.7442184833402,12.788998179968));
#67940=CARTESIAN_POINT('Ctrl Pts',(86.7393936515874,62.7081100719423,12.4272468679575));
#67941=CARTESIAN_POINT('Ctrl Pts',(86.7389078838356,62.6720016605445,12.0658832058784));
#67942=CARTESIAN_POINT('Ctrl Pts',(87.1806428339316,62.9499311262155,13.0269406728612));
#67943=CARTESIAN_POINT('Ctrl Pts',(87.1433791946131,62.944739113474,12.9947408390777));
#67944=CARTESIAN_POINT('Ctrl Pts',(87.108016329931,62.9395420260643,12.960397503884));
#67945=CARTESIAN_POINT('Ctrl Pts',(87.0625530535798,62.9325407977779,12.9107919488461));
#67946=CARTESIAN_POINT('Ctrl Pts',(87.0506551050908,62.9306754776798,12.8972417369129));
#67947=CARTESIAN_POINT('Ctrl Pts',(87.0306252328578,62.927482436221,12.873425905078));
#67948=CARTESIAN_POINT('Ctrl Pts',(87.0223562773478,62.9261477280882,12.8632796963223));
#67949=CARTESIAN_POINT('Ctrl Pts',(87.0103629800675,62.9241889703896,12.8480900200647));
#67950=CARTESIAN_POINT('Ctrl Pts',(87.0065171522817,62.9235572508871,12.8431444266552));
#67951=CARTESIAN_POINT('Ctrl Pts',(86.9996918831079,62.9224298617817,12.8342320610732));
#67952=CARTESIAN_POINT('Ctrl Pts',(86.9966989327656,62.9219333018418,12.8302760988669));
#67953=CARTESIAN_POINT('Ctrl Pts',(86.9900289722101,62.9208216979861,12.821351811777));
#67954=CARTESIAN_POINT('Ctrl Pts',(86.9863649519595,62.920207542262,12.8163740556274));
#67955=CARTESIAN_POINT('Ctrl Pts',(86.9753153668611,62.9183438972974,12.8011307761641));
#67956=CARTESIAN_POINT('Ctrl Pts',(86.9680462789525,62.917101866923,12.7907809998036));
#67957=CARTESIAN_POINT('Ctrl Pts',(86.9076245032036,62.9066218592343,12.7019599974306));
#67958=CARTESIAN_POINT('Ctrl Pts',(86.8632451504339,62.8978556902477,12.6178592567991));
#67959=CARTESIAN_POINT('Ctrl Pts',(86.8120435309469,62.8846939376316,12.4872710647938));
#67960=CARTESIAN_POINT('Ctrl Pts',(86.797737170153,62.8804118909068,12.4440986417557));
#67961=CARTESIAN_POINT('Ctrl Pts',(86.7778977787751,62.8732063716651,12.3713767649928));
#67962=CARTESIAN_POINT('Ctrl Pts',(86.7710435342713,62.8703207914111,12.3422312372952));
#67963=CARTESIAN_POINT('Ctrl Pts',(86.7628438354002,62.8662083313521,12.3008538486188));
#67964=CARTESIAN_POINT('Ctrl Pts',(86.760636128876,62.86500858807,12.2888010451757));
#67965=CARTESIAN_POINT('Ctrl Pts',(86.7571150434095,62.8629210377034,12.2678736370288));
#67966=CARTESIAN_POINT('Ctrl Pts',(86.7557206356046,62.8620358443886,12.2590133586977));
#67967=CARTESIAN_POINT('Ctrl Pts',(86.753210552202,62.8603214536186,12.2418843732614));
#67968=CARTESIAN_POINT('Ctrl Pts',(86.7520822810731,62.8594927010816,12.2336179471988));
#67969=CARTESIAN_POINT('Ctrl Pts',(86.749296409748,62.8572800408884,12.211589133669));
#67970=CARTESIAN_POINT('Ctrl Pts',(86.7477826072347,62.8558917132922,12.1978101852589));
#67971=CARTESIAN_POINT('Ctrl Pts',(86.7428025431166,62.8504959103562,12.1444475692518));
#67972=CARTESIAN_POINT('Ctrl Pts',(86.7409696098582,62.8464392205915,12.1047396041735));
#67973=CARTESIAN_POINT('Ctrl Pts',(86.7410589749626,62.8345149724814,11.9893751411073));
#67974=CARTESIAN_POINT('Ctrl Pts',(86.7478752831577,62.8265310814682,11.9138991982498));
#67975=CARTESIAN_POINT('Ctrl Pts',(86.7712715191255,62.8127130106134,11.784824310722));
#67976=CARTESIAN_POINT('Ctrl Pts',(86.7847581257179,62.8068881620656,11.7308593486531));
#67977=CARTESIAN_POINT('Ctrl Pts',(86.8047731226141,62.8002010235078,11.6684885787134));
#67978=CARTESIAN_POINT('Ctrl Pts',(86.8079183356741,62.7991923889187,11.659068628593));
#67979=CARTESIAN_POINT('Ctrl Pts',(86.8130185285439,62.7976215560043,11.6443697599716));
#67980=CARTESIAN_POINT('Ctrl Pts',(86.8148985357381,62.7970553418018,11.6390656292004));
#67981=CARTESIAN_POINT('Ctrl Pts',(86.8185297461466,62.7959857694399,11.62903305095));
#67982=CARTESIAN_POINT('Ctrl Pts',(86.820273868521,62.7954820668185,11.6243024760838));
#67983=CARTESIAN_POINT('Ctrl Pts',(86.8245409864969,62.7942732402089,11.612937773907));
#67984=CARTESIAN_POINT('Ctrl Pts',(86.8270915145438,62.7935697338764,11.606314152707));
#67985=CARTESIAN_POINT('Ctrl Pts',(86.8363212762383,62.7910885876214,11.5829313086721));
#67986=CARTESIAN_POINT('Ctrl Pts',(86.8433024251292,62.7893273737669,11.5662921268863));
#67987=CARTESIAN_POINT('Ctrl Pts',(86.8568627030759,62.7860982077692,11.5358096956931));
#67988=CARTESIAN_POINT('Ctrl Pts',(86.8633420674851,62.7846264287682,11.5219264894434));
#67989=CARTESIAN_POINT('Ctrl Pts',(86.8991752926949,62.7768324716451,11.4486377717621));
#67990=CARTESIAN_POINT('Ctrl Pts',(86.9328956309561,62.77066260478,11.3914757807092));
#67991=CARTESIAN_POINT('Ctrl Pts',(87.0128023029992,62.7576084276197,11.2774402711952));
#67992=CARTESIAN_POINT('Ctrl Pts',(87.0597439113232,62.7507365325286,11.2214089448764));
#67993=CARTESIAN_POINT('Ctrl Pts',(87.1224224945011,62.7421252329423,11.1584860495682));
#67994=CARTESIAN_POINT('Ctrl Pts',(87.1338245763913,62.7405791787491,11.1474605201462));
#67995=CARTESIAN_POINT('Ctrl Pts',(87.152515989458,62.7380743166155,11.1300518265597));
#67996=CARTESIAN_POINT('Ctrl Pts',(87.1596774556089,62.7371213335899,11.1235331877363));
#67997=CARTESIAN_POINT('Ctrl Pts',(87.1735559808104,62.7352866523315,11.1111876760583));
#67998=CARTESIAN_POINT('Ctrl Pts',(87.1802610984983,62.7344055500059,11.1053481762235));
#67999=CARTESIAN_POINT('Ctrl Pts',(87.1959621840866,62.7323539453808,11.091961376563));
#68000=CARTESIAN_POINT('Ctrl Pts',(87.205002436343,62.7311813508958,11.0844676343211));
#68001=CARTESIAN_POINT('Ctrl Pts',(87.2349106283793,62.7273286283388,11.0603676137202));
#68002=CARTESIAN_POINT('Ctrl Pts',(87.2561961454741,62.7246279843959,11.0442945248148));
#68003=CARTESIAN_POINT('Ctrl Pts',(87.3092895191518,62.7179824610759,11.0067675505312));
#68004=CARTESIAN_POINT('Ctrl Pts',(87.3415921612879,62.7140140732761,10.9860632174867));
#68005=CARTESIAN_POINT('Ctrl Pts',(87.4167386008631,62.7049481046193,10.9425659921023));
#68006=CARTESIAN_POINT('Ctrl Pts',(87.4600529630847,62.6998356123842,10.9207020514793));
#68007=CARTESIAN_POINT('Ctrl Pts',(87.5616385382153,62.68815776398,10.8765230210915));
#68008=CARTESIAN_POINT('Ctrl Pts',(87.620528822372,62.6816067513663,10.8559108080824));
#68009=CARTESIAN_POINT('Ctrl Pts',(87.6903679333165,62.6742218425332,10.8370999757573));
#68010=CARTESIAN_POINT('Ctrl Pts',(87.7000640618789,62.6732050309305,10.8346109238143));
#68011=CARTESIAN_POINT('Ctrl Pts',(87.7152722625885,62.6716243546968,10.8308979953796));
#68012=CARTESIAN_POINT('Ctrl Pts',(87.7207644347833,62.6710563946387,10.8295958679565));
#68013=CARTESIAN_POINT('Ctrl Pts',(87.7311733995009,62.669985619489,10.8272012116369));
#68014=CARTESIAN_POINT('Ctrl Pts',(87.7360880687867,62.6694824444908,10.8261012959068));
#68015=CARTESIAN_POINT('Ctrl Pts',(87.7479089375651,62.6682777200108,10.8235294976661));
#68016=CARTESIAN_POINT('Ctrl Pts',(87.7548211289282,62.6675777592842,10.8220859149863));
#68017=CARTESIAN_POINT('Ctrl Pts',(87.7791973950296,62.6651238706717,10.8172068505516));
#68018=CARTESIAN_POINT('Ctrl Pts',(87.7967225959644,62.6633858956163,10.8140806385057));
#68019=CARTESIAN_POINT('Ctrl Pts',(87.8291518133399,62.6602077265317,10.8089968373496));
#68020=CARTESIAN_POINT('Ctrl Pts',(87.8440353196457,62.6587636566323,10.8069334557988));
#68021=CARTESIAN_POINT('Ctrl Pts',(87.9224506713874,62.6512142320144,10.7974773835015));
#68022=CARTESIAN_POINT('Ctrl Pts',(87.9864424020208,62.6452522442995,10.7946270746109));
#68023=CARTESIAN_POINT('Ctrl Pts',(88.1199609341826,62.6327333142382,10.7987693895041));
#68024=CARTESIAN_POINT('Ctrl Pts',(88.1892343164074,62.626189479526,10.8066445604288));
#68025=CARTESIAN_POINT('Ctrl Pts',(88.2746226438355,62.6177857247768,10.8235397279944));
#68026=CARTESIAN_POINT('Ctrl Pts',(88.2916660001255,62.6160916433296,10.8272785006196));
#68027=CARTESIAN_POINT('Ctrl Pts',(88.3193309958117,62.6133104794803,10.8339475442777));
#68028=CARTESIAN_POINT('Ctrl Pts',(88.3300015623747,62.6122300912854,10.8366671560904));
#68029=CARTESIAN_POINT('Ctrl Pts',(88.3491433812361,62.6102772115095,10.8418118300876));
#68030=CARTESIAN_POINT('Ctrl Pts',(88.3576274477218,62.6094063786029,10.8441869929377));
#68031=CARTESIAN_POINT('Ctrl Pts',(88.3757776516177,62.6075315428667,10.8494724986596));
#68032=CARTESIAN_POINT('Ctrl Pts',(88.385435092201,62.606526705791,10.8524101832707));
#68033=CARTESIAN_POINT('Ctrl Pts',(88.4120432692606,62.6037372065946,10.8608519161765));
#68034=CARTESIAN_POINT('Ctrl Pts',(88.4289139243583,62.6019447918908,10.866597866962));
#68035=CARTESIAN_POINT('Ctrl Pts',(88.4569810053032,62.5989207250518,10.8768212125249));
#68036=CARTESIAN_POINT('Ctrl Pts',(88.4682451948143,62.5976955105722,10.8811067336158));
#68037=CARTESIAN_POINT('Ctrl Pts',(88.4976272202324,62.5944685153569,10.8927666250495));
#68038=CARTESIAN_POINT('Ctrl Pts',(88.5156379010013,62.5924589797896,10.9004001137468));
#68039=CARTESIAN_POINT('Ctrl Pts',(88.6012220653557,62.5827559232614,10.939028674083));
#68040=CARTESIAN_POINT('Ctrl Pts',(88.6661560173032,62.5749135399887,10.9754981660358));
#68041=CARTESIAN_POINT('Ctrl Pts',(88.7748062549928,62.5610482153719,11.0497420662984));
#68042=CARTESIAN_POINT('Ctrl Pts',(88.8198610111603,62.5550388882672,11.0852216938908));
#68043=CARTESIAN_POINT('Ctrl Pts',(88.869745794583,62.5481756287941,11.1302893566437));
#68044=CARTESIAN_POINT('Ctrl Pts',(88.8770414251558,62.5471662782208,11.1370376648898));
#68045=CARTESIAN_POINT('Ctrl Pts',(88.8883443961492,62.5455945830015,11.1477415981505));
#68046=CARTESIAN_POINT('Ctrl Pts',(88.8924056700894,62.545028215541,11.151639167899));
#68047=CARTESIAN_POINT('Ctrl Pts',(88.9000551195701,62.5439585387242,11.1590786086015));
#68048=CARTESIAN_POINT('Ctrl Pts',(88.9036481661449,62.5434548835483,11.1626148832188));
#68049=CARTESIAN_POINT('Ctrl Pts',(88.9122465863263,62.5422464217476,11.1711788356179));
#68050=CARTESIAN_POINT('Ctrl Pts',(88.917231086483,62.5415432302122,11.1762272468921));
#68051=CARTESIAN_POINT('Ctrl Pts',(88.9347252923499,62.5390645134546,11.1942452928932));
#68052=CARTESIAN_POINT('Ctrl Pts',(88.9470019555683,62.5373053718389,11.2074400754319));
#68053=CARTESIAN_POINT('Ctrl Pts',(88.9691707308139,62.53408076329,11.2323077897075));
#68054=CARTESIAN_POINT('Ctrl Pts',(88.9791403513253,62.5326114648582,11.2439062299215));
#68055=CARTESIAN_POINT('Ctrl Pts',(89.0310413237334,62.5248397364948,11.3065408089215));
#68056=CARTESIAN_POINT('Ctrl Pts',(89.0691562555416,62.5186887949476,11.360613900233));
#68057=CARTESIAN_POINT('Ctrl Pts',(89.1402993869349,62.505629442459,11.4803828552764));
#68058=CARTESIAN_POINT('Ctrl Pts',(89.1721808417437,62.4987329955045,11.5464610835943));
#68059=CARTESIAN_POINT('Ctrl Pts',(89.2038215845881,62.4900957292954,11.6297338543119));
#68060=CARTESIAN_POINT('Ctrl Pts',(89.2091757823394,62.488549889618,11.6446613909262));
#68061=CARTESIAN_POINT('Ctrl Pts',(89.2173468917407,62.4860452898067,11.6688590334791));
#68062=CARTESIAN_POINT('Ctrl Pts',(89.2203398312756,62.4850923523463,11.6780683951022));
#68063=CARTESIAN_POINT('Ctrl Pts',(89.2258783888689,62.4832577023811,11.6957979444549));
#68064=CARTESIAN_POINT('Ctrl Pts',(89.2284404166907,62.4823765853551,11.704312450803));
#68065=CARTESIAN_POINT('Ctrl Pts',(89.2341781972224,62.4803248618264,11.7241330618631));
#68066=CARTESIAN_POINT('Ctrl Pts',(89.2372868869979,62.4791521623453,11.7354574876019));
#68067=CARTESIAN_POINT('Ctrl Pts',(89.2469419002753,62.4752986946338,11.7726415753913));
#68068=CARTESIAN_POINT('Ctrl Pts',(89.2528300575248,62.4725973993981,11.79866241952));
#68069=CARTESIAN_POINT('Ctrl Pts',(89.265179396688,62.4659498580604,11.8625153029414));
#68070=CARTESIAN_POINT('Ctrl Pts',(89.2707530312328,62.461980084049,11.900489853666));
#68071=CARTESIAN_POINT('Ctrl Pts',(89.2794593312291,62.4529141160188,11.9868788144894));
#68072=CARTESIAN_POINT('Ctrl Pts',(89.2815544512035,62.4478030726399,12.0353394041807));
#68073=CARTESIAN_POINT('Ctrl Pts',(89.2800023232546,62.4361275012476,12.1460834024374));
#68074=CARTESIAN_POINT('Ctrl Pts',(89.2745478735421,62.4295773198751,12.2082301121597));
#68075=CARTESIAN_POINT('Ctrl Pts',(89.2629462537092,62.4221932266182,12.2796135867246));
#68076=CARTESIAN_POINT('Ctrl Pts',(89.2612237193261,62.4211764415598,12.2894745198848));
#68077=CARTESIAN_POINT('Ctrl Pts',(89.2583477839624,62.4195957976267,12.3048626418574));
#68078=CARTESIAN_POINT('Ctrl Pts',(89.2572738835781,62.4190278435774,12.3104039023854));
#68079=CARTESIAN_POINT('Ctrl Pts',(89.255171880457,62.4179570729542,12.3208758451309));
#68080=CARTESIAN_POINT('Ctrl Pts',(89.2541513827881,62.4174538965239,12.3258076326089));
#68081=CARTESIAN_POINT('Ctrl Pts',(89.2516296345187,62.4162491598077,12.3376394076895));
#68082=CARTESIAN_POINT('Ctrl Pts',(89.2501001246333,62.4155491883655,12.3445332072949));
#68083=CARTESIAN_POINT('Ctrl Pts',(89.244513063512,62.4130952176246,12.3687578668005));
#68084=CARTESIAN_POINT('Ctrl Pts',(89.2401484677956,62.4113571725731,12.3860171302879));
#68085=CARTESIAN_POINT('Ctrl Pts',(89.2314330436529,62.408178850244,12.4176659301506));
#68086=CARTESIAN_POINT('Ctrl Pts',(89.2271870719114,62.4067346972337,12.432080318919));
#68087=CARTESIAN_POINT('Ctrl Pts',(89.2035260151192,62.3991845513688,12.5074444266972));
#68088=CARTESIAN_POINT('Ctrl Pts',(89.1797809556355,62.3932219515589,12.5669432457179));
#68089=CARTESIAN_POINT('Ctrl Pts',(89.1210479956575,62.3807034005792,12.6869169268394));
#68090=CARTESIAN_POINT('Ctrl Pts',(89.0853626190001,62.3741605695807,12.7467988218024));
#68091=CARTESIAN_POINT('Ctrl Pts',(89.0348245758325,62.3657577642902,12.8176566415711));
#68092=CARTESIAN_POINT('Ctrl Pts',(89.0244013519534,62.364063565159,12.8316514216929));
#68093=CARTESIAN_POINT('Ctrl Pts',(89.0069354096129,62.3612822479815,12.8541205011843));
#68094=CARTESIAN_POINT('Ctrl Pts',(89.0000645723537,62.3602018254031,12.8627261245267));
#68095=CARTESIAN_POINT('Ctrl Pts',(88.9874967836739,62.3582489085707,12.8780539721045));
#68096=CARTESIAN_POINT('Ctrl Pts',(88.9818400409602,62.3573780732614,12.8848084190568));
#68097=CARTESIAN_POINT('Ctrl Pts',(88.9695524438061,62.3555032600932,12.899174113933));
#68098=CARTESIAN_POINT('Ctrl Pts',(88.9629002557104,62.3544984481892,12.9067661861288));
#68099=CARTESIAN_POINT('Ctrl Pts',(88.9442556777132,62.3517090953319,12.927540135494));
#68100=CARTESIAN_POINT('Ctrl Pts',(88.9320758217262,62.3499168031515,12.9405494913639));
#68101=CARTESIAN_POINT('Ctrl Pts',(88.91120774864,62.3468929722629,12.9619192088314));
#68102=CARTESIAN_POINT('Ctrl Pts',(88.9026664921936,62.3456678705976,12.970420290242));
#68103=CARTESIAN_POINT('Ctrl Pts',(88.8799489236012,62.3424412366849,12.9923963938229));
#68104=CARTESIAN_POINT('Ctrl Pts',(88.8655806194148,62.3404319516515,13.0056671632343));
#68105=CARTESIAN_POINT('Ctrl Pts',(88.7951641216555,62.3307308995756,13.0677537629437));
#68106=CARTESIAN_POINT('Ctrl Pts',(88.7352149377256,62.3228903338298,13.1119129491414));
#68107=CARTESIAN_POINT('Ctrl Pts',(88.6228297269834,62.3090244060096,13.1803819340748));
#68108=CARTESIAN_POINT('Ctrl Pts',(88.5719311668976,62.3030127076248,13.2068509874287));
#68109=CARTESIAN_POINT('Ctrl Pts',(88.5103050122751,62.2961471849633,13.2337727751677));
#68110=CARTESIAN_POINT('Ctrl Pts',(88.501151844084,62.2951378245419,13.2376441190833));
#68111=CARTESIAN_POINT('Ctrl Pts',(88.4867442014944,62.2935661173436,13.2435394418066));
#68112=CARTESIAN_POINT('Ctrl Pts',(88.4815204377722,62.2929997476592,13.2456364713034));
#68113=CARTESIAN_POINT('Ctrl Pts',(88.4715918361634,62.2919300691468,13.2495457643093));
#68114=CARTESIAN_POINT('Ctrl Pts',(88.4668900937431,62.2914264144808,13.2513647709104));
#68115=CARTESIAN_POINT('Ctrl Pts',(88.4555461109623,62.2902179572032,13.2556760400377));
#68116=CARTESIAN_POINT('Ctrl Pts',(88.4488935667797,62.2895147696475,13.2581407458328));
#68117=CARTESIAN_POINT('Ctrl Pts',(88.4252721772428,62.287036084062,13.2666678300997));
#68118=CARTESIAN_POINT('Ctrl Pts',(88.408194066485,62.2852769690884,13.2724251607249));
#68119=CARTESIAN_POINT('Ctrl Pts',(88.3764063644706,62.2820524191901,13.282393040631));
#68120=CARTESIAN_POINT('Ctrl Pts',(88.3617327589074,62.2805831527074,13.2867048898454));
#68121=CARTESIAN_POINT('Ctrl Pts',(88.2832901774769,62.2728117103869,13.3082239202145));
#68122=CARTESIAN_POINT('Ctrl Pts',(88.2183243942324,62.266661012315,13.3207033314787));
#68123=CARTESIAN_POINT('Ctrl Pts',(88.0798879341141,62.2536015935324,13.3362438765491));
#68124=CARTESIAN_POINT('Ctrl Pts',(88.0065406774849,62.2467048311341,13.3381015112467));
#68125=CARTESIAN_POINT('Ctrl Pts',(87.9176221056591,62.2380672313637,13.3326617742859));
#68126=CARTESIAN_POINT('Ctrl Pts',(87.901813929081,62.2365213945311,13.3313971036218));
#68127=CARTESIAN_POINT('Ctrl Pts',(87.8763978805762,62.2340167981256,13.3288840167805));
#68128=CARTESIAN_POINT('Ctrl Pts',(87.8667729144214,62.2330638611957,13.3278210274302));
#68129=CARTESIAN_POINT('Ctrl Pts',(87.8483351807288,62.2312292114518,13.3255710453545));
#68130=CARTESIAN_POINT('Ctrl Pts',(87.8395208366278,62.2303480941103,13.3244013461605));
#68131=CARTESIAN_POINT('Ctrl Pts',(87.8190953670635,62.2282963686421,13.3214722289983));
#68132=CARTESIAN_POINT('Ctrl Pts',(87.8074951481664,62.2271236675252,13.3196441510184));
#68133=CARTESIAN_POINT('Ctrl Pts',(87.7696328270019,62.2232701887127,13.3131380993795));
#68134=CARTESIAN_POINT('Ctrl Pts',(87.7434947366105,62.2205688838502,13.3077939493914));
#68135=CARTESIAN_POINT('Ctrl Pts',(87.6802183364985,62.2139213128436,13.2927662722651));
#68136=CARTESIAN_POINT('Ctrl Pts',(87.6433154714811,62.209951518508,13.2822151990422));
#68137=CARTESIAN_POINT('Ctrl Pts',(87.5610003636374,62.200885550192,13.2545914120624));
#68138=CARTESIAN_POINT('Ctrl Pts',(87.5159730832973,62.1957745277555,13.2365541499383));
#68139=CARTESIAN_POINT('Ctrl Pts',(87.4157226182924,62.1841034336349,13.189574573481));
#68140=CARTESIAN_POINT('Ctrl Pts',(87.361365105638,62.1775576871242,13.1590470561495));
#68141=CARTESIAN_POINT('Ctrl Pts',(87.3011922078794,62.1701869844216,13.1191719957983));
#68142=CARTESIAN_POINT('Ctrl Pts',(87.2929892300229,62.1691794445907,13.1135967310127));
#68143=CARTESIAN_POINT('Ctrl Pts',(87.280190913868,62.167604071799,13.1046772150821));
#68144=CARTESIAN_POINT('Ctrl Pts',(87.2755515539515,62.1670322871443,13.1013974431837));
#68145=CARTESIAN_POINT('Ctrl Pts',(87.2669730803864,62.1659738993181,13.0952461809038));
#68146=CARTESIAN_POINT('Ctrl Pts',(87.2630284318849,62.1654868006496,13.0923831122532));
#68147=CARTESIAN_POINT('Ctrl Pts',(87.2590170003332,62.164990941786,13.0894361625684));
#68148=CARTESIAN_POINT('Ctrl Pts',(87.2589338756575,62.1649806663939,13.0893750804359));
#68149=CARTESIAN_POINT('Ctrl Pts',(87.2587683973564,62.164960210461,13.0892534517079));
#68150=CARTESIAN_POINT('Ctrl Pts',(87.2586860435144,62.1649500298977,13.0891929052359));
#68151=CARTESIAN_POINT('Ctrl Pts',(87.2585219935161,62.1649297496186,13.0890722653085));
#68152=CARTESIAN_POINT('Ctrl Pts',(87.25844029735,62.1649196499052,13.0890121720844));
#68153=CARTESIAN_POINT('Ctrl Pts',(87.2582774551191,62.1648995180339,13.0888923602115));
#68154=CARTESIAN_POINT('Ctrl Pts',(87.2581963090161,62.1648894858743,13.0888326417317));
#68155=CARTESIAN_POINT('Ctrl Pts',(87.2580344644899,62.1648694764549,13.088713504544));
#68156=CARTESIAN_POINT('Ctrl Pts',(87.2579537658418,62.1648594991696,13.0886540858292));
#68157=CARTESIAN_POINT('Ctrl Pts',(87.2577927172652,62.1648395872686,13.0885354757635));
#68158=CARTESIAN_POINT('Ctrl Pts',(87.2577123673709,62.164829652659,13.0884762845601));
#68159=CARTESIAN_POINT('Ctrl Pts',(87.2575519213096,62.1648098143674,13.088358059888));
#68160=CARTESIAN_POINT('Ctrl Pts',(87.2574718251357,62.164799910686,13.0882990265015));
#68161=CARTESIAN_POINT('Ctrl Pts',(87.2573117946532,62.1647801228943,13.0881810500028));
#68162=CARTESIAN_POINT('Ctrl Pts',(87.2572318602742,62.1647702387761,13.0881221068924));
#68163=CARTESIAN_POINT('Ctrl Pts',(87.2570720638502,62.1647504790402,13.0880042450705));
#68164=CARTESIAN_POINT('Ctrl Pts',(87.2569922018351,62.1647406034266,13.0879453264025));
#68165=CARTESIAN_POINT('Ctrl Pts',(87.2568324626802,62.1647208498836,13.08782744899));
#68166=CARTESIAN_POINT('Ctrl Pts',(87.2567525856333,62.1647109719655,13.0877684903037));
#68167=CARTESIAN_POINT('Ctrl Pts',(87.2565927311676,62.1646912032691,13.0876504698856));
#68168=CARTESIAN_POINT('Ctrl Pts',(87.256512753621,62.1646813124743,13.087591408018));
#68169=CARTESIAN_POINT('Ctrl Pts',(87.2508373134831,62.1639794167997,13.0833991755097));
#68170=CARTESIAN_POINT('Ctrl Pts',(87.2452756632314,62.1632904898426,13.0792199368835));
#68171=CARTESIAN_POINT('Ctrl Pts',(87.2329558257454,62.1617611950182,13.069802948668));
#68172=CARTESIAN_POINT('Ctrl Pts',(87.2262155353611,62.1609223058157,13.0645421645983));
#68173=CARTESIAN_POINT('Ctrl Pts',(87.2069824453511,62.1585204073847,13.0492157100055));
#68174=CARTESIAN_POINT('Ctrl Pts',(87.1946259607741,62.1569672034051,13.0389804022322));
#68175=CARTESIAN_POINT('Ctrl Pts',(87.181857685817,62.1553471829244,13.0279894317539));
#68176=CARTESIAN_POINT('Ctrl Pts',(87.1812500062644,62.1552700449772,13.0274653357362));
#68177=CARTESIAN_POINT('Ctrl Pts',(87.180642835277,62.1551929346177,13.0269406740237));
#68178=CARTESIAN_POINT('Origin',(88.011,66.41344859951,12.066));
#68179=CARTESIAN_POINT('',(87.1806429942553,61.1927093932679,13.0269408113983));
#68180=CARTESIAN_POINT('',(87.1806428320421,61.3633558149692,13.0269406712284));
#68181=CARTESIAN_POINT('',(87.1806428354228,66.41344859951,13.0269406741497));
#68182=CARTESIAN_POINT('',(86.7410004953938,61.8782514005452,12.0671217397436));
#68183=CARTESIAN_POINT('Ctrl Pts',(87.1806429942554,61.1927093932679,13.0269408113983));
#68184=CARTESIAN_POINT('Ctrl Pts',(87.226202739937,61.1983609392697,13.0663093693343));
#68185=CARTESIAN_POINT('Ctrl Pts',(87.2745233771969,61.2040483236492,13.1024044361032));
#68186=CARTESIAN_POINT('Ctrl Pts',(87.3398033310188,61.2115377385228,13.1442829214061));
#68187=CARTESIAN_POINT('Ctrl Pts',(87.3545464917767,61.2132169908147,13.1533213651565));
#68188=CARTESIAN_POINT('Ctrl Pts',(87.3789344233228,61.2159789596357,13.167595842728));
#68189=CARTESIAN_POINT('Ctrl Pts',(87.3884710784503,61.2170551410657,13.1730131061858));
#68190=CARTESIAN_POINT('Ctrl Pts',(87.4057913394993,61.2190036867216,13.1825572407154));
#68191=CARTESIAN_POINT('Ctrl Pts',(87.4135501138054,61.2198744265838,13.186727985794));
#68192=CARTESIAN_POINT('Ctrl Pts',(87.4303228075975,61.2217527048303,13.1955205187292));
#68193=CARTESIAN_POINT('Ctrl Pts',(87.4393498166435,61.2227611042524,13.2001158038841));
#68194=CARTESIAN_POINT('Ctrl Pts',(87.4645542245857,61.2255706365563,13.2125689926564));
#68195=CARTESIAN_POINT('Ctrl Pts',(87.4808442502163,61.2273797059881,13.2201915942497));
#68196=CARTESIAN_POINT('Ctrl Pts',(87.5178291351539,61.2314746860894,13.2365498283068));
#68197=CARTESIAN_POINT('Ctrl Pts',(87.5386043843642,61.2337664975491,13.2450872012963));
#68198=CARTESIAN_POINT('Ctrl Pts',(87.6092134874384,61.2415315852857,13.2719377200415));
#68199=CARTESIAN_POINT('Ctrl Pts',(87.6599609025706,61.2470756255832,13.2876743688528));
#68200=CARTESIAN_POINT('Ctrl Pts',(87.7935595927618,61.2615398492225,13.3200906863389));
#68201=CARTESIAN_POINT('Ctrl Pts',(87.8773693634491,61.2704976609898,13.3317683761111));
#68202=CARTESIAN_POINT('Ctrl Pts',(87.9732851900097,61.2803264147909,13.3354925817345));
#68203=CARTESIAN_POINT('Ctrl Pts',(87.9848509626102,61.2815043310443,13.3357834791417));
#68204=CARTESIAN_POINT('Ctrl Pts',(88.0024612729697,61.2832853737246,13.3359856668994));
#68205=CARTESIAN_POINT('Ctrl Pts',(88.0085033752815,61.2838942139818,13.3360119197725));
#68206=CARTESIAN_POINT('Ctrl Pts',(88.019015068809,61.2849493069948,13.3359825724927));
#68207=CARTESIAN_POINT('Ctrl Pts',(88.0234843566758,61.2853965855964,13.3359465023504));
#68208=CARTESIAN_POINT('Ctrl Pts',(88.0341075069042,61.2864566486703,13.3358046779072));
#68209=CARTESIAN_POINT('Ctrl Pts',(88.0402609381663,61.2870682604056,13.335677785987));
#68210=CARTESIAN_POINT('Ctrl Pts',(88.0589150464705,61.2889157031898,13.3351574213276));
#68211=CARTESIAN_POINT('Ctrl Pts',(88.0714116832344,61.2901442641383,13.3346240118687));
#68212=CARTESIAN_POINT('Ctrl Pts',(88.1347917163672,61.2963391007048,13.3309799269565));
#68213=CARTESIAN_POINT('Ctrl Pts',(88.1854705936178,61.3011749427533,13.3249917987697));
#68214=CARTESIAN_POINT('Ctrl Pts',(88.3269870846292,61.3147063336274,13.2995567484761));
#68215=CARTESIAN_POINT('Ctrl Pts',(88.4162328832904,61.3232923762391,13.2731847002324));
#68216=CARTESIAN_POINT('Ctrl Pts',(88.5266621450235,61.3347600478721,13.2269129237382));
#68217=CARTESIAN_POINT('Ctrl Pts',(88.5511776277616,61.337361531208,13.2157104656436));
#68218=CARTESIAN_POINT('Ctrl Pts',(88.5850962488991,61.3410536478627,13.1988868761668));
#68219=CARTESIAN_POINT('Ctrl Pts',(88.5948128305017,61.3421223011867,13.1939103413491));
#68220=CARTESIAN_POINT('Ctrl Pts',(88.6124264363243,61.3440806079502,13.1846006259585));
#68221=CARTESIAN_POINT('Ctrl Pts',(88.6203439220776,61.3449688157178,13.180307449877));
#68222=CARTESIAN_POINT('Ctrl Pts',(88.636308819522,61.3467764981403,13.1714296230262));
#68223=CARTESIAN_POINT('Ctrl Pts',(88.6443530586291,61.3476960896704,13.1668404347347));
#68224=CARTESIAN_POINT('Ctrl Pts',(88.664270802737,61.3499955643799,13.1551869140628));
#68225=CARTESIAN_POINT('Ctrl Pts',(88.676080217368,61.3513792163533,13.1480162388583));
#68226=CARTESIAN_POINT('Ctrl Pts',(88.7237582802333,61.3570514906309,13.1179907160773));
#68227=CARTESIAN_POINT('Ctrl Pts',(88.7585799835022,61.3613976006141,13.0935368368419));
#68228=CARTESIAN_POINT('Ctrl Pts',(88.8511827005763,61.3735549601707,13.0213045195983));
#68229=CARTESIAN_POINT('Ctrl Pts',(88.9060602632938,61.3814686671783,12.9700897233082));
#68230=CARTESIAN_POINT('Ctrl Pts',(88.9919041594862,61.3950012984119,12.8744555545538));
#68231=CARTESIAN_POINT('Ctrl Pts',(89.0251551104515,61.4006166018615,12.8323318759416));
#68232=CARTESIAN_POINT('Ctrl Pts',(89.0612864701626,61.4071026191606,12.7800704712377));
#68233=CARTESIAN_POINT('Ctrl Pts',(89.0668295745033,61.4081096824103,12.7718485950256));
#68234=CARTESIAN_POINT('Ctrl Pts',(89.0753655271757,61.4096786967616,12.7588619352497));
#68235=CARTESIAN_POINT('Ctrl Pts',(89.0784237862478,61.4102446480521,12.7541410479154));
#68236=CARTESIAN_POINT('Ctrl Pts',(89.084165076899,61.4113141920218,12.745148115447));
#68237=CARTESIAN_POINT('Ctrl Pts',(89.0868540583634,61.4118181258645,12.7408803538612));
#68238=CARTESIAN_POINT('Ctrl Pts',(89.0932705223589,61.4130281625144,12.7305607792229));
#68239=CARTESIAN_POINT('Ctrl Pts',(89.096972778952,61.4137326402702,12.7244934661483));
#68240=CARTESIAN_POINT('Ctrl Pts',(89.1099227638895,61.4162207128967,12.7028645260095));
#68241=CARTESIAN_POINT('Ctrl Pts',(89.118889226718,61.417987762615,12.6871354507227));
#68242=CARTESIAN_POINT('Ctrl Pts',(89.1348522018291,61.4212296792539,12.6576866943066));
#68243=CARTESIAN_POINT('Ctrl Pts',(89.1419411249495,61.4227083610607,12.6440217507854));
#68244=CARTESIAN_POINT('Ctrl Pts',(89.1784772357889,61.4305642392608,12.5703460703639));
#68245=CARTESIAN_POINT('Ctrl Pts',(89.2034028057491,61.4367868304831,12.5082050131075));
#68246=CARTESIAN_POINT('Ctrl Pts',(89.2447796625721,61.4498077663473,12.3756362576421));
#68247=CARTESIAN_POINT('Ctrl Pts',(89.2603471258637,61.4565921357858,12.3051982879379));
#68248=CARTESIAN_POINT('Ctrl Pts',(89.2719724658581,61.4651205091818,12.2179983969105));
#68249=CARTESIAN_POINT('Ctrl Pts',(89.273784087429,61.4666771594713,12.202129960316));
#68250=CARTESIAN_POINT('Ctrl Pts',(89.2762150400988,61.469195084633,12.1765674402439));
#68251=CARTESIAN_POINT('Ctrl Pts',(89.2770232738425,61.4701504239857,12.1668925845295));
#68252=CARTESIAN_POINT('Ctrl Pts',(89.2783587093729,61.4719869451115,12.1483460621131));
#68253=CARTESIAN_POINT('Ctrl Pts',(89.2789038635231,61.4728675102045,12.1394762193943));
#68254=CARTESIAN_POINT('Ctrl Pts',(89.2799507912079,61.4749138442851,12.1189213808966));
#68255=CARTESIAN_POINT('Ctrl Pts',(89.2803843078585,61.4760816687021,12.1072339482793));
#68256=CARTESIAN_POINT('Ctrl Pts',(89.2812698902079,61.4798999463446,12.0691742707471));
#68257=CARTESIAN_POINT('Ctrl Pts',(89.2810617980457,61.482570402152,12.0427957863362));
#68258=CARTESIAN_POINT('Ctrl Pts',(89.2785598504354,61.4891224931139,11.9787240779547));
#68259=CARTESIAN_POINT('Ctrl Pts',(89.2754059352939,61.4930267431569,11.9410918475918));
#68260=CARTESIAN_POINT('Ctrl Pts',(89.2643048376743,61.5020905419596,11.8549594080511));
#68261=CARTESIAN_POINT('Ctrl Pts',(89.2552093068928,61.5072678714401,11.8066667097667));
#68262=CARTESIAN_POINT('Ctrl Pts',(89.2281916228537,61.5190514146889,11.6982049817284));
#68263=CARTESIAN_POINT('Ctrl Pts',(89.2085572671254,61.5256434354852,11.6385802708363));
#68264=CARTESIAN_POINT('Ctrl Pts',(89.1808091521236,61.533056949719,11.5714853649247));
#68265=CARTESIAN_POINT('Ctrl Pts',(89.1769151936337,61.5340635645813,11.5623731936873));
#68266=CARTESIAN_POINT('Ctrl Pts',(89.1706217593238,61.5356378866358,11.548110399672));
#68267=CARTESIAN_POINT('Ctrl Pts',(89.1682938354428,61.5362095362179,11.5429290240215));
#68268=CARTESIAN_POINT('Ctrl Pts',(89.1638403235007,61.5372830838689,11.5331919133314));
#68269=CARTESIAN_POINT('Ctrl Pts',(89.1617224284848,61.5377853733405,11.5286331204347));
#68270=CARTESIAN_POINT('Ctrl Pts',(89.156594195425,61.5389823720837,11.5177639037361));
#68271=CARTESIAN_POINT('Ctrl Pts',(89.1535587111232,61.5396755483464,11.5114655305448));
#68272=CARTESIAN_POINT('Ctrl Pts',(89.14281586985,61.5420774524038,11.4896378021043));
#68273=CARTESIAN_POINT('Ctrl Pts',(89.134842125066,61.5437711118576,11.4742403089391));
#68274=CARTESIAN_POINT('Ctrl Pts',(89.113855017367,61.5480252175316,11.4356692392767));
#68275=CARTESIAN_POINT('Ctrl Pts',(89.1004245704549,61.5505659213823,11.4127309658727));
#68276=CARTESIAN_POINT('Ctrl Pts',(89.0557922227107,61.5585246538168,11.3417122335432));
#68277=CARTESIAN_POINT('Ctrl Pts',(89.0220510698514,61.5638656778992,11.295311950015));
#68278=CARTESIAN_POINT('Ctrl Pts',(88.9394071484531,61.5759464932351,11.1964734289822));
#68279=CARTESIAN_POINT('Ctrl Pts',(88.8889789013189,61.5826865179429,11.1455834825062));
#68280=CARTESIAN_POINT('Ctrl Pts',(88.8224299876539,61.5911621594658,11.0888948065194));
#68281=CARTESIAN_POINT('Ctrl Pts',(88.8101249990369,61.5927131332464,11.0788058115395));
#68282=CARTESIAN_POINT('Ctrl Pts',(88.7900221656423,61.5952241294975,11.0629454251947));
#68283=CARTESIAN_POINT('Ctrl Pts',(88.7823417024375,61.596178276283,11.0570272651263));
#68284=CARTESIAN_POINT('Ctrl Pts',(88.7674906014966,61.5980139905157,11.0458524576989));
#68285=CARTESIAN_POINT('Ctrl Pts',(88.7603310135025,61.5988949526088,11.040582007087));
#68286=CARTESIAN_POINT('Ctrl Pts',(88.7436039352837,61.6009444295243,11.0285372807499));
#68287=CARTESIAN_POINT('Ctrl Pts',(88.733996992695,61.6021150205043,11.0218195823129));
#68288=CARTESIAN_POINT('Ctrl Pts',(88.7023402600098,61.6059527369942,11.0003297774613));
#68289=CARTESIAN_POINT('Ctrl Pts',(88.6799220277723,61.6086401519575,10.9861169365844));
#68290=CARTESIAN_POINT('Ctrl Pts',(88.6242867486978,61.6152445478641,10.9532421660584));
#68291=CARTESIAN_POINT('Ctrl Pts',(88.590645310124,61.6191846396407,10.9353535975616));
#68292=CARTESIAN_POINT('Ctrl Pts',(88.5122164309577,61.6282501476519,10.8980703179564));
#68293=CARTESIAN_POINT('Ctrl Pts',(88.4670114113355,61.6333917404362,10.8796903120918));
#68294=CARTESIAN_POINT('Ctrl Pts',(88.3617473026455,61.6451159608629,10.8437980755069));
#68295=CARTESIAN_POINT('Ctrl Pts',(88.3012138961776,61.651684309547,10.828026048106));
#68296=CARTESIAN_POINT('Ctrl Pts',(88.2299044629803,61.6590863666561,10.8149679612656));
#68297=CARTESIAN_POINT('Ctrl Pts',(88.2200304442919,61.6601038679105,10.8132803098658));
#68298=CARTESIAN_POINT('Ctrl Pts',(88.2045604724411,61.6616854468799,10.8108242257314));
#68299=CARTESIAN_POINT('Ctrl Pts',(88.1989779641956,61.6622536262999,10.8099760470663));
#68300=CARTESIAN_POINT('Ctrl Pts',(88.1884048909593,61.6633247015835,10.8084417002965));
#68301=CARTESIAN_POINT('Ctrl Pts',(88.1834158400728,61.6638279583402,10.8077479773424));
#68302=CARTESIAN_POINT('Ctrl Pts',(88.171423457607,61.6650327421636,10.8061531175499));
#68303=CARTESIAN_POINT('Ctrl Pts',(88.1644164746966,61.6657326811863,10.8052806629401));
#68304=CARTESIAN_POINT('Ctrl Pts',(88.139729985067,61.6681858268034,10.8024157697009));
#68305=CARTESIAN_POINT('Ctrl Pts',(88.1220149268341,61.6699230956557,10.8007362655214));
#68306=CARTESIAN_POINT('Ctrl Pts',(88.0892954620566,61.6730996258294,10.7983268409895));
#68307=CARTESIAN_POINT('Ctrl Pts',(88.074302830087,61.6745427657311,10.7974897626058));
#68308=CARTESIAN_POINT('Ctrl Pts',(87.9954649992886,61.6820838362316,10.7944893949248));
#68309=CARTESIAN_POINT('Ctrl Pts',(87.9315334858944,61.6880387094762,10.7968793578557));
#68310=CARTESIAN_POINT('Ctrl Pts',(87.7987559737044,61.700561632184,10.811920470054));
#68311=CARTESIAN_POINT('Ctrl Pts',(87.7302385640439,61.7071167161125,10.825462338102));
#68312=CARTESIAN_POINT('Ctrl Pts',(87.6464175564511,61.7155311713836,10.8493309375516));
#68313=CARTESIAN_POINT('Ctrl Pts',(87.6297506195043,61.7172239940159,10.8544502459733));
#68314=CARTESIAN_POINT('Ctrl Pts',(87.6027402170429,61.7200036371134,10.863359093958));
#68315=CARTESIAN_POINT('Ctrl Pts',(87.5923308708438,61.7210837777869,10.8669431452794));
#68316=CARTESIAN_POINT('Ctrl Pts',(87.573676054421,61.7230365610186,10.8736387231184));
#68317=CARTESIAN_POINT('Ctrl Pts',(87.5654137575607,61.7239075479385,10.8767016612133));
#68318=CARTESIAN_POINT('Ctrl Pts',(87.5564992318225,61.7248541601265,10.8801123199549));
#68319=CARTESIAN_POINT('Ctrl Pts',(87.5558144310191,61.7249269215843,10.8803750020591));
#68320=CARTESIAN_POINT('Ctrl Pts',(87.5547625100692,61.7250387582622,10.8807795531267));
#68321=CARTESIAN_POINT('Ctrl Pts',(87.5543952263649,61.7250778193648,10.8809210002714));
#68322=CARTESIAN_POINT('Ctrl Pts',(87.5538322525775,61.7251377119292,10.8811381115352));
#68323=CARTESIAN_POINT('Ctrl Pts',(87.5536365150372,61.7251585393026,10.8812136535888));
#68324=CARTESIAN_POINT('Ctrl Pts',(87.5530826468201,61.7252174836991,10.8814275686724));
#68325=CARTESIAN_POINT('Ctrl Pts',(87.5527245605298,61.7252556045258,10.8815660554584));
#68326=CARTESIAN_POINT('Ctrl Pts',(87.5520467871796,61.7253277813617,10.8818285318353));
#68327=CARTESIAN_POINT('Ctrl Pts',(87.5517270873131,61.7253618362699,10.8819524886031));
#68328=CARTESIAN_POINT('Ctrl Pts',(87.5511216901121,61.7254263425105,10.8821875004668));
#68329=CARTESIAN_POINT('Ctrl Pts',(87.5508359826368,61.7254567929691,10.8822985295776));
#68330=CARTESIAN_POINT('Ctrl Pts',(87.5502947119431,61.7255144958882,10.8825090989883));
#68331=CARTESIAN_POINT('Ctrl Pts',(87.5500391406471,61.7255417476572,10.8826086186872));
#68332=CARTESIAN_POINT('Ctrl Pts',(87.549554755207,61.7255934098882,10.8827974195494));
#68333=CARTESIAN_POINT('Ctrl Pts',(87.5493259346289,61.7256178198007,10.8828866843406));
#68334=CARTESIAN_POINT('Ctrl Pts',(87.5488920745094,61.7256641122354,10.8830560817768));
#68335=CARTESIAN_POINT('Ctrl Pts',(87.5486870298516,61.725685994318,10.8831362013761));
#68336=CARTESIAN_POINT('Ctrl Pts',(87.5482981034366,61.7257275076507,10.8832882879127));
#68337=CARTESIAN_POINT('Ctrl Pts',(87.5481142175871,61.7257471385503,10.8833602444397));
#68338=CARTESIAN_POINT('Ctrl Pts',(87.547765302289,61.7257843934745,10.8834968726241));
#68339=CARTESIAN_POINT('Ctrl Pts',(87.5476002695476,61.7258020172203,10.8835615359632));
#68340=CARTESIAN_POINT('Ctrl Pts',(87.5472870252589,61.7258354733534,10.8836843473908));
#68341=CARTESIAN_POINT('Ctrl Pts',(87.5471388110959,61.7258513055146,10.8837424888053));
#68342=CARTESIAN_POINT('Ctrl Pts',(87.5468574054316,61.725881369135,10.8838529396122));
#68343=CARTESIAN_POINT('Ctrl Pts',(87.5467242117966,61.7258956004162,10.8839052436609));
#68344=CARTESIAN_POINT('Ctrl Pts',(87.546471255137,61.7259226312072,10.884004627016));
#68345=CARTESIAN_POINT('Ctrl Pts',(87.5463514903956,61.7259354305739,10.8840517020267));
#68346=CARTESIAN_POINT('Ctrl Pts',(87.5461239800973,61.7259597474311,10.8841411676831));
#68347=CARTESIAN_POINT('Ctrl Pts',(87.5460162331613,61.7259712648059,10.8841835548688));
#68348=CARTESIAN_POINT('Ctrl Pts',(87.5458115050845,61.7259931508957,10.8842641263541));
#68349=CARTESIAN_POINT('Ctrl Pts',(87.5457145229153,61.7260035195085,10.884302307831));
#68350=CARTESIAN_POINT('Ctrl Pts',(87.5455302102126,61.7260232265774,10.8843748971836));
#68351=CARTESIAN_POINT('Ctrl Pts',(87.5454428787162,61.7260325649649,10.8844093028326));
#68352=CARTESIAN_POINT('Ctrl Pts',(87.5343117565712,61.7272229135989,10.8887960132382));
#68353=CARTESIAN_POINT('Ctrl Pts',(87.5233300207363,61.7284090700988,10.8933027353222));
#68354=CARTESIAN_POINT('Ctrl Pts',(87.486257465773,61.7324550371401,10.9091274622259));
#68355=CARTESIAN_POINT('Ctrl Pts',(87.4604866248465,61.7353387217691,10.9211666098219));
#68356=CARTESIAN_POINT('Ctrl Pts',(87.3973577272725,61.7425910885303,10.9532823833756));
#68357=CARTESIAN_POINT('Ctrl Pts',(87.3605625577542,61.7469899738083,10.9743830338249));
#68358=CARTESIAN_POINT('Ctrl Pts',(87.2545094905754,61.7601843116504,11.0424678188431));
#68359=CARTESIAN_POINT('Ctrl Pts',(87.1887610927681,61.7690748134121,11.0944963736558));
#68360=CARTESIAN_POINT('Ctrl Pts',(87.1113234548237,61.7802588183569,11.1693063588163));
#68361=CARTESIAN_POINT('Ctrl Pts',(87.0945173811954,61.7827345799203,11.1864903452943));
#68362=CARTESIAN_POINT('Ctrl Pts',(87.0726913868365,61.7860060052116,11.2101127332265));
#68363=CARTESIAN_POINT('Ctrl Pts',(87.0672325659757,61.7868291470079,11.2161358284276));
#68364=CARTESIAN_POINT('Ctrl Pts',(87.0586961424002,61.7881237265417,11.2257383531058));
#68365=CARTESIAN_POINT('Ctrl Pts',(87.0555801800205,61.7885978602121,11.2292830569781));
#68366=CARTESIAN_POINT('Ctrl Pts',(87.0490945564464,61.7895879368212,11.2367445442307));
#68367=CARTESIAN_POINT('Ctrl Pts',(87.0457289068002,61.7901035573684,11.2406646666474));
#68368=CARTESIAN_POINT('Ctrl Pts',(87.038963018133,61.7911440990802,11.2486432019622));
#68369=CARTESIAN_POINT('Ctrl Pts',(87.03556402159,61.791668930026,11.2527025851185));
#68370=CARTESIAN_POINT('Ctrl Pts',(87.0231015165286,61.7936015669048,11.2677769386517));
#68371=CARTESIAN_POINT('Ctrl Pts',(87.0141978009505,61.7949988132923,11.278923823769));
#68372=CARTESIAN_POINT('Ctrl Pts',(86.9741931207279,61.8013673011782,11.3307753020688));
#68373=CARTESIAN_POINT('Ctrl Pts',(86.9453803986258,61.8062149785939,11.3731938484325));
#68374=CARTESIAN_POINT('Ctrl Pts',(86.8784122344624,61.8185380260373,11.485894800254));
#68375=CARTESIAN_POINT('Ctrl Pts',(86.8441872383224,61.825949051452,11.5582361458506));
#68376=CARTESIAN_POINT('Ctrl Pts',(86.8054383949488,61.8367836788245,11.6651643772905));
#68377=CARTESIAN_POINT('Ctrl Pts',(86.7951754145612,61.8400401063371,11.6974649176347));
#68378=CARTESIAN_POINT('Ctrl Pts',(86.7827442295446,61.8446159864587,11.7427970119311));
#68379=CARTESIAN_POINT('Ctrl Pts',(86.7794684810918,61.8459000410156,11.7555124866401));
#68380=CARTESIAN_POINT('Ctrl Pts',(86.7744647080963,61.8479977955314,11.776262251709));
#68381=CARTESIAN_POINT('Ctrl Pts',(86.7726164071108,61.8488076090809,11.7842668641605));
#68382=CARTESIAN_POINT('Ctrl Pts',(86.7690484418068,61.8504446302505,11.8004328946085));
#68383=CARTESIAN_POINT('Ctrl Pts',(86.7673312634105,61.8512718735468,11.8085944337633));
#68384=CARTESIAN_POINT('Ctrl Pts',(86.7639520337192,61.8529852793786,11.8254792687191));
#68385=CARTESIAN_POINT('Ctrl Pts',(86.7623008505689,61.8538717398495,11.8342042358313));
#68386=CARTESIAN_POINT('Ctrl Pts',(86.7586393092271,61.8559599218336,11.8547278035169));
#68387=CARTESIAN_POINT('Ctrl Pts',(86.7567040227462,61.8571639310088,11.8665386826224));
#68388=CARTESIAN_POINT('Ctrl Pts',(86.745598878384,61.8647592814387,11.9408824265292));
#68389=CARTESIAN_POINT('Ctrl Pts',(86.7409429218177,61.8712869956939,12.0039849629062));
#68390=CARTESIAN_POINT('Ctrl Pts',(86.7410005280162,61.8779044320784,12.0671580849455));
#68391=CARTESIAN_POINT('Ctrl Pts',(87.1806428354228,61.9866340346925,13.0269406741497));
#68392=CARTESIAN_POINT('Ctrl Pts',(87.1430320818341,61.9817037570677,12.994440896018));
#68393=CARTESIAN_POINT('Ctrl Pts',(87.1073198343453,61.9767734794429,12.959719041223));
#68394=CARTESIAN_POINT('Ctrl Pts',(87.0737708946988,61.9718432018181,12.9230306903352));
#68395=CARTESIAN_POINT('Ctrl Pts',(87.0401932787146,61.9669087099825,12.8863109796621));
#68396=CARTESIAN_POINT('Ctrl Pts',(87.0087830388915,61.9619742181468,12.8476218169232));
#68397=CARTESIAN_POINT('Ctrl Pts',(86.9797666153935,61.9570397263112,12.8072541443209));
#68398=CARTESIAN_POINT('Ctrl Pts',(86.9507389769443,61.9521033272768,12.7668708694692));
#68399=CARTESIAN_POINT('Ctrl Pts',(86.9241072961311,61.9471669282425,12.7248082534978));
#68400=CARTESIAN_POINT('Ctrl Pts',(86.9000542692074,61.9422305292081,12.6813857190687));
#68401=CARTESIAN_POINT('Ctrl Pts',(86.8759531642927,61.937284263135,12.637876390232));
#68402=CARTESIAN_POINT('Ctrl Pts',(86.8544412525289,61.9323379970619,12.5930022062731));
#68403=CARTESIAN_POINT('Ctrl Pts',(86.8356542887356,61.9273917309888,12.5471054551886));
#68404=CARTESIAN_POINT('Ctrl Pts',(86.8186942982478,61.9229264737779,12.5056720191969));
#68405=CARTESIAN_POINT('Ctrl Pts',(86.8039544882604,61.9184612165669,12.4634057728746));
#68406=CARTESIAN_POINT('Ctrl Pts',(86.7914994313964,61.913995959356,12.4205678541202));
#68407=CARTESIAN_POINT('Ctrl Pts',(86.7744754181363,61.9078926875044,12.36201546814));
#68408=CARTESIAN_POINT('Ctrl Pts',(86.761658527776,61.9017894156528,12.3021883648507));
#68409=CARTESIAN_POINT('Ctrl Pts',(86.7532024055706,61.8956861438012,12.2416280485787));
#68410=CARTESIAN_POINT('Ctrl Pts',(86.7451504227884,61.8898745627158,12.1839620626737));
#68411=CARTESIAN_POINT('Ctrl Pts',(86.7410521745367,61.8840629816305,12.1256312882053));
#68412=CARTESIAN_POINT('Ctrl Pts',(86.7410004953938,61.8782514005452,12.0671217397436));
#68413=CARTESIAN_POINT('',(86.7409997144605,62.0467094537538,12.065715168206));
#68414=CARTESIAN_POINT('Ctrl Pts',(87.180642835277,62.1551929346177,13.0269406740237));
#68415=CARTESIAN_POINT('Ctrl Pts',(87.1258041329939,62.1482284515714,12.9795540761038));
#68416=CARTESIAN_POINT('Ctrl Pts',(87.0751143957215,62.1414835135495,12.9275532301801));
#68417=CARTESIAN_POINT('Ctrl Pts',(86.982329632258,62.1277709095857,12.8144534499568));
#68418=CARTESIAN_POINT('Ctrl Pts',(86.940595638107,62.1208256454524,12.7534422569748));
#68419=CARTESIAN_POINT('Ctrl Pts',(86.8965423834688,62.112122338035,12.6752129982176));
#68420=CARTESIAN_POINT('Ctrl Pts',(86.8889524671294,62.1105621404608,12.6611180850041));
#68421=CARTESIAN_POINT('Ctrl Pts',(86.8771878063937,62.1080400149971,12.6382449579432));
#68422=CARTESIAN_POINT('Ctrl Pts',(86.8728436805683,62.1070840610393,12.6295552872296));
#68423=CARTESIAN_POINT('Ctrl Pts',(86.8647194887141,62.1052473721894,12.6128271058738));
#68424=CARTESIAN_POINT('Ctrl Pts',(86.8609232129233,62.1043672614304,12.6047970563204));
#68425=CARTESIAN_POINT('Ctrl Pts',(86.8523328864518,62.1023234980466,12.5861219212143));
#68426=CARTESIAN_POINT('Ctrl Pts',(86.8476008686531,62.1011578049328,12.5754494388245));
#68427=CARTESIAN_POINT('Ctrl Pts',(86.8327056874406,62.0973535821993,12.5405650531874));
#68428=CARTESIAN_POINT('Ctrl Pts',(86.8231469645094,62.094695252629,12.51610485739));
#68429=CARTESIAN_POINT('Ctrl Pts',(86.8017898676855,62.088180254359,12.4560230689288));
#68430=CARTESIAN_POINT('Ctrl Pts',(86.7907994632039,62.0843013155685,12.4201428434782));
#68431=CARTESIAN_POINT('Ctrl Pts',(86.7691936428836,62.0752925712175,12.3365573507273));
#68432=CARTESIAN_POINT('Ctrl Pts',(86.7597109154249,62.0701449566621,12.2886192700193));
#68433=CARTESIAN_POINT('Ctrl Pts',(86.7450013314751,62.0588429392308,12.1824289822729));
#68434=CARTESIAN_POINT('Ctrl Pts',(86.7409870002166,62.0527003764799,12.1241101969471));
#68435=CARTESIAN_POINT('Ctrl Pts',(86.7410000316247,62.04670904774,12.0657165805304));
#68436=CARTESIAN_POINT('Ctrl Pts',(86.7410000319281,62.0467089085791,12.0657152242193));
#68437=CARTESIAN_POINT('Ctrl Pts',(86.7410028199225,62.0454332038684,12.0532817480931));
#68438=CARTESIAN_POINT('Ctrl Pts',(86.7411881963702,62.0441648464695,12.0408480693285));
#68439=CARTESIAN_POINT('Ctrl Pts',(86.7417089181389,62.0423826618144,12.0232590341084));
#68440=CARTESIAN_POINT('Ctrl Pts',(86.7418931107228,62.0418614665008,12.0181006513168));
#68441=CARTESIAN_POINT('Ctrl Pts',(86.7423038126814,62.0408720051917,12.0082783886585));
#68442=CARTESIAN_POINT('Ctrl Pts',(86.7425246029727,62.0404034401319,12.0036143389891));
#68443=CARTESIAN_POINT('Ctrl Pts',(86.7430549289509,62.0393985551119,11.9935831833163));
#68444=CARTESIAN_POINT('Ctrl Pts',(86.7433728278458,62.038862708404,11.9882166152299));
#68445=CARTESIAN_POINT('Ctrl Pts',(86.7442988734846,62.0374576512393,11.9741025623904));
#68446=CARTESIAN_POINT('Ctrl Pts',(86.7449635668555,62.0365914747207,11.9653588119135));
#68447=CARTESIAN_POINT('Ctrl Pts',(86.748336277368,62.0327425734185,11.9263433338939));
#68448=CARTESIAN_POINT('Ctrl Pts',(86.7520401459002,62.0298085641766,11.8961640765638));
#68449=CARTESIAN_POINT('Ctrl Pts',(86.7697652971787,62.0190523885109,11.7849322938948));
#68450=CARTESIAN_POINT('Ctrl Pts',(86.7905646280958,62.0114430278792,11.7051641760554));
#68451=CARTESIAN_POINT('Ctrl Pts',(86.8371075865748,61.9987448109254,11.5785032807828));
#68452=CARTESIAN_POINT('Ctrl Pts',(86.8583395542204,61.9937483060922,11.5302304232081));
#68453=CARTESIAN_POINT('Ctrl Pts',(86.8907031728052,61.9869250408361,11.4675399605217));
#68454=CARTESIAN_POINT('Ctrl Pts',(86.8992351703239,61.9851863929965,11.4518352926345));
#68455=CARTESIAN_POINT('Ctrl Pts',(86.9131052702072,61.9824464676901,11.4275414901062));
#68456=CARTESIAN_POINT('Ctrl Pts',(86.918219725893,61.9814531757426,11.4188266349074));
#68457=CARTESIAN_POINT('Ctrl Pts',(86.927986497966,61.979586842588,11.4026303019402));
#68458=CARTESIAN_POINT('Ctrl Pts',(86.9326137689311,61.978714757115,11.395134343847));
#68459=CARTESIAN_POINT('Ctrl Pts',(86.9431919772588,61.9767474523965,11.3783904030365));
#68460=CARTESIAN_POINT('Ctrl Pts',(86.9491857186099,61.9756507042034,11.3691705061139));
#68461=CARTESIAN_POINT('Ctrl Pts',(86.9649687275369,61.9728071711409,11.3455687236375));
#68462=CARTESIAN_POINT('Ctrl Pts',(86.9749347463562,61.9710539047597,11.3313086632255));
#68463=CARTESIAN_POINT('Ctrl Pts',(87.0257859179714,61.9623060378165,11.2616402153814));
#68464=CARTESIAN_POINT('Ctrl Pts',(87.0708292505141,61.9551563369666,11.2094273892294));
#68465=CARTESIAN_POINT('Ctrl Pts',(87.165921409992,61.9411288684737,11.1157792026558));
#68466=CARTESIAN_POINT('Ctrl Pts',(87.2153673299618,61.9342821610506,11.0740088530863));
#68467=CARTESIAN_POINT('Ctrl Pts',(87.2841847601351,61.9254309942041,11.0243431771584));
#68468=CARTESIAN_POINT('Ctrl Pts',(87.3008722713642,61.9233329925577,11.0128959855754));
#68469=CARTESIAN_POINT('Ctrl Pts',(87.3262006894194,61.9202263791202,10.9963973803056));
#68470=CARTESIAN_POINT('Ctrl Pts',(87.3346384516869,61.919203961748,10.9910418909633));
#68471=CARTESIAN_POINT('Ctrl Pts',(87.3484590123076,61.917550442911,10.9824970875497));
#68472=CARTESIAN_POINT('Ctrl Pts',(87.3538034691465,61.9169160777634,10.979247108508));
#68473=CARTESIAN_POINT('Ctrl Pts',(87.3640622425559,61.9157083111018,10.9731120796999));
#68474=CARTESIAN_POINT('Ctrl Pts',(87.3689723768306,61.9151345235978,10.9702203670039));
#68475=CARTESIAN_POINT('Ctrl Pts',(87.377218578839,61.9141782228872,10.9654384119774));
#68476=CARTESIAN_POINT('Ctrl Pts',(87.3805438429761,61.9137945853355,10.9635301662902));
#68477=CARTESIAN_POINT('Ctrl Pts',(87.389125172068,61.9128096153146,10.9586571843795));
#68478=CARTESIAN_POINT('Ctrl Pts',(87.3943938408958,61.9122097086623,10.9557147830471));
#68479=CARTESIAN_POINT('Ctrl Pts',(87.4097950771983,61.9104694611233,10.9472570807477));
#68480=CARTESIAN_POINT('Ctrl Pts',(87.419982513142,61.9093350726934,10.9418418958677));
#68481=CARTESIAN_POINT('Ctrl Pts',(87.5054489629294,61.8999438497759,10.8978948939304));
#68482=CARTESIAN_POINT('Ctrl Pts',(87.5843454823855,61.8920707804842,10.8668239435082));
#68483=CARTESIAN_POINT('Ctrl Pts',(87.7167709292999,61.8791784072329,10.8294164137846));
#68484=CARTESIAN_POINT('Ctrl Pts',(87.7686292085582,61.8742064696035,10.8182158418731));
#68485=CARTESIAN_POINT('Ctrl Pts',(87.8537009602796,61.8660015737358,10.8053459254994));
#68486=CARTESIAN_POINT('Ctrl Pts',(87.8865468478743,61.8628227863612,10.8016809450371));
#68487=CARTESIAN_POINT('Ctrl Pts',(87.9321571752695,61.8583679425721,10.7983861112518));
#68488=CARTESIAN_POINT('Ctrl Pts',(87.9448315697366,61.8571257400884,10.7976613730748));
#68489=CARTESIAN_POINT('Ctrl Pts',(87.9665515414348,61.8549882740241,10.7967458276447));
#68490=CARTESIAN_POINT('Ctrl Pts',(87.9755924420562,61.8540959772331,10.7964614563854));
#68491=CARTESIAN_POINT('Ctrl Pts',(87.9928799902242,61.8523843514883,10.7961024965952));
#68492=CARTESIAN_POINT('Ctrl Pts',(88.0011258797463,61.8515655764097,10.7960116152273));
#68493=CARTESIAN_POINT('Ctrl Pts',(88.0226900943668,61.8494177547867,10.7959839692702));
#68494=CARTESIAN_POINT('Ctrl Pts',(88.0360071363192,61.8480847650173,10.7961763961106));
#68495=CARTESIAN_POINT('Ctrl Pts',(88.0845728089279,61.8431973241815,10.7976423720828));
#68496=CARTESIAN_POINT('Ctrl Pts',(88.1197632634945,61.8396049491638,10.8001745891025));
#68497=CARTESIAN_POINT('Ctrl Pts',(88.2537733853057,61.8257098836156,10.8154464007892));
#68498=CARTESIAN_POINT('Ctrl Pts',(88.3510675993396,61.8151353341048,10.8383309125452));
#68499=CARTESIAN_POINT('Ctrl Pts',(88.4811154812576,61.8006340727124,10.8855783712691));
#68500=CARTESIAN_POINT('Ctrl Pts',(88.5169430754296,61.796602833171,10.9004845548079));
#68501=CARTESIAN_POINT('Ctrl Pts',(88.5602931877284,61.791718694583,10.9208972642893));
#68502=CARTESIAN_POINT('Ctrl Pts',(88.5685078079727,61.790792912838,10.92487408975));
#68503=CARTESIAN_POINT('Ctrl Pts',(88.5815619275314,61.7893220478666,10.9313684176577));
#68504=CARTESIAN_POINT('Ctrl Pts',(88.5864290588108,61.7887737201429,10.9338290132583));
#68505=CARTESIAN_POINT('Ctrl Pts',(88.5957804158729,61.7877205419562,10.9386325093589));
#68506=CARTESIAN_POINT('Ctrl Pts',(88.6002665871631,61.7872154686659,10.9409708958824));
#68507=CARTESIAN_POINT('Ctrl Pts',(88.6113607303852,61.7859665754378,10.9468382124495));
#68508=CARTESIAN_POINT('Ctrl Pts',(88.6179517588532,61.7852247212754,10.9503989575729));
#68509=CARTESIAN_POINT('Ctrl Pts',(88.6414219955573,61.782581931677,10.9633481353055));
#68510=CARTESIAN_POINT('Ctrl Pts',(88.658119405484,61.7806997288893,10.9730637500738));
#68511=CARTESIAN_POINT('Ctrl Pts',(88.7408430946724,61.7713283041086,11.0237586855808));
#68512=CARTESIAN_POINT('Ctrl Pts',(88.8032399604741,61.764101069542,11.0703608325041));
#68513=CARTESIAN_POINT('Ctrl Pts',(88.9138215166358,61.7501513437213,11.1699704676299));
#68514=CARTESIAN_POINT('Ctrl Pts',(88.9625533990916,61.7434626154976,11.2219033295985));
#68515=CARTESIAN_POINT('Ctrl Pts',(89.0177284563536,61.7348656799369,11.2915875858614));
#68516=CARTESIAN_POINT('Ctrl Pts',(89.0284815860225,61.7331340796478,11.3057711401159));
#68517=CARTESIAN_POINT('Ctrl Pts',(89.044857746256,61.7304027474901,11.3283415699957));
#68518=CARTESIAN_POINT('Ctrl Pts',(89.0506852230236,61.7294109170032,11.3365780224454));
#68519=CARTESIAN_POINT('Ctrl Pts',(89.0614166236631,61.7275458660714,11.3521354835805));
#68520=CARTESIAN_POINT('Ctrl Pts',(89.0663437276059,61.7266735889723,11.3594398555397));
#68521=CARTESIAN_POINT('Ctrl Pts',(89.077260630831,61.7247038974704,11.3759929878436));
#68522=CARTESIAN_POINT('Ctrl Pts',(89.0832067670937,61.7236049377698,11.3852694816493));
#68523=CARTESIAN_POINT('Ctrl Pts',(89.0982676274108,61.7207515670569,11.409452687925));
#68524=CARTESIAN_POINT('Ctrl Pts',(89.107196390347,61.7189905982982,11.4244716197857));
#68525=CARTESIAN_POINT('Ctrl Pts',(89.1500840920726,61.7101698658229,11.5001230674396));
#68526=CARTESIAN_POINT('Ctrl Pts',(89.1793291489598,61.7029520231919,11.5632750179026));
#68527=CARTESIAN_POINT('Ctrl Pts',(89.2253163104422,61.6889189597483,11.6885941927771));
#68528=CARTESIAN_POINT('Ctrl Pts',(89.2427964755464,61.6821374134764,11.750283183016));
#68529=CARTESIAN_POINT('Ctrl Pts',(89.2585445650095,61.6738926551828,11.8277595331751));
#68530=CARTESIAN_POINT('Ctrl Pts',(89.261277187835,61.6723317174103,11.84254314808));
#68531=CARTESIAN_POINT('Ctrl Pts',(89.2666717190363,61.6689422583581,11.8749357346361));
#68532=CARTESIAN_POINT('Ctrl Pts',(89.2692272121659,61.6671177753191,11.8925600536375));
#68533=CARTESIAN_POINT('Ctrl Pts',(89.2722775473009,61.6645946864081,11.9172424140383));
#68534=CARTESIAN_POINT('Ctrl Pts',(89.2730852600916,61.6638810956051,11.9242584199928));
#68535=CARTESIAN_POINT('Ctrl Pts',(89.2743686749144,61.6626640235626,11.9362889545822));
#68536=CARTESIAN_POINT('Ctrl Pts',(89.2748731381651,61.6621590164857,11.9413001224971));
#68537=CARTESIAN_POINT('Ctrl Pts',(89.2758796667905,61.6610917139736,11.9519330042115));
#68538=CARTESIAN_POINT('Ctrl Pts',(89.2763740906652,61.6605298408851,11.95755523881));
#68539=CARTESIAN_POINT('Ctrl Pts',(89.2776412269268,61.6589771708189,11.9731552449886));
#68540=CARTESIAN_POINT('Ctrl Pts',(89.2783335425097,61.6579906404385,11.9831395068201));
#68541=CARTESIAN_POINT('Ctrl Pts',(89.2824745699471,61.6509158291123,12.0551931314855));
#68542=CARTESIAN_POINT('Ctrl Pts',(89.2814805335318,61.6450405748864,12.1174457634074));
#68543=CARTESIAN_POINT('Ctrl Pts',(89.2716212554652,61.6346702014124,12.2274351010088));
#68544=CARTESIAN_POINT('Ctrl Pts',(89.2645800550495,61.6301700405048,12.2751990635647));
#68545=CARTESIAN_POINT('Ctrl Pts',(89.2470499440718,61.6220003956576,12.3602251447053));
#68546=CARTESIAN_POINT('Ctrl Pts',(89.2375445688236,61.6183499769934,12.3976260666504));
#68547=CARTESIAN_POINT('Ctrl Pts',(89.2185832334045,61.6120873521357,12.4601568841308));
#68548=CARTESIAN_POINT('Ctrl Pts',(89.2100057992326,61.6095008227215,12.4855256500594));
#68549=CARTESIAN_POINT('Ctrl Pts',(89.1965169643472,61.6057409156812,12.5216180642673));
#68550=CARTESIAN_POINT('Ctrl Pts',(89.1922474505703,61.6045886059016,12.5325755363549));
#68551=CARTESIAN_POINT('Ctrl Pts',(89.1844827770048,61.6025558291926,12.5517131609034));
#68552=CARTESIAN_POINT('Ctrl Pts',(89.1810526124823,61.6016775914689,12.5599189979002));
#68553=CARTESIAN_POINT('Ctrl Pts',(89.1737112431256,61.5998376918088,12.5769757262692));
#68554=CARTESIAN_POINT('Ctrl Pts',(89.1697845196326,61.5988755521522,12.5858192488831));
#68555=CARTESIAN_POINT('Ctrl Pts',(89.159171125065,61.5963307390361,12.6090040892284));
#68556=CARTESIAN_POINT('Ctrl Pts',(89.1523170710355,61.5947424334543,12.6232662366914));
#68557=CARTESIAN_POINT('Ctrl Pts',(89.113485644348,61.5860278813024,12.7003451288164));
#68558=CARTESIAN_POINT('Ctrl Pts',(89.0765944984042,61.5787330923175,12.7605303808079));
#68559=CARTESIAN_POINT('Ctrl Pts',(89.0002316581315,61.5651840946521,12.8645970484931));
#68560=CARTESIAN_POINT('Ctrl Pts',(88.962320720361,61.5589790397651,12.9094010456045));
#68561=CARTESIAN_POINT('Ctrl Pts',(88.9029671412863,61.5500548139998,12.9704321438013));
#68562=CARTESIAN_POINT('Ctrl Pts',(88.8838911541433,61.5472906586879,12.9888565190327));
#68563=CARTESIAN_POINT('Ctrl Pts',(88.8514308595378,61.5427697947982,13.0183001329849));
#68564=CARTESIAN_POINT('Ctrl Pts',(88.8383734114396,61.5409970255744,13.0296663922288));
#68565=CARTESIAN_POINT('Ctrl Pts',(88.8197245374676,61.5385325667359,13.0452412509537));
#68566=CARTESIAN_POINT('Ctrl Pts',(88.8143254366397,61.5378267658218,13.0496752798563));
#68567=CARTESIAN_POINT('Ctrl Pts',(88.8049803162172,61.5366186233422,13.0572217250383));
#68568=CARTESIAN_POINT('Ctrl Pts',(88.801052008383,61.5361148157008,13.0603556101724));
#68569=CARTESIAN_POINT('Ctrl Pts',(88.7926434254985,61.5350450903718,13.066982429417));
#68570=CARTESIAN_POINT('Ctrl Pts',(88.7881581847139,61.5344796296872,13.070468729832));
#68571=CARTESIAN_POINT('Ctrl Pts',(88.7757814636557,61.5329328266663,13.0799564083644));
#68572=CARTESIAN_POINT('Ctrl Pts',(88.7678425853573,61.5319556028821,13.0858958812332));
#68573=CARTESIAN_POINT('Ctrl Pts',(88.7091107381839,61.5248276813325,13.1287725789126));
#68574=CARTESIAN_POINT('Ctrl Pts',(88.6556994824167,61.5188945516076,13.1619972134143));
#68575=CARTESIAN_POINT('Ctrl Pts',(88.5555188933138,61.5082772582139,13.2144443250592));
#68576=CARTESIAN_POINT('Ctrl Pts',(88.509656082103,61.5035906647227,13.2350882015239));
#68577=CARTESIAN_POINT('Ctrl Pts',(88.428111734402,61.4953729266357,13.2661194542478));
#68578=CARTESIAN_POINT('Ctrl Pts',(88.3929767189535,61.4918675952603,13.277759983306));
#68579=CARTESIAN_POINT('Ctrl Pts',(88.3454882189434,61.487133560578,13.2912226637341));
#68580=CARTESIAN_POINT('Ctrl Pts',(88.3335418484475,61.4859430321718,13.2944216205689));
#68581=CARTESIAN_POINT('Ctrl Pts',(88.3039349389782,61.4829910387025,13.3018880154039));
#68582=CARTESIAN_POINT('Ctrl Pts',(88.2862265835771,61.4812240870242,13.3059517383963));
#68583=CARTESIAN_POINT('Ctrl Pts',(88.2584834508096,61.4784496629028,13.311694699743));
#68584=CARTESIAN_POINT('Ctrl Pts',(88.2485046867726,61.47745051783,13.3136357049626));
#68585=CARTESIAN_POINT('Ctrl Pts',(88.2298431210603,61.4755789713147,13.3170336474334));
#68586=CARTESIAN_POINT('Ctrl Pts',(88.2211663106254,61.4747075748821,13.3185205030736));
#68587=CARTESIAN_POINT('Ctrl Pts',(88.2017003306559,61.4727494437517,13.3216482289899));
#68588=CARTESIAN_POINT('Ctrl Pts',(88.1909042198743,61.4716612433343,13.3232404478233));
#68589=CARTESIAN_POINT('Ctrl Pts',(88.1631342445674,61.4688556244314,13.326970989135));
#68590=CARTESIAN_POINT('Ctrl Pts',(88.1461359403385,61.4671320144544,13.3289057242592));
#68591=CARTESIAN_POINT('Ctrl Pts',(88.0401074397547,61.4563357863369,13.338808854493));
#68592=CARTESIAN_POINT('Ctrl Pts',(87.9505025925264,61.4469875989152,13.3377005012535));
#68593=CARTESIAN_POINT('Ctrl Pts',(87.8126183112931,61.4323493303676,13.321386512206));
#68594=CARTESIAN_POINT('Ctrl Pts',(87.7638367075291,61.4271262506289,13.312700261283));
#68595=CARTESIAN_POINT('Ctrl Pts',(87.6986031353953,61.4201512268202,13.2971038252658));
#68596=CARTESIAN_POINT('Ctrl Pts',(87.6816076574998,61.4183351472497,13.2926658891446));
#68597=CARTESIAN_POINT('Ctrl Pts',(87.6523615453121,61.4152172273181,13.2843772615347));
#68598=CARTESIAN_POINT('Ctrl Pts',(87.6400674484234,61.4139088047979,13.2806908168292));
#68599=CARTESIAN_POINT('Ctrl Pts',(87.6219037560744,61.4119809465445,13.2749428262475));
#68600=CARTESIAN_POINT('Ctrl Pts',(87.6159906173178,61.4113541719552,13.2730237105095));
#68601=CARTESIAN_POINT('Ctrl Pts',(87.6053849337812,61.4102317765184,13.2694953354569));
#68602=CARTESIAN_POINT('Ctrl Pts',(87.6006875091621,61.4097353047805,13.2679019375483));
#68603=CARTESIAN_POINT('Ctrl Pts',(87.5901133215982,61.4086191465328,13.2642458801508));
#68604=CARTESIAN_POINT('Ctrl Pts',(87.5842422398027,61.4080003866912,13.2621674654846));
#68605=CARTESIAN_POINT('Ctrl Pts',(87.5662647073072,61.4061079374555,13.2556540439802));
#68606=CARTESIAN_POINT('Ctrl Pts',(87.5542096783003,61.4048420457589,13.2510775814095));
#68607=CARTESIAN_POINT('Ctrl Pts',(87.4860058371124,61.397685632907,13.2239897836112));
#68608=CARTESIAN_POINT('Ctrl Pts',(87.4314427977759,61.3919806488829,13.1976692407666));
#68609=CARTESIAN_POINT('Ctrl Pts',(87.3149673821541,61.3793791376846,13.1308385449483));
#68610=CARTESIAN_POINT('Ctrl Pts',(87.2543042240963,61.3725153337452,13.0886206264755));
#68611=CARTESIAN_POINT('Ctrl Pts',(87.191938763816,61.3647774823412,13.0366152717074));
#68612=CARTESIAN_POINT('Ctrl Pts',(87.1862692440195,61.3640674112978,13.0318025026143));
#68613=CARTESIAN_POINT('Ctrl Pts',(87.1806428320421,61.3633558149692,13.0269406712284));
#68614=CARTESIAN_POINT('Origin',(88.011,66.41344859951,12.066));
#68615=CARTESIAN_POINT('',(87.1806428354305,60.4003450897931,13.0269406741564));
#68616=CARTESIAN_POINT('',(87.180642808438,60.5693987930815,13.0269406508319));
#68617=CARTESIAN_POINT('',(87.1806428354228,66.41344859951,13.0269406741497));
#68618=CARTESIAN_POINT('Ctrl Pts',(87.1806428354305,60.4003450897931,13.0269406741563));
#68619=CARTESIAN_POINT('Ctrl Pts',(87.1818235457003,60.4005030384075,13.0279609361332));
#68620=CARTESIAN_POINT('Ctrl Pts',(87.183006150907,60.4006608448018,13.0289790345607));
#68621=CARTESIAN_POINT('Ctrl Pts',(87.1883032417142,60.4013659091017,13.0335222992003));
#68622=CARTESIAN_POINT('Ctrl Pts',(87.1924385094708,60.4019115463032,13.0370234012454));
#68623=CARTESIAN_POINT('Ctrl Pts',(87.2001912229078,60.4029254359064,13.0435024694305));
#68624=CARTESIAN_POINT('Ctrl Pts',(87.2038028005578,60.4033941165757,13.046486937284));
#68625=CARTESIAN_POINT('Ctrl Pts',(87.2123614349539,60.4044963384234,13.053480116595));
#68626=CARTESIAN_POINT('Ctrl Pts',(87.2173222500813,60.4051286646051,13.0574717211992));
#68627=CARTESIAN_POINT('Ctrl Pts',(87.2329986405361,60.4071071941662,13.0698922970969));
#68628=CARTESIAN_POINT('Ctrl Pts',(87.2438206326235,60.4084445437355,13.0781866096631));
#68629=CARTESIAN_POINT('Ctrl Pts',(87.3215569159369,60.4178691040628,13.1358028049835));
#68630=CARTESIAN_POINT('Ctrl Pts',(87.3930503351943,60.4256038617588,13.1786334918077));
#68631=CARTESIAN_POINT('Ctrl Pts',(87.515181244556,60.4382618428318,13.2363677913222));
#68632=CARTESIAN_POINT('Ctrl Pts',(87.5634452938574,60.4431359090961,13.2556600366186));
#68633=CARTESIAN_POINT('Ctrl Pts',(87.6338056398892,60.4502041844216,13.2788957251422));
#68634=CARTESIAN_POINT('Ctrl Pts',(87.6550369818825,60.4523320140989,13.285295629218));
#68635=CARTESIAN_POINT('Ctrl Pts',(87.6936033195649,60.4561987754467,13.2958278334117));
#68636=CARTESIAN_POINT('Ctrl Pts',(87.7108787134513,60.4579313985905,13.3001573202425));
#68637=CARTESIAN_POINT('Ctrl Pts',(87.7380781588305,60.4606641076622,13.3063691139301));
#68638=CARTESIAN_POINT('Ctrl Pts',(87.7479439690297,60.461656280952,13.3084988451494));
#68639=CARTESIAN_POINT('Ctrl Pts',(87.7664694706385,60.4635218446625,13.3122674198115));
#68640=CARTESIAN_POINT('Ctrl Pts',(87.7751229431287,60.4643942901964,13.3139341591509));
#68641=CARTESIAN_POINT('Ctrl Pts',(87.7946340537761,60.46636419222,13.3174820001018));
#68642=CARTESIAN_POINT('Ctrl Pts',(87.8055000673036,60.4674631932169,13.3193120829443));
#68643=CARTESIAN_POINT('Ctrl Pts',(87.8336509584641,60.4703163338593,13.3236774190162));
#68644=CARTESIAN_POINT('Ctrl Pts',(87.850966083578,60.4720770275225,13.325997714557));
#68645=CARTESIAN_POINT('Ctrl Pts',(87.9374121288136,60.4809011960646,13.3357713264499));
#68646=CARTESIAN_POINT('Ctrl Pts',(88.0070116415135,60.4881229405543,13.3378941071811));
#68647=CARTESIAN_POINT('Ctrl Pts',(88.14033476812,60.502157152959,13.3310171185709));
#68648=CARTESIAN_POINT('Ctrl Pts',(88.2039085896951,60.5089358068787,13.3228939852102));
#68649=CARTESIAN_POINT('Ctrl Pts',(88.2813220326698,60.517177406491,13.3069882621684));
#68650=CARTESIAN_POINT('Ctrl Pts',(88.2959893885601,60.5187380173635,13.3037022929366));
#68651=CARTESIAN_POINT('Ctrl Pts',(88.3278965393121,60.5221269677771,13.2959567227708));
#68652=CARTESIAN_POINT('Ctrl Pts',(88.3451086933597,60.5239512677949,13.2913931819824));
#68653=CARTESIAN_POINT('Ctrl Pts',(88.3690077503675,60.5264742388476,13.2845156256566));
#68654=CARTESIAN_POINT('Ctrl Pts',(88.375778714417,60.5271878908095,13.2825058065376));
#68655=CARTESIAN_POINT('Ctrl Pts',(88.3873496830548,60.5284051169061,13.2789659061668));
#68656=CARTESIAN_POINT('Ctrl Pts',(88.3921578798775,60.5289102168012,13.2774635978164));
#68657=CARTESIAN_POINT('Ctrl Pts',(88.4023357079058,60.529977786217,13.2742169650245));
#68658=CARTESIAN_POINT('Ctrl Pts',(88.4077028162123,60.5305398327136,13.2724653957062));
#68659=CARTESIAN_POINT('Ctrl Pts',(88.4225554360673,60.5320931508309,13.2675083712489));
#68660=CARTESIAN_POINT('Ctrl Pts',(88.4320153458227,60.5330801511957,13.2642263328636));
#68661=CARTESIAN_POINT('Ctrl Pts',(88.5000220765551,60.5401659294441,13.2397270471169));
#68662=CARTESIAN_POINT('Ctrl Pts',(88.5569886562945,60.5460509438944,13.2143367338943));
#68663=CARTESIAN_POINT('Ctrl Pts',(88.6545537301216,60.5564504935943,13.1619405892929));
#68664=CARTESIAN_POINT('Ctrl Pts',(88.6958888513917,60.5609697956643,13.1365953465336));
#68665=CARTESIAN_POINT('Ctrl Pts',(88.7671948193609,60.5691416584645,13.087049738998));
#68666=CARTESIAN_POINT('Ctrl Pts',(88.7977030773002,60.5727744517393,13.0637329175712));
#68667=CARTESIAN_POINT('Ctrl Pts',(88.8475515616372,60.579010451814,13.0219254676001));
#68668=CARTESIAN_POINT('Ctrl Pts',(88.8674492276917,60.5815882885321,13.0041399150839));
#68669=CARTESIAN_POINT('Ctrl Pts',(88.8952771946967,60.5853380351467,12.9776423735909));
#68670=CARTESIAN_POINT('Ctrl Pts',(88.9036707639428,60.5864890432026,12.9694250710635));
#68671=CARTESIAN_POINT('Ctrl Pts',(88.91821700976,60.5885204883688,12.9547836595667));
#68672=CARTESIAN_POINT('Ctrl Pts',(88.9244185530755,60.5893987076884,12.9484089942142));
#68673=CARTESIAN_POINT('Ctrl Pts',(88.9372328688173,60.5912395269298,12.9349571222238));
#68674=CARTESIAN_POINT('Ctrl Pts',(88.9438326139202,60.5922026113499,12.9278683824296));
#68675=CARTESIAN_POINT('Ctrl Pts',(88.9610248223903,60.5947521932668,12.9089735519185));
#68676=CARTESIAN_POINT('Ctrl Pts',(88.9714778832212,60.5963443595617,12.8970437712062));
#68677=CARTESIAN_POINT('Ctrl Pts',(89.0289240580398,60.6053401616578,12.8289503018001));
#68678=CARTESIAN_POINT('Ctrl Pts',(89.0712031951646,60.6129267965022,12.7690128165869));
#68679=CARTESIAN_POINT('Ctrl Pts',(89.141358493305,60.6275566034683,12.6487128009007));
#68680=CARTESIAN_POINT('Ctrl Pts',(89.1701360753813,60.6345569155692,12.5891332674651));
#68681=CARTESIAN_POINT('Ctrl Pts',(89.1997068907329,60.6430441963511,12.5133363729505));
#68682=CARTESIAN_POINT('Ctrl Pts',(89.2050079721939,60.6446328049968,12.4989883560411));
#68683=CARTESIAN_POINT('Ctrl Pts',(89.2159880026012,60.6480724241271,12.4675329091262));
#68684=CARTESIAN_POINT('Ctrl Pts',(89.2215648760738,60.6499194150829,12.4503924570919));
#68685=CARTESIAN_POINT('Ctrl Pts',(89.2288265944031,60.6524680472548,12.4263452907856));
#68686=CARTESIAN_POINT('Ctrl Pts',(89.2308208555399,60.6531850601008,12.41953561584));
#68687=CARTESIAN_POINT('Ctrl Pts',(89.2341345518813,60.6544061558909,12.4078585851044));
#68688=CARTESIAN_POINT('Ctrl Pts',(89.2354822311421,60.65491179038,12.4029995469194));
#68689=CARTESIAN_POINT('Ctrl Pts',(89.2382734172852,60.6559783944958,12.3926981142844));
#68690=CARTESIAN_POINT('Ctrl Pts',(89.2397097240939,60.6565389556276,12.3872539760174));
#68691=CARTESIAN_POINT('Ctrl Pts',(89.2435816974858,60.6580837784724,12.372171808707));
#68692=CARTESIAN_POINT('Ctrl Pts',(89.2459405754572,60.6590638446109,12.3625141060716));
#68693=CARTESIAN_POINT('Ctrl Pts',(89.2612211512837,60.665697018692,12.2966040914199));
#68694=CARTESIAN_POINT('Ctrl Pts',(89.270410985598,60.6711671553571,12.2395445707144));
#68695=CARTESIAN_POINT('Ctrl Pts',(89.2824480332011,60.6835540456412,12.1083646942831));
#68696=CARTESIAN_POINT('Ctrl Pts',(89.282756795416,60.6904252659034,12.0342351866708));
#68697=CARTESIAN_POINT('Ctrl Pts',(89.274989777182,60.6993003612147,11.9410578186938));
#68698=CARTESIAN_POINT('Ctrl Pts',(89.2729211592636,60.7011610843257,11.9216545174111));
#68699=CARTESIAN_POINT('Ctrl Pts',(89.2688559280903,60.7041878769031,11.890377711165));
#68700=CARTESIAN_POINT('Ctrl Pts',(89.2671359706872,60.7053465992457,11.8784709982653));
#68701=CARTESIAN_POINT('Ctrl Pts',(89.2624525692833,60.7082315952085,11.8490132446152));
#68702=CARTESIAN_POINT('Ctrl Pts',(89.2592889111503,60.7099632312611,11.8314973246124));
#68703=CARTESIAN_POINT('Ctrl Pts',(89.2537565683444,60.7126947366908,11.804164290217));
#68704=CARTESIAN_POINT('Ctrl Pts',(89.2516369724662,60.7136867051908,11.7942984816242));
#68705=CARTESIAN_POINT('Ctrl Pts',(89.2474464429995,60.7155520897741,11.7758657909649));
#68706=CARTESIAN_POINT('Ctrl Pts',(89.2454034378665,60.7164245627095,11.7672931063713));
#68707=CARTESIAN_POINT('Ctrl Pts',(89.2406048145838,60.7183948018869,11.7480479803434));
#68708=CARTESIAN_POINT('Ctrl Pts',(89.237799180225,60.7194941149436,11.7373889250765));
#68709=CARTESIAN_POINT('Ctrl Pts',(89.230186224627,60.7223486445919,11.7099234726828));
#68710=CARTESIAN_POINT('Ctrl Pts',(89.2251702066942,60.7241104259952,11.6931780922213));
#68711=CARTESIAN_POINT('Ctrl Pts',(89.1985235430636,60.7329242255433,11.6104713120563));
#68712=CARTESIAN_POINT('Ctrl Pts',(89.1718600995691,60.7401339181801,11.5462707161571));
#68713=CARTESIAN_POINT('Ctrl Pts',(89.1107606974387,60.7541635742319,11.4276179459689));
#68714=CARTESIAN_POINT('Ctrl Pts',(89.0771587470441,60.7609501413926,11.3729551363371));
#68715=CARTESIAN_POINT('Ctrl Pts',(89.0307531605401,60.7692005270281,11.3088806905279));
#68716=CARTESIAN_POINT('Ctrl Pts',(89.0217159320494,60.7707621534588,11.296857938134));
#68717=CARTESIAN_POINT('Ctrl Pts',(89.0015135749182,60.774152945064,11.2709527705344));
#68718=CARTESIAN_POINT('Ctrl Pts',(88.9902651036156,60.7759780713757,11.2571383251341));
#68719=CARTESIAN_POINT('Ctrl Pts',(88.9741543530414,60.7785019775746,11.2381814278303));
#68720=CARTESIAN_POINT('Ctrl Pts',(88.9695349496019,60.7792157525372,11.2328369576447));
#68721=CARTESIAN_POINT('Ctrl Pts',(88.9615452521861,60.7804331200762,11.2237476038366));
#68722=CARTESIAN_POINT('Ctrl Pts',(88.9581969108303,60.7809382393567,11.2199838109235));
#68723=CARTESIAN_POINT('Ctrl Pts',(88.9510490725428,60.7820057726023,11.212044728525));
#68724=CARTESIAN_POINT('Ctrl Pts',(88.947244018508,60.7825677640794,11.2078747137815));
#68725=CARTESIAN_POINT('Ctrl Pts',(88.9366151718135,60.7841207672902,11.1963812652628));
#68726=CARTESIAN_POINT('Ctrl Pts',(88.9297321621756,60.7851075105839,11.1891126484477));
#68727=CARTESIAN_POINT('Ctrl Pts',(88.8794707434954,60.7921851921374,11.1372770370207));
#68728=CARTESIAN_POINT('Ctrl Pts',(88.8329477885672,60.798062921411,11.0958594470615));
#68729=CARTESIAN_POINT('Ctrl Pts',(88.7452332758582,60.8084411299462,11.0286311007822));
#68730=CARTESIAN_POINT('Ctrl Pts',(88.7052547864094,60.8129465739439,11.0014611384871));
#68731=CARTESIAN_POINT('Ctrl Pts',(88.6307849874536,60.821116789458,10.9568334812509));
#68732=CARTESIAN_POINT('Ctrl Pts',(88.5968628543753,60.8247623030063,10.9385479870025));
#68733=CARTESIAN_POINT('Ctrl Pts',(88.5380648875935,60.8310175850487,10.9102239866045));
#68734=CARTESIAN_POINT('Ctrl Pts',(88.5136062182713,60.8336017636904,10.8993799497752));
#68735=CARTESIAN_POINT('Ctrl Pts',(88.4779320745104,60.8373590267209,10.8848934552966));
#68736=CARTESIAN_POINT('Ctrl Pts',(88.4669783100613,60.8385110891188,10.8806215835111));
#68737=CARTESIAN_POINT('Ctrl Pts',(88.4476359648191,60.8405437364103,10.8733859980256));
#68738=CARTESIAN_POINT('Ctrl Pts',(88.4392724302413,60.8414220950631,10.8703571441139));
#68739=CARTESIAN_POINT('Ctrl Pts',(88.42174188407,60.8432625561468,10.864215985656));
#68740=CARTESIAN_POINT('Ctrl Pts',(88.412569770061,60.8442251386009,10.8611201641078));
#68741=CARTESIAN_POINT('Ctrl Pts',(88.3883005701939,60.8467718616328,10.8532365800518));
#68742=CARTESIAN_POINT('Ctrl Pts',(88.373148354498,60.8483616478028,10.8486260459293));
#68743=CARTESIAN_POINT('Ctrl Pts',(88.2851879697798,60.8575943736303,10.8236487498949));
#68744=CARTESIAN_POINT('Ctrl Pts',(88.2107801797756,60.865433453224,10.8095373426119));
#68745=CARTESIAN_POINT('Ctrl Pts',(88.0716513455794,60.8801291206798,10.7958238113302));
#68746=CARTESIAN_POINT('Ctrl Pts',(88.0073392444037,60.8869331618185,10.7943816821399));
#68747=CARTESIAN_POINT('Ctrl Pts',(87.9281544325711,60.8952029446871,10.7986155252594));
#68748=CARTESIAN_POINT('Ctrl Pts',(87.9131308565589,60.8967668094308,10.7996870547881));
#68749=CARTESIAN_POINT('Ctrl Pts',(87.880370959071,60.9001616581843,10.8026101488551));
#68750=CARTESIAN_POINT('Ctrl Pts',(87.8626465375777,60.9019886048038,10.8045685806001));
#68751=CARTESIAN_POINT('Ctrl Pts',(87.8379619933267,60.9045145709251,10.8078236285326));
#68752=CARTESIAN_POINT('Ctrl Pts',(87.8309638087539,60.9052286166913,10.8088059370702));
#68753=CARTESIAN_POINT('Ctrl Pts',(87.8189910262652,60.9064462956846,10.8105885402172));
#68754=CARTESIAN_POINT('Ctrl Pts',(87.8140124437935,60.9069514576935,10.8113600967529));
#68755=CARTESIAN_POINT('Ctrl Pts',(87.8034664913107,60.9080189115332,10.8130587830223));
#68756=CARTESIAN_POINT('Ctrl Pts',(87.797900534944,60.9085807820554,10.8139934213466));
#68757=CARTESIAN_POINT('Ctrl Pts',(87.7824865048628,60.9101330930373,10.8166875266389));
#68758=CARTESIAN_POINT('Ctrl Pts',(87.7726523430076,60.9111192712444,10.8185263566091));
#68759=CARTESIAN_POINT('Ctrl Pts',(87.7020269615263,60.9181785548535,10.8325978982789));
#68760=CARTESIAN_POINT('Ctrl Pts',(87.6421700351697,60.9240397109677,10.8491546507382));
#68761=CARTESIAN_POINT('Ctrl Pts',(87.5386139137096,60.9343668730824,10.8861487892692));
#68762=CARTESIAN_POINT('Ctrl Pts',(87.4944249805767,60.938838327223,10.904816245598));
#68763=CARTESIAN_POINT('Ctrl Pts',(87.4165215302357,60.9470037629158,10.9430553396457));
#68764=CARTESIAN_POINT('Ctrl Pts',(87.3824528756208,60.9506796972496,10.9617638866863));
#68765=CARTESIAN_POINT('Ctrl Pts',(87.3263289178861,60.9569810451816,10.9960235266602));
#68766=CARTESIAN_POINT('Ctrl Pts',(87.3038136527362,60.9595803392451,11.0107695162515));
#68767=CARTESIAN_POINT('Ctrl Pts',(87.2721381929844,60.9633555102512,11.0329839906344));
#68768=CARTESIAN_POINT('Ctrl Pts',(87.2625859596756,60.9645100774377,11.0398834145438));
#68769=CARTESIAN_POINT('Ctrl Pts',(87.2459908340444,60.9665455835743,11.0522247958457));
#68770=CARTESIAN_POINT('Ctrl Pts',(87.2389064224069,60.9674242761944,11.0576098543521));
#68771=CARTESIAN_POINT('Ctrl Pts',(87.224243725225,60.969263901424,11.0690004748285));
#68772=CARTESIAN_POINT('Ctrl Pts',(87.21667630813,60.9702253034973,11.0750189969647));
#68773=CARTESIAN_POINT('Ctrl Pts',(87.1969391023736,60.9727653039277,11.0910877200085));
#68774=CARTESIAN_POINT('Ctrl Pts',(87.1848871442495,60.9743494934518,11.1012790089521));
#68775=CARTESIAN_POINT('Ctrl Pts',(87.1208285702406,60.982956709329,11.15752836861));
#68776=CARTESIAN_POINT('Ctrl Pts',(87.0724891052819,60.9901431269842,11.2075600840623));
#68777=CARTESIAN_POINT('Ctrl Pts',(86.984660276668,61.0046878356518,11.3147933334829));
#68778=CARTESIAN_POINT('Ctrl Pts',(86.9452760834755,61.0120213220525,11.3717973221253));
#68779=CARTESIAN_POINT('Ctrl Pts',(86.9029004350045,61.0208762787525,11.4453059659719));
#68780=CARTESIAN_POINT('Ctrl Pts',(86.8953231713088,61.0225052556663,11.4590313036091));
#68781=CARTESIAN_POINT('Ctrl Pts',(86.8838468872093,61.0250431114313,11.4807607286703));
#68782=CARTESIAN_POINT('Ctrl Pts',(86.8797747993739,61.0259586279153,11.4886710619168));
#68783=CARTESIAN_POINT('Ctrl Pts',(86.8703168278749,61.0281204190384,11.5075282296498));
#68784=CARTESIAN_POINT('Ctrl Pts',(86.8650046735154,61.029363248991,11.5185115811269));
#68785=CARTESIAN_POINT('Ctrl Pts',(86.8572770465514,61.0312137873292,11.5350946509773));
#68786=CARTESIAN_POINT('Ctrl Pts',(86.8547425174462,61.031828035699,11.5406374750529));
#68787=CARTESIAN_POINT('Ctrl Pts',(86.8504196176335,61.0328883104789,11.5502741722144));
#68788=CARTESIAN_POINT('Ctrl Pts',(86.8486128588339,61.0333354059779,11.5543594134715));
#68789=CARTESIAN_POINT('Ctrl Pts',(86.844390175985,61.0343898403386,11.5640451056216));
#68790=CARTESIAN_POINT('Ctrl Pts',(86.8419929803356,61.0349960489823,11.5696535573522));
#68791=CARTESIAN_POINT('Ctrl Pts',(86.8350613103306,61.0367723789586,11.5861996434745));
#68792=CARTESIAN_POINT('Ctrl Pts',(86.8306390634038,61.0379361722533,11.5971841723812));
#68793=CARTESIAN_POINT('Ctrl Pts',(86.7969364963393,61.0470682195402,11.6844004936831));
#68794=CARTESIAN_POINT('Ctrl Pts',(86.7749112460985,61.0546819141872,11.7632486704293));
#68795=CARTESIAN_POINT('Ctrl Pts',(86.747586714649,61.0693042938117,11.916929712529));
#68796=CARTESIAN_POINT('Ctrl Pts',(86.7410263188956,61.0762791249421,11.9911708868403));
#68797=CARTESIAN_POINT('Ctrl Pts',(86.7409937160777,61.0851952413026,12.0835881886303));
#68798=CARTESIAN_POINT('Ctrl Pts',(86.7413715720823,61.0869454454075,12.1016213816465));
#68799=CARTESIAN_POINT('Ctrl Pts',(86.7426055350587,61.0897997207293,12.1308114111767));
#68800=CARTESIAN_POINT('Ctrl Pts',(86.7432253267581,61.0908964873843,12.1419762859805));
#68801=CARTESIAN_POINT('Ctrl Pts',(86.7445980041939,61.0928672786699,12.1619369299044));
#68802=CARTESIAN_POINT('Ctrl Pts',(86.7452953406335,61.0937395163781,12.1707359290083));
#68803=CARTESIAN_POINT('Ctrl Pts',(86.7469769078808,61.0956047155684,12.1894719742893));
#68804=CARTESIAN_POINT('Ctrl Pts',(86.7479867296546,61.0965984206984,12.1994060349801));
#68805=CARTESIAN_POINT('Ctrl Pts',(86.751064811346,61.0993230420021,12.2265062679242));
#68806=CARTESIAN_POINT('Ctrl Pts',(86.7533665709165,61.1010611189094,12.2436429677218));
#68807=CARTESIAN_POINT('Ctrl Pts',(86.7690739057215,61.1114251476751,12.3448744677802));
#68808=CARTESIAN_POINT('Ctrl Pts',(86.7905573747488,61.1203012032526,12.427475203825));
#68809=CARTESIAN_POINT('Ctrl Pts',(86.8460860157505,61.1371390301722,12.5773262869857));
#68810=CARTESIAN_POINT('Ctrl Pts',(86.8781710899104,61.1450429541316,12.6449476925472));
#68811=CARTESIAN_POINT('Ctrl Pts',(86.9223877843024,61.1539922390763,12.7202029611383));
#68812=CARTESIAN_POINT('Ctrl Pts',(86.9289179388271,61.1552736962705,12.7309485142304));
#68813=CARTESIAN_POINT('Ctrl Pts',(86.9388877847896,61.1571698641732,12.7468182080522));
#68814=CARTESIAN_POINT('Ctrl Pts',(86.9422066463362,61.1577915801697,12.7520166232814));
#68815=CARTESIAN_POINT('Ctrl Pts',(86.9482638459595,61.1589090498527,12.7613534979219));
#68816=CARTESIAN_POINT('Ctrl Pts',(86.9509886757856,61.159405613115,12.7655002614634));
#68817=CARTESIAN_POINT('Ctrl Pts',(86.9572181881596,61.1605271525424,12.7748606009751));
#68818=CARTESIAN_POINT('Ctrl Pts',(86.9607373373136,61.161151159148,12.7800642857004));
#68819=CARTESIAN_POINT('Ctrl Pts',(86.9717556774926,61.1630763550506,12.7960991574369));
#68820=CARTESIAN_POINT('Ctrl Pts',(86.9793852818383,61.1643693537997,12.8068405123835));
#68821=CARTESIAN_POINT('Ctrl Pts',(86.997942895831,61.1674263987363,12.8321240730532));
#68822=CARTESIAN_POINT('Ctrl Pts',(87.0090191575784,61.1691821336079,12.8465544737062));
#68823=CARTESIAN_POINT('Ctrl Pts',(87.0533894015635,61.1759776120283,12.9018592103304));
#68824=CARTESIAN_POINT('Ctrl Pts',(87.088907793503,61.1809202758021,12.9408861691967));
#68825=CARTESIAN_POINT('Ctrl Pts',(87.1442488648199,61.188144009566,12.9945669604313));
#68826=CARTESIAN_POINT('Ctrl Pts',(87.1622201789556,61.1904240998232,13.0110215023542));
#68827=CARTESIAN_POINT('Ctrl Pts',(87.1806429942554,61.1927093932679,13.0269408113983));
#68828=CARTESIAN_POINT('Ctrl Pts',(87.1806428320421,61.3633558149692,13.0269406712284));
#68829=CARTESIAN_POINT('Ctrl Pts',(87.1604885363056,61.3608068151966,13.0095251694904));
#68830=CARTESIAN_POINT('Ctrl Pts',(87.1408873812754,61.3582380582144,12.9914801488475));
#68831=CARTESIAN_POINT('Ctrl Pts',(87.1127044862172,61.3543939148636,12.9638473539881));
#68832=CARTESIAN_POINT('Ctrl Pts',(87.103677906826,61.3531383888453,12.9547245305709));
#68833=CARTESIAN_POINT('Ctrl Pts',(87.0885102340277,61.3509851290083,12.9389231959377));
#68834=CARTESIAN_POINT('Ctrl Pts',(87.0822994499866,61.350090474729,12.9323126179523));
#68835=CARTESIAN_POINT('Ctrl Pts',(87.0705959386853,61.3483791469246,12.9195852492142));
#68836=CARTESIAN_POINT('Ctrl Pts',(87.0650907243153,61.3475630596248,12.9134805073078));
#68837=CARTESIAN_POINT('Ctrl Pts',(87.0523180097064,61.3456429490747,12.8990373235115));
#68838=CARTESIAN_POINT('Ctrl Pts',(87.0450995568168,61.3445369685392,12.8906566890633));
#68839=CARTESIAN_POINT('Ctrl Pts',(87.0200884312836,61.3406292549831,12.8608398151946));
#68840=CARTESIAN_POINT('Ctrl Pts',(87.0028940895592,61.337804144048,12.8389154116862));
#68841=CARTESIAN_POINT('Ctrl Pts',(86.9321560112146,61.3255473174032,12.7423385423571));
#68842=CARTESIAN_POINT('Ctrl Pts',(86.8860859670684,61.3158598779851,12.6625737176514));
#68843=CARTESIAN_POINT('Ctrl Pts',(86.8285799303909,61.3008521932784,12.5322074239055));
#68844=CARTESIAN_POINT('Ctrl Pts',(86.8109224720278,61.2955400149956,12.4846668162996));
#68845=CARTESIAN_POINT('Ctrl Pts',(86.79251601967,61.2890665721679,12.4242629102094));
#68846=CARTESIAN_POINT('Ctrl Pts',(86.7890565392687,61.2877956355853,12.4122798638718));
#68847=CARTESIAN_POINT('Ctrl Pts',(86.7841561763778,61.2859119585795,12.3943169431151));
#68848=CARTESIAN_POINT('Ctrl Pts',(86.782581441654,61.2852923404082,12.3883749897075));
#68849=CARTESIAN_POINT('Ctrl Pts',(86.7799366135299,61.2842265496947,12.3780943811035));
#68850=CARTESIAN_POINT('Ctrl Pts',(86.7788462158416,61.2837792670188,12.3737613017979));
#68851=CARTESIAN_POINT('Ctrl Pts',(86.7763341001985,61.2827298252713,12.3635511269907));
#68852=CARTESIAN_POINT('Ctrl Pts',(86.7749314472001,61.2821287541778,12.3576694972454));
#68853=CARTESIAN_POINT('Ctrl Pts',(86.7709622309102,61.2803818012319,12.34048263653));
#68854=CARTESIAN_POINT('Ctrl Pts',(86.768508266707,61.2792419410337,12.3291515038521));
#68855=CARTESIAN_POINT('Ctrl Pts',(86.7495248860956,61.2698861062995,12.2353012656534));
#68856=CARTESIAN_POINT('Ctrl Pts',(86.7410768704604,61.2620495744167,12.1513431498856));
#68857=CARTESIAN_POINT('Ctrl Pts',(86.740934028576,61.2472922714272,11.993827225442));
#68858=CARTESIAN_POINT('Ctrl Pts',(86.7472175375862,61.240411302849,11.9206458297219));
#68859=CARTESIAN_POINT('Ctrl Pts',(86.7627722994671,61.231645973084,11.8311950488852));
#68860=CARTESIAN_POINT('Ctrl Pts',(86.7661232965139,61.2299482547671,11.8140323811844));
#68861=CARTESIAN_POINT('Ctrl Pts',(86.7721625378048,61.2271623559286,11.7861728360493));
#68862=CARTESIAN_POINT('Ctrl Pts',(86.7746377912754,61.2260809086662,11.7754316440335));
#68863=CARTESIAN_POINT('Ctrl Pts',(86.7793426699757,61.224126891157,11.7561647888799));
#68864=CARTESIAN_POINT('Ctrl Pts',(86.7815218522959,61.2232559879457,11.7476274021184));
#68865=CARTESIAN_POINT('Ctrl Pts',(86.7863858478783,61.2213818584544,11.7293667869308));
#68866=CARTESIAN_POINT('Ctrl Pts',(86.789098002472,61.2203778041361,11.7196515698128));
#68867=CARTESIAN_POINT('Ctrl Pts',(86.7969111550221,61.2175928385922,11.6928987224275));
#68868=CARTESIAN_POINT('Ctrl Pts',(86.8022545213241,61.215804216653,11.6759351691524));
#68869=CARTESIAN_POINT('Ctrl Pts',(86.8150438105204,61.2117633614103,11.6381230059911));
#68870=CARTESIAN_POINT('Ctrl Pts',(86.8226820462052,61.2095054611166,11.6173462140696));
#68871=CARTESIAN_POINT('Ctrl Pts',(86.8588691665552,61.1994417745509,11.526331293098));
#68872=CARTESIAN_POINT('Ctrl Pts',(86.8931274079359,61.191470383299,11.4585422020029));
#68873=CARTESIAN_POINT('Ctrl Pts',(86.965202114098,61.1771042629775,11.3429072263564));
#68874=CARTESIAN_POINT('Ctrl Pts',(87.0008155311453,61.1707375673016,11.2939341729726));
#68875=CARTESIAN_POINT('Ctrl Pts',(87.0480951903352,61.1632107300248,11.2378209507132));
#68876=CARTESIAN_POINT('Ctrl Pts',(87.0565524969098,61.1618962034919,11.2280881786942));
#68877=CARTESIAN_POINT('Ctrl Pts',(87.0693130828877,61.1599611637829,11.213847118109));
#68878=CARTESIAN_POINT('Ctrl Pts',(87.0735032483444,61.1593332354386,11.2092394555024));
#68879=CARTESIAN_POINT('Ctrl Pts',(87.0810914547256,61.1582096809646,11.2010175135799));
#68880=CARTESIAN_POINT('Ctrl Pts',(87.0844769280797,61.1577131947244,11.1973921455412));
#68881=CARTESIAN_POINT('Ctrl Pts',(87.0921532048355,61.1565981260506,11.1892678786788));
#68882=CARTESIAN_POINT('Ctrl Pts',(87.0964559088106,61.1559804611541,11.1847805285864));
#68883=CARTESIAN_POINT('Ctrl Pts',(87.1097416404478,61.1540948872056,11.1711267818698));
#68884=CARTESIAN_POINT('Ctrl Pts',(87.1188312642634,61.1528346942871,11.1620643271838));
#68885=CARTESIAN_POINT('Ctrl Pts',(87.1406815195704,61.1498699967572,11.1409301609979));
#68886=CARTESIAN_POINT('Ctrl Pts',(87.1535585926777,61.1481731429188,11.1289819682498));
#68887=CARTESIAN_POINT('Ctrl Pts',(87.2036620712746,61.1417388791285,11.0843909242261));
#68888=CARTESIAN_POINT('Ctrl Pts',(87.2425406993975,61.1370881237777,11.0536649486747));
#68889=CARTESIAN_POINT('Ctrl Pts',(87.356348863081,61.1240699380585,10.9740668895071));
#68890=CARTESIAN_POINT('Ctrl Pts',(87.4347697595617,61.1157448178542,10.9307284802098));
#68891=CARTESIAN_POINT('Ctrl Pts',(87.5328437137496,61.105462649378,10.8893270340845));
#68892=CARTESIAN_POINT('Ctrl Pts',(87.5487373255274,61.1038009429318,10.8829928752773));
#68893=CARTESIAN_POINT('Ctrl Pts',(87.5749705045162,61.1010619571658,10.8731473780626));
#68894=CARTESIAN_POINT('Ctrl Pts',(87.5852364499097,61.0999910288497,10.8694447443717));
#68895=CARTESIAN_POINT('Ctrl Pts',(87.6038674442362,61.0980482446964,10.8629951865937));
#68896=CARTESIAN_POINT('Ctrl Pts',(87.6122158885585,61.0971779728037,10.8602020394627));
#68897=CARTESIAN_POINT('Ctrl Pts',(87.6302657337038,61.0952965013182,10.8543710317888));
#68898=CARTESIAN_POINT('Ctrl Pts',(87.6399758362254,61.0942844103567,10.8513624439303));
#68899=CARTESIAN_POINT('Ctrl Pts',(87.6671365777793,61.0914527806203,10.8433029941487));
#68900=CARTESIAN_POINT('Ctrl Pts',(87.6846601772915,61.0896250953969,10.8385097745132));
#68901=CARTESIAN_POINT('Ctrl Pts',(87.714274428277,61.0865329805987,10.8310883223467));
#68902=CARTESIAN_POINT('Ctrl Pts',(87.7263121731393,61.0852751641626,10.8282578091236));
#68903=CARTESIAN_POINT('Ctrl Pts',(87.774521455922,61.0802331881509,10.8176624944004));
#68904=CARTESIAN_POINT('Ctrl Pts',(87.8109795044834,61.0764091539188,10.8113048901459));
#68905=CARTESIAN_POINT('Ctrl Pts',(87.8974968938016,61.067309091157,10.8000842701767));
#68906=CARTESIAN_POINT('Ctrl Pts',(87.9476713247721,61.0620107311654,10.7965850118377));
#68907=CARTESIAN_POINT('Ctrl Pts',(88.0607301794632,61.0500912236701,10.7954202989757));
#68908=CARTESIAN_POINT('Ctrl Pts',(88.1235143050014,61.0434843535356,10.7994342424218));
#68909=CARTESIAN_POINT('Ctrl Pts',(88.1955697362612,61.0360563850724,10.809444286739));
#68910=CARTESIAN_POINT('Ctrl Pts',(88.2053717229579,61.0350493984819,10.8109231483707));
#68911=CARTESIAN_POINT('Ctrl Pts',(88.2207621876077,61.0334746972684,10.8134298069568));
#68912=CARTESIAN_POINT('Ctrl Pts',(88.2263624573441,61.0329030362407,10.8143805368816));
#68913=CARTESIAN_POINT('Ctrl Pts',(88.2369050316431,61.0318296238916,10.8162431554671));
#68914=CARTESIAN_POINT('Ctrl Pts',(88.2418483653488,61.0313274801299,10.8171468108872));
#68915=CARTESIAN_POINT('Ctrl Pts',(88.253651932329,61.0301310568997,10.819377019088));
#68916=CARTESIAN_POINT('Ctrl Pts',(88.2605068330879,61.0294383075161,10.8207308863672));
#68917=CARTESIAN_POINT('Ctrl Pts',(88.2843077099293,61.0270390483697,10.825636079233));
#68918=CARTESIAN_POINT('Ctrl Pts',(88.3011932016384,61.0253475649794,10.8294775484408));
#68919=CARTESIAN_POINT('Ctrl Pts',(88.3437333254339,61.0211001923123,10.8400750290017));
#68920=CARTESIAN_POINT('Ctrl Pts',(88.3692656287461,61.0185639679914,10.8472918696938));
#68921=CARTESIAN_POINT('Ctrl Pts',(88.4501762774964,61.0105104628984,10.8729248259525));
#68922=CARTESIAN_POINT('Ctrl Pts',(88.5045198787597,61.005073948271,10.8943587963042));
#68923=CARTESIAN_POINT('Ctrl Pts',(88.6210301410554,60.9929708391837,10.9498628262516));
#68924=CARTESIAN_POINT('Ctrl Pts',(88.6821990394206,60.9863054711784,10.9855426450779));
#68925=CARTESIAN_POINT('Ctrl Pts',(88.753044660125,60.9779160091621,11.0352135982266));
#68926=CARTESIAN_POINT('Ctrl Pts',(88.7658419663205,60.9763719803194,11.0445478786973));
#68927=CARTESIAN_POINT('Ctrl Pts',(88.7861729448367,60.9738695905455,11.0599678936001));
#68928=CARTESIAN_POINT('Ctrl Pts',(88.7938177910461,60.9729170333199,11.0659050111927));
#68929=CARTESIAN_POINT('Ctrl Pts',(88.8083545369346,60.9710826353569,11.0774632904678));
#68930=CARTESIAN_POINT('Ctrl Pts',(88.8152567515651,60.970201386458,11.0830706276716));
#68931=CARTESIAN_POINT('Ctrl Pts',(88.8311424705024,60.9681486344805,11.0962554757889));
#68932=CARTESIAN_POINT('Ctrl Pts',(88.8400806297975,60.9669750316463,11.1038859737154));
#68933=CARTESIAN_POINT('Ctrl Pts',(88.8689971129555,60.9631151768505,11.1292741111193));
#68934=CARTESIAN_POINT('Ctrl Pts',(88.8885192136849,60.9604083025854,11.1475370490353));
#68935=CARTESIAN_POINT('Ctrl Pts',(88.9347047723489,60.9537434668865,11.193560855304));
#68936=CARTESIAN_POINT('Ctrl Pts',(88.9607088606649,60.9497618104299,11.2219425553835));
#68937=CARTESIAN_POINT('Ctrl Pts',(89.0163915522431,60.9406959988066,11.2885519780994));
#68938=CARTESIAN_POINT('Ctrl Pts',(89.0452557537259,60.9355975275298,11.327385017742));
#68939=CARTESIAN_POINT('Ctrl Pts',(89.1060456107791,60.9239415903658,11.4197437121655));
#68940=CARTESIAN_POINT('Ctrl Pts',(89.1363959033959,60.9173984971018,11.4741735715995));
#68941=CARTESIAN_POINT('Ctrl Pts',(89.1668546779078,60.9100213509881,11.5396920034315));
#68942=CARTESIAN_POINT('Ctrl Pts',(89.1709661546454,60.9090047869203,11.5488165832606));
#68943=CARTESIAN_POINT('Ctrl Pts',(89.1772270701165,60.9074244088925,11.5631617838762));
#68944=CARTESIAN_POINT('Ctrl Pts',(89.179450151319,60.9068565019175,11.5683494206702));
#68945=CARTESIAN_POINT('Ctrl Pts',(89.1835915678772,60.9057857640645,11.5781943204696));
#68946=CARTESIAN_POINT('Ctrl Pts',(89.1855168093425,60.9052825737449,11.5828482303154));
#68947=CARTESIAN_POINT('Ctrl Pts',(89.1900751038955,60.9040777278912,11.5940553306564));
#68948=CARTESIAN_POINT('Ctrl Pts',(89.1926812861844,60.9033776619704,11.6006192762808));
#68949=CARTESIAN_POINT('Ctrl Pts',(89.2016649977172,60.9009229681647,11.623807852012));
#68950=CARTESIAN_POINT('Ctrl Pts',(89.2077480261505,60.8991843069884,11.6405457599817));
#68951=CARTESIAN_POINT('Ctrl Pts',(89.2183138738299,60.896004635772,11.6716407926697));
#68952=CARTESIAN_POINT('Ctrl Pts',(89.2228974043795,60.8945597512141,11.6859595955782));
#68953=CARTESIAN_POINT('Ctrl Pts',(89.2456589669431,60.8870032528819,11.7616706560523));
#68954=CARTESIAN_POINT('Ctrl Pts',(89.2594309872615,60.8810352614868,11.8242961205546));
#68955=CARTESIAN_POINT('Ctrl Pts',(89.2781796805407,60.8685199852618,11.9565160652157));
#68956=CARTESIAN_POINT('Ctrl Pts',(89.2822707927093,60.8619859315341,12.0260082065138));
#68957=CARTESIAN_POINT('Ctrl Pts',(89.280252563712,60.8535914638408,12.1129335871577));
#68958=CARTESIAN_POINT('Ctrl Pts',(89.2794874279133,60.8518962720116,12.1303770765571));
#68959=CARTESIAN_POINT('Ctrl Pts',(89.2776535696369,60.8491136624061,12.1587904374643));
#68960=CARTESIAN_POINT('Ctrl Pts',(89.2768011647089,60.8480329507486,12.169772459961));
#68961=CARTESIAN_POINT('Ctrl Pts',(89.2750100442652,60.8460797235869,12.1895161292931));
#68962=CARTESIAN_POINT('Ctrl Pts',(89.274122767168,60.8452088693105,12.1982818633572));
#68963=CARTESIAN_POINT('Ctrl Pts',(89.2720236368538,60.8433342498632,12.2170669934459));
#68964=CARTESIAN_POINT('Ctrl Pts',(89.2707834174856,60.8423296523453,12.2270825103945));
#68965=CARTESIAN_POINT('Ctrl Pts',(89.2670248058407,60.8395415410742,12.254729674854));
#68966=CARTESIAN_POINT('Ctrl Pts',(89.2642547881442,60.8377502875678,12.2723239112516));
#68967=CARTESIAN_POINT('Ctrl Pts',(89.2589934742126,60.8347284564266,12.3017059307708));
#68968=CARTESIAN_POINT('Ctrl Pts',(89.2567026399418,60.8335043106551,12.3135275855586));
#68969=CARTESIAN_POINT('Ctrl Pts',(89.2389980980549,60.824652893876,12.3984093721431));
#68970=CARTESIAN_POINT('Ctrl Pts',(89.2173384930778,60.8168427602217,12.4700031991672));
#68971=CARTESIAN_POINT('Ctrl Pts',(89.1626360546246,60.8013719478287,12.6062225263108));
#68972=CARTESIAN_POINT('Ctrl Pts',(89.1300881947497,60.7937436940406,12.6707727794641));
#68973=CARTESIAN_POINT('Ctrl Pts',(89.0856267235519,60.7850533668111,12.7429311819748));
#68974=CARTESIAN_POINT('Ctrl Pts',(89.0788647144251,60.783770472458,12.7535488455974));
#68975=CARTESIAN_POINT('Ctrl Pts',(89.0685546012126,60.7818726872346,12.7692185460344));
#68976=CARTESIAN_POINT('Ctrl Pts',(89.0651260620089,60.7812507729356,12.7743475907114));
#68977=CARTESIAN_POINT('Ctrl Pts',(89.0588733419653,60.7801332160649,12.7835556202448));
#68978=CARTESIAN_POINT('Ctrl Pts',(89.0560625253225,60.7796367615692,12.7876432153033));
#68979=CARTESIAN_POINT('Ctrl Pts',(89.0496409850005,60.7785158198425,12.7968654462353));
#68980=CARTESIAN_POINT('Ctrl Pts',(89.0460160555439,60.7778922988448,12.8019899232609));
#68981=CARTESIAN_POINT('Ctrl Pts',(89.0346789594999,60.7759697717492,12.8177674790722));
#68982=CARTESIAN_POINT('Ctrl Pts',(89.0268387989926,60.7746789252239,12.8283283668475));
#68983=CARTESIAN_POINT('Ctrl Pts',(89.0077931929692,60.7716278772176,12.8531674889036));
#68984=CARTESIAN_POINT('Ctrl Pts',(88.9964426871776,60.7698759442727,12.8673314783633));
#68985=CARTESIAN_POINT('Ctrl Pts',(88.9510873718701,60.7631039097122,12.9215071458703));
#68986=CARTESIAN_POINT('Ctrl Pts',(88.9149153462751,60.7581802009993,12.9596413994253));
#68987=CARTESIAN_POINT('Ctrl Pts',(88.8143090140788,60.7452996489449,13.0533257270498));
#68988=CARTESIAN_POINT('Ctrl Pts',(88.7464928553373,60.7373692821362,13.1048284635556));
#68989=CARTESIAN_POINT('Ctrl Pts',(88.6593103316625,60.7274982961221,13.1581961392912));
#68990=CARTESIAN_POINT('Ctrl Pts',(88.6443882420474,60.7258199663285,13.1669168725673));
#68991=CARTESIAN_POINT('Ctrl Pts',(88.6197168925839,60.7230593173874,13.1806676413267));
#68992=CARTESIAN_POINT('Ctrl Pts',(88.6100717616313,60.7219835244706,13.1858808918232));
#68993=CARTESIAN_POINT('Ctrl Pts',(88.5925596452606,60.7200355639199,13.1950553301142));
#68994=CARTESIAN_POINT('Ctrl Pts',(88.5847165324487,60.7191650186697,13.1990608500753));
#68995=CARTESIAN_POINT('Ctrl Pts',(88.5677650927728,60.7172870337944,13.2074969186101));
#68996=CARTESIAN_POINT('Ctrl Pts',(88.5586442293293,60.7162787325571,13.2119006791855));
#68997=CARTESIAN_POINT('Ctrl Pts',(88.5331827029968,60.7134691410883,13.2238206775217));
#68998=CARTESIAN_POINT('Ctrl Pts',(88.5167343548591,60.7116599115199,13.2310992119881));
#68999=CARTESIAN_POINT('Ctrl Pts',(88.479408356469,60.7075643917685,13.2466770004623));
#69000=CARTESIAN_POINT('Ctrl Pts',(88.4584544621202,60.7052721971682,13.2547762260141));
#69001=CARTESIAN_POINT('Ctrl Pts',(88.3872739183882,60.6975047363219,13.280140911208));
#69002=CARTESIAN_POINT('Ctrl Pts',(88.336187508737,60.6919586518948,13.2948091072172));
#69003=CARTESIAN_POINT('Ctrl Pts',(88.2019451115022,60.6774955219948,13.3243952643226));
#69004=CARTESIAN_POINT('Ctrl Pts',(88.1179380832077,60.6685410013155,13.3343003868593));
#69005=CARTESIAN_POINT('Ctrl Pts',(88.0219927568398,60.6587150348582,13.3360051344541));
#69006=CARTESIAN_POINT('Ctrl Pts',(88.0104208184317,60.6575368493075,13.3360525898162));
#69007=CARTESIAN_POINT('Ctrl Pts',(87.9928077368159,60.6557555584152,13.3358840668625));
#69008=CARTESIAN_POINT('Ctrl Pts',(87.98676660887,60.6551467357265,13.3357831507682));
#69009=CARTESIAN_POINT('Ctrl Pts',(87.9762590791396,60.654091762245,13.3355326049295));
#69010=CARTESIAN_POINT('Ctrl Pts',(87.9717925690407,60.6536445851165,13.3354025154184));
#69011=CARTESIAN_POINT('Ctrl Pts',(87.9611784734092,60.6525848889832,13.3350372962565));
#69012=CARTESIAN_POINT('Ctrl Pts',(87.9550317626866,60.65197354117,13.3347810709605));
#69013=CARTESIAN_POINT('Ctrl Pts',(87.9364053494587,60.650127336134,13.3338690000461));
#69014=CARTESIAN_POINT('Ctrl Pts',(87.923932617156,60.6488997362385,13.3330735878738));
#69015=CARTESIAN_POINT('Ctrl Pts',(87.8607344508875,60.6427137320059,13.3281056032403));
#69016=CARTESIAN_POINT('Ctrl Pts',(87.8102730065004,60.6378853542181,13.3210699938175));
#69017=CARTESIAN_POINT('Ctrl Pts',(87.669639195398,60.6243844507333,13.2927587679696));
#69018=CARTESIAN_POINT('Ctrl Pts',(87.5811911999741,60.6158212116285,13.2646355601221));
#69019=CARTESIAN_POINT('Ctrl Pts',(87.4717296322412,60.6043568101499,13.216141992184));
#69020=CARTESIAN_POINT('Ctrl Pts',(87.4472349491453,60.601732816823,13.2043355626842));
#69021=CARTESIAN_POINT('Ctrl Pts',(87.4134303393534,60.5980142202727,13.1866830431926));
#69022=CARTESIAN_POINT('Ctrl Pts',(87.4037871783418,60.596942031329,13.1814875856111));
#69023=CARTESIAN_POINT('Ctrl Pts',(87.3866573811285,60.5950159276153,13.1719706137417));
#69024=CARTESIAN_POINT('Ctrl Pts',(87.3791452659407,60.5941637161662,13.1676960969297));
#69025=CARTESIAN_POINT('Ctrl Pts',(87.3644879467617,60.5924855983681,13.1591566226551));
#69026=CARTESIAN_POINT('Ctrl Pts',(87.3573398616816,60.5916599360368,13.1548974477872));
#69027=CARTESIAN_POINT('Ctrl Pts',(87.3425504892741,60.5899360419425,13.145887127631));
#69028=CARTESIAN_POINT('Ctrl Pts',(87.3349168460184,60.5890374233177,13.1411244183783));
#69029=CARTESIAN_POINT('Ctrl Pts',(87.3169723512385,60.586903576258,13.1296619832101));
#69030=CARTESIAN_POINT('Ctrl Pts',(87.306707156875,60.5856658523402,13.1228929726749));
#69031=CARTESIAN_POINT('Ctrl Pts',(87.2794312088592,60.5823298592722,13.1043330195237));
#69032=CARTESIAN_POINT('Ctrl Pts',(87.2626085781958,60.5802219721444,13.0922740917119));
#69033=CARTESIAN_POINT('Ctrl Pts',(87.2236901005184,60.5752223005046,13.0629104536629));
#69034=CARTESIAN_POINT('Ctrl Pts',(87.201862967003,60.5723202688287,13.0452771747944));
#69035=CARTESIAN_POINT('Ctrl Pts',(87.180642808438,60.5693987930815,13.0269406508319));
#69036=CARTESIAN_POINT('Origin',(88.011,66.41344859951,12.066));
#69037=CARTESIAN_POINT('',(87.1806428411249,59.6047173123478,13.026940679077));
#69038=CARTESIAN_POINT('',(87.1806428354195,59.7737921350435,13.0269406741468));
#69039=CARTESIAN_POINT('',(87.1806428354228,66.41344859951,13.0269406741497));
#69040=CARTESIAN_POINT('',(86.7410003192602,60.2915568442934,12.0650994886321));
#69041=CARTESIAN_POINT('Ctrl Pts',(87.1806428411249,59.6047173123478,13.026940679077));
#69042=CARTESIAN_POINT('Ctrl Pts',(87.1864097172424,59.6055103894119,13.0319238866493));
#69043=CARTESIAN_POINT('Ctrl Pts',(87.1922216809976,59.606304961203,13.0368553793557));
#69044=CARTESIAN_POINT('Ctrl Pts',(87.2352838327035,59.6121574675507,13.072732113043));
#69045=CARTESIAN_POINT('Ctrl Pts',(87.2742300148467,59.6172640675625,13.1015745071691));
#69046=CARTESIAN_POINT('Ctrl Pts',(87.3667989435877,59.6289324183003,13.1622581943341));
#69047=CARTESIAN_POINT('Ctrl Pts',(87.4213210504429,59.6354798136871,13.1925248111393));
#69048=CARTESIAN_POINT('Ctrl Pts',(87.4868321943151,59.6428495403356,13.2228258344779));
#69049=CARTESIAN_POINT('Ctrl Pts',(87.4958612845595,59.6438547139304,13.2268746813009));
#69050=CARTESIAN_POINT('Ctrl Pts',(87.5101440154885,59.6454272862379,13.2330799073028));
#69051=CARTESIAN_POINT('Ctrl Pts',(87.5153660527098,59.6459986135798,13.2353071547618));
#69052=CARTESIAN_POINT('Ctrl Pts',(87.5252408018775,59.6470719273441,13.2394407864639));
#69053=CARTESIAN_POINT('Ctrl Pts',(87.5298899555873,59.6475743023467,13.2413545869324));
#69054=CARTESIAN_POINT('Ctrl Pts',(87.541037097452,59.6487720045797,13.2458660246204));
#69055=CARTESIAN_POINT('Ctrl Pts',(87.5475454258268,59.6494657938174,13.2484376651068));
#69056=CARTESIAN_POINT('Ctrl Pts',(87.5702883978015,59.6518723037355,13.257207474264));
#69057=CARTESIAN_POINT('Ctrl Pts',(87.5866299078509,59.6535698789825,13.2631265999381));
#69058=CARTESIAN_POINT('Ctrl Pts',(87.6283376759949,59.6578363645302,13.2772722072251));
#69059=CARTESIAN_POINT('Ctrl Pts',(87.6538519698315,59.6603853856485,13.2850391172413));
#69060=CARTESIAN_POINT('Ctrl Pts',(87.7780622303438,59.67259281175,13.3186150362462));
#69061=CARTESIAN_POINT('Ctrl Pts',(87.8793770561229,59.6819728373679,13.3332729795152));
#69062=CARTESIAN_POINT('Ctrl Pts',(87.9960907178478,59.6931026882281,13.3359980075827));
#69063=CARTESIAN_POINT('Ctrl Pts',(88.0108295516206,59.6945133750901,13.3360854940337));
#69064=CARTESIAN_POINT('Ctrl Pts',(88.0485557527999,59.6981421129972,13.3356527730552));
#69065=CARTESIAN_POINT('Ctrl Pts',(88.0715323361801,59.7003692108582,13.33476486405));
#69066=CARTESIAN_POINT('Ctrl Pts',(88.1055527931119,59.703700584226,13.3325240299627));
#69067=CARTESIAN_POINT('Ctrl Pts',(88.1166245510807,59.7047900686572,13.331648760194));
#69068=CARTESIAN_POINT('Ctrl Pts',(88.1364654235879,59.7067529318179,13.3298181100854));
#69069=CARTESIAN_POINT('Ctrl Pts',(88.1452388992882,59.7076245811301,13.3289163455667));
#69070=CARTESIAN_POINT('Ctrl Pts',(88.1639721613022,59.7094941193103,13.3267934797504));
#69071=CARTESIAN_POINT('Ctrl Pts',(88.1739282115889,59.7104927918946,13.3255455782775));
#69072=CARTESIAN_POINT('Ctrl Pts',(88.2012288276228,59.7132460293099,13.3217946005028));
#69073=CARTESIAN_POINT('Ctrl Pts',(88.2185371968415,59.7150080124499,13.3190504054622));
#69074=CARTESIAN_POINT('Ctrl Pts',(88.3157681182293,59.7250055510302,13.3015650725707));
#69075=CARTESIAN_POINT('Ctrl Pts',(88.394169293903,59.7334663216204,13.2795402324954));
#69076=CARTESIAN_POINT('Ctrl Pts',(88.5433942704597,59.7503199452271,13.2217105435813));
#69077=CARTESIAN_POINT('Ctrl Pts',(88.6140739312873,59.7586695006284,13.1864530980265));
#69078=CARTESIAN_POINT('Ctrl Pts',(88.6913663863026,59.7679925812268,13.1384502198198));
#69079=CARTESIAN_POINT('Ctrl Pts',(88.701605302034,59.7692314905063,13.1318856644774));
#69080=CARTESIAN_POINT('Ctrl Pts',(88.7168255736375,59.7710773894026,13.1218159459799));
#69081=CARTESIAN_POINT('Ctrl Pts',(88.7218781294407,59.7716908725467,13.1184207062269));
#69082=CARTESIAN_POINT('Ctrl Pts',(88.7305961863776,59.772750421393,13.1124708718982));
#69083=CARTESIAN_POINT('Ctrl Pts',(88.7342727838351,59.7731975499993,13.1099331586263));
#69084=CARTESIAN_POINT('Ctrl Pts',(88.7429434987344,59.7742527741648,13.1038805356081));
#69085=CARTESIAN_POINT('Ctrl Pts',(88.7479257749815,59.7748597336624,13.1003489253615));
#69086=CARTESIAN_POINT('Ctrl Pts',(88.7628342433868,59.7766784885708,13.0896188781199));
#69087=CARTESIAN_POINT('Ctrl Pts',(88.7726823438275,59.7778833397084,13.0823121494428));
#69088=CARTESIAN_POINT('Ctrl Pts',(88.8211592819316,59.7838406141739,13.0452444361687));
#69089=CARTESIAN_POINT('Ctrl Pts',(88.8581633820857,59.7884735469755,13.0134141081119));
#69090=CARTESIAN_POINT('Ctrl Pts',(88.9553545022076,59.8012014539556,12.9195507615541));
#69091=CARTESIAN_POINT('Ctrl Pts',(89.0111779383046,59.8091935424723,12.8533993574653));
#69092=CARTESIAN_POINT('Ctrl Pts',(89.0788260111468,59.8206247317788,12.7543162161129));
#69093=CARTESIAN_POINT('Ctrl Pts',(89.0966804607157,59.823858328215,12.7257947399214));
#69094=CARTESIAN_POINT('Ctrl Pts',(89.1198832983829,59.8284075651725,12.6852328744903));
#69095=CARTESIAN_POINT('Ctrl Pts',(89.126209721781,59.8296883706978,12.6737653887985));
#69096=CARTESIAN_POINT('Ctrl Pts',(89.136211366755,59.831782303417,12.6549539678651));
#69097=CARTESIAN_POINT('Ctrl Pts',(89.1399948398496,59.832591573042,12.6476683245687));
#69098=CARTESIAN_POINT('Ctrl Pts',(89.1478162076839,59.8343017754174,12.6322432858404));
#69099=CARTESIAN_POINT('Ctrl Pts',(89.1518378942699,59.8352032178089,12.6240962612856));
#69100=CARTESIAN_POINT('Ctrl Pts',(89.1613608888962,59.8373928856997,12.6042717208092));
#69101=CARTESIAN_POINT('Ctrl Pts',(89.1667720959559,59.8386841189874,12.5925524196967));
#69102=CARTESIAN_POINT('Ctrl Pts',(89.1860430979034,59.84346339771,12.5490875137389));
#69103=CARTESIAN_POINT('Ctrl Pts',(89.1987795089136,59.8469882551037,12.5168648171855));
#69104=CARTESIAN_POINT('Ctrl Pts',(89.2290399227496,59.8564470715648,12.4300864458039));
#69105=CARTESIAN_POINT('Ctrl Pts',(89.2442154831554,59.8624416981865,12.3748009500596));
#69106=CARTESIAN_POINT('Ctrl Pts',(89.2709802489522,59.876610886668,12.2429718009351));
#69107=CARTESIAN_POINT('Ctrl Pts',(89.2794129723557,59.8847926316677,12.1660025816947));
#69108=CARTESIAN_POINT('Ctrl Pts',(89.2810159498217,59.8939688087022,12.0764783079947));
#69109=CARTESIAN_POINT('Ctrl Pts',(89.281057939044,59.8952179381108,12.0642169003687));
#69110=CARTESIAN_POINT('Ctrl Pts',(89.2808548198468,59.8970759276727,12.0458499340424));
#69111=CARTESIAN_POINT('Ctrl Pts',(89.2807432524481,59.8976914027513,12.039744197116));
#69112=CARTESIAN_POINT('Ctrl Pts',(89.2804738281,59.8987528852676,12.0291740447635));
#69113=CARTESIAN_POINT('Ctrl Pts',(89.2803364583437,59.8991999714567,12.0247094549634));
#69114=CARTESIAN_POINT('Ctrl Pts',(89.2799562305113,59.9002532161487,12.0141624067431));
#69115=CARTESIAN_POINT('Ctrl Pts',(89.2796931961772,59.9008582537826,12.0080808266201));
#69116=CARTESIAN_POINT('Ctrl Pts',(89.2787736243369,59.9026652327298,11.9898559320102));
#69117=CARTESIAN_POINT('Ctrl Pts',(89.2779863633824,59.9038603613856,11.977719330808));
#69118=CARTESIAN_POINT('Ctrl Pts',(89.2763244812151,59.9059127747364,11.9567643369617));
#69119=CARTESIAN_POINT('Ctrl Pts',(89.2755317333161,59.9067735818509,11.9479407712464));
#69120=CARTESIAN_POINT('Ctrl Pts',(89.2730897073606,59.909138897631,11.9236185738));
#69121=CARTESIAN_POINT('Ctrl Pts',(89.271247309638,59.9106357267777,11.9081403248429));
#69122=CARTESIAN_POINT('Ctrl Pts',(89.2597845629129,59.9186578040058,11.8249237544407));
#69123=CARTESIAN_POINT('Ctrl Pts',(89.2449866405748,59.9250221903631,11.75800758475));
#69124=CARTESIAN_POINT('Ctrl Pts',(89.2041894126595,59.9380363026289,11.6253803430995));
#69125=CARTESIAN_POINT('Ctrl Pts',(89.1779660158645,59.9446679931572,11.5600016955939));
#69126=CARTESIAN_POINT('Ctrl Pts',(89.1393850022589,59.9530198165272,11.4829926702472));
#69127=CARTESIAN_POINT('Ctrl Pts',(89.1320357610648,59.9545619574872,11.4689832255249));
#69128=CARTESIAN_POINT('Ctrl Pts',(89.1197725492024,59.9570621731697,11.4466317146102));
#69129=CARTESIAN_POINT('Ctrl Pts',(89.1150212922957,59.9580144648305,11.4382017743882));
#69130=CARTESIAN_POINT('Ctrl Pts',(89.1057179510166,59.9598489450729,11.4221275340114));
#69131=CARTESIAN_POINT('Ctrl Pts',(89.1011809354346,59.9607305460383,11.414475125187));
#69132=CARTESIAN_POINT('Ctrl Pts',(89.0904576251176,59.9627850188581,11.3968141746501));
#69133=CARTESIAN_POINT('Ctrl Pts',(89.0842120113998,59.9639599998065,11.3868428842323));
#69134=CARTESIAN_POINT('Ctrl Pts',(89.0632870827719,59.9678287305611,11.3544451587661));
#69135=CARTESIAN_POINT('Ctrl Pts',(89.0480375049121,59.9705432319403,11.3323983821087));
#69136=CARTESIAN_POINT('Ctrl Pts',(89.0091343643087,59.9772315374075,11.2797939179607));
#69137=CARTESIAN_POINT('Ctrl Pts',(88.9847630422855,59.9812292611661,11.2498032924139));
#69138=CARTESIAN_POINT('Ctrl Pts',(88.9270065427525,59.9902944739702,11.185004216518));
#69139=CARTESIAN_POINT('Ctrl Pts',(88.8929278862889,59.9953755545205,11.1508911396011));
#69140=CARTESIAN_POINT('Ctrl Pts',(88.8106526160103,60.0070045235533,11.0774067049815));
#69141=CARTESIAN_POINT('Ctrl Pts',(88.7613264999452,60.0135380054576,11.0394652815236));
#69142=CARTESIAN_POINT('Ctrl Pts',(88.7010562978377,60.0209058781142,10.9997812520955));
#69143=CARTESIAN_POINT('Ctrl Pts',(88.6926342869865,60.0219222813916,10.9943774759073));
#69144=CARTESIAN_POINT('Ctrl Pts',(88.6793628225291,60.0235025390601,10.9860819509878));
#69145=CARTESIAN_POINT('Ctrl Pts',(88.6745567692603,60.0240704844305,10.9831222258957));
#69146=CARTESIAN_POINT('Ctrl Pts',(88.6654237918273,60.0251413967369,10.9775814772922));
#69147=CARTESIAN_POINT('Ctrl Pts',(88.6611011912416,60.0256447224984,10.9749941233115));
#69148=CARTESIAN_POINT('Ctrl Pts',(88.6506791329427,60.0268500484688,10.9688397893295));
#69149=CARTESIAN_POINT('Ctrl Pts',(88.6445650759542,60.02755045681,10.9652978494961));
#69150=CARTESIAN_POINT('Ctrl Pts',(88.62292558838,60.0300071937132,10.9530019196291));
#69151=CARTESIAN_POINT('Ctrl Pts',(88.607244606253,60.0317475226326,10.9445232332478));
#69152=CARTESIAN_POINT('Ctrl Pts',(88.5780001452554,60.0349307524802,10.9294977277729));
#69153=CARTESIAN_POINT('Ctrl Pts',(88.5644893508698,60.0363775259461,10.922856889301));
#69154=CARTESIAN_POINT('Ctrl Pts',(88.4927741574754,60.0439501632778,10.8891770815599));
#69155=CARTESIAN_POINT('Ctrl Pts',(88.43269557612,60.049931829868,10.8663363191612));
#69156=CARTESIAN_POINT('Ctrl Pts',(88.2985520681039,60.06304185434,10.8266679337592));
#69157=CARTESIAN_POINT('Ctrl Pts',(88.2242004812316,60.0701614273871,10.8117382201878));
#69158=CARTESIAN_POINT('Ctrl Pts',(88.1332438405693,60.0790334730091,10.8017979816399));
#69159=CARTESIAN_POINT('Ctrl Pts',(88.1174867396182,60.0805757348901,10.8003733485823));
#69160=CARTESIAN_POINT('Ctrl Pts',(88.0920556933111,60.0830760981488,10.7985523211855));
#69161=CARTESIAN_POINT('Ctrl Pts',(88.0823961825634,60.0840284152009,10.7979715239093));
#69162=CARTESIAN_POINT('Ctrl Pts',(88.0638455724982,60.0858629121552,10.7970687612349));
#69163=CARTESIAN_POINT('Ctrl Pts',(88.0549558346225,60.0867445041974,10.7967297302787));
#69164=CARTESIAN_POINT('Ctrl Pts',(88.0343028683971,60.0887989077393,10.7961593030879));
#69165=CARTESIAN_POINT('Ctrl Pts',(88.0225387612108,60.0899738278763,10.7959979321907));
#69166=CARTESIAN_POINT('Ctrl Pts',(87.9839753426639,60.0938421275821,10.7960047761247));
#69167=CARTESIAN_POINT('Ctrl Pts',(87.9571856743054,60.096556252264,10.7968577924654));
#69168=CARTESIAN_POINT('Ctrl Pts',(87.8919016807957,60.1032433876287,10.8010070282923));
#69169=CARTESIAN_POINT('Ctrl Pts',(87.8534943888634,60.1072403065903,10.8052133700512));
#69170=CARTESIAN_POINT('Ctrl Pts',(87.7677270955098,60.116305550617,10.8185864142649));
#69171=CARTESIAN_POINT('Ctrl Pts',(87.7205753850193,60.1213875033316,10.8287145161416));
#69172=CARTESIAN_POINT('Ctrl Pts',(87.6187766849386,60.1325175375429,10.856721232812));
#69173=CARTESIAN_POINT('Ctrl Pts',(87.5645253362169,60.1385536229741,10.8756822297417));
#69174=CARTESIAN_POINT('Ctrl Pts',(87.4998954229557,60.1457636480785,10.9033143340654));
#69175=CARTESIAN_POINT('Ctrl Pts',(87.4881309988338,60.1470767142894,10.9085571719467));
#69176=CARTESIAN_POINT('Ctrl Pts',(87.4708001538758,60.1490101144421,10.916598900991));
#69177=CARTESIAN_POINT('Ctrl Pts',(87.4651718654194,60.1496378446864,10.9192609653247));
#69178=CARTESIAN_POINT('Ctrl Pts',(87.4584587260366,60.1503862057366,10.9224967670559));
#69179=CARTESIAN_POINT('Ctrl Pts',(87.4573550483126,60.1505092286417,10.9230307218889));
#69180=CARTESIAN_POINT('Ctrl Pts',(87.4518139404406,60.1511268101697,10.9257213967998));
#69181=CARTESIAN_POINT('Ctrl Pts',(87.447388432745,60.1516198142492,10.9279023129664));
#69182=CARTESIAN_POINT('Ctrl Pts',(87.4369574145216,60.1527814766958,10.9331185480976));
#69183=CARTESIAN_POINT('Ctrl Pts',(87.430963106902,60.153448774139,10.9361759056805));
#69184=CARTESIAN_POINT('Ctrl Pts',(87.4180891489265,60.1548820069591,10.9428716541163));
#69185=CARTESIAN_POINT('Ctrl Pts',(87.4112180120408,60.1556470071798,10.9465259556218));
#69186=CARTESIAN_POINT('Ctrl Pts',(87.3921310462667,60.1577735138657,10.9569032395713));
#69187=CARTESIAN_POINT('Ctrl Pts',(87.379991180918,60.1591277146882,10.9637648492937));
#69188=CARTESIAN_POINT('Ctrl Pts',(87.3389280877992,60.1637232982886,10.9878751295065));
#69189=CARTESIAN_POINT('Ctrl Pts',(87.3105766907857,60.166922265155,11.0060747442042));
#69190=CARTESIAN_POINT('Ctrl Pts',(87.1896864994572,60.1808407732127,11.0906499720599));
#69191=CARTESIAN_POINT('Ctrl Pts',(87.1056036715962,60.1913174326432,11.1681589650204));
#69192=CARTESIAN_POINT('Ctrl Pts',(87.0216008061686,60.2040500693866,11.2695658862431));
#69193=CARTESIAN_POINT('Ctrl Pts',(87.0105150689038,60.205784669366,11.2835372916383));
#69194=CARTESIAN_POINT('Ctrl Pts',(86.9935569676644,60.2085296434995,11.3058593985644));
#69195=CARTESIAN_POINT('Ctrl Pts',(86.9874844467381,60.2095321587437,11.3140558829107));
#69196=CARTESIAN_POINT('Ctrl Pts',(86.9764062663062,60.2113986689382,11.3293916798485));
#69197=CARTESIAN_POINT('Ctrl Pts',(86.9713740751679,60.2122615789653,11.3365111804052));
#69198=CARTESIAN_POINT('Ctrl Pts',(86.9602553064012,60.2142029402878,11.3525906441391));
#69199=CARTESIAN_POINT('Ctrl Pts',(86.9542093497211,60.2152828483266,11.3615776671915));
#69200=CARTESIAN_POINT('Ctrl Pts',(86.9368718658452,60.2184529129293,11.3880746152205));
#69201=CARTESIAN_POINT('Ctrl Pts',(86.9258960611566,60.2205544333014,11.4057853483354));
#69202=CARTESIAN_POINT('Ctrl Pts',(86.9109833777392,60.2235513745861,11.4312257205569));
#69203=CARTESIAN_POINT('Ctrl Pts',(86.906681793585,60.2244338403733,11.4387390933388));
#69204=CARTESIAN_POINT('Ctrl Pts',(86.859744542713,60.2342672364061,11.5227016095568));
#69205=CARTESIAN_POINT('Ctrl Pts',(86.8250534618013,60.2434742647721,11.6033045255132));
#69206=CARTESIAN_POINT('Ctrl Pts',(86.7837308148364,60.258063347428,11.7353926333651));
#69207=CARTESIAN_POINT('Ctrl Pts',(86.7714658491329,60.2634163764788,11.7848468198341));
#69208=CARTESIAN_POINT('Ctrl Pts',(86.759208191377,60.2703618972674,11.8510862059905));
#69209=CARTESIAN_POINT('Ctrl Pts',(86.7565289271417,60.2720465568103,11.8673216457429));
#69210=CARTESIAN_POINT('Ctrl Pts',(86.753249072366,60.2743635426589,11.8899223411687));
#69211=CARTESIAN_POINT('Ctrl Pts',(86.7523800106275,60.2750087739223,11.8962458644839));
#69212=CARTESIAN_POINT('Ctrl Pts',(86.7509044314333,60.2761633440632,11.9076175386922));
#69213=CARTESIAN_POINT('Ctrl Pts',(86.7502804857078,60.2766736045223,11.9126632568548));
#69214=CARTESIAN_POINT('Ctrl Pts',(86.7491470064829,60.2776445714408,11.9223044967434));
#69215=CARTESIAN_POINT('Ctrl Pts',(86.7486322439709,60.2781055773062,11.9268992236152));
#69216=CARTESIAN_POINT('Ctrl Pts',(86.7475693927491,60.2791032882756,11.9368783878494));
#69217=CARTESIAN_POINT('Ctrl Pts',(86.7470306024409,60.2796394848085,11.9422637646658));
#69218=CARTESIAN_POINT('Ctrl Pts',(86.7457924025061,60.2809515945659,11.9554932170553));
#69219=CARTESIAN_POINT('Ctrl Pts',(86.7451314758564,60.2817255473663,11.9633408346356));
#69220=CARTESIAN_POINT('Ctrl Pts',(86.7422046944127,60.2855620549366,12.0024381294605));
#69221=CARTESIAN_POINT('Ctrl Pts',(86.7410225400618,60.288574242465,12.0337612824082));
#69222=CARTESIAN_POINT('Ctrl Pts',(86.7410003192602,60.2915568442934,12.0650994886321));
#69223=CARTESIAN_POINT('Ctrl Pts',(86.7410003205439,60.2915566721542,12.0650976799659));
#69224=CARTESIAN_POINT('Ctrl Pts',(86.7409240894383,60.3017683369366,12.172391628948));
#69225=CARTESIAN_POINT('Ctrl Pts',(86.754444143447,60.311612008104,12.2792703672195));
#69226=CARTESIAN_POINT('Ctrl Pts',(86.7868810513014,60.323995469413,12.4050305636389));
#69227=CARTESIAN_POINT('Ctrl Pts',(86.7930959706329,60.3261595322167,12.4267195163374));
#69228=CARTESIAN_POINT('Ctrl Pts',(86.8038000312691,60.3295984662617,12.4606358664787));
#69229=CARTESIAN_POINT('Ctrl Pts',(86.8079055126792,60.3308617568952,12.4729801683709));
#69230=CARTESIAN_POINT('Ctrl Pts',(86.816091144573,60.3332812383934,12.4963856159086));
#69231=CARTESIAN_POINT('Ctrl Pts',(86.8201371385682,60.3344362366402,12.5074573293389));
#69232=CARTESIAN_POINT('Ctrl Pts',(86.8275071434947,60.3364722351848,12.5267861308992));
#69233=CARTESIAN_POINT('Ctrl Pts',(86.8307650107969,60.3373509856935,12.5350677562282));
#69234=CARTESIAN_POINT('Ctrl Pts',(86.8377427669702,60.3391904691869,12.5522724710941));
#69235=CARTESIAN_POINT('Ctrl Pts',(86.8414780275297,60.3401516698282,12.5611886445296));
#69236=CARTESIAN_POINT('Ctrl Pts',(86.8515750531427,60.3426905230499,12.5845389049693));
#69237=CARTESIAN_POINT('Ctrl Pts',(86.8581043362792,60.3442737575296,12.5988980524637));
#69238=CARTESIAN_POINT('Ctrl Pts',(86.8946905820938,60.3528479841825,12.6755369723726));
#69239=CARTESIAN_POINT('Ctrl Pts',(86.9295224661454,60.3600007777607,12.735391022093));
#69240=CARTESIAN_POINT('Ctrl Pts',(87.0006619609761,60.3730558770103,12.8374762724348));
#69241=CARTESIAN_POINT('Ctrl Pts',(87.0352106775988,60.3789064665732,12.8807352945362));
#69242=CARTESIAN_POINT('Ctrl Pts',(87.0923204614892,60.3878080199549,12.9433803113379));
#69243=CARTESIAN_POINT('Ctrl Pts',(87.1129261481408,60.3908867910529,12.9644608840851));
#69244=CARTESIAN_POINT('Ctrl Pts',(87.143513253291,60.3952544368415,12.9936479634496));
#69245=CARTESIAN_POINT('Ctrl Pts',(87.1529119460423,60.3965707182698,13.0023487229686));
#69246=CARTESIAN_POINT('Ctrl Pts',(87.1684569822063,60.3987043115595,13.0163087069261));
#69247=CARTESIAN_POINT('Ctrl Pts',(87.1745244669532,60.3995266097241,13.02165373893));
#69248=CARTESIAN_POINT('Ctrl Pts',(87.1806428354305,60.4003450897931,13.0269406741563));
#69249=CARTESIAN_POINT('',(86.7410004024462,60.4614604378065,12.0655714700173));
#69250=CARTESIAN_POINT('Ctrl Pts',(87.180642808438,60.5693987930815,13.0269406508319));
#69251=CARTESIAN_POINT('Ctrl Pts',(87.1668514509425,60.5675000741667,13.01502341862));
#69252=CARTESIAN_POINT('Ctrl Pts',(87.1533164697531,60.5655932091657,13.0028091364898));
#69253=CARTESIAN_POINT('Ctrl Pts',(87.0902562106591,60.5565023682665,12.9433888841665));
#69254=CARTESIAN_POINT('Ctrl Pts',(87.0443378827768,60.5492501406696,12.8925257476688));
#69255=CARTESIAN_POINT('Ctrl Pts',(86.9836260945219,60.5388235484186,12.8132556304197));
#69256=CARTESIAN_POINT('Ctrl Pts',(86.9654433422184,60.5355685429781,12.7875953848512));
#69257=CARTESIAN_POINT('Ctrl Pts',(86.9433660937757,60.5314600235669,12.7538493754804));
#69258=CARTESIAN_POINT('Ctrl Pts',(86.9385804134176,60.5305591617554,12.7463639964599));
#69259=CARTESIAN_POINT('Ctrl Pts',(86.9310121372483,60.5291184268294,12.7342479970414));
#69260=CARTESIAN_POINT('Ctrl Pts',(86.9281799871311,60.528575528943,12.7296489983488));
#69261=CARTESIAN_POINT('Ctrl Pts',(86.922704460818,60.5275187001039,12.7206291674848));
#69262=CARTESIAN_POINT('Ctrl Pts',(86.9200585628836,60.5270046387168,12.7162102050521));
#69263=CARTESIAN_POINT('Ctrl Pts',(86.9135217458638,60.5257257833404,12.705140708422));
#69264=CARTESIAN_POINT('Ctrl Pts',(86.9096642653894,60.5249630975142,12.6984705322085));
#69265=CARTESIAN_POINT('Ctrl Pts',(86.8947589117912,60.5219823209744,12.6721469433502));
#69266=CARTESIAN_POINT('Ctrl Pts',(86.8841734188367,60.519790652363,12.6522340506068));
#69267=CARTESIAN_POINT('Ctrl Pts',(86.8264091406283,60.5073140274506,12.536217506743));
#69268=CARTESIAN_POINT('Ctrl Pts',(86.7909981577031,60.4975005910672,12.434729157224));
#69269=CARTESIAN_POINT('Ctrl Pts',(86.7594527720076,60.4831399417659,12.2862858467083));
#69270=CARTESIAN_POINT('Ctrl Pts',(86.7524792764846,60.4788719375758,12.2421277125554));
#69271=CARTESIAN_POINT('Ctrl Pts',(86.7463868075961,60.4731635595118,12.1836934824722));
#69272=CARTESIAN_POINT('Ctrl Pts',(86.7451596832995,60.471788774652,12.169665504591));
#69273=CARTESIAN_POINT('Ctrl Pts',(86.743501041776,60.4694817297081,12.1462197636754));
#69274=CARTESIAN_POINT('Ctrl Pts',(86.7429406715925,60.468553531286,12.1368120560072));
#69275=CARTESIAN_POINT('Ctrl Pts',(86.7420794162229,60.4667926861632,12.1190184430685));
#69276=CARTESIAN_POINT('Ctrl Pts',(86.7417568407576,60.4659607651159,12.1106340379479));
#69277=CARTESIAN_POINT('Ctrl Pts',(86.7413353038258,60.4644916989347,12.0958706284977));
#69278=CARTESIAN_POINT('Ctrl Pts',(86.7412012842004,60.4638556810233,12.089492822161));
#69279=CARTESIAN_POINT('Ctrl Pts',(86.7410365108009,60.4626336662859,12.0772666904037));
#69280=CARTESIAN_POINT('Ctrl Pts',(86.7409980955029,60.4620479267567,12.0714186239221));
#69281=CARTESIAN_POINT('Ctrl Pts',(86.7410000725785,60.461460928294,12.0655706407219));
#69282=CARTESIAN_POINT('Ctrl Pts',(86.7410000723177,60.461461005802,12.0655714128966));
#69283=CARTESIAN_POINT('Ctrl Pts',(86.7410035807468,60.4604174682608,12.0551751485843));
#69284=CARTESIAN_POINT('Ctrl Pts',(86.7411347450475,60.4593700001011,12.0447796619893));
#69285=CARTESIAN_POINT('Ctrl Pts',(86.7418258923645,60.4565618163828,12.017022315309));
#69286=CARTESIAN_POINT('Ctrl Pts',(86.7426144618169,60.4547943684841,11.9996691485679));
#69287=CARTESIAN_POINT('Ctrl Pts',(86.7511911621361,60.4414687211118,11.8697555220417));
#69288=CARTESIAN_POINT('Ctrl Pts',(86.7735938023613,60.4294794896274,11.7586792191251));
#69289=CARTESIAN_POINT('Ctrl Pts',(86.8183459995588,60.4151066597492,11.6288758128013));
#69290=CARTESIAN_POINT('Ctrl Pts',(86.8270075634458,60.412554435905,11.6059312774439));
#69291=CARTESIAN_POINT('Ctrl Pts',(86.8406456191914,60.4088572623326,11.572745910137));
#69292=CARTESIAN_POINT('Ctrl Pts',(86.8451034389896,60.4076925848355,11.5622994822151));
#69293=CARTESIAN_POINT('Ctrl Pts',(86.8534249291597,60.405596820135,11.5435015922258));
#69294=CARTESIAN_POINT('Ctrl Pts',(86.8572403075064,60.4046634579642,11.535129751527));
#69295=CARTESIAN_POINT('Ctrl Pts',(86.8634687010888,60.4031834317717,11.5218476008105));
#69296=CARTESIAN_POINT('Ctrl Pts',(86.8658229229311,60.4026334552944,11.5169104063442));
#69297=CARTESIAN_POINT('Ctrl Pts',(86.8704123063253,60.4015794416878,11.5074436264952));
#69298=CARTESIAN_POINT('Ctrl Pts',(86.872642630001,60.4010751666809,11.5029120765135));
#69299=CARTESIAN_POINT('Ctrl Pts',(86.8782274057073,60.3998315914154,11.4917337937369));
#69300=CARTESIAN_POINT('Ctrl Pts',(86.8816134170237,60.3990942195876,11.4851029504363));
#69301=CARTESIAN_POINT('Ctrl Pts',(86.8938590972146,60.3964840240597,11.4616340557894));
#69302=CARTESIAN_POINT('Ctrl Pts',(86.903039280859,60.3946293413746,11.4449644339018));
#69303=CARTESIAN_POINT('Ctrl Pts',(86.9517207621961,60.3852583232002,11.3610857758765));
#69304=CARTESIAN_POINT('Ctrl Pts',(86.9969802688381,60.3780078841744,11.2974011283249));
#69305=CARTESIAN_POINT('Ctrl Pts',(87.0564013825561,60.3694627320686,11.2282556696287));
#69306=CARTESIAN_POINT('Ctrl Pts',(87.0651560968994,60.3682252131986,11.218383702993));
#69307=CARTESIAN_POINT('Ctrl Pts',(87.1022505248767,60.3630621687693,11.1778458292569));
#69308=CARTESIAN_POINT('Ctrl Pts',(87.1319375668493,60.3591192240722,11.1484532035725));
#69309=CARTESIAN_POINT('Ctrl Pts',(87.184065838396,60.3524164661497,11.1016974168239));
#69310=CARTESIAN_POINT('Ctrl Pts',(87.2057386177599,60.3496876729087,11.0835268911102));
#69311=CARTESIAN_POINT('Ctrl Pts',(87.2353850712284,60.3460149119566,11.0603114216465));
#69312=CARTESIAN_POINT('Ctrl Pts',(87.2428359185309,60.3450967167567,11.0546088951904));
#69313=CARTESIAN_POINT('Ctrl Pts',(87.2508293253045,60.3441164270506,11.0486303989867));
#69314=CARTESIAN_POINT('Ctrl Pts',(87.2513098777843,60.3440575115723,11.0482715106976));
#69315=CARTESIAN_POINT('Ctrl Pts',(87.2522663812217,60.3439402807316,11.0475582255901));
#69316=CARTESIAN_POINT('Ctrl Pts',(87.252742326716,60.3438819656568,11.0472038216451));
#69317=CARTESIAN_POINT('Ctrl Pts',(87.2537139055923,60.3437629591703,11.046481411499));
#69318=CARTESIAN_POINT('Ctrl Pts',(87.2542095591504,60.343702266734,11.0461134329164));
#69319=CARTESIAN_POINT('Ctrl Pts',(87.2552549889167,60.3435742945126,11.0453384762276));
#69320=CARTESIAN_POINT('Ctrl Pts',(87.255804825802,60.3435070116127,11.0449315807693));
#69321=CARTESIAN_POINT('Ctrl Pts',(87.2570208608039,60.3433582579121,11.0440331986613));
#69322=CARTESIAN_POINT('Ctrl Pts',(87.2576872106543,60.3432767792883,11.0435419193037));
#69323=CARTESIAN_POINT('Ctrl Pts',(87.2592921318584,60.3430806167553,11.0423610805626));
#69324=CARTESIAN_POINT('Ctrl Pts',(87.260231170386,60.3429659086248,11.0416721614296));
#69325=CARTESIAN_POINT('Ctrl Pts',(87.2621136708337,60.3427360838546,11.0402950571854));
#69326=CARTESIAN_POINT('Ctrl Pts',(87.263057136918,60.3426209670621,11.0396068797636));
#69327=CARTESIAN_POINT('Ctrl Pts',(87.2709222483913,60.3416618527035,11.0338865598796));
#69328=CARTESIAN_POINT('Ctrl Pts',(87.2778934288681,60.340815259967,11.0289233499963));
#69329=CARTESIAN_POINT('Ctrl Pts',(87.2935367570152,60.3389228130798,11.0180224474262));
#69330=CARTESIAN_POINT('Ctrl Pts',(87.3022334074025,60.3378756486871,11.012121280272));
#69331=CARTESIAN_POINT('Ctrl Pts',(87.3267690010726,60.3349340319622,10.99591354545));
#69332=CARTESIAN_POINT('Ctrl Pts',(87.3427653999889,60.3330307288329,10.9858520930195));
#69333=CARTESIAN_POINT('Ctrl Pts',(87.418702325631,60.3240562334648,10.9404214924469));
#69334=CARTESIAN_POINT('Ctrl Pts',(87.4812483949609,60.3168282414633,10.9096683593934));
#69335=CARTESIAN_POINT('Ctrl Pts',(87.6056152978249,60.3027788501164,10.8607325657639));
#69336=CARTESIAN_POINT('Ctrl Pts',(87.666937179747,60.2959913578817,10.8418155617989));
#69337=CARTESIAN_POINT('Ctrl Pts',(87.7440912572341,60.2877399980517,10.824273016366));
#69338=CARTESIAN_POINT('Ctrl Pts',(87.7588150967908,60.2861782974198,10.8211992115709));
#69339=CARTESIAN_POINT('Ctrl Pts',(87.7910878738539,60.2827874553803,10.8150579995158));
#69340=CARTESIAN_POINT('Ctrl Pts',(87.8086545999132,60.2809623517163,10.8120966209827));
#69341=CARTESIAN_POINT('Ctrl Pts',(87.8332670448773,60.2784385604387,10.808478278488));
#69342=CARTESIAN_POINT('Ctrl Pts',(87.8402635047551,60.2777248772666,10.8075092606052));
#69343=CARTESIAN_POINT('Ctrl Pts',(87.852262361929,60.2765076989983,10.8059493154246));
#69344=CARTESIAN_POINT('Ctrl Pts',(87.8572607360853,60.2760026773558,10.8053296985583));
#69345=CARTESIAN_POINT('Ctrl Pts',(87.8678673663526,60.2749354019706,10.8040788870211));
#69346=CARTESIAN_POINT('Ctrl Pts',(87.8734763180977,60.274373570172,10.8034553126008));
#69347=CARTESIAN_POINT('Ctrl Pts',(87.8890406482697,60.2728211364145,10.8018299073994));
#69348=CARTESIAN_POINT('Ctrl Pts',(87.8990043603895,60.2718347989403,10.8009082617405));
#69349=CARTESIAN_POINT('Ctrl Pts',(87.9708800065457,60.2647662168117,10.7951156341521));
#69350=CARTESIAN_POINT('Ctrl Pts',(88.0330768875784,60.2588965723373,10.7946729880727));
#69351=CARTESIAN_POINT('Ctrl Pts',(88.143081768284,60.248543272269,10.8019707624097));
#69352=CARTESIAN_POINT('Ctrl Pts',(88.1908756794449,60.2440544141098,10.8078822746404));
#69353=CARTESIAN_POINT('Ctrl Pts',(88.2762782741895,60.2358863023116,10.8234124275309));
#69354=CARTESIAN_POINT('Ctrl Pts',(88.3139984831386,60.2322257082214,10.8320681210994));
#69355=CARTESIAN_POINT('Ctrl Pts',(88.3771099069978,60.2259476711114,10.8496187638149));
#69356=CARTESIAN_POINT('Ctrl Pts',(88.4027211524813,60.2233560817217,10.8576233716813));
#69357=CARTESIAN_POINT('Ctrl Pts',(88.4391735922175,60.2195901794098,10.8702969124738));
#69358=CARTESIAN_POINT('Ctrl Pts',(88.4502347460606,60.2184370305506,10.8743157659184));
#69359=CARTESIAN_POINT('Ctrl Pts',(88.4695554479623,60.2164032963423,10.8816410909241));
#69360=CARTESIAN_POINT('Ctrl Pts',(88.4778392527569,60.2155249469263,10.8848817898675));
#69361=CARTESIAN_POINT('Ctrl Pts',(88.4950580776298,60.2136853282097,10.8918273848197));
#69362=CARTESIAN_POINT('Ctrl Pts',(88.5039861316425,60.2127235847301,10.8955478593701));
#69363=CARTESIAN_POINT('Ctrl Pts',(88.5273888837836,60.2101810279045,10.9056154465698));
#69364=CARTESIAN_POINT('Ctrl Pts',(88.5417885325414,60.2085946007076,10.9121311743097));
#69365=CARTESIAN_POINT('Ctrl Pts',(88.6193866698178,60.199920133697,10.9490035458384));
#69366=CARTESIAN_POINT('Ctrl Pts',(88.6800962160467,60.1926654590606,10.9842784650478));
#69367=CARTESIAN_POINT('Ctrl Pts',(88.7860179497301,60.1791111783608,11.0581628201464));
#69368=CARTESIAN_POINT('Ctrl Pts',(88.832044237341,60.1728589534857,11.0952915641633));
#69369=CARTESIAN_POINT('Ctrl Pts',(88.8947304013727,60.1638904419361,11.1535185163842));
#69370=CARTESIAN_POINT('Ctrl Pts',(88.9135742311848,60.1611283003945,11.1721533269596));
#69371=CARTESIAN_POINT('Ctrl Pts',(88.9437367336272,60.1566103283159,11.2039086714241));
#69372=CARTESIAN_POINT('Ctrl Pts',(88.9553942355162,60.1548384607041,11.2166950457194));
#69373=CARTESIAN_POINT('Ctrl Pts',(88.9713871659355,60.1523750259205,11.2349733591058));
#69374=CARTESIAN_POINT('Ctrl Pts',(88.9759432948644,60.1516693624717,11.2402680626605));
#69375=CARTESIAN_POINT('Ctrl Pts',(88.9837016489877,60.1504613770383,11.2494360093404));
#69376=CARTESIAN_POINT('Ctrl Pts',(88.9869249149359,60.1499575900331,11.2532910644673));
#69377=CARTESIAN_POINT('Ctrl Pts',(88.993743647671,60.1488878194823,11.2615454026442));
#69378=CARTESIAN_POINT('Ctrl Pts',(88.9973325879527,60.1483222935644,11.2659498097992));
#69379=CARTESIAN_POINT('Ctrl Pts',(89.007104646624,60.1467751317129,11.278107953104));
#69380=CARTESIAN_POINT('Ctrl Pts',(89.0132269183259,60.1457976174498,11.2859105364497));
#69381=CARTESIAN_POINT('Ctrl Pts',(89.0574941722516,60.1386613871084,11.3437088969176));
#69382=CARTESIAN_POINT('Ctrl Pts',(89.0919779055933,60.1327208098248,11.3964147368404));
#69383=CARTESIAN_POINT('Ctrl Pts',(89.1462822463006,60.1221838011303,11.4946276801337));
#69384=CARTESIAN_POINT('Ctrl Pts',(89.16761116009,60.1175837780683,11.5391388604007));
#69385=CARTESIAN_POINT('Ctrl Pts',(89.2005041785097,60.1094098795592,11.6194739592221));
#69386=CARTESIAN_POINT('Ctrl Pts',(89.2131660534888,60.105859016346,11.6547798270784));
#69387=CARTESIAN_POINT('Ctrl Pts',(89.2320060692898,60.0997475788723,11.7156670526248));
#69388=CARTESIAN_POINT('Ctrl Pts',(89.2389851802726,60.0972109851532,11.7409751273761));
#69389=CARTESIAN_POINT('Ctrl Pts',(89.2479277393318,60.0935103013973,11.777822926435));
#69390=CARTESIAN_POINT('Ctrl Pts',(89.250524086615,60.0923663414885,11.7892035502385));
#69391=CARTESIAN_POINT('Ctrl Pts',(89.254819109716,60.0903430669625,11.8093038507849));
#69392=CARTESIAN_POINT('Ctrl Pts',(89.2565838894772,60.0894659147324,11.8180087604568));
#69393=CARTESIAN_POINT('Ctrl Pts',(89.2600876186308,60.0876230875028,11.8362729515883));
#69394=CARTESIAN_POINT('Ctrl Pts',(89.261808450685,60.0866568989133,11.8458350571947));
#69395=CARTESIAN_POINT('Ctrl Pts',(89.2660742599571,60.0840890239914,11.8712053258467));
#69396=CARTESIAN_POINT('Ctrl Pts',(89.2684301742466,60.082481517482,11.8870428550306));
#69397=CARTESIAN_POINT('Ctrl Pts',(89.2803290575921,60.0731227931811,11.978939199359));
#69398=CARTESIAN_POINT('Ctrl Pts',(89.2832672337271,60.0651698650312,12.0556750447371));
#69399=CARTESIAN_POINT('Ctrl Pts',(89.2759825011512,60.0504723506936,12.1952581467968));
#69400=CARTESIAN_POINT('Ctrl Pts',(89.2679913186369,60.0437843209604,12.2579939507808));
#69401=CARTESIAN_POINT('Ctrl Pts',(89.2523839156594,60.0356434746613,12.3344930333221));
#69402=CARTESIAN_POINT('Ctrl Pts',(89.2491443787244,60.0340946241693,12.3490566743505));
#69403=CARTESIAN_POINT('Ctrl Pts',(89.2414992647507,60.0307270969404,12.3807780454337));
#69404=CARTESIAN_POINT('Ctrl Pts',(89.2369896492882,60.0289124659539,12.3979083451577));
#69405=CARTESIAN_POINT('Ctrl Pts',(89.2301863727758,60.0264005306688,12.4217165405199));
#69406=CARTESIAN_POINT('Ctrl Pts',(89.2281935443151,60.0256884096909,12.4284769688235));
#69407=CARTESIAN_POINT('Ctrl Pts',(89.2246809140559,60.0244730269173,12.4400374059579));
#69408=CARTESIAN_POINT('Ctrl Pts',(89.2231886980304,60.0239682505586,12.4448454926776));
#69409=CARTESIAN_POINT('Ctrl Pts',(89.219960934189,60.0229005114568,12.4550313449205));
#69410=CARTESIAN_POINT('Ctrl Pts',(89.2182180376411,60.0223379774899,12.4604065692954));
#69411=CARTESIAN_POINT('Ctrl Pts',(89.2132791408332,60.0207815236983,12.4752989762207));
#69412=CARTESIAN_POINT('Ctrl Pts',(89.2100059659657,60.0197919043522,12.4847905218853));
#69413=CARTESIAN_POINT('Ctrl Pts',(89.1853562213914,60.0126264878535,12.5536106804058));
#69414=CARTESIAN_POINT('Ctrl Pts',(89.159695304005,60.0066699312221,12.6113246708353));
#69415=CARTESIAN_POINT('Ctrl Pts',(89.1064504115018,59.9961046686516,12.7104635749966));
#69416=CARTESIAN_POINT('Ctrl Pts',(89.08053128416,59.99149256359,12.7526204619303));
#69417=CARTESIAN_POINT('Ctrl Pts',(89.0308598552331,59.9833230716655,12.8237451421177));
#69418=CARTESIAN_POINT('Ctrl Pts',(89.0081635509789,59.9797893012435,12.8533729973936));
#69419=CARTESIAN_POINT('Ctrl Pts',(88.9673921916165,59.97370389382,12.9020013105836));
#69420=CARTESIAN_POINT('Ctrl Pts',(88.9499725673572,59.971175952334,12.9215200236929));
#69421=CARTESIAN_POINT('Ctrl Pts',(88.923936967622,59.9674855406958,12.9489394073195));
#69422=CARTESIAN_POINT('Ctrl Pts',(88.91579406881,59.9663430403737,12.9572819838977));
#69423=CARTESIAN_POINT('Ctrl Pts',(88.9012483083111,59.9643214218385,12.9717796664334));
#69424=CARTESIAN_POINT('Ctrl Pts',(88.8948934384974,59.9634444543544,12.9779820359312));
#69425=CARTESIAN_POINT('Ctrl Pts',(88.8814453254431,59.9616010900584,12.9908348337416));
#69426=CARTESIAN_POINT('Ctrl Pts',(88.8743397418646,59.9606341732648,12.9974714224986));
#69427=CARTESIAN_POINT('Ctrl Pts',(88.8553078899832,59.9580621497967,13.0148422603398));
#69428=CARTESIAN_POINT('Ctrl Pts',(88.8432536697442,59.9564511888635,13.0254327577625));
#69429=CARTESIAN_POINT('Ctrl Pts',(88.7747344669429,59.9473883160021,13.083368858269));
#69430=CARTESIAN_POINT('Ctrl Pts',(88.7144457707105,59.9397513181878,13.1259476384312));
#69431=CARTESIAN_POINT('Ctrl Pts',(88.5943043129406,59.9251372769315,13.1960162677878));
#69432=CARTESIAN_POINT('Ctrl Pts',(88.5353238618296,59.9182053643943,13.2245618378079));
#69433=CARTESIAN_POINT('Ctrl Pts',(88.4602416383834,59.9097938564587,13.2539871106655));
#69434=CARTESIAN_POINT('Ctrl Pts',(88.445978479973,59.9082138332476,13.2592833685066));
#69435=CARTESIAN_POINT('Ctrl Pts',(88.4146823637691,59.9047898163276,13.2702686108586));
#69436=CARTESIAN_POINT('Ctrl Pts',(88.3976161507287,59.9029498475891,13.2758555308192));
#69437=CARTESIAN_POINT('Ctrl Pts',(88.3736577803236,59.9004092422257,13.283139893964));
#69438=CARTESIAN_POINT('Ctrl Pts',(88.3668624355003,59.8996933544845,13.2851440122975));
#69439=CARTESIAN_POINT('Ctrl Pts',(88.3552047631862,59.898473638634,13.2884763718148));
#69440=CARTESIAN_POINT('Ctrl Pts',(88.3503507650248,59.897968267069,13.2898326935102));
#69441=CARTESIAN_POINT('Ctrl Pts',(88.3400542305945,59.8969016283688,13.2926438139266));
#69442=CARTESIAN_POINT('Ctrl Pts',(88.3346099184957,59.8963407736305,13.2940913476253));
#69443=CARTESIAN_POINT('Ctrl Pts',(88.3195151938453,59.8947939288,13.2979973795316));
#69444=CARTESIAN_POINT('Ctrl Pts',(88.3098448673158,59.8938121533718,13.3003787652032));
#69445=CARTESIAN_POINT('Ctrl Pts',(88.2417261463093,59.8869539501636,13.3163059729705));
#69446=CARTESIAN_POINT('Ctrl Pts',(88.1823988697835,59.8812757216819,13.3258114299898));
#69447=CARTESIAN_POINT('Ctrl Pts',(88.0201373592412,59.86596941425,13.3401267949362));
#69448=CARTESIAN_POINT('Ctrl Pts',(87.916959183455,59.8564458532353,13.3366830576952));
#69449=CARTESIAN_POINT('Ctrl Pts',(87.7975017999039,59.8447555443272,13.3180559818069));
#69450=CARTESIAN_POINT('Ctrl Pts',(87.7797335304784,59.84300021778,13.314896074688));
#69451=CARTESIAN_POINT('Ctrl Pts',(87.7520956316299,59.840239960759,13.3093709676742));
#69452=CARTESIAN_POINT('Ctrl Pts',(87.7421761491564,59.839243216483,13.3072640966704));
#69453=CARTESIAN_POINT('Ctrl Pts',(87.7236923906209,59.8373738231152,13.3031062508994));
#69454=CARTESIAN_POINT('Ctrl Pts',(87.7151220824073,59.8365021588852,13.30108452601));
#69455=CARTESIAN_POINT('Ctrl Pts',(87.6959461452258,59.8345403378165,13.2963499096497));
#69456=CARTESIAN_POINT('Ctrl Pts',(87.685353339423,59.8334486897486,13.2935887197072));
#69457=CARTESIAN_POINT('Ctrl Pts',(87.6581885350384,59.8306277992675,13.2861314411078));
#69458=CARTESIAN_POINT('Ctrl Pts',(87.6416746636329,59.8288922492665,13.2812347035655));
#69459=CARTESIAN_POINT('Ctrl Pts',(87.5425887613669,59.818346943232,13.249647407893));
#69460=CARTESIAN_POINT('Ctrl Pts',(87.4628497427745,59.8092792674951,13.2148927773552));
#69461=CARTESIAN_POINT('Ctrl Pts',(87.3426482152655,59.7947334783239,13.1471256126053));
#69462=CARTESIAN_POINT('Ctrl Pts',(87.2995650812477,59.7893228471679,13.1192747533207));
#69463=CARTESIAN_POINT('Ctrl Pts',(87.2438584374867,59.7821274010227,13.0782818073894));
#69464=CARTESIAN_POINT('Ctrl Pts',(87.2296612000493,59.7802750336801,13.0673642733483));
#69465=CARTESIAN_POINT('Ctrl Pts',(87.2055470978375,59.777101726245,13.0479954994836));
#69466=CARTESIAN_POINT('Ctrl Pts',(87.1955208469836,59.7757739068447,13.0396854405763));
#69467=CARTESIAN_POINT('Ctrl Pts',(87.1839596089517,59.7742344080539,13.0297992449294));
#69468=CARTESIAN_POINT('Ctrl Pts',(87.1822993815485,59.7740131259758,13.0283721100135));
#69469=CARTESIAN_POINT('Ctrl Pts',(87.1806428354195,59.7737921350435,13.0269406741468));
#69470=CARTESIAN_POINT('Origin',(88.011,66.41344859951,12.066));
#69471=CARTESIAN_POINT('',(87.1806428565926,58.8108193550848,13.0269406924427));
#69472=CARTESIAN_POINT('',(87.1806427698474,58.9814779498304,13.0269406174855));
#69473=CARTESIAN_POINT('',(87.1806428354228,66.41344859951,13.0269406741497));
#69474=CARTESIAN_POINT('Ctrl Pts',(87.1806428565926,58.8108193550848,13.0269406924427));
#69475=CARTESIAN_POINT('Ctrl Pts',(87.20042835637,58.8133182957622,13.0440375135111));
#69476=CARTESIAN_POINT('Ctrl Pts',(87.2207392038508,58.8158360863611,13.0605209604405));
#69477=CARTESIAN_POINT('Ctrl Pts',(87.2527546337551,58.8197477207029,13.0849025608701));
#69478=CARTESIAN_POINT('Ctrl Pts',(87.2641030172102,58.8211237165168,13.0932503701278));
#69479=CARTESIAN_POINT('Ctrl Pts',(87.2780236979588,58.8228003901362,13.1031377298773));
#69480=CARTESIAN_POINT('Ctrl Pts',(87.2804660979789,58.8230941523717,13.1048595418577));
#69481=CARTESIAN_POINT('Ctrl Pts',(87.2836168211224,58.8234725926762,13.107064093018));
#69482=CARTESIAN_POINT('Ctrl Pts',(87.2843196109945,58.8235569733901,13.1075547738411));
#69483=CARTESIAN_POINT('Ctrl Pts',(87.2920511895596,58.8244849088787,13.1129412498741));
#69484=CARTESIAN_POINT('Ctrl Pts',(87.2991286210109,58.8253310756176,13.1177663730261));
#69485=CARTESIAN_POINT('Ctrl Pts',(87.3141869378347,58.8271250357397,13.1278109468503));
#69486=CARTESIAN_POINT('Ctrl Pts',(87.3221788350464,58.828073422718,13.1330128023858));
#69487=CARTESIAN_POINT('Ctrl Pts',(87.3432463527802,58.8305644699172,13.1463901453943));
#69488=CARTESIAN_POINT('Ctrl Pts',(87.3564131430209,58.8321124069524,13.1544180228542));
#69489=CARTESIAN_POINT('Ctrl Pts',(87.4296178306994,58.8406746803733,13.1972426789486));
#69490=CARTESIAN_POINT('Ctrl Pts',(87.49227059893,58.8478524819101,13.2273057100564));
#69491=CARTESIAN_POINT('Ctrl Pts',(87.6217876555552,58.8624035273499,13.2768750985825));
#69492=CARTESIAN_POINT('Ctrl Pts',(87.6884439007816,58.8697525513365,13.296309898838));
#69493=CARTESIAN_POINT('Ctrl Pts',(87.7717278820269,58.8786246089714,13.3133552530622));
#69494=CARTESIAN_POINT('Ctrl Pts',(87.7871601715485,58.8802554192932,13.3162168051109));
#69495=CARTESIAN_POINT('Ctrl Pts',(87.8114252777765,58.8827958521998,13.3202524480686));
#69496=CARTESIAN_POINT('Ctrl Pts',(87.8202236684018,58.8837121261571,13.3216208334788));
#69497=CARTESIAN_POINT('Ctrl Pts',(87.841116556915,58.8858754362119,13.3246455468171));
#69498=CARTESIAN_POINT('Ctrl Pts',(87.8532224412059,58.8871190257414,13.3262203293242));
#69499=CARTESIAN_POINT('Ctrl Pts',(87.8714056624524,58.8889704627371,13.3283195243027));
#69500=CARTESIAN_POINT('Ctrl Pts',(87.8774665695662,58.8895848592042,13.3289750548276));
#69501=CARTESIAN_POINT('Ctrl Pts',(87.8879766019236,58.8906452875258,13.3300352832618));
#69502=CARTESIAN_POINT('Ctrl Pts',(87.892423339008,58.8910923895879,13.3304601739987));
#69503=CARTESIAN_POINT('Ctrl Pts',(87.9029453796193,58.8921466909904,13.3314095697335));
#69504=CARTESIAN_POINT('Ctrl Pts',(87.909022361407,58.8927527612634,13.3319137992205));
#69505=CARTESIAN_POINT('Ctrl Pts',(87.927282728033,58.8945660621896,13.3332965775776));
#69506=CARTESIAN_POINT('Ctrl Pts',(87.9394759827535,58.8957664096804,13.3340431982068));
#69507=CARTESIAN_POINT('Ctrl Pts',(88.0293939076067,58.9045545341321,13.338247809032));
#69508=CARTESIAN_POINT('Ctrl Pts',(88.1072944280662,58.9118233216788,13.334733626028));
#69509=CARTESIAN_POINT('Ctrl Pts',(88.2408111521557,58.9244485726821,13.3163319226117));
#69510=CARTESIAN_POINT('Ctrl Pts',(88.2966345062918,58.9297790612417,13.3047716316912));
#69511=CARTESIAN_POINT('Ctrl Pts',(88.3847479776103,58.938491664867,13.2802504559741));
#69512=CARTESIAN_POINT('Ctrl Pts',(88.4176106472612,58.9418099046252,13.2696440607536));
#69513=CARTESIAN_POINT('Ctrl Pts',(88.4620957264268,58.9464267017707,13.2532568700053));
#69514=CARTESIAN_POINT('Ctrl Pts',(88.474124855026,58.9476879396393,13.2486164081792));
#69515=CARTESIAN_POINT('Ctrl Pts',(88.4945041336013,58.9498481266325,13.240396121808));
#69516=CARTESIAN_POINT('Ctrl Pts',(88.5028905644028,58.9507439484894,13.2369082628568));
#69517=CARTESIAN_POINT('Ctrl Pts',(88.5187868651132,58.9524555884808,13.2300961898133));
#69518=CARTESIAN_POINT('Ctrl Pts',(88.5263033532051,58.9532708071425,13.2267884758215));
#69519=CARTESIAN_POINT('Ctrl Pts',(88.5457367153453,58.9553942618235,13.2180106657623));
#69520=CARTESIAN_POINT('Ctrl Pts',(88.5576015170478,58.9567062640746,13.212428662046));
#69521=CARTESIAN_POINT('Ctrl Pts',(88.5996908155426,58.9614184437597,13.1918251361288));
#69522=CARTESIAN_POINT('Ctrl Pts',(88.629396994961,58.9648530345703,13.1757854436728));
#69523=CARTESIAN_POINT('Ctrl Pts',(88.7326226601733,58.9771992434842,13.1146176228813));
#69524=CARTESIAN_POINT('Ctrl Pts',(88.8021374202715,58.9863069869873,13.0632136702568));
#69525=CARTESIAN_POINT('Ctrl Pts',(88.9019303280797,59.000514619764,12.9723760070195));
#69526=CARTESIAN_POINT('Ctrl Pts',(88.936051838383,59.0056190514468,12.9375243571157));
#69527=CARTESIAN_POINT('Ctrl Pts',(88.976146442892,59.0118702069012,12.8915559221556));
#69528=CARTESIAN_POINT('Ctrl Pts',(88.9840696552696,59.013119037286,12.8822020111672));
#69529=CARTESIAN_POINT('Ctrl Pts',(88.9957353056992,59.0149766732382,12.8680184907107));
#69530=CARTESIAN_POINT('Ctrl Pts',(88.9995799937007,59.0155920901654,12.8632746599897));
#69531=CARTESIAN_POINT('Ctrl Pts',(89.0061781467855,59.0166535780965,12.8550123022171));
#69532=CARTESIAN_POINT('Ctrl Pts',(89.00894739034,59.0171007270134,12.8515068207103));
#69533=CARTESIAN_POINT('Ctrl Pts',(89.0154467524411,59.0181541200805,12.8431896700297));
#69534=CARTESIAN_POINT('Ctrl Pts',(89.0191608609133,59.0187592430454,12.838365681435));
#69535=CARTESIAN_POINT('Ctrl Pts',(89.0301921724978,59.0205667439344,12.8238227401848));
#69536=CARTESIAN_POINT('Ctrl Pts',(89.037404924874,59.0217623033926,12.8140247055767));
#69537=CARTESIAN_POINT('Ctrl Pts',(89.090239810529,59.0306381076001,12.7400485060891));
#69538=CARTESIAN_POINT('Ctrl Pts',(89.1299546589741,59.0379909803779,12.6718426987577));
#69539=CARTESIAN_POINT('Ctrl Pts',(89.1868169011372,59.0506497537866,12.5492511874));
#69540=CARTESIAN_POINT('Ctrl Pts',(89.2071018933188,59.0559273217316,12.4966001691001));
#69541=CARTESIAN_POINT('Ctrl Pts',(89.2340006019402,59.0645654925653,12.4100154148328));
#69542=CARTESIAN_POINT('Ctrl Pts',(89.2428462254894,59.0678637077985,12.3768560527067));
#69543=CARTESIAN_POINT('Ctrl Pts',(89.2531480468877,59.0724573103752,12.3308277667658));
#69544=CARTESIAN_POINT('Ctrl Pts',(89.2557669168646,59.0737158869787,12.3182316589206));
#69545=CARTESIAN_POINT('Ctrl Pts',(89.2599064864946,59.0758729107632,12.2966837523067));
#69546=CARTESIAN_POINT('Ctrl Pts',(89.2615234095638,59.0767682533639,12.2877512051467));
#69547=CARTESIAN_POINT('Ctrl Pts',(89.2644212435786,59.0784799146793,12.2707015047651));
#69548=CARTESIAN_POINT('Ctrl Pts',(89.2657194051358,59.0792956402615,12.2625877060577));
#69549=CARTESIAN_POINT('Ctrl Pts',(89.2685771599844,59.0812134016638,12.2435432165187));
#69550=CARTESIAN_POINT('Ctrl Pts',(89.2700730876087,59.0823173810698,12.2326038633817));
#69551=CARTESIAN_POINT('Ctrl Pts',(89.2748242710187,59.0862098080011,12.1941288388923));
#69552=CARTESIAN_POINT('Ctrl Pts',(89.2773199658707,59.0890213908358,12.166509835723));
#69553=CARTESIAN_POINT('Ctrl Pts',(89.2841856217554,59.1012771224713,12.0469909280814));
#69554=CARTESIAN_POINT('Ctrl Pts',(89.2794655964512,59.1109784350131,11.9548624127588));
#69555=CARTESIAN_POINT('Ctrl Pts',(89.2567821845668,59.1260050797377,11.8140122977366));
#69556=CARTESIAN_POINT('Ctrl Pts',(89.2457281555832,59.1313220014191,11.7644725044365));
#69557=CARTESIAN_POINT('Ctrl Pts',(89.2282980038939,59.1378006255098,11.7037276722194));
#69558=CARTESIAN_POINT('Ctrl Pts',(89.2246799980459,59.1390721698871,11.6917853899793));
#69559=CARTESIAN_POINT('Ctrl Pts',(89.2190170220599,59.1409566416904,11.6740399503544));
#69560=CARTESIAN_POINT('Ctrl Pts',(89.2171051321596,59.1415764536782,11.6681957490556));
#69561=CARTESIAN_POINT('Ctrl Pts',(89.2137304100429,59.1426425369518,11.6581280423667));
#69562=CARTESIAN_POINT('Ctrl Pts',(89.2122876642428,59.143089919284,11.6538981639411));
#69563=CARTESIAN_POINT('Ctrl Pts',(89.2088401792962,59.1441395514509,11.6439627111359));
#69564=CARTESIAN_POINT('Ctrl Pts',(89.2068169742698,59.1447407131677,11.6382637051677));
#69565=CARTESIAN_POINT('Ctrl Pts',(89.2007965305368,59.1464878362064,11.6216818467075));
#69566=CARTESIAN_POINT('Ctrl Pts',(89.196690714073,59.1476277754067,11.6108385223394));
#69567=CARTESIAN_POINT('Ctrl Pts',(89.161560846331,59.1569836003768,11.521764767786));
#69568=CARTESIAN_POINT('Ctrl Pts',(89.1229732973776,59.1648200580543,11.4467234370874));
#69569=CARTESIAN_POINT('Ctrl Pts',(89.036087144621,59.1798035551961,11.3124531627067));
#69570=CARTESIAN_POINT('Ctrl Pts',(88.9893407595759,59.1869118510022,11.2526839429608));
#69571=CARTESIAN_POINT('Ctrl Pts',(88.9252419498696,59.1959748567709,11.184305158124));
#69572=CARTESIAN_POINT('Ctrl Pts',(88.9126518999797,59.1977261352381,11.17143423319));
#69573=CARTESIAN_POINT('Ctrl Pts',(88.8925549813114,59.2004815879532,11.1517442917592));
#69574=CARTESIAN_POINT('Ctrl Pts',(88.8852323409658,59.201477625847,11.144739730361));
#69575=CARTESIAN_POINT('Ctrl Pts',(88.8713893423093,59.2033465992572,11.131811706739));
#69576=CARTESIAN_POINT('Ctrl Pts',(88.8648895949125,59.2042185572042,11.1258669576052));
#69577=CARTESIAN_POINT('Ctrl Pts',(88.8501630272104,59.2061822418571,11.1126765573942));
#69578=CARTESIAN_POINT('Ctrl Pts',(88.8419032935047,59.207275470377,11.1054689646174));
#69579=CARTESIAN_POINT('Ctrl Pts',(88.8203908190485,59.2101029595542,11.0871819011128));
#69580=CARTESIAN_POINT('Ctrl Pts',(88.8070040030946,59.2118435763466,11.076264721991));
#69581=CARTESIAN_POINT('Ctrl Pts',(88.7262081480871,59.2222448987157,11.0130738036725));
#69582=CARTESIAN_POINT('Ctrl Pts',(88.6539092432021,59.2311538713852,10.9674385199425));
#69583=CARTESIAN_POINT('Ctrl Pts',(88.5308236030654,59.2456499173512,10.9060795073854));
#69584=CARTESIAN_POINT('Ctrl Pts',(88.4826464475312,59.2511698430702,10.8856685180178));
#69585=CARTESIAN_POINT('Ctrl Pts',(88.4081413378865,59.2593906019846,10.8593960815787));
#69586=CARTESIAN_POINT('Ctrl Pts',(88.3826595355958,59.2621483006796,10.851305065599));
#69587=CARTESIAN_POINT('Ctrl Pts',(88.3490770164703,59.2656988046165,10.841797938812));
#69588=CARTESIAN_POINT('Ctrl Pts',(88.3411938796637,59.2665262908386,10.8396481865353));
#69589=CARTESIAN_POINT('Ctrl Pts',(88.3282149127199,59.2678783704152,10.836243019787));
#69590=CARTESIAN_POINT('Ctrl Pts',(88.3231312718628,59.2684053742483,10.8349428915374));
#69591=CARTESIAN_POINT('Ctrl Pts',(88.3135282096159,59.2693958546461,10.83255024509));
#69592=CARTESIAN_POINT('Ctrl Pts',(88.3090106071136,59.269859718943,10.8314509745845));
#69593=CARTESIAN_POINT('Ctrl Pts',(88.2969446227447,59.2710933422148,10.8285850459517));
#69594=CARTESIAN_POINT('Ctrl Pts',(88.289385717149,59.2718606427278,10.8268625986448));
#69595=CARTESIAN_POINT('Ctrl Pts',(88.2611205236775,59.2747110025524,10.8206935239507));
#69596=CARTESIAN_POINT('Ctrl Pts',(88.2403180102299,59.2767712421674,10.8166954207947));
#69597=CARTESIAN_POINT('Ctrl Pts',(88.144290196095,59.2861533146342,10.800719429957));
#69598=CARTESIAN_POINT('Ctrl Pts',(88.0681746429535,59.2932369390329,10.7950021774295));
#69599=CARTESIAN_POINT('Ctrl Pts',(87.9426409780847,59.3050057424609,10.7968807936223));
#69600=CARTESIAN_POINT('Ctrl Pts',(87.893374824232,59.3096451917788,10.8004961095204));
#69601=CARTESIAN_POINT('Ctrl Pts',(87.8231179570695,59.3164107584551,10.8097901261253));
#69602=CARTESIAN_POINT('Ctrl Pts',(87.8018649828742,59.318476958615,10.8131531060513));
#69603=CARTESIAN_POINT('Ctrl Pts',(87.7635949953298,59.3222427143637,10.8202096448806));
#69604=CARTESIAN_POINT('Ctrl Pts',(87.7465487434599,59.3239364586888,10.8237164944718));
#69605=CARTESIAN_POINT('Ctrl Pts',(87.7198209668696,59.3266217440068,10.829790088454));
#69606=CARTESIAN_POINT('Ctrl Pts',(87.7100879642262,59.3276058298153,10.832123139344));
#69607=CARTESIAN_POINT('Ctrl Pts',(87.6918286584813,59.3294644461623,10.8367288730171));
#69608=CARTESIAN_POINT('Ctrl Pts',(87.683296425485,59.3303381010539,10.8389758738516));
#69609=CARTESIAN_POINT('Ctrl Pts',(87.6640411194625,59.3323219442653,10.8442619969252));
#69610=CARTESIAN_POINT('Ctrl Pts',(87.6533334280845,59.3334337719267,10.847353695317));
#69611=CARTESIAN_POINT('Ctrl Pts',(87.6204610892129,59.3368749005233,10.8573156705795));
#69612=CARTESIAN_POINT('Ctrl Pts',(87.5984445170747,59.3392190550098,10.864652322754));
#69613=CARTESIAN_POINT('Ctrl Pts',(87.4850780319608,59.3515077337974,10.9059134233345));
#69614=CARTESIAN_POINT('Ctrl Pts',(87.3976715855024,59.361767224919,10.9496601802298));
#69615=CARTESIAN_POINT('Ctrl Pts',(87.2834896249894,59.3761395652548,11.0242943647909));
#69616=CARTESIAN_POINT('Ctrl Pts',(87.251832404272,59.3802381198795,11.0471344355979));
#69617=CARTESIAN_POINT('Ctrl Pts',(87.2037183856132,59.386608476093,11.0853375000817));
#69618=CARTESIAN_POINT('Ctrl Pts',(87.1865323817673,59.3889143995621,11.099741286753));
#69619=CARTESIAN_POINT('Ctrl Pts',(87.1639740662499,59.3919742167761,11.119688103195));
#69620=CARTESIAN_POINT('Ctrl Pts',(87.1582591960133,59.3927523402118,11.1248346210421));
#69621=CARTESIAN_POINT('Ctrl Pts',(87.1487970147668,59.3940451945232,11.1335127257806));
#69622=CARTESIAN_POINT('Ctrl Pts',(87.1450238936592,59.394561947883,11.137015666303));
#69623=CARTESIAN_POINT('Ctrl Pts',(87.1373318641946,59.3956177661504,11.1442444877149));
#69624=CARTESIAN_POINT('Ctrl Pts',(87.1334152742032,59.3961566506239,11.1479726098554));
#69625=CARTESIAN_POINT('Ctrl Pts',(87.1231090258598,59.3975785375933,11.1579091539092));
#69626=CARTESIAN_POINT('Ctrl Pts',(87.1167604782221,59.3984583751657,11.1641601799838));
#69627=CARTESIAN_POINT('Ctrl Pts',(87.0881157300684,59.4024497217391,11.1929648585689));
#69628=CARTESIAN_POINT('Ctrl Pts',(87.0666005671462,59.4055080814184,11.2162847546263));
#69629=CARTESIAN_POINT('Ctrl Pts',(87.001638542249,59.4150398291157,11.2922161011766));
#69630=CARTESIAN_POINT('Ctrl Pts',(86.9615420501439,59.4213830409135,11.3475351957514));
#69631=CARTESIAN_POINT('Ctrl Pts',(86.8929888236457,59.4337545119134,11.460192029403));
#69632=CARTESIAN_POINT('Ctrl Pts',(86.8640377282759,59.4397578093198,11.5169755367276));
#69633=CARTESIAN_POINT('Ctrl Pts',(86.8322438536021,59.4477144488283,11.5929418828067));
#69634=CARTESIAN_POINT('Ctrl Pts',(86.8254033875868,59.4495331718521,11.6103569144862));
#69635=CARTESIAN_POINT('Ctrl Pts',(86.8154051157657,59.4523707714907,11.6375627134683));
#69636=CARTESIAN_POINT('Ctrl Pts',(86.8119771344629,59.4533806799752,11.6472521184742));
#69637=CARTESIAN_POINT('Ctrl Pts',(86.8058339135177,59.455262312639,11.6653104693713));
#69638=CARTESIAN_POINT('Ctrl Pts',(86.803087287703,59.4561329437163,11.6736681690772));
#69639=CARTESIAN_POINT('Ctrl Pts',(86.7971702585409,59.458076390183,11.6923243891));
#69640=CARTESIAN_POINT('Ctrl Pts',(86.7940436972816,59.4591505661996,11.7026359369477));
#69641=CARTESIAN_POINT('Ctrl Pts',(86.7864256821505,59.4618939360299,11.7289623611367));
#69642=CARTESIAN_POINT('Ctrl Pts',(86.7821171183554,59.4635688562637,11.7450273751129));
#69643=CARTESIAN_POINT('Ctrl Pts',(86.7533768577916,59.4757006435426,11.8612669109769));
#69644=CARTESIAN_POINT('Ctrl Pts',(86.7409162936534,59.4865367345118,11.9639798325527));
#69645=CARTESIAN_POINT('Ctrl Pts',(86.74104864501,59.5036229477905,12.1261075805094));
#69646=CARTESIAN_POINT('Ctrl Pts',(86.7452181313658,59.5098257394367,12.1851125158358));
#69647=CARTESIAN_POINT('Ctrl Pts',(86.7548737243046,59.5168739471894,12.2534720238416));
#69648=CARTESIAN_POINT('Ctrl Pts',(86.7563809530928,59.5178845017504,12.2633069936988));
#69649=CARTESIAN_POINT('Ctrl Pts',(86.7589222007596,59.5194577196056,12.2786802835506));
#69650=CARTESIAN_POINT('Ctrl Pts',(86.759877689846,59.5200244169316,12.2842308134261));
#69651=CARTESIAN_POINT('Ctrl Pts',(86.7617584837041,59.521094468543,12.2947379595655));
#69652=CARTESIAN_POINT('Ctrl Pts',(86.7626763869126,59.5215981706109,12.2996954837547));
#69653=CARTESIAN_POINT('Ctrl Pts',(86.7649564113522,59.522806425434,12.3116128335686));
#69654=CARTESIAN_POINT('Ctrl Pts',(86.7663473512566,59.5235093656812,12.3185669841474));
#69655=CARTESIAN_POINT('Ctrl Pts',(86.7714737600949,59.525985557474,12.3431255119582));
#69656=CARTESIAN_POINT('Ctrl Pts',(86.7755253409287,59.5277424718368,12.3606630872153));
#69657=CARTESIAN_POINT('Ctrl Pts',(86.7836996735767,59.5309620891077,12.392904976564));
#69658=CARTESIAN_POINT('Ctrl Pts',(86.7877172404363,59.5324286298095,12.4076318202338));
#69659=CARTESIAN_POINT('Ctrl Pts',(86.8104630413104,59.540175427238,12.4854550706755));
#69660=CARTESIAN_POINT('Ctrl Pts',(86.8338108622215,59.5463051252134,12.5471017748254));
#69661=CARTESIAN_POINT('Ctrl Pts',(86.8931428388922,59.5593698738862,12.6732097604881));
#69662=CARTESIAN_POINT('Ctrl Pts',(86.9301660976612,59.5662934406023,12.7368975075675));
#69663=CARTESIAN_POINT('Ctrl Pts',(86.981612859275,59.5749595443459,12.8099849243284));
#69664=CARTESIAN_POINT('Ctrl Pts',(86.9909819323649,59.5765052960202,12.8227790570389));
#69665=CARTESIAN_POINT('Ctrl Pts',(87.0064547594228,59.5790099184621,12.8430988688454));
#69666=CARTESIAN_POINT('Ctrl Pts',(87.0124096649597,59.579962968376,12.8507363392715));
#69667=CARTESIAN_POINT('Ctrl Pts',(87.023999666922,59.5817979498255,12.8652555555867));
#69668=CARTESIAN_POINT('Ctrl Pts',(87.0296208830115,59.5826792864769,12.8721477030477));
#69669=CARTESIAN_POINT('Ctrl Pts',(87.0428342296356,59.5847317012978,12.8880055089261));
#69670=CARTESIAN_POINT('Ctrl Pts',(87.0504791555469,59.5859048749956,12.896925808437));
#69671=CARTESIAN_POINT('Ctrl Pts',(87.0758970956893,59.5897608126251,12.9257645922062));
#69672=CARTESIAN_POINT('Ctrl Pts',(87.0941730110331,59.59246413685,12.9452272714945));
#69673=CARTESIAN_POINT('Ctrl Pts',(87.1348137693455,59.5983384439217,12.9858614793107));
#69674=CARTESIAN_POINT('Ctrl Pts',(87.1573608824744,59.6015155117477,13.006822537074));
#69675=CARTESIAN_POINT('Ctrl Pts',(87.1806428411249,59.6047173123478,13.026940679077));
#69676=CARTESIAN_POINT('Ctrl Pts',(87.1806428354195,59.7737921350435,13.0269406741468));
#69677=CARTESIAN_POINT('Ctrl Pts',(87.1775687030115,59.7733820315304,13.0242842896909));
#69678=CARTESIAN_POINT('Ctrl Pts',(87.1745072481833,59.7729729306308,13.0216130936167));
#69679=CARTESIAN_POINT('Ctrl Pts',(87.1677366033509,59.7720667300509,13.015648066149));
#69680=CARTESIAN_POINT('Ctrl Pts',(87.1640338713773,59.7715701992528,13.0123471804472));
#69681=CARTESIAN_POINT('Ctrl Pts',(87.1557520415292,59.7704574349153,13.0048766044911));
#69682=CARTESIAN_POINT('Ctrl Pts',(87.1511839790451,59.7698420994443,13.0006950117345));
#69683=CARTESIAN_POINT('Ctrl Pts',(87.1373352292863,59.7679711011719,12.9878304525414));
#69684=CARTESIAN_POINT('Ctrl Pts',(87.1281536532909,59.7667229830059,12.9790410111749));
#69685=CARTESIAN_POINT('Ctrl Pts',(87.0695725790788,59.758696016311,12.9212516882754));
#69686=CARTESIAN_POINT('Ctrl Pts',(87.0241297518223,59.752167136254,12.8683913087438));
#69687=CARTESIAN_POINT('Ctrl Pts',(86.9350170653384,59.737951773346,12.7456318500562));
#69688=CARTESIAN_POINT('Ctrl Pts',(86.8933540033589,59.7302944763121,12.6746900289191));
#69689=CARTESIAN_POINT('Ctrl Pts',(86.8495629533283,59.7202723018389,12.5802462782872));
#69690=CARTESIAN_POINT('Ctrl Pts',(86.8408188455265,59.7181368831593,12.5600254818589));
#69691=CARTESIAN_POINT('Ctrl Pts',(86.8285309583209,59.714915887302,12.5294504889283));
#69692=CARTESIAN_POINT('Ctrl Pts',(86.8245875550023,59.7138436757156,12.5192602809311));
#69693=CARTESIAN_POINT('Ctrl Pts',(86.8177050436893,59.7118995292467,12.500769665071));
#69694=CARTESIAN_POINT('Ctrl Pts',(86.8147198025089,59.7110291884513,12.4924870380719));
#69695=CARTESIAN_POINT('Ctrl Pts',(86.8084770616258,59.7091486524475,12.4745850205568));
#69696=CARTESIAN_POINT('Ctrl Pts',(86.8052483833388,59.7081375738011,12.4649563383163));
#69697=CARTESIAN_POINT('Ctrl Pts',(86.7967309594642,59.7053604379232,12.4385071576622));
#69698=CARTESIAN_POINT('Ctrl Pts',(86.7916767389639,59.703586918852,12.4216143841025));
#69699=CARTESIAN_POINT('Ctrl Pts',(86.756373901532,59.6901824515533,12.2940048476749));
#69700=CARTESIAN_POINT('Ctrl Pts',(86.7409157376895,59.678069612099,12.1797740406136));
#69701=CARTESIAN_POINT('Ctrl Pts',(86.7410363465161,59.660868729895,12.0162530732113));
#69702=CARTESIAN_POINT('Ctrl Pts',(86.7438862449935,59.6557670195673,11.9674778025694));
#69703=CARTESIAN_POINT('Ctrl Pts',(86.7506721580243,59.6497842119694,11.9092529076282));
#69704=CARTESIAN_POINT('Ctrl Pts',(86.7519184841986,59.6487896291652,11.8995377573297));
#69705=CARTESIAN_POINT('Ctrl Pts',(86.7540536492045,59.6472357210878,11.8842936204428));
#69706=CARTESIAN_POINT('Ctrl Pts',(86.7548668196986,59.6466725152218,11.8787547732185));
#69707=CARTESIAN_POINT('Ctrl Pts',(86.7564835233413,59.6456049469763,11.8682275671591));
#69708=CARTESIAN_POINT('Ctrl Pts',(86.7572802040074,59.6451002669231,11.8632385626636));
#69709=CARTESIAN_POINT('Ctrl Pts',(86.759278313206,59.6438840597824,11.8511881761662));
#69710=CARTESIAN_POINT('Ctrl Pts',(86.760509749671,59.64317420222,11.844131922957));
#69711=CARTESIAN_POINT('Ctrl Pts',(86.7651321695339,59.6406435483792,11.8189070486074));
#69712=CARTESIAN_POINT('Ctrl Pts',(86.7688602124104,59.6388400565203,11.8008011043753));
#69713=CARTESIAN_POINT('Ctrl Pts',(86.7765198997636,59.6355174631427,11.7673187551984));
#69714=CARTESIAN_POINT('Ctrl Pts',(86.7803468330588,59.6339946413354,11.7519228633101));
#69715=CARTESIAN_POINT('Ctrl Pts',(86.8028102751746,59.6257271890354,11.668278576211));
#69716=CARTESIAN_POINT('Ctrl Pts',(86.8268373938344,59.6191528676266,11.6016020627902));
#69717=CARTESIAN_POINT('Ctrl Pts',(86.8844327363165,59.6061710091304,11.4758186262596));
#69718=CARTESIAN_POINT('Ctrl Pts',(86.9174258561234,59.5997896423517,11.4167227378667));
#69719=CARTESIAN_POINT('Ctrl Pts',(86.9636996266891,59.5917112425151,11.3474531604039));
#69720=CARTESIAN_POINT('Ctrl Pts',(86.972682846553,59.5901770833041,11.3345322501892));
#69721=CARTESIAN_POINT('Ctrl Pts',(86.9875628362294,59.5876867382795,11.313956353478));
#69722=CARTESIAN_POINT('Ctrl Pts',(86.9933112175547,59.5867362532257,11.306195549019));
#69723=CARTESIAN_POINT('Ctrl Pts',(87.0045257829804,59.5849032096789,11.2914105233264));
#69724=CARTESIAN_POINT('Ctrl Pts',(87.0099784208113,59.5840212230813,11.2843766926243));
#69725=CARTESIAN_POINT('Ctrl Pts',(87.0228323379905,59.5819627696884,11.2681504253961));
#69726=CARTESIAN_POINT('Ctrl Pts',(87.030288575361,59.5807841655702,11.2590028814561));
#69727=CARTESIAN_POINT('Ctrl Pts',(87.055239165879,59.5768887855074,11.2292492239817));
#69728=CARTESIAN_POINT('Ctrl Pts',(87.0732624626855,59.5741508529629,11.2090993866752));
#69729=CARTESIAN_POINT('Ctrl Pts',(87.1188993892084,59.5673893805207,11.16124280233));
#69730=CARTESIAN_POINT('Ctrl Pts',(87.1471749435473,59.5633411989541,11.1342089011216));
#69731=CARTESIAN_POINT('Ctrl Pts',(87.2125730646819,59.5542790536115,11.0772204776791));
#69732=CARTESIAN_POINT('Ctrl Pts',(87.2502285805024,59.5492537564951,11.0479642152911));
#69733=CARTESIAN_POINT('Ctrl Pts',(87.3403632700887,59.5377075891573,10.9857332504184));
#69734=CARTESIAN_POINT('Ctrl Pts',(87.393800342804,59.5312012305805,10.9543360147804));
#69735=CARTESIAN_POINT('Ctrl Pts',(87.4582878093801,59.5238600275004,10.9225363287019));
#69736=CARTESIAN_POINT('Ctrl Pts',(87.4673060571095,59.5228445478086,10.9182209043483));
#69737=CARTESIAN_POINT('Ctrl Pts',(87.4814920068698,59.5212654747772,10.9116373574472));
#69738=CARTESIAN_POINT('Ctrl Pts',(87.4866251352479,59.5206977990061,10.9092965673608));
#69739=CARTESIAN_POINT('Ctrl Pts',(87.4963708534544,59.5196272218521,10.9049305727487));
#69740=CARTESIAN_POINT('Ctrl Pts',(87.5009799484567,59.5191239630705,10.9028985760763));
#69741=CARTESIAN_POINT('Ctrl Pts',(87.5120843617653,59.5179185803153,10.8980817131152));
#69742=CARTESIAN_POINT('Ctrl Pts',(87.5185910786153,59.5172180497405,10.8953235281889));
#69743=CARTESIAN_POINT('Ctrl Pts',(87.541600773772,59.514759797852,10.8857955575515));
#69744=CARTESIAN_POINT('Ctrl Pts',(87.5582242388993,59.5130181046345,10.8793187512209));
#69745=CARTESIAN_POINT('Ctrl Pts',(87.5891348776697,59.509831792911,10.8680196385438));
#69746=CARTESIAN_POINT('Ctrl Pts',(87.6033814241371,59.5083833059317,10.8630975608054));
#69747=CARTESIAN_POINT('Ctrl Pts',(87.6788702439027,59.5007954455854,10.8385120148546));
#69748=CARTESIAN_POINT('Ctrl Pts',(87.7414580836853,59.4948008291481,10.8232668530131));
#69749=CARTESIAN_POINT('Ctrl Pts',(87.8794203547817,59.481697196394,10.8005812642215));
#69750=CARTESIAN_POINT('Ctrl Pts',(87.9548344247613,59.4745971736984,10.7950003455266));
#69751=CARTESIAN_POINT('Ctrl Pts',(88.0461250336752,59.4657444414998,10.7963870382767));
#69752=CARTESIAN_POINT('Ctrl Pts',(88.0619543923873,59.4642005431782,10.7969237859735));
#69753=CARTESIAN_POINT('Ctrl Pts',(88.0874346192412,59.4616983127024,10.7982652339914));
#69754=CARTESIAN_POINT('Ctrl Pts',(88.0970940138646,59.4607457828876,10.7988845767473));
#69755=CARTESIAN_POINT('Ctrl Pts',(88.1156127389095,59.4589114030595,10.8002846844128));
#69756=CARTESIAN_POINT('Ctrl Pts',(88.1244728400448,59.458030144622,10.801048226379));
#69757=CARTESIAN_POINT('Ctrl Pts',(88.1450221050418,59.4559773183308,10.8030367366401));
#69758=CARTESIAN_POINT('Ctrl Pts',(88.1567035038372,59.4548036502318,10.804331028232));
#69759=CARTESIAN_POINT('Ctrl Pts',(88.1948916107426,59.4509433336054,10.8090996374006));
#69760=CARTESIAN_POINT('Ctrl Pts',(88.221304558554,59.4482360558747,10.8132484825475));
#69761=CARTESIAN_POINT('Ctrl Pts',(88.2853771750694,59.4415699687114,10.8253959713326));
#69762=CARTESIAN_POINT('Ctrl Pts',(88.3228397922843,59.4375874521361,10.8342790673587));
#69763=CARTESIAN_POINT('Ctrl Pts',(88.4063179390522,59.4285216584483,10.8581256356881));
#69764=CARTESIAN_POINT('Ctrl Pts',(88.4520000035814,59.4234241038386,10.8740456358033));
#69765=CARTESIAN_POINT('Ctrl Pts',(88.5541526719112,59.4117695876333,10.9163232318382));
#69766=CARTESIAN_POINT('Ctrl Pts',(88.609827460965,59.4052270005217,10.9443139702107));
#69767=CARTESIAN_POINT('Ctrl Pts',(88.6718193091844,59.397850350359,10.9814180615258));
#69768=CARTESIAN_POINT('Ctrl Pts',(88.680345274137,59.3968338019355,10.9866589661164));
#69769=CARTESIAN_POINT('Ctrl Pts',(88.6935814950587,59.3952534427346,10.9950124403596));
#69770=CARTESIAN_POINT('Ctrl Pts',(88.6983341598425,59.3946855390946,10.9980563649833));
#69771=CARTESIAN_POINT('Ctrl Pts',(88.7072895256839,59.3936148035626,11.0038765313924));
#69772=CARTESIAN_POINT('Ctrl Pts',(88.7114960576605,59.393111612259,11.006646120843));
#69773=CARTESIAN_POINT('Ctrl Pts',(88.7215614239542,59.3919067586762,11.0133593512951));
#69774=CARTESIAN_POINT('Ctrl Pts',(88.727404064009,59.391206686065,11.0173269822442));
#69775=CARTESIAN_POINT('Ctrl Pts',(88.7478600191035,59.3887519410587,11.0314690140069));
#69776=CARTESIAN_POINT('Ctrl Pts',(88.7622932610998,59.3870132362549,11.0419025434653));
#69777=CARTESIAN_POINT('Ctrl Pts',(88.7884987538707,59.3838334695196,11.061698412505));
#69778=CARTESIAN_POINT('Ctrl Pts',(88.8003328145283,59.3823885331565,11.0709724867041));
#69779=CARTESIAN_POINT('Ctrl Pts',(88.8616875060043,59.3748315847663,11.120838414535));
#69780=CARTESIAN_POINT('Ctrl Pts',(88.9082546248101,59.3688632113717,11.1649254331858));
#69781=CARTESIAN_POINT('Ctrl Pts',(88.9980166167357,59.3563481608872,11.2637978184337));
#69782=CARTESIAN_POINT('Ctrl Pts',(89.040422579967,59.3498147227811,11.3189946510523));
#69783=CARTESIAN_POINT('Ctrl Pts',(89.087564994343,59.3414208424022,11.3920469826745));
#69784=CARTESIAN_POINT('Ctrl Pts',(89.0967281837991,59.3397255835919,11.4069104020161));
#69785=CARTESIAN_POINT('Ctrl Pts',(89.1111676166378,59.3369428867795,11.4314509077059));
#69786=CARTESIAN_POINT('Ctrl Pts',(89.1166296901801,59.3358621556153,11.4410165564696));
#69787=CARTESIAN_POINT('Ctrl Pts',(89.1262354061474,59.3339089075042,11.4583589749287));
#69788=CARTESIAN_POINT('Ctrl Pts',(89.1304239095464,59.3330380519393,11.4661102373577));
#69789=CARTESIAN_POINT('Ctrl Pts',(89.1392363104646,59.3311634455286,11.4828322075904));
#69790=CARTESIAN_POINT('Ctrl Pts',(89.1438345620471,59.3301588624505,11.4918156338765));
#69791=CARTESIAN_POINT('Ctrl Pts',(89.1562502987068,59.3273708348178,11.5168015549994));
#69792=CARTESIAN_POINT('Ctrl Pts',(89.1638385967034,59.3255796512824,11.5329143915446));
#69793=CARTESIAN_POINT('Ctrl Pts',(89.1801091563551,59.321532010175,11.5694362941811));
#69794=CARTESIAN_POINT('Ctrl Pts',(89.188600382898,59.3192698564289,11.589923408886));
#69795=CARTESIAN_POINT('Ctrl Pts',(89.2151772370692,59.3116537690743,11.6591145272864));
#69796=CARTESIAN_POINT('Ctrl Pts',(89.2308086071154,59.3062320730919,11.7086987779864));
#69797=CARTESIAN_POINT('Ctrl Pts',(89.2635481026253,59.2919834056348,11.8401619153047));
#69798=CARTESIAN_POINT('Ctrl Pts',(89.2756903839064,59.2831146054344,11.9230303097981));
#69799=CARTESIAN_POINT('Ctrl Pts',(89.2801702207618,59.273299975523,12.0185413451439));
#69800=CARTESIAN_POINT('Ctrl Pts',(89.2805636191433,59.2720692182234,12.0305933997062));
#69801=CARTESIAN_POINT('Ctrl Pts',(89.2808980580573,59.2702251665408,12.0487803525101));
#69802=CARTESIAN_POINT('Ctrl Pts',(89.280966396804,59.2696057476745,12.0549116860172));
#69803=CARTESIAN_POINT('Ctrl Pts',(89.2810099256633,59.2684833635755,12.0660649661424));
#69804=CARTESIAN_POINT('Ctrl Pts',(89.2809997423851,59.2679796322227,12.0710867029397));
#69805=CARTESIAN_POINT('Ctrl Pts',(89.2809157406367,59.2669245590828,12.0816400660853));
#69806=CARTESIAN_POINT('Ctrl Pts',(89.2808355694342,59.2663735691534,12.0871714643996));
#69807=CARTESIAN_POINT('Ctrl Pts',(89.2805197944581,59.2648828748999,12.1021868266455));
#69808=CARTESIAN_POINT('Ctrl Pts',(89.2802140604217,59.2639468987511,12.1116692846327));
#69809=CARTESIAN_POINT('Ctrl Pts',(89.277819126275,59.2585346990348,12.1667701124972));
#69810=CARTESIAN_POINT('Ctrl Pts',(89.2733766094805,59.2541721118022,12.2122602170451));
#69811=CARTESIAN_POINT('Ctrl Pts',(89.2524073825708,59.2410214654827,12.3497942815233));
#69812=CARTESIAN_POINT('Ctrl Pts',(89.2281723648696,59.232398921879,12.4403300246576));
#69813=CARTESIAN_POINT('Ctrl Pts',(89.1818046795263,59.2202430267664,12.559239471477));
#69814=CARTESIAN_POINT('Ctrl Pts',(89.1681047975308,59.2169578471152,12.5905729689641));
#69815=CARTESIAN_POINT('Ctrl Pts',(89.1474000411343,59.2123485878971,12.6331582022505));
#69816=CARTESIAN_POINT('Ctrl Pts',(89.1414572346811,59.2110606237555,12.6449126782262));
#69817=CARTESIAN_POINT('Ctrl Pts',(89.1315100541561,59.2089583917186,12.6638501513143));
#69818=CARTESIAN_POINT('Ctrl Pts',(89.1276166807497,59.2081480457571,12.6710907082465));
#69819=CARTESIAN_POINT('Ctrl Pts',(89.1192805777984,59.2064383664324,12.6862390067684));
#69820=CARTESIAN_POINT('Ctrl Pts',(89.1148229022142,59.2055385407913,12.6941379261746));
#69821=CARTESIAN_POINT('Ctrl Pts',(89.1038558267501,59.2033583100933,12.7130940954957));
#69822=CARTESIAN_POINT('Ctrl Pts',(89.0972628793226,59.2020749591309,12.7241014757712));
#69823=CARTESIAN_POINT('Ctrl Pts',(89.0725642201419,59.1973625527552,12.7639550697698));
#69824=CARTESIAN_POINT('Ctrl Pts',(89.0534689672233,59.1938980280824,12.7921664894641));
#69825=CARTESIAN_POINT('Ctrl Pts',(88.9895394103307,59.1828143381107,12.8788905984753));
#69826=CARTESIAN_POINT('Ctrl Pts',(88.9407398803989,59.1750647491252,12.9342804660689));
#69827=CARTESIAN_POINT('Ctrl Pts',(88.8435584940192,59.1609069904611,13.0269475010758));
#69828=CARTESIAN_POINT('Ctrl Pts',(88.7967490268963,59.1545248419355,13.0655869873199));
#69829=CARTESIAN_POINT('Ctrl Pts',(88.7368477457672,59.1469831778354,13.1082146060289));
#69830=CARTESIAN_POINT('Ctrl Pts',(88.72622895842,59.1456685513683,13.1155302846455));
#69831=CARTESIAN_POINT('Ctrl Pts',(88.7103180724264,59.1437333941151,13.1261382078961));
#69832=CARTESIAN_POINT('Ctrl Pts',(88.705110734582,59.1431054469085,13.1295549258966));
#69833=CARTESIAN_POINT('Ctrl Pts',(88.6957111152456,59.1419818734538,13.1356239026172));
#69834=CARTESIAN_POINT('Ctrl Pts',(88.6915282389876,59.1414853869444,13.1382900370571));
#69835=CARTESIAN_POINT('Ctrl Pts',(88.6820680105997,59.1403703359417,13.1442422586879));
#69836=CARTESIAN_POINT('Ctrl Pts',(88.6767820167762,59.1397526888371,13.1475141956512));
#69837=CARTESIAN_POINT('Ctrl Pts',(88.6605110417331,59.1378672264789,13.1574211328747));
#69838=CARTESIAN_POINT('Ctrl Pts',(88.6494487797031,59.1366071260384,13.1639289069564));
#69839=CARTESIAN_POINT('Ctrl Pts',(88.6230193045955,59.133642687993,13.178942394603));
#69840=CARTESIAN_POINT('Ctrl Pts',(88.6075701675413,59.1319459993446,13.1872994838511));
#69841=CARTESIAN_POINT('Ctrl Pts',(88.5479360131498,59.125512727448,13.2179764575562));
#69842=CARTESIAN_POINT('Ctrl Pts',(88.5026296342627,59.1208627709275,13.2380287485289));
#69843=CARTESIAN_POINT('Ctrl Pts',(88.3725590638776,59.1078441305012,13.2867225186989));
#69844=CARTESIAN_POINT('Ctrl Pts',(88.285792999167,59.0995178121364,13.3091306915422));
#69845=CARTESIAN_POINT('Ctrl Pts',(88.1804787445415,59.0892344098652,13.3247571779809));
#69846=CARTESIAN_POINT('Ctrl Pts',(88.1635081609346,59.0875727726781,13.3269258001105));
#69847=CARTESIAN_POINT('Ctrl Pts',(88.1356491520638,59.0848338771964,13.3299152198127));
#69848=CARTESIAN_POINT('Ctrl Pts',(88.1247842935386,59.0837629691797,13.3309396073695));
#69849=CARTESIAN_POINT('Ctrl Pts',(88.1051336008588,59.0818202065573,13.3325371546034));
#69850=CARTESIAN_POINT('Ctrl Pts',(88.0963523141284,59.0809499357357,13.3331592131248));
#69851=CARTESIAN_POINT('Ctrl Pts',(88.0774183424928,59.07906844936,13.3343027813302));
#69852=CARTESIAN_POINT('Ctrl Pts',(88.0672645337648,59.0780563423113,13.3347937689663));
#69853=CARTESIAN_POINT('Ctrl Pts',(88.0389510199128,59.0752246188918,13.3358223456954));
#69854=CARTESIAN_POINT('Ctrl Pts',(88.0207849372825,59.0733968551869,13.3360922078435));
#69855=CARTESIAN_POINT('Ctrl Pts',(87.9902541179674,59.0703045886684,13.3358907599685));
#69856=CARTESIAN_POINT('Ctrl Pts',(87.9778901498451,59.0690466993831,13.3356285460765));
#69857=CARTESIAN_POINT('Ctrl Pts',(87.928558390022,59.0640043542464,13.3338612783503));
#69858=CARTESIAN_POINT('Ctrl Pts',(87.8916642327907,59.0601800178747,13.3309218166989));
#69859=CARTESIAN_POINT('Ctrl Pts',(87.8050826073693,59.0510798606278,13.3202022977591));
#69860=CARTESIAN_POINT('Ctrl Pts',(87.7556238678647,59.0457817207991,13.3110733917178));
#69861=CARTESIAN_POINT('Ctrl Pts',(87.6504357810763,59.0343602010464,13.2851260876271));
#69862=CARTESIAN_POINT('Ctrl Pts',(87.5950454516706,59.0282489514472,13.2673569744814));
#69863=CARTESIAN_POINT('Ctrl Pts',(87.5290886683098,59.0209663168652,13.2410861765387));
#69864=CARTESIAN_POINT('Ctrl Pts',(87.5171895707621,59.0196524175389,13.2361356161176));
#69865=CARTESIAN_POINT('Ctrl Pts',(87.4996553280921,59.0177181155823,13.2285254389165));
#69866=CARTESIAN_POINT('Ctrl Pts',(87.4939616586705,59.0170903056412,13.2260043660288));
#69867=CARTESIAN_POINT('Ctrl Pts',(87.4837658884295,59.0159668702914,13.2213998424652));
#69868=CARTESIAN_POINT('Ctrl Pts',(87.479257239905,59.0154703857178,13.2193318016494));
#69869=CARTESIAN_POINT('Ctrl Pts',(87.4747189595692,59.0149709276236,13.2172178976095));
#69870=CARTESIAN_POINT('Ctrl Pts',(87.4746774000621,59.014966353836,13.217198536699));
#69871=CARTESIAN_POINT('Ctrl Pts',(87.4745975007062,59.0149575606398,13.217161309522));
#69872=CARTESIAN_POINT('Ctrl Pts',(87.4745591608392,59.0149533412259,13.2171434436549));
#69873=CARTESIAN_POINT('Ctrl Pts',(87.4744854462499,59.0149452287573,13.217109089156));
#69874=CARTESIAN_POINT('Ctrl Pts',(87.4744500713418,59.0149413356793,13.2170926007842));
#69875=CARTESIAN_POINT('Ctrl Pts',(87.4743603401096,59.0149314606222,13.2170507716993));
#69876=CARTESIAN_POINT('Ctrl Pts',(87.474305984671,59.0149254787623,13.2170254286968));
#69877=CARTESIAN_POINT('Ctrl Pts',(87.4741981788308,59.0149136147174,13.2169751553652));
#69878=CARTESIAN_POINT('Ctrl Pts',(87.474144728382,59.0149077325259,13.2169502251681));
#69879=CARTESIAN_POINT('Ctrl Pts',(87.4740387115215,59.0148960655027,13.2169007681118));
#69880=CARTESIAN_POINT('Ctrl Pts',(87.4739861451921,59.0148902806789,13.2168762414391));
#69881=CARTESIAN_POINT('Ctrl Pts',(87.4738818762983,59.0148788061562,13.2168275824148));
#69882=CARTESIAN_POINT('Ctrl Pts',(87.4738301737658,59.0148731164596,13.2168034502203));
#69883=CARTESIAN_POINT('Ctrl Pts',(87.473727613119,59.0148618300587,13.2167555715466));
#69884=CARTESIAN_POINT('Ctrl Pts',(87.4736767548182,59.0148562333327,13.2167318251173));
#69885=CARTESIAN_POINT('Ctrl Pts',(87.4735758629358,59.0148451307014,13.2166847091842));
#69886=CARTESIAN_POINT('Ctrl Pts',(87.4735258294574,59.0148396248064,13.2166613398602));
#69887=CARTESIAN_POINT('Ctrl Pts',(87.4734265689441,59.0148287018227,13.2166149699944));
#69888=CARTESIAN_POINT('Ctrl Pts',(87.4733773417245,59.0148232847127,13.2165919694927));
#69889=CARTESIAN_POINT('Ctrl Pts',(87.4732796753336,59.0148125372712,13.216546329054));
#69890=CARTESIAN_POINT('Ctrl Pts',(87.4732312361289,59.0148072069352,13.2165236892231));
#69891=CARTESIAN_POINT('Ctrl Pts',(87.4674760496392,59.0141738994355,13.2138333498241));
#69892=CARTESIAN_POINT('Ctrl Pts',(87.4617890066033,59.0135484914819,13.2111231263483));
#69893=CARTESIAN_POINT('Ctrl Pts',(87.4436846533991,59.0115580331591,13.202329390986));
#69894=CARTESIAN_POINT('Ctrl Pts',(87.431345719996,59.0102021865128,13.1960850233949));
#69895=CARTESIAN_POINT('Ctrl Pts',(87.4017719098353,59.0069479368493,13.1805066937269));
#69896=CARTESIAN_POINT('Ctrl Pts',(87.3846457807235,59.0050595671684,13.1709726483241));
#69897=CARTESIAN_POINT('Ctrl Pts',(87.3154370641298,58.9973820615851,13.1303178940989));
#69898=CARTESIAN_POINT('Ctrl Pts',(87.2653919453477,58.9917178198013,13.0958788629775));
#69899=CARTESIAN_POINT('Ctrl Pts',(87.2053439521476,58.9845156109244,13.0478761243235));
#69900=CARTESIAN_POINT('Ctrl Pts',(87.1928905788101,58.9829980406649,13.0375240568162));
#69901=CARTESIAN_POINT('Ctrl Pts',(87.1806427698475,58.9814779498304,13.0269406174854));
#69902=CARTESIAN_POINT('Origin',(88.011,66.41344859951,12.066));
#69903=CARTESIAN_POINT('',(87.1795113209163,58.0179748583214,13.028265366586));
#69904=CARTESIAN_POINT('',(87.1806428261678,58.1885986874538,13.0269406661524));
#69905=CARTESIAN_POINT('',(87.1806428354228,66.41344859951,13.0269406741497));
#69906=CARTESIAN_POINT('',(86.7429300722972,58.7031861779361,12.066150707506));
#69907=CARTESIAN_POINT('Ctrl Pts',(86.7430439769444,58.70325140049,12.0661441982405));
#69908=CARTESIAN_POINT('Ctrl Pts',(86.7432677167238,58.6813761345907,11.8453854404656));
#69909=CARTESIAN_POINT('Ctrl Pts',(86.9032087774569,58.6174961205304,11.200423640207));
#69910=CARTESIAN_POINT('Ctrl Pts',(87.9302701790554,58.5116113583089,10.567102535751));
#69911=CARTESIAN_POINT('Ctrl Pts',(89.2264677377329,58.3855971138258,11.1851770377356));
#69912=CARTESIAN_POINT('Ctrl Pts',(89.4102662159187,58.2595828693425,12.6093828938329));
#69913=CARTESIAN_POINT('Ctrl Pts',(88.3436856703656,58.1370421175078,13.5107340312985));
#69914=CARTESIAN_POINT('Ctrl Pts',(87.4731169939088,58.056506113834,13.2786948377731));
#69915=CARTESIAN_POINT('Ctrl Pts',(87.1795113209163,58.0179748583214,13.028265366586));
#69916=CARTESIAN_POINT('Ctrl Pts',(86.7410000268199,58.7020810211383,12.06626100308));
#69917=CARTESIAN_POINT('Ctrl Pts',(86.7410018040281,58.702942207406,12.074908618816));
#69918=CARTESIAN_POINT('Ctrl Pts',(86.7410919053835,58.703806135607,12.0835557449932));
#69919=CARTESIAN_POINT('Ctrl Pts',(86.7415580182283,58.7060706472586,12.1061440589256));
#69920=CARTESIAN_POINT('Ctrl Pts',(86.7420753634555,58.707475518576,12.1200806591847));
#69921=CARTESIAN_POINT('Ctrl Pts',(86.746768418057,58.7163494988146,12.2075978878099));
#69922=CARTESIAN_POINT('Ctrl Pts',(86.7571121162255,58.7240041119405,12.280690462698));
#69923=CARTESIAN_POINT('Ctrl Pts',(86.7891895874481,58.7389602834226,12.4192392532306));
#69924=CARTESIAN_POINT('Ctrl Pts',(86.8100325125482,58.7462237510326,12.4846604536736));
#69925=CARTESIAN_POINT('Ctrl Pts',(86.8454095501306,58.7559058844029,12.5708824252684));
#69926=CARTESIAN_POINT('Ctrl Pts',(86.8554272387554,58.7584451220267,12.5934080250685));
#69927=CARTESIAN_POINT('Ctrl Pts',(86.8695357928023,58.7617597370289,12.6227967860943));
#69928=CARTESIAN_POINT('Ctrl Pts',(86.8730436278863,58.7625645312254,12.6299312940433));
#69929=CARTESIAN_POINT('Ctrl Pts',(86.8789567462526,58.7638892888397,12.6416779636251));
#69930=CARTESIAN_POINT('Ctrl Pts',(86.8813237029761,58.7644114831957,12.646308981877));
#69931=CARTESIAN_POINT('Ctrl Pts',(86.8861759776172,58.7654656107405,12.6556603884779));
#69932=CARTESIAN_POINT('Ctrl Pts',(86.8886627078911,58.7659974467432,12.6603798968008));
#69933=CARTESIAN_POINT('Ctrl Pts',(86.8952239367357,58.7673794680054,12.6726442930866));
#69934=CARTESIAN_POINT('Ctrl Pts',(86.8993453542373,58.7682267976695,12.6801640539018));
#69935=CARTESIAN_POINT('Ctrl Pts',(86.9172956736287,58.771832675551,12.7121426107563));
#69936=CARTESIAN_POINT('Ctrl Pts',(86.9318595553397,58.7745498882907,12.7361833539785));
#69937=CARTESIAN_POINT('Ctrl Pts',(87.0016234939353,58.786770857829,12.8431626629664));
#69938=CARTESIAN_POINT('Ctrl Pts',(87.0656672784881,58.7959285372272,12.9199158702169));
#69939=CARTESIAN_POINT('Ctrl Pts',(87.1519442992313,58.8071691545005,13.001569548852));
#69940=CARTESIAN_POINT('Ctrl Pts',(87.1661526887944,58.8089892234156,13.0144196134261));
#69941=CARTESIAN_POINT('Ctrl Pts',(87.1806428565926,58.8108193550848,13.0269406924427));
#69942=CARTESIAN_POINT('',(86.7410003988283,58.8721740503657,12.0670064908467));
#69943=CARTESIAN_POINT('Ctrl Pts',(87.1806427698475,58.9814779498304,13.0269406174854));
#69944=CARTESIAN_POINT('Ctrl Pts',(87.1370767857196,58.9760709212452,12.9892948678408));
#69945=CARTESIAN_POINT('Ctrl Pts',(87.0961118985498,58.9706283137381,12.9487219918335));
#69946=CARTESIAN_POINT('Ctrl Pts',(87.046488376277,58.9633806464135,12.8923911806852));
#69947=CARTESIAN_POINT('Ctrl Pts',(87.0352153516528,58.9616848434087,12.8790493874646));
#69948=CARTESIAN_POINT('Ctrl Pts',(87.0172863890674,58.9589014380845,12.8569201167021));
#69949=CARTESIAN_POINT('Ctrl Pts',(87.0104630860139,58.9578205484458,12.848270564808));
#69950=CARTESIAN_POINT('Ctrl Pts',(86.998386982045,58.9558671301214,12.8325458268004));
#69951=CARTESIAN_POINT('Ctrl Pts',(86.9930935744683,58.954996264069,12.8255025527875));
#69952=CARTESIAN_POINT('Ctrl Pts',(86.9818958327033,58.9531217634808,12.8102757795346));
#69953=CARTESIAN_POINT('Ctrl Pts',(86.9760149465933,58.9521172976422,12.8020759113662));
#69954=CARTESIAN_POINT('Ctrl Pts',(86.964170595174,58.9500520129862,12.7851384369864));
#69955=CARTESIAN_POINT('Ctrl Pts',(86.9582173669713,58.9489909004524,12.7763946822364));
#69956=CARTESIAN_POINT('Ctrl Pts',(86.9276630636191,58.943420692495,12.7302906495264));
#69957=CARTESIAN_POINT('Ctrl Pts',(86.904943165941,58.9388443760581,12.6917300161594));
#69958=CARTESIAN_POINT('Ctrl Pts',(86.8627625679972,58.9293682023556,12.610637976312));
#69959=CARTESIAN_POINT('Ctrl Pts',(86.8435204478985,58.9244698166207,12.5680661457923));
#69960=CARTESIAN_POINT('Ctrl Pts',(86.8057233730358,58.9134398154253,12.4704416824064));
#69961=CARTESIAN_POINT('Ctrl Pts',(86.7885092840389,58.9073082070982,12.4149729282886));
#69962=CARTESIAN_POINT('Ctrl Pts',(86.7695260317669,58.8987446860058,12.3347711262844));
#69963=CARTESIAN_POINT('Ctrl Pts',(86.7645901871672,58.896229604006,12.3108639874167));
#69964=CARTESIAN_POINT('Ctrl Pts',(86.758925072365,58.8929152561057,12.278779590411));
#69965=CARTESIAN_POINT('Ctrl Pts',(86.7575817969577,58.8920876253673,12.2707183422853));
#69966=CARTESIAN_POINT('Ctrl Pts',(86.7555844325409,58.8907877905039,12.2579742130376));
#69967=CARTESIAN_POINT('Ctrl Pts',(86.7548785547574,58.8903128530538,12.2532999279555));
#69968=CARTESIAN_POINT('Ctrl Pts',(86.7535263231813,58.8893710399795,12.2439938783842));
#69969=CARTESIAN_POINT('Ctrl Pts',(86.7528794396254,58.888904167553,12.2393624123626));
#69970=CARTESIAN_POINT('Ctrl Pts',(86.7515738464782,58.8879260168383,12.2296224062515));
#69971=CARTESIAN_POINT('Ctrl Pts',(86.7509206057112,58.8874150485045,12.2245132532131));
#69972=CARTESIAN_POINT('Ctrl Pts',(86.7494288906419,58.8861937344408,12.2122537603548));
#69973=CARTESIAN_POINT('Ctrl Pts',(86.7486200793685,58.8854849261736,12.2050998591358));
#69974=CARTESIAN_POINT('Ctrl Pts',(86.7433293527182,58.8804911841479,12.1544487596178));
#69975=CARTESIAN_POINT('Ctrl Pts',(86.7410350631278,58.8763112249515,12.1107462294122));
#69976=CARTESIAN_POINT('Ctrl Pts',(86.7410003988283,58.8721740503657,12.0670064908467));
#69977=CARTESIAN_POINT('Ctrl Pts',(86.7410004001107,58.8721742032935,12.0670081076555));
#69978=CARTESIAN_POINT('Ctrl Pts',(86.7409117877615,58.8616153025445,11.9553755380898));
#69979=CARTESIAN_POINT('Ctrl Pts',(86.7555409402393,58.8513590986153,11.8442192881856));
#69980=CARTESIAN_POINT('Ctrl Pts',(86.788652066914,58.8390852970701,11.7210078015403));
#69981=CARTESIAN_POINT('Ctrl Pts',(86.7930781763349,58.8375441668072,11.7056939255015));
#69982=CARTESIAN_POINT('Ctrl Pts',(86.8008723323203,58.8349809045229,11.6805137991907));
#69983=CARTESIAN_POINT('Ctrl Pts',(86.8040758469691,58.8339639243966,11.6705981075384));
#69984=CARTESIAN_POINT('Ctrl Pts',(86.8105862816504,58.8319650394509,11.651263284215));
#69985=CARTESIAN_POINT('Ctrl Pts',(86.8138829697394,58.8309835284974,11.6418414914347));
#69986=CARTESIAN_POINT('Ctrl Pts',(86.8203028284725,58.8291272884535,11.6241650474497));
#69987=CARTESIAN_POINT('Ctrl Pts',(86.8234016777888,58.8282534141291,11.6159021276743));
#69988=CARTESIAN_POINT('Ctrl Pts',(86.830621571191,58.8262656671969,11.5972444221609));
#69989=CARTESIAN_POINT('Ctrl Pts',(86.834794226551,58.8251501267197,11.5868705969163));
#69990=CARTESIAN_POINT('Ctrl Pts',(86.8460551654791,58.8222226105092,11.5599081757565));
#69991=CARTESIAN_POINT('Ctrl Pts',(86.8533605720975,58.820403489325,11.5434138620995));
#69992=CARTESIAN_POINT('Ctrl Pts',(86.9039389873504,58.8083048477157,11.4354856982928));
#69993=CARTESIAN_POINT('Ctrl Pts',(86.9576436566689,58.7976670723019,11.3493670463497));
#69994=CARTESIAN_POINT('Ctrl Pts',(87.0459893537253,58.7828032407126,11.239410576555));
#69995=CARTESIAN_POINT('Ctrl Pts',(87.0724658980973,58.7786048267982,11.2094663575879));
#69996=CARTESIAN_POINT('Ctrl Pts',(87.1111100452255,58.7728541027258,11.1697087077035));
#69997=CARTESIAN_POINT('Ctrl Pts',(87.1221111980039,58.7712559615836,11.1587972806687));
#69998=CARTESIAN_POINT('Ctrl Pts',(87.1393460502387,58.7688143821583,11.1423176212434));
#69999=CARTESIAN_POINT('Ctrl Pts',(87.1454391614459,58.7679627251687,11.1366054700783));
#70000=CARTESIAN_POINT('Ctrl Pts',(87.1565861965223,58.766426000806,11.1263601062111));
#70001=CARTESIAN_POINT('Ctrl Pts',(87.1616208960014,58.7657396245582,11.1218065755442));
#70002=CARTESIAN_POINT('Ctrl Pts',(87.1703544593622,58.7645624953415,11.1140340806524));
#70003=CARTESIAN_POINT('Ctrl Pts',(87.1740358354661,58.7640703743801,11.1107958188212));
#70004=CARTESIAN_POINT('Ctrl Pts',(87.1812876699972,58.763109024542,11.1044909785051));
#70005=CARTESIAN_POINT('Ctrl Pts',(87.1848565589396,58.7626396705554,11.1014228043025));
#70006=CARTESIAN_POINT('Ctrl Pts',(87.1945858387831,58.7613700223425,11.0931521547797));
#70007=CARTESIAN_POINT('Ctrl Pts',(87.2007790360743,58.7605724558272,11.0879882338703));
#70008=CARTESIAN_POINT('Ctrl Pts',(87.2252140227933,58.7574649368521,11.0680056508454));
#70009=CARTESIAN_POINT('Ctrl Pts',(87.2438182685265,58.7551834181135,11.0536340776646));
#70010=CARTESIAN_POINT('Ctrl Pts',(87.3471877401853,58.7428863943113,10.9782699792461));
#70011=CARTESIAN_POINT('Ctrl Pts',(87.4388353139457,58.7333041414434,10.9273885918752));
#70012=CARTESIAN_POINT('Ctrl Pts',(87.5783697371137,58.7190710324237,10.8710734169435));
#70013=CARTESIAN_POINT('Ctrl Pts',(87.6219507121271,58.7146756262845,10.8561826098825));
#70014=CARTESIAN_POINT('Ctrl Pts',(87.6798584196734,58.7088278358892,10.839849312189));
#70015=CARTESIAN_POINT('Ctrl Pts',(87.6935407575736,58.7074457508682,10.8362358574955));
#70016=CARTESIAN_POINT('Ctrl Pts',(87.7163370649298,58.7051404629563,10.8306212071289));
#70017=CARTESIAN_POINT('Ctrl Pts',(87.7254181552078,58.7042214644977,10.8284904018527));
#70018=CARTESIAN_POINT('Ctrl Pts',(87.743262549955,58.7024137538193,10.8245102242282));
#70019=CARTESIAN_POINT('Ctrl Pts',(87.7520235928515,58.7015253453244,10.8226531394818));
#70020=CARTESIAN_POINT('Ctrl Pts',(87.7732504249262,58.6993701950009,10.818387749608));
#70021=CARTESIAN_POINT('Ctrl Pts',(87.7857337963603,58.698100555286,10.8160734840956));
#70022=CARTESIAN_POINT('Ctrl Pts',(87.8286137385708,58.6937300750784,10.8087872579349));
#70023=CARTESIAN_POINT('Ctrl Pts',(87.8591523925783,58.6906011732947,10.8047345569668));
#70024=CARTESIAN_POINT('Ctrl Pts',(87.9784353889358,58.6783012289841,10.7932992900981));
#70025=CARTESIAN_POINT('Ctrl Pts',(88.067699914573,58.6689047041998,10.794148126335));
#70026=CARTESIAN_POINT('Ctrl Pts',(88.2054946442493,58.6542982785079,10.809997750042));
#70027=CARTESIAN_POINT('Ctrl Pts',(88.2544974247389,58.6490896776457,10.8185705767224));
#70028=CARTESIAN_POINT('Ctrl Pts',(88.3149112348361,58.6427270035871,10.8328370560962));
#70029=CARTESIAN_POINT('Ctrl Pts',(88.3269035998228,58.6414670526868,10.8358545444968));
#70030=CARTESIAN_POINT('Ctrl Pts',(88.3447692409538,58.6395963491309,10.8406283734652));
#70031=CARTESIAN_POINT('Ctrl Pts',(88.3506764199351,58.6389788514012,10.8422526956962));
#70032=CARTESIAN_POINT('Ctrl Pts',(88.3608704792266,58.63791528378,10.845135304943));
#70033=CARTESIAN_POINT('Ctrl Pts',(88.3651626780616,58.6374681197263,10.8463735179295));
#70034=CARTESIAN_POINT('Ctrl Pts',(88.3752675515055,58.6364168922349,10.8493464161891));
#70035=CARTESIAN_POINT('Ctrl Pts',(88.3810744688797,58.6358139325587,10.8511001336936));
#70036=CARTESIAN_POINT('Ctrl Pts',(88.3983850683685,58.6340192525014,10.8564636570658));
#70037=CARTESIAN_POINT('Ctrl Pts',(88.4098506962277,58.6328342100168,10.8601959043312));
#70038=CARTESIAN_POINT('Ctrl Pts',(88.4976553892865,58.6237738875421,10.8901673495209));
#70039=CARTESIAN_POINT('Ctrl Pts',(88.5714044312577,58.6162440517771,10.9234729705172));
#70040=CARTESIAN_POINT('Ctrl Pts',(88.7119240501686,58.6010799772221,11.003838706996));
#70041=CARTESIAN_POINT('Ctrl Pts',(88.778312033937,58.5934762488734,11.0507611068985));
#70042=CARTESIAN_POINT('Ctrl Pts',(88.8523737681701,58.5840088797201,11.1145447861536));
#70043=CARTESIAN_POINT('Ctrl Pts',(88.8647659290384,58.5823882705203,11.1256487259842));
#70044=CARTESIAN_POINT('Ctrl Pts',(88.8841393004861,58.5797923868578,11.1437068045899));
#70045=CARTESIAN_POINT('Ctrl Pts',(88.8912642844276,58.5788237398503,11.1505046409948));
#70046=CARTESIAN_POINT('Ctrl Pts',(88.9046403991701,58.5769778010686,11.1635670961257));
#70047=CARTESIAN_POINT('Ctrl Pts',(88.9109065443432,58.5761012503558,11.169815582375));
#70048=CARTESIAN_POINT('Ctrl Pts',(88.9251025132104,58.5740876090394,11.1842705538872));
#70049=CARTESIAN_POINT('Ctrl Pts',(88.9329879016964,58.5729486773214,11.1925193144278));
#70050=CARTESIAN_POINT('Ctrl Pts',(88.9536019177779,58.5699153258734,11.2146734028036));
#70051=CARTESIAN_POINT('Ctrl Pts',(88.9661333172046,58.568012881167,11.2287571442493));
#70052=CARTESIAN_POINT('Ctrl Pts',(89.0496665149654,58.5549133065949,11.3269547691037));
#70053=CARTESIAN_POINT('Ctrl Pts',(89.1097694970408,58.5432873123365,11.4196953926493));
#70054=CARTESIAN_POINT('Ctrl Pts',(89.1781065003179,58.526600131987,11.562881542631));
#70055=CARTESIAN_POINT('Ctrl Pts',(89.196520648374,58.5215176853357,11.6079519533705));
#70056=CARTESIAN_POINT('Ctrl Pts',(89.2154232907968,58.5155731287881,11.6630646562695));
#70057=CARTESIAN_POINT('Ctrl Pts',(89.2184379953646,58.514597477717,11.6721905761405));
#70058=CARTESIAN_POINT('Ctrl Pts',(89.2230324687728,58.5130663936297,11.6866476696338));
#70059=CARTESIAN_POINT('Ctrl Pts',(89.2246812294648,58.5125072593936,11.6919561876885));
#70060=CARTESIAN_POINT('Ctrl Pts',(89.2277664843263,58.5114422578257,11.7021250148485));
#70061=CARTESIAN_POINT('Ctrl Pts',(89.2292087646248,58.5109361094244,11.7069831620253));
#70062=CARTESIAN_POINT('Ctrl Pts',(89.232645388408,58.5097092492029,11.7188182120293));
#70063=CARTESIAN_POINT('Ctrl Pts',(89.2346091063273,58.5089902815678,11.725803860849));
#70064=CARTESIAN_POINT('Ctrl Pts',(89.2411970534292,58.5065130044844,11.7500348515875));
#70065=CARTESIAN_POINT('Ctrl Pts',(89.2455177807447,58.5047705156264,11.7673618739297));
#70066=CARTESIAN_POINT('Ctrl Pts',(89.2669603556061,58.4953996100657,11.8617919774794));
#70067=CARTESIAN_POINT('Ctrl Pts',(89.2772293546733,58.4880534419646,11.9402840041561));
#70068=CARTESIAN_POINT('Ctrl Pts',(89.2819951784243,58.4759241693202,12.0696144020795));
#70069=CARTESIAN_POINT('Ctrl Pts',(89.2808499059722,58.4711883895201,12.1200579776393));
#70070=CARTESIAN_POINT('Ctrl Pts',(89.2740808794595,58.4633221547994,12.2022047800746));
#70071=CARTESIAN_POINT('Ctrl Pts',(89.27024621205,58.4602399467561,12.2339989251376));
#70072=CARTESIAN_POINT('Ctrl Pts',(89.2632418669668,58.4558975424663,12.2780092113431));
#70073=CARTESIAN_POINT('Ctrl Pts',(89.2610850943507,58.4546689023842,12.2903765331183));
#70074=CARTESIAN_POINT('Ctrl Pts',(89.2570641707339,58.452547453924,12.311571680849));
#70075=CARTESIAN_POINT('Ctrl Pts',(89.2552885801581,58.4516574985606,12.3204155788569));
#70076=CARTESIAN_POINT('Ctrl Pts',(89.2514730509701,58.4498350906204,12.3384238389548));
#70077=CARTESIAN_POINT('Ctrl Pts',(89.2494253994663,58.4489024444644,12.3475859656692));
#70078=CARTESIAN_POINT('Ctrl Pts',(89.2439695450625,58.4465262794236,12.3707864536412));
#70079=CARTESIAN_POINT('Ctrl Pts',(89.2404231516483,58.445078433943,12.384790450371));
#70080=CARTESIAN_POINT('Ctrl Pts',(89.2247991316418,58.4390690122588,12.4423428064532));
#70081=CARTESIAN_POINT('Ctrl Pts',(89.2106420066052,58.4344424531357,12.4852851696894));
#70082=CARTESIAN_POINT('Ctrl Pts',(89.1609531959061,58.4202532957062,12.6127154717471));
#70083=CARTESIAN_POINT('Ctrl Pts',(89.1185428065423,58.4105211119895,12.6942006333123));
#70084=CARTESIAN_POINT('Ctrl Pts',(89.048390739255,58.3972908421033,12.7994428383259));
#70085=CARTESIAN_POINT('Ctrl Pts',(89.0278425470015,58.3936709820817,12.8276756806663));
#70086=CARTESIAN_POINT('Ctrl Pts',(89.0006440106737,58.3892109097503,12.8619795218085));
#70087=CARTESIAN_POINT('Ctrl Pts',(88.9950606346836,58.3883115206806,12.8688719390346));
#70088=CARTESIAN_POINT('Ctrl Pts',(88.9859638161077,58.3868725669035,12.8798640506232));
#70089=CARTESIAN_POINT('Ctrl Pts',(88.9824958172821,58.3863299902342,12.8840006214246));
#70090=CARTESIAN_POINT('Ctrl Pts',(88.9757055829966,58.3852794046092,12.8919957993825));
#70091=CARTESIAN_POINT('Ctrl Pts',(88.9723864299962,58.3847712259424,12.8958566484953));
#70092=CARTESIAN_POINT('Ctrl Pts',(88.9640132241627,58.3835022689435,12.9054787218968));
#70093=CARTESIAN_POINT('Ctrl Pts',(88.9589299964689,58.3827435975447,12.9112144476724));
#70094=CARTESIAN_POINT('Ctrl Pts',(88.9399992934022,58.3799592000895,12.9321895157328));
#70095=CARTESIAN_POINT('Ctrl Pts',(88.9258325639842,58.3779549763666,12.9471387610327));
#70096=CARTESIAN_POINT('Ctrl Pts',(88.857241230216,58.3685757050472,13.0160799497583));
#70097=CARTESIAN_POINT('Ctrl Pts',(88.7983586355497,58.3614463243779,13.0654227539293));
#70098=CARTESIAN_POINT('Ctrl Pts',(88.6946773653598,58.3496142310001,13.1374198284483));
#70099=CARTESIAN_POINT('Ctrl Pts',(88.6523624066709,58.3449575386355,13.1632733072907));
#70100=CARTESIAN_POINT('Ctrl Pts',(88.5896220205865,58.3381697481612,13.196734955352));
#70101=CARTESIAN_POINT('Ctrl Pts',(88.5703413516156,58.3360990337979,13.206395597784));
#70102=CARTESIAN_POINT('Ctrl Pts',(88.535046751526,58.3323259332403,13.2229696904649));
#70103=CARTESIAN_POINT('Ctrl Pts',(88.5191182975175,58.3306293947817,13.2300530863234));
#70104=CARTESIAN_POINT('Ctrl Pts',(88.4938186334599,58.3279408297784,13.2406856759083));
#70105=CARTESIAN_POINT('Ctrl Pts',(88.4845420248605,58.3269562918225,13.2444558568179));
#70106=CARTESIAN_POINT('Ctrl Pts',(88.4670121477407,58.3250975134683,13.2513399173737));
#70107=CARTESIAN_POINT('Ctrl Pts',(88.458769069066,58.324224154033,13.2544782915241));
#70108=CARTESIAN_POINT('Ctrl Pts',(88.4400500964841,58.3222419319001,13.2613827566492));
#70109=CARTESIAN_POINT('Ctrl Pts',(88.4295562022615,58.3211314386496,13.2650974128277));
#70110=CARTESIAN_POINT('Ctrl Pts',(88.4020967793693,58.3182265664748,13.2744132109398));
#70111=CARTESIAN_POINT('Ctrl Pts',(88.3850602172566,58.3164252240534,13.2797948961812));
#70112=CARTESIAN_POINT('Ctrl Pts',(88.2706129929587,58.3043230017434,13.3133095345537));
#70113=CARTESIAN_POINT('Ctrl Pts',(88.1702692631488,58.2936613478557,13.330042398711));
#70114=CARTESIAN_POINT('Ctrl Pts',(88.0290736568651,58.2787665736703,13.336501306081));
#70115=CARTESIAN_POINT('Ctrl Pts',(87.9890452397125,58.2745619939403,13.3364403701319));
#70116=CARTESIAN_POINT('Ctrl Pts',(87.9263363182777,58.2680498841345,13.3333794727661));
#70117=CARTESIAN_POINT('Ctrl Pts',(87.903620648719,58.2657066236617,13.3316573634987));
#70118=CARTESIAN_POINT('Ctrl Pts',(87.8732694413172,58.2626059193666,13.3285332013652));
#70119=CARTESIAN_POINT('Ctrl Pts',(87.8655846306259,58.2618234450197,13.3276711824862));
#70120=CARTESIAN_POINT('Ctrl Pts',(87.8527895999044,58.2605254806098,13.3261174753903));
#70121=CARTESIAN_POINT('Ctrl Pts',(87.8476749955015,58.2600079337665,13.3254647791904));
#70122=CARTESIAN_POINT('Ctrl Pts',(87.8378775906762,58.2590191728347,13.3241538020797));
#70123=CARTESIAN_POINT('Ctrl Pts',(87.8331943014986,58.2585476764829,13.3235004948725));
#70124=CARTESIAN_POINT('Ctrl Pts',(87.8204206684261,58.2572645136297,13.3216458145816));
#70125=CARTESIAN_POINT('Ctrl Pts',(87.8123378573726,58.2564556772551,13.3203923865316));
#70126=CARTESIAN_POINT('Ctrl Pts',(87.7801305916342,58.2532430094398,13.3150787628242));
#70127=CARTESIAN_POINT('Ctrl Pts',(87.7561111497571,58.2508701164471,13.3103996097835));
#70128=CARTESIAN_POINT('Ctrl Pts',(87.6604818668318,58.2414573869847,13.2888846184787));
#70129=CARTESIAN_POINT('Ctrl Pts',(87.5902540031261,58.2346174625761,13.2665353614745));
#70130=CARTESIAN_POINT('Ctrl Pts',(87.4777213102011,58.2231863794653,13.2196253976678));
#70131=CARTESIAN_POINT('Ctrl Pts',(87.4341963076196,58.2186392853675,13.1984903992423));
#70132=CARTESIAN_POINT('Ctrl Pts',(87.3647690740798,58.2110461799235,13.1597353874689));
#70133=CARTESIAN_POINT('Ctrl Pts',(87.3381244210555,58.2080439466192,13.1435479578421));
#70134=CARTESIAN_POINT('Ctrl Pts',(87.301722704792,58.2037948979502,13.1195560341631));
#70135=CARTESIAN_POINT('Ctrl Pts',(87.2914425164443,58.2025777995275,13.1125617993605));
#70136=CARTESIAN_POINT('Ctrl Pts',(87.2739014351877,58.2004699301109,13.1002469238456));
#70137=CARTESIAN_POINT('Ctrl Pts',(87.2665911833855,58.1995819160712,13.094997811952));
#70138=CARTESIAN_POINT('Ctrl Pts',(87.2526467505545,58.1978690179649,13.0847586824416));
#70139=CARTESIAN_POINT('Ctrl Pts',(87.2460044687283,58.1970446245268,13.0797804164424));
#70140=CARTESIAN_POINT('Ctrl Pts',(87.2285883359835,58.1948600599779,13.066458730388));
#70141=CARTESIAN_POINT('Ctrl Pts',(87.2178995121185,58.1934956773863,13.0580066845039));
#70142=CARTESIAN_POINT('Ctrl Pts',(87.1983434524692,58.1909539173572,13.0420249009918));
#70143=CARTESIAN_POINT('Ctrl Pts',(87.189440499867,58.1897786506171,13.0345428123893));
#70144=CARTESIAN_POINT('Ctrl Pts',(87.1806428261678,58.1885986874538,13.0269406661524));
#70145=CARTESIAN_POINT('Origin',(88.011,66.41344859951,12.066));
#70146=CARTESIAN_POINT('',(87.1806428354228,57.224088141927,13.0269406741497));
#70147=CARTESIAN_POINT('',(87.1806427720391,57.39301128552,13.0269406193793));
#70148=CARTESIAN_POINT('',(87.1806428354228,66.41344859951,13.0269406741497));
#70149=CARTESIAN_POINT('',(86.7410005228783,57.90950140049,12.0648475632288));
#70150=CARTESIAN_POINT('Ctrl Pts',(86.7410005228783,57.90950140049,12.0648475632288));
#70151=CARTESIAN_POINT('Ctrl Pts',(86.7410619857771,57.9027591545593,11.9971146937284));
#70152=CARTESIAN_POINT('Ctrl Pts',(86.7465456957433,57.8960169086286,11.929620021689));
#70153=CARTESIAN_POINT('Ctrl Pts',(86.7573167636289,57.8892746626979,11.8630755242906));
#70154=CARTESIAN_POINT('Ctrl Pts',(86.7614355253459,57.8866964870962,11.8376294931931));
#70155=CARTESIAN_POINT('Ctrl Pts',(86.7663269456463,57.8841183114945,11.8123221050166));
#70156=CARTESIAN_POINT('Ctrl Pts',(86.7719817452547,57.8815401358928,11.7871922447137));
#70157=CARTESIAN_POINT('Ctrl Pts',(86.7828344623163,57.8765920895821,11.7389629028177));
#70158=CARTESIAN_POINT('Ctrl Pts',(86.7965314004248,57.8716440432713,11.691261574028));
#70159=CARTESIAN_POINT('Ctrl Pts',(86.8130042208988,57.8666959969606,11.6444479708794));
#70160=CARTESIAN_POINT('Ctrl Pts',(86.8294467317454,57.8617570549463,11.5977205037312));
#70161=CARTESIAN_POINT('Ctrl Pts',(86.8486548145271,57.8568181129319,11.55187803535));
#70162=CARTESIAN_POINT('Ctrl Pts',(86.8705096968997,57.8518791709176,11.5072676235135));
#70163=CARTESIAN_POINT('Ctrl Pts',(86.8923423888668,57.8469452436695,11.4627025069625));
#70164=CARTESIAN_POINT('Ctrl Pts',(86.9168163203082,57.8420113164214,11.4193674601876));
#70165=CARTESIAN_POINT('Ctrl Pts',(86.9437645123884,57.8370773891734,11.3775899376226));
#70166=CARTESIAN_POINT('Ctrl Pts',(86.9706968097254,57.8321463720837,11.3358370565249));
#70167=CARTESIAN_POINT('Ctrl Pts',(87.0001001801263,57.827215354994,11.2956403393399));
#70168=CARTESIAN_POINT('Ctrl Pts',(87.0317628358655,57.8222843379043,11.2573006885264));
#70169=CARTESIAN_POINT('Ctrl Pts',(87.0634202885994,57.8173541311101,11.2189673379237));
#70170=CARTESIAN_POINT('Ctrl Pts',(87.0973359401222,57.8124239243159,11.1824908695214));
#70171=CARTESIAN_POINT('Ctrl Pts',(87.133257610372,57.8074937175218,11.1481392821075));
#70172=CARTESIAN_POINT('Ctrl Pts',(87.1692143770386,57.8025586937859,11.1137541322891));
#70173=CARTESIAN_POINT('Ctrl Pts',(87.2071806781485,57.79762367005,11.0814983872616));
#70174=CARTESIAN_POINT('Ctrl Pts',(87.2468686439494,57.7926886463141,11.0516020156269));
#70175=CARTESIAN_POINT('Ctrl Pts',(87.2865779685748,57.7877509667024,11.021689554698));
#70176=CARTESIAN_POINT('Ctrl Pts',(87.3280103461592,57.7828132870908,10.9941392993314));
#70177=CARTESIAN_POINT('Ctrl Pts',(87.3708490295984,57.7778756074791,10.9691377775245));
#70178=CARTESIAN_POINT('Ctrl Pts',(87.4137677090518,57.7729287073532,10.9440895684263));
#70179=CARTESIAN_POINT('Ctrl Pts',(87.4580974467746,57.7679818072274,10.9215998401677));
#70180=CARTESIAN_POINT('Ctrl Pts',(87.5034984997004,57.7630349071015,10.9018083374317));
#70181=CARTESIAN_POINT('Ctrl Pts',(87.5264702739549,57.7605319018709,10.8917943420789));
#70182=CARTESIAN_POINT('Ctrl Pts',(87.5497160264354,57.7580288966402,10.8824703397855));
#70183=CARTESIAN_POINT('Ctrl Pts',(87.573190329049,57.7555258914096,10.8738495514316));
#70184=CARTESIAN_POINT('Ctrl Pts',(87.6195953205454,57.7505778450988,10.8568076134095));
#70185=CARTESIAN_POINT('Ctrl Pts',(87.6670994190304,57.7456297987881,10.8424415593594));
#70186=CARTESIAN_POINT('Ctrl Pts',(87.7153633555719,57.7406817524774,10.8308890841421));
#70187=CARTESIAN_POINT('Ctrl Pts',(87.7635384875313,57.735742810463,10.8193578652253));
#70188=CARTESIAN_POINT('Ctrl Pts',(87.8124701560871,57.7308038684487,10.8106300840773));
#70189=CARTESIAN_POINT('Ctrl Pts',(87.8618023686802,57.7258649264344,10.8047942012469));
#70190=CARTESIAN_POINT('Ctrl Pts',(87.9110844916965,57.7209309991863,10.7989642438936));
#70191=CARTESIAN_POINT('Ctrl Pts',(87.960765812076,57.7159970719382,10.7960204360653));
#70192=CARTESIAN_POINT('Ctrl Pts',(88.0104806593026,57.7110631446902,10.7960001061869));
#70193=CARTESIAN_POINT('Ctrl Pts',(88.0601661834216,57.7061321276005,10.7959797882996));
#70194=CARTESIAN_POINT('Ctrl Pts',(88.1098846482655,57.7012011105108,10.7988795325896));
#70195=CARTESIAN_POINT('Ctrl Pts',(88.1592683859079,57.6962700934211,10.8046846208262));
#70196=CARTESIAN_POINT('Ctrl Pts',(88.208644008506,57.6913398866269,10.8104887551345));
#70197=CARTESIAN_POINT('Ctrl Pts',(88.2576844692856,57.6864096798327,10.8191972206621));
#70198=CARTESIAN_POINT('Ctrl Pts',(88.3060278346373,57.6814794730386,10.8307435178113));
#70199=CARTESIAN_POINT('Ctrl Pts',(88.3544184327286,57.6765444493027,10.8423010959965));
#70200=CARTESIAN_POINT('Ctrl Pts',(88.4021100417701,57.6716094255668,10.856701913136));
#70201=CARTESIAN_POINT('Ctrl Pts',(88.4487533200729,57.6666744018309,10.8738288584414));
#70202=CARTESIAN_POINT('Ctrl Pts',(88.4954217003324,57.6617367222192,10.8909650209343));
#70203=CARTESIAN_POINT('Ctrl Pts',(88.5410401234826,57.6567990426076,10.9108300140715));
#70204=CARTESIAN_POINT('Ctrl Pts',(88.5852800801664,57.6518613629959,10.9332589044605));
#70205=CARTESIAN_POINT('Ctrl Pts',(88.6296026495712,57.6469144628701,10.9557296780655));
#70206=CARTESIAN_POINT('Ctrl Pts',(88.6725411413171,57.6419675627442,10.9807736284387));
#70207=CARTESIAN_POINT('Ctrl Pts',(88.7137938767186,57.6370206626184,11.0081811275806));
#70208=CARTESIAN_POINT('Ctrl Pts',(88.7346667081612,57.6345176573877,11.0220486227729));
#70209=CARTESIAN_POINT('Ctrl Pts',(88.7551084672777,57.632014652157,11.0365205442552));
#70210=CARTESIAN_POINT('Ctrl Pts',(88.7750834067852,57.6295116469264,11.0515658979138));
#70211=CARTESIAN_POINT('Ctrl Pts',(88.8145707096986,57.6245636006156,11.081308187603));
#70212=CARTESIAN_POINT('Ctrl Pts',(88.8524061001075,57.6196155543049,11.113425256499));
#70213=CARTESIAN_POINT('Ctrl Pts',(88.8882898785945,57.6146675079941,11.1477067631113));
#70214=CARTESIAN_POINT('Ctrl Pts',(88.9241076317183,57.6097285659798,11.1819251925053));
#70215=CARTESIAN_POINT('Ctrl Pts',(88.957980501935,57.6047896239655,11.2182997854886));
#70216=CARTESIAN_POINT('Ctrl Pts',(88.9896410817415,57.5998506819511,11.2565794460678));
#70217=CARTESIAN_POINT('Ctrl Pts',(89.0212695149046,57.5949167547031,11.2948202393047));
#70218=CARTESIAN_POINT('Ctrl Pts',(89.0506897569054,57.589982827455,11.3349618506302));
#70219=CARTESIAN_POINT('Ctrl Pts',(89.0776721081081,57.5850489002069,11.3767173193934));
#70220=CARTESIAN_POINT('Ctrl Pts',(89.1046385444195,57.5801178831172,11.4184481596971));
#70221=CARTESIAN_POINT('Ctrl Pts',(89.1291696416839,57.5751868660275,11.4617905123143));
#70222=CARTESIAN_POINT('Ctrl Pts',(89.1510783423698,57.5702558489378,11.5064275084859));
#70223=CARTESIAN_POINT('Ctrl Pts',(89.1729834428811,57.5653256421437,11.5510571696275));
#70224=CARTESIAN_POINT('Ctrl Pts',(89.1922667618919,57.5603954353495,11.5969805598905));
#70225=CARTESIAN_POINT('Ctrl Pts',(89.2087878547802,57.5554652285553,11.6438575418877));
#70226=CARTESIAN_POINT('Ctrl Pts',(89.2253250892107,57.5505302048195,11.6907803239294));
#70227=CARTESIAN_POINT('Ctrl Pts',(89.2390945276057,57.5455951810836,11.738658039764));
#70228=CARTESIAN_POINT('Ctrl Pts',(89.250005074718,57.5406601573477,11.787133679296));
#70229=CARTESIAN_POINT('Ctrl Pts',(89.2609214935463,57.535722477736,11.8356354069045));
#70230=CARTESIAN_POINT('Ctrl Pts',(89.2689758685409,57.5307847981243,11.8847351576829));
#70231=CARTESIAN_POINT('Ctrl Pts',(89.274128580668,57.5258471185127,11.9340674842974));
#70232=CARTESIAN_POINT('Ctrl Pts',(89.2792909148563,57.5209002183868,11.9834919330123));
#70233=CARTESIAN_POINT('Ctrl Pts',(89.281540746755,57.515953318261,12.0331492766801));
#70234=CARTESIAN_POINT('Ctrl Pts',(89.2808905591385,57.5110064181352,12.0826723666826));
#70235=CARTESIAN_POINT('Ctrl Pts',(89.2805615807958,57.5085034129045,12.1077297865134));
#70236=CARTESIAN_POINT('Ctrl Pts',(89.2794909980342,57.5060004076738,12.1327528934289));
#70237=CARTESIAN_POINT('Ctrl Pts',(89.2776854603828,57.5034974024432,12.1576948442112));
#70238=CARTESIAN_POINT('Ctrl Pts',(89.2741161974,57.4985493561325,12.2070011445093));
#70239=CARTESIAN_POINT('Ctrl Pts',(89.2676558368303,57.4936013098217,12.2562077154442));
#70240=CARTESIAN_POINT('Ctrl Pts',(89.2583185344195,57.488653263511,12.3049486842262));
#70241=CARTESIAN_POINT('Ctrl Pts',(89.2489984124399,57.4837143214966,12.3535999706975));
#70242=CARTESIAN_POINT('Ctrl Pts',(89.2368119496979,57.4787753794823,12.4017868203275));
#70243=CARTESIAN_POINT('Ctrl Pts',(89.2218250557544,57.473836437468,12.4491483842551));
#70244=CARTESIAN_POINT('Ctrl Pts',(89.2068533787886,57.4689025102199,12.4964618595086));
#70245=CARTESIAN_POINT('Ctrl Pts',(89.1890870641493,57.4639685829718,12.5429511879973));
#70246=CARTESIAN_POINT('Ctrl Pts',(89.1686426047564,57.4590346557237,12.5882677470921));
#70247=CARTESIAN_POINT('Ctrl Pts',(89.1482102040365,57.454103638634,12.6335575773039));
#70248=CARTESIAN_POINT('Ctrl Pts',(89.1251030128179,57.4491726215443,12.6776755099094));
#70249=CARTESIAN_POINT('Ctrl Pts',(89.0994857794802,57.4442416044546,12.7202925246932));
#70250=CARTESIAN_POINT('Ctrl Pts',(89.0738727557262,57.4393113976605,12.762902536383));
#70251=CARTESIAN_POINT('Ctrl Pts',(89.0457507917049,57.4343811908663,12.8040116510038));
#70252=CARTESIAN_POINT('Ctrl Pts',(89.0153294670472,57.4294509840721,12.8433173879573));
#70253=CARTESIAN_POINT('Ctrl Pts',(88.984878419955,57.4245159603362,12.8826615276497));
#70254=CARTESIAN_POINT('Ctrl Pts',(88.9521238636205,57.4195809366003,12.9201983382039));
#70255=CARTESIAN_POINT('Ctrl Pts',(88.9173163198337,57.4146459128644,12.95565764674));
#70256=CARTESIAN_POINT('Ctrl Pts',(88.8824900437131,57.4097082332528,12.9911360383694));
#70257=CARTESIAN_POINT('Ctrl Pts',(88.8456089866316,57.4047705536411,13.0245343334098));
#70258=CARTESIAN_POINT('Ctrl Pts',(88.8069586793161,57.3998328740294,13.05562102889));
#70259=CARTESIAN_POINT('Ctrl Pts',(88.7682361972678,57.3948859739036,13.0867657749809));
#70260=CARTESIAN_POINT('Ctrl Pts',(88.7277383175997,57.3899390737777,13.1155899881723));
#70261=CARTESIAN_POINT('Ctrl Pts',(88.6857802602803,57.3849921736519,13.141905014551));
#70262=CARTESIAN_POINT('Ctrl Pts',(88.6645505539457,57.3824891684212,13.1552197464022));
#70263=CARTESIAN_POINT('Ctrl Pts',(88.6429474292981,57.3799861631906,13.1678928293979));
#70264=CARTESIAN_POINT('Ctrl Pts',(88.6210138470131,57.3774831579599,13.1799044422446));
#70265=CARTESIAN_POINT('Ctrl Pts',(88.5776546164459,57.3725351116492,13.2036495051411));
#70266=CARTESIAN_POINT('Ctrl Pts',(88.5328110428732,57.3675870653385,13.2249116026642));
#70267=CARTESIAN_POINT('Ctrl Pts',(88.4867981818304,57.3626390190277,13.2435041784074));
#70268=CARTESIAN_POINT('Ctrl Pts',(88.44086998344,57.3577000770134,13.2620625442201));
#70269=CARTESIAN_POINT('Ctrl Pts',(88.3937772685885,57.3527611349991,13.277960926507));
#70270=CARTESIAN_POINT('Ctrl Pts',(88.345858943308,57.3478221929847,13.2910589733097));
#70271=CARTESIAN_POINT('Ctrl Pts',(88.2979892720104,57.3428882657367,13.3041437209802));
#70272=CARTESIAN_POINT('Ctrl Pts',(88.2492961758408,57.3379543384886,13.3144336181903));
#70273=CARTESIAN_POINT('Ctrl Pts',(88.2001357256658,57.3330204112405,13.3218374406255));
#70274=CARTESIAN_POINT('Ctrl Pts',(88.1510042716006,57.3280893941508,13.3292368960941));
#70275=CARTESIAN_POINT('Ctrl Pts',(88.1014065504667,57.3231583770611,13.3337535676249));
#70276=CARTESIAN_POINT('Ctrl Pts',(88.0517083384299,57.3182273599714,13.3353474036615));
#70277=CARTESIAN_POINT('Ctrl Pts',(88.0020182931138,57.3132971531773,13.3369409777891));
#70278=CARTESIAN_POINT('Ctrl Pts',(87.9522283371031,57.3083669463831,13.3356126533678));
#70279=CARTESIAN_POINT('Ctrl Pts',(87.9027062664847,57.3034367395889,13.3313744375802));
#70280=CARTESIAN_POINT('Ctrl Pts',(87.8531358115008,57.298501715853,13.3271320809442));
#70281=CARTESIAN_POINT('Ctrl Pts',(87.8038343114249,57.2935666921171,13.3199742043374));
#70282=CARTESIAN_POINT('Ctrl Pts',(87.7551646269224,57.2886316683812,13.3099647349834));
#70283=CARTESIAN_POINT('Ctrl Pts',(87.7064687499145,57.2836939887696,13.2999498788453));
#70284=CARTESIAN_POINT('Ctrl Pts',(87.658405895437,57.2787563091579,13.2870805159034));
#70285=CARTESIAN_POINT('Ctrl Pts',(87.6113254255502,57.2738186295463,13.2714709596412));
#70286=CARTESIAN_POINT('Ctrl Pts',(87.5641570386307,57.2688717294204,13.2558322544374));
#70287=CARTESIAN_POINT('Ctrl Pts',(87.5179752070549,57.2639248292946,13.2374433459321));
#70288=CARTESIAN_POINT('Ctrl Pts',(87.4731093978903,57.2589779291688,13.2164667314452));
#70289=CARTESIAN_POINT('Ctrl Pts',(87.4504084433207,57.2564749239381,13.2058530997875));
#70290=CARTESIAN_POINT('Ctrl Pts',(87.4280440099079,57.2539719187074,13.1945777219539));
#70291=CARTESIAN_POINT('Ctrl Pts',(87.4060560517573,57.2514689134767,13.1826659390725));
#70292=CARTESIAN_POINT('Ctrl Pts',(87.3626043588745,57.2465225781316,13.1591263667343));
#70293=CARTESIAN_POINT('Ctrl Pts',(87.3204326650643,57.2415762427864,13.1329948052886));
#70294=CARTESIAN_POINT('Ctrl Pts',(87.2798682499743,57.2366299074413,13.1044345738198));
#70295=CARTESIAN_POINT('Ctrl Pts',(87.2455836502466,57.2324493189365,13.080295778724));
#70296=CARTESIAN_POINT('Ctrl Pts',(87.2124470760778,57.2282687304318,13.0544229941328));
#70297=CARTESIAN_POINT('Ctrl Pts',(87.1806428354228,57.224088141927,13.0269406741497));
#70298=CARTESIAN_POINT('Ctrl Pts',(87.1795113209163,58.0179748583214,13.028265366586));
#70299=CARTESIAN_POINT('Ctrl Pts',(87.1530435317638,58.014501365673,13.0056897999309));
#70300=CARTESIAN_POINT('Ctrl Pts',(86.8879207557325,57.9783435977464,12.7588929134556));
#70301=CARTESIAN_POINT('Ctrl Pts',(86.743865944262,57.9421858298198,12.3932421316416));
#70302=CARTESIAN_POINT('Ctrl Pts',(86.7408356874277,57.9095015545417,12.0648489614637));
#70303=CARTESIAN_POINT('Ctrl Pts',(87.1806428261678,58.1885986874538,13.0269406661524));
#70304=CARTESIAN_POINT('Ctrl Pts',(87.1609641663325,58.1859593427242,13.0099361653115));
#70305=CARTESIAN_POINT('Ctrl Pts',(87.1418122557908,58.1832963391464,12.9923309966038));
#70306=CARTESIAN_POINT('Ctrl Pts',(87.0519099702601,58.1703207988888,12.9044446282297));
#70307=CARTESIAN_POINT('Ctrl Pts',(86.9890694800532,58.1597250790729,12.8265891326154));
#70308=CARTESIAN_POINT('Ctrl Pts',(86.9168429676078,58.1455276365694,12.7117659337051));
#70309=CARTESIAN_POINT('Ctrl Pts',(86.8989940863025,58.1417952157628,12.6805216162562));
#70310=CARTESIAN_POINT('Ctrl Pts',(86.8783909365337,58.1372185375922,12.6406100448996));
#70311=CARTESIAN_POINT('Ctrl Pts',(86.8743721386058,58.1363114800545,12.6326190216156));
#70312=CARTESIAN_POINT('Ctrl Pts',(86.8680566715997,58.1348632524529,12.6197236304901));
#70313=CARTESIAN_POINT('Ctrl Pts',(86.8657064771589,58.1343190035126,12.6148461182345));
#70314=CARTESIAN_POINT('Ctrl Pts',(86.8612110354625,58.133267718598,12.6053618062651));
#70315=CARTESIAN_POINT('Ctrl Pts',(86.8590621872782,58.1327604973651,12.6007570466441));
#70316=CARTESIAN_POINT('Ctrl Pts',(86.8542796468877,58.1316205956781,12.5903459450481));
#70317=CARTESIAN_POINT('Ctrl Pts',(86.8516619172355,58.1309888755473,12.5845324112614));
#70318=CARTESIAN_POINT('Ctrl Pts',(86.8424647967122,58.1287401517919,12.5636893024982));
#70319=CARTESIAN_POINT('Ctrl Pts',(86.8361325237269,58.1271367843992,12.5485512075589));
#70320=CARTESIAN_POINT('Ctrl Pts',(86.7886810831452,58.1146339648853,12.4286358554004));
#70321=CARTESIAN_POINT('Ctrl Pts',(86.7613571608766,58.1043366032532,12.3189217790707));
#70322=CARTESIAN_POINT('Ctrl Pts',(86.743632010035,58.0892456771226,12.1602880143216));
#70323=CARTESIAN_POINT('Ctrl Pts',(86.7410104748876,58.0847568795635,12.1133009844547));
#70324=CARTESIAN_POINT('Ctrl Pts',(86.740996868144,58.0788036501029,12.052040829192));
#70325=CARTESIAN_POINT('Ctrl Pts',(86.7412332481562,58.0774129161942,12.0378012425294));
#70326=CARTESIAN_POINT('Ctrl Pts',(86.7420212575764,58.0750971481515,12.0142283650332));
#70327=CARTESIAN_POINT('Ctrl Pts',(86.7424366055087,58.074176399149,12.0048914621107));
#70328=CARTESIAN_POINT('Ctrl Pts',(86.7434567202418,58.0723579862332,11.9865275074311));
#70329=CARTESIAN_POINT('Ctrl Pts',(86.7440549754702,58.071460579516,11.9775006375718));
#70330=CARTESIAN_POINT('Ctrl Pts',(86.7457249556406,58.0692957366276,11.9558164744029));
#70331=CARTESIAN_POINT('Ctrl Pts',(86.7468902189997,58.0680254580803,11.9431676809069));
#70332=CARTESIAN_POINT('Ctrl Pts',(86.7517749053325,58.0634236855104,11.8976330572363));
#70333=CARTESIAN_POINT('Ctrl Pts',(86.756589305555,58.0600588922583,11.8648817128486));
#70334=CARTESIAN_POINT('Ctrl Pts',(86.772453910004,58.0511944786744,11.7801183743937));
#70335=CARTESIAN_POINT('Ctrl Pts',(86.7854998204982,58.0456438345551,11.7285499263457));
#70336=CARTESIAN_POINT('Ctrl Pts',(86.8274903724479,58.0311843007983,11.5976941116045));
#70337=CARTESIAN_POINT('Ctrl Pts',(86.8611751512743,58.0222383138625,11.5201875718347));
#70338=CARTESIAN_POINT('Ctrl Pts',(86.9079437883526,58.0124193633623,11.4364755161873));
#70339=CARTESIAN_POINT('Ctrl Pts',(86.9137297331258,58.0112402871914,11.4264438434461));
#70340=CARTESIAN_POINT('Ctrl Pts',(86.9227432303269,58.009457928551,11.4112987498286));
#70341=CARTESIAN_POINT('Ctrl Pts',(86.9258711589752,58.0088489188173,11.406127339856));
#70342=CARTESIAN_POINT('Ctrl Pts',(86.9313757794217,58.0077937671844,11.3971715406549));
#70343=CARTESIAN_POINT('Ctrl Pts',(86.9337356165596,58.0073465974539,11.3933772111385));
#70344=CARTESIAN_POINT('Ctrl Pts',(86.9393909518938,58.0062871022269,11.3843902380527));
#70345=CARTESIAN_POINT('Ctrl Pts',(86.942704216949,58.0056759464112,11.37920895078));
#70346=CARTESIAN_POINT('Ctrl Pts',(86.952858197018,58.0038309301573,11.3635814397178));
#70347=CARTESIAN_POINT('Ctrl Pts',(86.9598157884563,58.0026043134095,11.3532113178333));
#70348=CARTESIAN_POINT('Ctrl Pts',(86.9958487821804,57.996428302522,11.3011805417272));
#70349=CARTESIAN_POINT('Ctrl Pts',(87.0272567431343,57.9916084654011,11.261182180699));
#70350=CARTESIAN_POINT('Ctrl Pts',(87.1222147346365,57.978141883981,11.1541481154597));
#70351=CARTESIAN_POINT('Ctrl Pts',(87.1907809981661,57.9696041795622,11.0920120775261));
#70352=CARTESIAN_POINT('Ctrl Pts',(87.2876959135263,57.9581433880395,11.0217371494635));
#70353=CARTESIAN_POINT('Ctrl Pts',(87.3104361379208,57.9554941484458,11.006347356427));
#70354=CARTESIAN_POINT('Ctrl Pts',(87.3429568488521,57.9517457394591,10.9858429456714));
#70355=CARTESIAN_POINT('Ctrl Pts',(87.3523338410237,57.9506694754437,10.9800995504004));
#70356=CARTESIAN_POINT('Ctrl Pts',(87.3688360722683,57.948782343433,10.9702843355352));
#70357=CARTESIAN_POINT('Ctrl Pts',(87.375928543253,57.9479734752513,10.9661583912467));
#70358=CARTESIAN_POINT('Ctrl Pts',(87.390958198284,57.9462636010808,10.9576089476924));
#70359=CARTESIAN_POINT('Ctrl Pts',(87.3989038260318,57.9453620824566,10.953201355333));
#70360=CARTESIAN_POINT('Ctrl Pts',(87.4182599298711,57.9431712081381,10.9427341729519));
#70361=CARTESIAN_POINT('Ctrl Pts',(87.4297166114248,57.941878834594,10.9367628683981));
#70362=CARTESIAN_POINT('Ctrl Pts',(87.4723077139112,57.9370883796243,10.9153839396885));
#70363=CARTESIAN_POINT('Ctrl Pts',(87.5039758057764,57.9335532532777,10.9010825882101));
#70364=CARTESIAN_POINT('Ctrl Pts',(87.5895634271671,57.92405495113,10.8665821096539));
#70365=CARTESIAN_POINT('Ctrl Pts',(87.644333837879,57.9180304225882,10.8487217945282));
#70366=CARTESIAN_POINT('Ctrl Pts',(87.7745554703628,57.9038826152027,10.8158448090695));
#70367=CARTESIAN_POINT('Ctrl Pts',(87.8505511980966,57.8957537821757,10.8038379996809));
#70368=CARTESIAN_POINT('Ctrl Pts',(87.9394594854289,57.8866215687176,10.7979568027595));
#70369=CARTESIAN_POINT('Ctrl Pts',(87.9517570443401,57.8853670215096,10.7973227722495));
#70370=CARTESIAN_POINT('Ctrl Pts',(87.9701744362412,57.883502703665,10.7966416274773));
#70371=CARTESIAN_POINT('Ctrl Pts',(87.9762879710333,57.8828862528051,10.7964597346695));
#70372=CARTESIAN_POINT('Ctrl Pts',(87.9873637270242,57.8817740447275,10.7962102734071));
#70373=CARTESIAN_POINT('Ctrl Pts',(87.9923252151887,57.8812775196486,10.7961276132986));
#70374=CARTESIAN_POINT('Ctrl Pts',(88.0036217064928,57.8801508037054,10.7960056342756));
#70375=CARTESIAN_POINT('Ctrl Pts',(88.0099566904224,57.8795216258223,10.7959846276501));
#70376=CARTESIAN_POINT('Ctrl Pts',(88.029754002933,57.8775629671159,10.7960671194802));
#70377=CARTESIAN_POINT('Ctrl Pts',(88.0432154353562,57.8762420915072,10.7963372682181));
#70378=CARTESIAN_POINT('Ctrl Pts',(88.0753857551097,57.873105788758,10.7974949073793));
#70379=CARTESIAN_POINT('Ctrl Pts',(88.0940848225632,57.8712992662735,10.7985822633269));
#70380=CARTESIAN_POINT('Ctrl Pts',(88.1682107234434,57.8641775894275,10.8045405053188));
#70381=CARTESIAN_POINT('Ctrl Pts',(88.2233200250708,57.8589694229288,10.8126378192746));
#70382=CARTESIAN_POINT('Ctrl Pts',(88.3565005736143,57.846208996109,10.841246474797));
#70383=CARTESIAN_POINT('Ctrl Pts',(88.4334745726621,57.8386726683573,10.8656233351135));
#70384=CARTESIAN_POINT('Ctrl Pts',(88.5236148066165,57.829216322951,10.9039207038179));
#70385=CARTESIAN_POINT('Ctrl Pts',(88.539473121397,57.8275282550573,10.9110461818542));
#70386=CARTESIAN_POINT('Ctrl Pts',(88.5651124000053,57.8247549217802,10.9232050474758));
#70387=CARTESIAN_POINT('Ctrl Pts',(88.5749835067088,57.8236762862583,10.9280441832448));
#70388=CARTESIAN_POINT('Ctrl Pts',(88.5926487836561,57.8217252859572,10.9369905714201));
#70389=CARTESIAN_POINT('Ctrl Pts',(88.6004655141809,57.8208545660127,10.9410520033975));
#70390=CARTESIAN_POINT('Ctrl Pts',(88.6171589828715,57.818978545179,10.9499473832506));
#70391=CARTESIAN_POINT('Ctrl Pts',(88.6260214504087,57.8179723996883,10.9548066071781));
#70392=CARTESIAN_POINT('Ctrl Pts',(88.6504021131356,57.8151753175194,10.9685553493259));
#70393=CARTESIAN_POINT('Ctrl Pts',(88.6657912235772,57.8133765580079,10.9776672414249));
#70394=CARTESIAN_POINT('Ctrl Pts',(88.6999225936818,57.8093088324409,10.9988623542658));
#70395=CARTESIAN_POINT('Ctrl Pts',(88.7185487882275,57.8070340833539,11.0111200760454));
#70396=CARTESIAN_POINT('Ctrl Pts',(88.7798653177869,57.799354787376,11.0538265292159));
#70397=CARTESIAN_POINT('Ctrl Pts',(88.8209863768143,57.7938812109666,11.0864237412434));
#70398=CARTESIAN_POINT('Ctrl Pts',(88.9236575888081,57.7793597596115,11.1787069624114));
#70399=CARTESIAN_POINT('Ctrl Pts',(88.9813974752437,57.7702681986845,11.2422497155887));
#70400=CARTESIAN_POINT('Ctrl Pts',(89.0390994169243,57.760330080863,11.3203176261556));
#70401=CARTESIAN_POINT('Ctrl Pts',(89.0457685290178,57.7591665785606,11.3296001507021));
#70402=CARTESIAN_POINT('Ctrl Pts',(89.0557532165843,57.7574029020035,11.3439010765878));
#70403=CARTESIAN_POINT('Ctrl Pts',(89.0591596966055,57.7567971728477,11.3488546907348));
#70404=CARTESIAN_POINT('Ctrl Pts',(89.0652903250764,57.7556999152783,11.3579066986006));
#70405=CARTESIAN_POINT('Ctrl Pts',(89.0680259161355,57.7552076742686,11.3619968549412));
#70406=CARTESIAN_POINT('Ctrl Pts',(89.0742824271566,57.7540756656837,11.371470052077));
#70407=CARTESIAN_POINT('Ctrl Pts',(89.077786328161,57.7534370185408,11.3768640880782));
#70408=CARTESIAN_POINT('Ctrl Pts',(89.0887826794301,57.7514168741067,11.3940771546875));
#70409=CARTESIAN_POINT('Ctrl Pts',(89.0961212788388,57.7500447680257,11.4059941791689));
#70410=CARTESIAN_POINT('Ctrl Pts',(89.1133297238051,57.7467614707615,11.4350019380987));
#70411=CARTESIAN_POINT('Ctrl Pts',(89.1230014481502,57.7448603427926,11.4522066463369));
#70412=CARTESIAN_POINT('Ctrl Pts',(89.1611440219771,57.7370923930166,11.5239208000006));
#70413=CARTESIAN_POINT('Ctrl Pts',(89.1860408894176,57.7313535011974,11.5802412803928));
#70414=CARTESIAN_POINT('Ctrl Pts',(89.2312269251569,57.7187869905285,11.7065275287635));
#70415=CARTESIAN_POINT('Ctrl Pts',(89.2497794423937,57.7119699055572,11.7768681740403));
#70416=CARTESIAN_POINT('Ctrl Pts',(89.265223803704,57.7032681522485,11.865675099231));
#70417=CARTESIAN_POINT('Ctrl Pts',(89.2678696946986,57.7015659162922,11.8830084263556));
#70418=CARTESIAN_POINT('Ctrl Pts',(89.2715949578838,57.6987741367308,11.9113321195205));
#70419=CARTESIAN_POINT('Ctrl Pts',(89.2728913664648,57.6976913750341,11.9222920966106));
#70420=CARTESIAN_POINT('Ctrl Pts',(89.274965734422,57.6957359435524,11.9420311416621));
#70421=CARTESIAN_POINT('Ctrl Pts',(89.2757954658817,57.6948649511802,11.9508041874718));
#70422=CARTESIAN_POINT('Ctrl Pts',(89.2773781971878,57.6929916887311,11.969626700734));
#70423=CARTESIAN_POINT('Ctrl Pts',(89.278103002836,57.6919885982722,11.979677834198));
#70424=CARTESIAN_POINT('Ctrl Pts',(89.2797733202122,57.689209211698,12.0074429575954));
#70425=CARTESIAN_POINT('Ctrl Pts',(89.280467371488,57.687425256254,12.0251689296196));
#70426=CARTESIAN_POINT('Ctrl Pts',(89.2811911548917,57.6833967562893,12.064959075668));
#70427=CARTESIAN_POINT('Ctrl Pts',(89.2810175744667,57.6811465977044,12.0870205909266));
#70428=CARTESIAN_POINT('Ctrl Pts',(89.2777098867373,57.6711249530162,12.184509763801));
#70429=CARTESIAN_POINT('Ctrl Pts',(89.2684289989737,57.6631891741562,12.2595644022451));
#70430=CARTESIAN_POINT('Ctrl Pts',(89.2518891570939,57.6549048247147,12.3363770794827));
#70431=CARTESIAN_POINT('Ctrl Pts',(89.2512235670153,57.6545770516432,12.3394139154327));
#70432=CARTESIAN_POINT('Ctrl Pts',(89.2369247911865,57.6476521657259,12.4035271822922));
#70433=CARTESIAN_POINT('Ctrl Pts',(89.2188047109582,57.6410708765688,12.4635253162702));
#70434=CARTESIAN_POINT('Ctrl Pts',(89.192775188052,57.6336680440243,12.5311940318788));
#70435=CARTESIAN_POINT('Ctrl Pts',(89.189111412272,57.6326619193675,12.5403960420601));
#70436=CARTESIAN_POINT('Ctrl Pts',(89.1831781482921,57.6310882645186,12.5548053101634));
#70437=CARTESIAN_POINT('Ctrl Pts',(89.1809808755076,57.6305167961573,12.5600414943702));
#70438=CARTESIAN_POINT('Ctrl Pts',(89.176772710023,57.6294435239744,12.5698841610954));
#70439=CARTESIAN_POINT('Ctrl Pts',(89.1747695724333,57.6289413293989,12.5744935038689));
#70440=CARTESIAN_POINT('Ctrl Pts',(89.1699147192715,57.6277444870236,12.5854858445216));
#70441=CARTESIAN_POINT('Ctrl Pts',(89.1670375636543,57.6270513722783,12.5918574226533));
#70442=CARTESIAN_POINT('Ctrl Pts',(89.1568422197554,57.624649370946,12.613947268851));
#70443=CARTESIAN_POINT('Ctrl Pts',(89.1492543679954,57.6229555565382,12.6295403298904));
#70444=CARTESIAN_POINT('Ctrl Pts',(89.1292329327532,57.6187008204597,12.6686287660051));
#70445=CARTESIAN_POINT('Ctrl Pts',(89.1163763078725,57.6161596508093,12.6918991995914));
#70446=CARTESIAN_POINT('Ctrl Pts',(89.0735902903707,57.6082124201461,12.763904737886));
#70447=CARTESIAN_POINT('Ctrl Pts',(89.0410952260603,57.602882921433,12.8110327169208));
#70448=CARTESIAN_POINT('Ctrl Pts',(88.9609866886082,57.5908046467616,12.9119054658519));
#70449=CARTESIAN_POINT('Ctrl Pts',(88.9117825183258,57.5840554810671,12.9641196130535));
#70450=CARTESIAN_POINT('Ctrl Pts',(88.8465890670682,57.5755692650659,13.0225272521232));
#70451=CARTESIAN_POINT('Ctrl Pts',(88.8345330716084,57.5740174217952,13.0329264184839));
#70452=CARTESIAN_POINT('Ctrl Pts',(88.8148251008043,57.5715054941576,13.0492900047145));
#70453=CARTESIAN_POINT('Ctrl Pts',(88.8072943459043,57.5705512955222,13.0553984676414));
#70454=CARTESIAN_POINT('Ctrl Pts',(88.7927285468054,57.5687158012079,13.0669392935383));
#70455=CARTESIAN_POINT('Ctrl Pts',(88.7857049368417,57.5678351130327,13.0723852348146));
#70456=CARTESIAN_POINT('Ctrl Pts',(88.7692927481366,57.5657867585359,13.0848372444535));
#70457=CARTESIAN_POINT('Ctrl Pts',(88.7598634212971,57.5646170214461,13.0917878801957));
#70458=CARTESIAN_POINT('Ctrl Pts',(88.7287948848014,57.5607844395237,13.1140327487044));
#70459=CARTESIAN_POINT('Ctrl Pts',(88.7067747408981,57.5581013777191,13.1287790841729));
#70460=CARTESIAN_POINT('Ctrl Pts',(88.6520895745806,57.5515102232162,13.1629723535767));
#70461=CARTESIAN_POINT('Ctrl Pts',(88.6189833787897,57.5475791426713,13.1816611231888));
#70462=CARTESIAN_POINT('Ctrl Pts',(88.5415196299343,57.5385138527237,13.2209178205029));
#70463=CARTESIAN_POINT('Ctrl Pts',(88.496711051912,57.5333630607269,13.2404660268192));
#70464=CARTESIAN_POINT('Ctrl Pts',(88.3922444390325,57.5216235072372,13.2790379285733));
#70465=CARTESIAN_POINT('Ctrl Pts',(88.3320695773349,57.5150490037439,13.2963353467067));
#70466=CARTESIAN_POINT('Ctrl Pts',(88.2611647219359,57.5076528329458,13.3111568782726));
#70467=CARTESIAN_POINT('Ctrl Pts',(88.2514487980308,57.5066469309627,13.3130695398332));
#70468=CARTESIAN_POINT('Ctrl Pts',(88.2361276606362,57.5050735464429,13.3158999053919));
#70469=CARTESIAN_POINT('Ctrl Pts',(88.2305373063819,57.5045021278631,13.3168939254882));
#70470=CARTESIAN_POINT('Ctrl Pts',(88.2199861028671,57.5034288918468,13.3186971180063));
#70471=CARTESIAN_POINT('Ctrl Pts',(88.2150270555444,57.5029266840923,13.3195143490282));
#70472=CARTESIAN_POINT('Ctrl Pts',(88.2031577874327,57.5017297331929,13.3213980514166));
#70473=CARTESIAN_POINT('Ctrl Pts',(88.1962433597143,57.5010365238713,13.3224369418294));
#70474=CARTESIAN_POINT('Ctrl Pts',(88.1721480599071,57.4986338122654,13.3258540086255));
#70475=CARTESIAN_POINT('Ctrl Pts',(88.1549260805346,57.4969393940372,13.3279374831467));
#70476=CARTESIAN_POINT('Ctrl Pts',(88.1112074005929,57.492682749731,13.3323196794481));
#70477=CARTESIAN_POINT('Ctrl Pts',(88.0846701814,57.4901402982706,13.3341403814033));
#70478=CARTESIAN_POINT('Ctrl Pts',(88.0012457782746,57.4822193999283,13.3372359749553));
#70479=CARTESIAN_POINT('Ctrl Pts',(87.9443178354556,57.4769164838844,13.3355236530341));
#70480=CARTESIAN_POINT('Ctrl Pts',(87.8161855663503,57.4648454525446,13.3230240240987));
#70481=CARTESIAN_POINT('Ctrl Pts',(87.7454105763784,57.4580766105689,13.3099941814995));
#70482=CARTESIAN_POINT('Ctrl Pts',(87.6607421340787,57.4495670288067,13.2868495923758));
#70483=CARTESIAN_POINT('Ctrl Pts',(87.6454411304861,57.4480126989241,13.2823556051771));
#70484=CARTESIAN_POINT('Ctrl Pts',(87.6209737679506,57.4454977360607,13.2746660706407));
#70485=CARTESIAN_POINT('Ctrl Pts',(87.6117519052563,57.4445430150088,13.2716513085726));
#70486=CARTESIAN_POINT('Ctrl Pts',(87.5941518556165,57.4427071675272,13.2656735330011));
#70487=CARTESIAN_POINT('Ctrl Pts',(87.5857684126008,57.4418266535634,13.2627276415808));
#70488=CARTESIAN_POINT('Ctrl Pts',(87.5772575048634,57.4409263455922,13.259636241344));
#70489=CARTESIAN_POINT('Ctrl Pts',(87.5770981816909,57.440909489639,13.259578334591));
#70490=CARTESIAN_POINT('Ctrl Pts',(87.5767956332609,57.4408774764845,13.2594683033642));
#70491=CARTESIAN_POINT('Ctrl Pts',(87.5766524056898,57.4408623194786,13.2594161849696));
#70492=CARTESIAN_POINT('Ctrl Pts',(87.57638033461,57.4408335241245,13.2593171268612));
#70493=CARTESIAN_POINT('Ctrl Pts',(87.5762514893518,57.4408198859451,13.2592701920743));
#70494=CARTESIAN_POINT('Ctrl Pts',(87.5760066664193,57.4407939687505,13.2591809648917));
#70495=CARTESIAN_POINT('Ctrl Pts',(87.5758906873032,57.440781689868,13.2591386764513));
#70496=CARTESIAN_POINT('Ctrl Pts',(87.5756702524212,57.4407583497771,13.2590582648125));
#70497=CARTESIAN_POINT('Ctrl Pts',(87.5755657954311,57.4407472886694,13.2590201447821));
#70498=CARTESIAN_POINT('Ctrl Pts',(87.5753672109313,57.4407262583743,13.2589476447566));
#70499=CARTESIAN_POINT('Ctrl Pts',(87.5752730825234,57.440716289278,13.2589132673536));
#70500=CARTESIAN_POINT('Ctrl Pts',(87.575094093768,57.4406973311302,13.2588478734002));
#70501=CARTESIAN_POINT('Ctrl Pts',(87.5750092326021,57.4406883421427,13.258816858913));
#70502=CARTESIAN_POINT('Ctrl Pts',(87.5748478326266,57.4406712444747,13.2587578520124));
#70503=CARTESIAN_POINT('Ctrl Pts',(87.574771293269,57.4406631358582,13.2587298613121));
#70504=CARTESIAN_POINT('Ctrl Pts',(87.574496330622,57.4406340042679,13.2586292765404));
#70505=CARTESIAN_POINT('Ctrl Pts',(87.5742979228688,57.4406129798909,13.2585566403617));
#70506=CARTESIAN_POINT('Ctrl Pts',(87.5636491170005,57.4394843814052,13.2546551469838));
#70507=CARTESIAN_POINT('Ctrl Pts',(87.5532499223203,57.4383722819139,13.2506892913613));
#70508=CARTESIAN_POINT('Ctrl Pts',(87.517424244737,57.4345051807202,13.2364846386856));
#70509=CARTESIAN_POINT('Ctrl Pts',(87.4922802822394,57.4317277149054,13.22556063883));
#70510=CARTESIAN_POINT('Ctrl Pts',(87.431207635568,57.4248152953361,13.1966433054023));
#70511=CARTESIAN_POINT('Ctrl Pts',(87.3957440674988,57.4206537988001,13.1777431587578));
#70512=CARTESIAN_POINT('Ctrl Pts',(87.320714236362,57.4115244271141,13.1330661438628));
#70513=CARTESIAN_POINT('Ctrl Pts',(87.2815667956405,57.4065487390504,13.1066975254403));
#70514=CARTESIAN_POINT('Ctrl Pts',(87.2223183995014,57.3987132783415,13.0618011373154));
#70515=CARTESIAN_POINT('Ctrl Pts',(87.2011957666037,57.3958534395397,13.0447006424742));
#70516=CARTESIAN_POINT('Ctrl Pts',(87.1806427720391,57.39301128552,13.0269406193793));
#70517=CARTESIAN_POINT('Origin',(88.011,66.41344859951,12.066));
#70518=CARTESIAN_POINT('',(87.1806428354357,56.4292380444866,13.0269406741609));
#70519=CARTESIAN_POINT('',(87.1801902653375,56.5998778161658,13.027459163232));
#70520=CARTESIAN_POINT('',(87.1806428354228,66.41344859951,13.0269406741497));
#70521=CARTESIAN_POINT('',(86.7410001292204,57.11575140049,12.0665729046198));
#70522=CARTESIAN_POINT('Ctrl Pts',(87.1806428354357,56.4292380444866,13.0269406741609));
#70523=CARTESIAN_POINT('Ctrl Pts',(87.1815511872673,56.4293562257376,13.0277255888508));
#70524=CARTESIAN_POINT('Ctrl Pts',(87.1824606515523,56.4294744595993,13.02850921516));
#70525=CARTESIAN_POINT('Ctrl Pts',(87.1900528136169,56.4304607079242,13.0350321539109));
#70526=CARTESIAN_POINT('Ctrl Pts',(87.1967937305493,56.4313314643143,13.0407028978344));
#70527=CARTESIAN_POINT('Ctrl Pts',(87.2114100591946,56.4332095500112,13.0527413484288));
#70528=CARTESIAN_POINT('Ctrl Pts',(87.2193036744075,56.4342177386951,13.0590858346253));
#70529=CARTESIAN_POINT('Ctrl Pts',(87.2414157120846,56.4370260473583,13.0764271888448));
#70530=CARTESIAN_POINT('Ctrl Pts',(87.2557923142829,56.4388340924591,13.0872170908351));
#70531=CARTESIAN_POINT('Ctrl Pts',(87.28862355028,56.4429263515667,13.1107851134188));
#70532=CARTESIAN_POINT('Ctrl Pts',(87.3071972126167,56.4452164544235,13.1233859979102));
#70533=CARTESIAN_POINT('Ctrl Pts',(87.3707427042797,56.452972877426,13.1640809353309));
#70534=CARTESIAN_POINT('Ctrl Pts',(87.417132463637,56.4585097847843,13.1898465303408));
#70535=CARTESIAN_POINT('Ctrl Pts',(87.5413048325652,56.4729796596785,13.2489754893543));
#70536=CARTESIAN_POINT('Ctrl Pts',(87.6210640173552,56.4819508507898,13.2776094421537));
#70537=CARTESIAN_POINT('Ctrl Pts',(87.7142942650251,56.4917905927181,13.3009085854228));
#70538=CARTESIAN_POINT('Ctrl Pts',(87.7255424902289,56.4929671037451,13.3035570902417));
#70539=CARTESIAN_POINT('Ctrl Pts',(87.7427225727965,56.4947464615107,13.3073555861693));
#70540=CARTESIAN_POINT('Ctrl Pts',(87.7486285925255,56.4953550064515,13.3086172859344));
#70541=CARTESIAN_POINT('Ctrl Pts',(87.7589211146403,56.4964098185702,13.3107394155931));
#70542=CARTESIAN_POINT('Ctrl Pts',(87.763303331121,56.4968571092307,13.3116188580882));
#70543=CARTESIAN_POINT('Ctrl Pts',(87.7737338532045,56.4979174911731,13.3136548765408));
#70544=CARTESIAN_POINT('Ctrl Pts',(87.7797860715061,56.4985294073228,13.3147906311591));
#70545=CARTESIAN_POINT('Ctrl Pts',(87.798170789801,56.5003787364104,13.3181024491282));
#70546=CARTESIAN_POINT('Ctrl Pts',(87.8105280501107,56.5016088575653,13.3201402857987));
#70547=CARTESIAN_POINT('Ctrl Pts',(87.8734755865306,56.5078195991908,13.3295667018586));
#70548=CARTESIAN_POINT('Ctrl Pts',(87.9244566752159,56.5126690358122,13.3340795605586));
#70549=CARTESIAN_POINT('Ctrl Pts',(88.068776159048,56.5262552720969,13.338106285534));
#70550=CARTESIAN_POINT('Ctrl Pts',(88.161968475598,56.5348821836411,13.3304364123718));
#70551=CARTESIAN_POINT('Ctrl Pts',(88.2795181168433,56.5463561243396,13.3075722809627));
#70552=CARTESIAN_POINT('Ctrl Pts',(88.3053902625239,56.5489176527014,13.3016932675965));
#70553=CARTESIAN_POINT('Ctrl Pts',(88.3415556306588,56.5525624846962,13.2922751172882));
#70554=CARTESIAN_POINT('Ctrl Pts',(88.3520180386733,56.5536245666161,13.2894068693012));
#70555=CARTESIAN_POINT('Ctrl Pts',(88.3710805309575,56.5555746554578,13.2839174123201));
#70556=CARTESIAN_POINT('Ctrl Pts',(88.3796920879425,56.5564612599687,13.2813382022595));
#70557=CARTESIAN_POINT('Ctrl Pts',(88.3971399866615,56.5582696339004,13.2759099553706));
#70558=CARTESIAN_POINT('Ctrl Pts',(88.4059738930652,56.5591915467965,13.273055011795));
#70559=CARTESIAN_POINT('Ctrl Pts',(88.427980633579,56.5615046675162,13.2656754300987));
#70560=CARTESIAN_POINT('Ctrl Pts',(88.4411114200283,56.5628997414632,13.2610305908167));
#70561=CARTESIAN_POINT('Ctrl Pts',(88.4950705603822,56.5686972339007,13.2409387988065));
#70562=CARTESIAN_POINT('Ctrl Pts',(88.5351594801019,56.5731604493787,13.2236101231282));
#70563=CARTESIAN_POINT('Ctrl Pts',(88.6550509179425,56.5870181018942,13.1642812294383));
#70564=CARTESIAN_POINT('Ctrl Pts',(88.7313401164117,56.5965839800609,13.1158237683423));
#70565=CARTESIAN_POINT('Ctrl Pts',(88.8316699345391,56.6100211258957,13.0359760959231));
#70566=CARTESIAN_POINT('Ctrl Pts',(88.8604138833674,56.6139832281062,13.0109072124338));
#70567=CARTESIAN_POINT('Ctrl Pts',(88.8947441243965,56.6188233342398,12.9781313070374));
#70568=CARTESIAN_POINT('Ctrl Pts',(88.9014272748383,56.619770959051,12.9716083511424));
#70569=CARTESIAN_POINT('Ctrl Pts',(88.9119317794159,56.6212682881089,12.9611269083194));
#70570=CARTESIAN_POINT('Ctrl Pts',(88.9158001990069,56.6218214336459,12.9572165041569));
#70571=CARTESIAN_POINT('Ctrl Pts',(88.9232033273231,56.6228831691662,12.949635137332));
#70572=CARTESIAN_POINT('Ctrl Pts',(88.9267414104244,56.6233919845579,12.9459679753269));
#70573=CARTESIAN_POINT('Ctrl Pts',(88.9353709620412,56.6246367395389,12.936915177881));
#70574=CARTESIAN_POINT('Ctrl Pts',(88.94043759056,56.625370810856,12.9315060355751));
#70575=CARTESIAN_POINT('Ctrl Pts',(88.9591665802194,56.6280980695201,12.9111567782944));
#70576=CARTESIAN_POINT('Ctrl Pts',(88.9725196154335,56.6300702256156,12.8959337553049));
#70577=CARTESIAN_POINT('Ctrl Pts',(89.0068866129423,56.6352432759506,12.854810312601));
#70578=CARTESIAN_POINT('Ctrl Pts',(89.0272552931815,56.6384118770012,12.8283893311679));
#70579=CARTESIAN_POINT('Ctrl Pts',(89.1129641916995,56.6523823990047,12.7076636042831));
#70580=CARTESIAN_POINT('Ctrl Pts',(89.1663826697847,56.6629334106132,12.6055791584121));
#70581=CARTESIAN_POINT('Ctrl Pts',(89.2113684280754,56.6757324723813,12.4811227602697));
#70582=CARTESIAN_POINT('Ctrl Pts',(89.2170190434689,56.6774487608568,12.4644084126889));
#70583=CARTESIAN_POINT('Ctrl Pts',(89.2253718145597,56.680171217308,12.4378928704803));
#70584=CARTESIAN_POINT('Ctrl Pts',(89.2283077698893,56.6811697417268,12.4281670742206));
#70585=CARTESIAN_POINT('Ctrl Pts',(89.2335701637644,56.6830409375251,12.4099472921285));
#70586=CARTESIAN_POINT('Ctrl Pts',(89.2359255607343,56.6839126104301,12.4014622271366));
#70587=CARTESIAN_POINT('Ctrl Pts',(89.2410055301142,56.6858724356546,12.3823949965554));
#70588=CARTESIAN_POINT('Ctrl Pts',(89.243682101606,56.686962063142,12.3718009404115));
#70589=CARTESIAN_POINT('Ctrl Pts',(89.2513401418302,56.6902613880028,12.3397541697793));
#70590=CARTESIAN_POINT('Ctrl Pts',(89.2559002857052,56.6924842041352,12.3182065353659));
#70591=CARTESIAN_POINT('Ctrl Pts',(89.277099381309,56.7043641161924,12.2033717274388));
#70592=CARTESIAN_POINT('Ctrl Pts',(89.283814830232,56.7143213038455,12.1085783189939));
#70593=CARTESIAN_POINT('Ctrl Pts',(89.2774131806424,56.7307848237239,11.9525263008568));
#70594=CARTESIAN_POINT('Ctrl Pts',(89.2704373403079,56.7372463275319,11.8913616833031));
#70595=CARTESIAN_POINT('Ctrl Pts',(89.2572077847251,56.7445439320123,11.8211206657119));
#70596=CARTESIAN_POINT('Ctrl Pts',(89.2552435678475,56.7455583684757,11.8113282552207));
#70597=CARTESIAN_POINT('Ctrl Pts',(89.2519895677624,56.7471362590663,11.7960431482084));
#70598=CARTESIAN_POINT('Ctrl Pts',(89.2507784352414,56.747703784987,11.7905344936574));
#70599=CARTESIAN_POINT('Ctrl Pts',(89.2484157682736,56.7487744064457,11.7801195884816));
#70600=CARTESIAN_POINT('Ctrl Pts',(89.2472717218303,56.749277857102,11.7752120617999));
#70601=CARTESIAN_POINT('Ctrl Pts',(89.2444513814456,56.7504841602544,11.7634314403725));
#70602=CARTESIAN_POINT('Ctrl Pts',(89.2427468109817,56.7511854139932,11.7565652800296));
#70603=CARTESIAN_POINT('Ctrl Pts',(89.2365318593605,56.7536486317145,11.7323963864265));
#70604=CARTESIAN_POINT('Ctrl Pts',(89.2317132139794,56.7553944840277,11.7151737242088));
#70605=CARTESIAN_POINT('Ctrl Pts',(89.2221507136994,56.7585898176861,11.683583163453));
#70606=CARTESIAN_POINT('Ctrl Pts',(89.2175110253315,56.7600431603729,11.669187842766));
#70607=CARTESIAN_POINT('Ctrl Pts',(89.1916654882579,56.7676732158,11.5936472835332));
#70608=CARTESIAN_POINT('Ctrl Pts',(89.1660643855557,56.7737036474884,11.5341015580417));
#70609=CARTESIAN_POINT('Ctrl Pts',(89.1041244740852,56.7862162170744,11.4158395538987));
#70610=CARTESIAN_POINT('Ctrl Pts',(89.0673251822746,56.7926839817483,11.3576183468105));
#70611=CARTESIAN_POINT('Ctrl Pts',(89.0155538552522,56.8010007094916,11.2887783067108));
#70612=CARTESIAN_POINT('Ctrl Pts',(89.0048252187677,56.80268816811,11.2751059649097));
#70613=CARTESIAN_POINT('Ctrl Pts',(88.9868578765319,56.8054608260815,11.2531517693297));
#70614=CARTESIAN_POINT('Ctrl Pts',(88.979785829117,56.8065394030033,11.2447358281463));
#70615=CARTESIAN_POINT('Ctrl Pts',(88.9668504630952,56.8084905100742,11.2297419545109));
#70616=CARTESIAN_POINT('Ctrl Pts',(88.9610261505693,56.8093613969358,11.2231311313195));
#70617=CARTESIAN_POINT('Ctrl Pts',(88.9483707781329,56.8112380190129,11.2090646071677));
#70618=CARTESIAN_POINT('Ctrl Pts',(88.9415185688234,56.8122446009229,11.2016288869434));
#70619=CARTESIAN_POINT('Ctrl Pts',(88.922293351752,56.8150435859577,11.1812600555145));
#70620=CARTESIAN_POINT('Ctrl Pts',(88.9097352072485,56.8168438273645,11.1685061082928));
#70621=CARTESIAN_POINT('Ctrl Pts',(88.8809212502997,56.8209153706759,11.1404541520472));
#70622=CARTESIAN_POINT('Ctrl Pts',(88.8645236180995,56.82319247096,11.1253112215245));
#70623=CARTESIAN_POINT('Ctrl Pts',(88.808229237616,56.8308831827854,11.0760082731423));
#70624=CARTESIAN_POINT('Ctrl Pts',(88.7666189437846,56.8363660484672,11.0438959697772));
#70625=CARTESIAN_POINT('Ctrl Pts',(88.6523829906287,56.8508794034788,10.9665310282105));
#70626=CARTESIAN_POINT('Ctrl Pts',(88.576956394807,56.8599527445137,10.9258682105593));
#70627=CARTESIAN_POINT('Ctrl Pts',(88.4874361105472,56.8698760798227,10.8886981260928));
#70628=CARTESIAN_POINT('Ctrl Pts',(88.47680319907,56.8710416412169,10.8844508124563));
#70629=CARTESIAN_POINT('Ctrl Pts',(88.4604967090254,56.872807863575,10.87819155285));
#70630=CARTESIAN_POINT('Ctrl Pts',(88.4548643135275,56.8734141015865,10.8760753489535));
#70631=CARTESIAN_POINT('Ctrl Pts',(88.4445976881036,56.8745119476096,10.8723010155149));
#70632=CARTESIAN_POINT('Ctrl Pts',(88.4399687211188,56.8750042716023,10.8706297395365));
#70633=CARTESIAN_POINT('Ctrl Pts',(88.4292705109998,56.8761360654688,10.8668373300499));
#70634=CARTESIAN_POINT('Ctrl Pts',(88.4231947097598,56.8767744179401,10.8647353092673));
#70635=CARTESIAN_POINT('Ctrl Pts',(88.4038644024565,56.8787921894322,10.8582116152764));
#70636=CARTESIAN_POINT('Ctrl Pts',(88.3905520089413,56.8801622498778,10.853962231432));
#70637=CARTESIAN_POINT('Ctrl Pts',(88.3583164420102,56.8834395398326,10.8442557455046));
#70638=CARTESIAN_POINT('Ctrl Pts',(88.3393306429984,56.8853367562984,10.8390171761421));
#70639=CARTESIAN_POINT('Ctrl Pts',(88.2608402413683,56.8930763748795,10.8193127169733));
#70640=CARTESIAN_POINT('Ctrl Pts',(88.2004448760899,56.8987918110998,10.8087166378623));
#70641=CARTESIAN_POINT('Ctrl Pts',(88.0668823765914,56.9113697479765,10.7951312845081));
#70642=CARTESIAN_POINT('Ctrl Pts',(87.9937585890848,56.9182218578444,10.7940210878684));
#70643=CARTESIAN_POINT('Ctrl Pts',(87.9034902106471,56.9269583025082,10.8004376383025));
#70644=CARTESIAN_POINT('Ctrl Pts',(87.8860572339359,56.9286578986099,10.8020396835717));
#70645=CARTESIAN_POINT('Ctrl Pts',(87.8577038196236,56.9314463602381,10.8052375590161));
#70646=CARTESIAN_POINT('Ctrl Pts',(87.8467607381644,56.9325284732268,10.8066163818838));
#70647=CARTESIAN_POINT('Ctrl Pts',(87.8271082537827,56.9344833750762,10.809353072017));
#70648=CARTESIAN_POINT('Ctrl Pts',(87.8183922627767,56.9353544927229,10.8106594383987));
#70649=CARTESIAN_POINT('Ctrl Pts',(87.7997326026262,56.937228737766,10.8136550757421));
#70650=CARTESIAN_POINT('Ctrl Pts',(87.7897941322235,56.93823269103,10.8153722890039));
#70651=CARTESIAN_POINT('Ctrl Pts',(87.7624008597505,56.9410164452931,10.820442147622));
#70652=CARTESIAN_POINT('Ctrl Pts',(87.7449951996424,56.9428039436267,10.8240429716981));
#70653=CARTESIAN_POINT('Ctrl Pts',(87.7159670845498,56.9458184727898,10.8306863726074));
#70654=CARTESIAN_POINT('Ctrl Pts',(87.7043013317597,56.9470390898627,10.8335309003409));
#70655=CARTESIAN_POINT('Ctrl Pts',(87.6738372558035,56.9502512670543,10.8414184145493));
#70656=CARTESIAN_POINT('Ctrl Pts',(87.6551122308213,56.9522504976668,10.846728670482));
#70657=CARTESIAN_POINT('Ctrl Pts',(87.5661396781767,56.9618711431419,10.87418456361));
#70658=CARTESIAN_POINT('Ctrl Pts',(87.497792659662,56.9696388136903,10.9019810114289));
#70659=CARTESIAN_POINT('Ctrl Pts',(87.380654283355,56.9835060490229,10.9619510911352));
#70660=CARTESIAN_POINT('Ctrl Pts',(87.3309203679017,56.9895902603073,10.9918708256271));
#70661=CARTESIAN_POINT('Ctrl Pts',(87.2752451129141,56.9965266414844,11.0307880888301));
#70662=CARTESIAN_POINT('Ctrl Pts',(87.2671586809928,56.9975372967341,11.0365831411089));
#70663=CARTESIAN_POINT('Ctrl Pts',(87.2545559664893,56.9991165231332,11.0458408032338));
#70664=CARTESIAN_POINT('Ctrl Pts',(87.2499937151712,56.9996890753513,11.0492395554058));
#70665=CARTESIAN_POINT('Ctrl Pts',(87.241573299093,57.0007472135728,11.0556009646502));
#70666=CARTESIAN_POINT('Ctrl Pts',(87.2377092603258,57.0012333071786,11.0585551665479));
#70667=CARTESIAN_POINT('Ctrl Pts',(87.2337880173248,57.0017272171201,11.0615889572738));
#70668=CARTESIAN_POINT('Ctrl Pts',(87.2337139793801,57.0017365429841,11.0616462521038));
#70669=CARTESIAN_POINT('Ctrl Pts',(87.2335669763132,57.0017550600373,11.0617600375427));
#70670=CARTESIAN_POINT('Ctrl Pts',(87.233494010923,57.0017642512537,11.0618165279868));
#70671=CARTESIAN_POINT('Ctrl Pts',(87.2333490519652,57.0017825117164,11.0619287817524));
#70672=CARTESIAN_POINT('Ctrl Pts',(87.23327705826,57.0017915809741,11.0619845448481));
#70673=CARTESIAN_POINT('Ctrl Pts',(87.2331339478638,57.0018096094471,11.0620954163724));
#70674=CARTESIAN_POINT('Ctrl Pts',(87.2330628309948,57.0018185686795,11.0621505246429));
#70675=CARTESIAN_POINT('Ctrl Pts',(87.2329213841737,57.001836388438,11.0622601554622));
#70676=CARTESIAN_POINT('Ctrl Pts',(87.2328510542875,57.0018452489512,11.0623146776975));
#70677=CARTESIAN_POINT('Ctrl Pts',(87.2327110965624,57.0018628819512,11.0624232014688));
#70678=CARTESIAN_POINT('Ctrl Pts',(87.2326414686106,57.0018716544482,11.0624772028611));
#70679=CARTESIAN_POINT('Ctrl Pts',(87.2325028341706,57.0018891215579,11.0625847467652));
#70680=CARTESIAN_POINT('Ctrl Pts',(87.2324338274016,57.0018978162023,11.0626382892923));
#70681=CARTESIAN_POINT('Ctrl Pts',(87.2322963576771,57.0019151373814,11.0627449751213));
#70682=CARTESIAN_POINT('Ctrl Pts',(87.2322278947359,57.0019237639109,11.0627981182365));
#70683=CARTESIAN_POINT('Ctrl Pts',(87.2320914388658,57.0019409581515,11.0629040620147));
#70684=CARTESIAN_POINT('Ctrl Pts',(87.2320234458504,57.0019495258705,11.0629568625945));
#70685=CARTESIAN_POINT('Ctrl Pts',(87.2318878586206,57.0019666114566,11.0630621761636));
#70686=CARTESIAN_POINT('Ctrl Pts',(87.2318202644013,57.001975129322,11.0631146890302));
#70687=CARTESIAN_POINT('Ctrl Pts',(87.231685406248,57.0019921238291,11.0632194800344));
#70688=CARTESIAN_POINT('Ctrl Pts',(87.2316181422467,57.0020006004775,11.0632717581207));
#70689=CARTESIAN_POINT('Ctrl Pts',(87.2262199904002,57.0026808945831,11.0674681135403));
#70690=CARTESIAN_POINT('Ctrl Pts',(87.2209220133654,57.0033498074512,11.0716548012747));
#70691=CARTESIAN_POINT('Ctrl Pts',(87.2091727749076,57.0048367223819,11.0810927524063));
#70692=CARTESIAN_POINT('Ctrl Pts',(87.2027391198258,57.0056533074955,11.0863656052262));
#70693=CARTESIAN_POINT('Ctrl Pts',(87.1845444142284,57.0079711291973,11.1015787887414));
#70694=CARTESIAN_POINT('Ctrl Pts',(87.1729111597567,57.0094633622371,11.1116707744877));
#70695=CARTESIAN_POINT('Ctrl Pts',(87.132071215514,57.0147521969192,11.1484229071398));
#70696=CARTESIAN_POINT('Ctrl Pts',(87.1039270099763,57.0184914708578,11.1762344201138));
#70697=CARTESIAN_POINT('Ctrl Pts',(87.0096790725315,57.0315680303241,11.2784972559531));
#70698=CARTESIAN_POINT('Ctrl Pts',(86.9510769971634,57.0407763206326,11.3593425295514));
#70699=CARTESIAN_POINT('Ctrl Pts',(86.8922110294999,57.0523963269993,11.4646208053566));
#70700=CARTESIAN_POINT('Ctrl Pts',(86.8823696485452,57.054443771096,11.4833001588955));
#70701=CARTESIAN_POINT('Ctrl Pts',(86.8681652021713,57.0575717417811,11.5119718515118));
#70702=CARTESIAN_POINT('Ctrl Pts',(86.8634572903073,57.0586403185192,11.5217902281683));
#70703=CARTESIAN_POINT('Ctrl Pts',(86.8551724281082,57.0605807851163,11.5396539860567));
#70704=CARTESIAN_POINT('Ctrl Pts',(86.8515517395434,57.0614511107281,11.5476784552092));
#70705=CARTESIAN_POINT('Ctrl Pts',(86.8439215543373,57.0633349035371,11.5650691697909));
#70706=CARTESIAN_POINT('Ctrl Pts',(86.8399407961342,57.0643492786296,11.5744472352828));
#70707=CARTESIAN_POINT('Ctrl Pts',(86.8291378979728,57.0671935874465,11.6007734547568));
#70708=CARTESIAN_POINT('Ctrl Pts',(86.8225683495071,57.0690317855879,11.6178215873962));
#70709=CARTESIAN_POINT('Ctrl Pts',(86.8085890649151,57.0732043169257,11.6565692746366));
#70710=CARTESIAN_POINT('Ctrl Pts',(86.8013949242058,57.0755448968069,11.6783391039054));
#70711=CARTESIAN_POINT('Ctrl Pts',(86.7590701631882,57.0906623334501,11.8190943868847));
#70712=CARTESIAN_POINT('Ctrl Pts',(86.7409544477374,57.1039345767614,11.9424578425332));
#70713=CARTESIAN_POINT('Ctrl Pts',(86.7410000860046,57.1167707803686,12.0664673881771));
#70714=CARTESIAN_POINT('Ctrl Pts',(87.1806428354228,57.224088141927,13.0269406741497));
#70715=CARTESIAN_POINT('Ctrl Pts',(87.1431026657818,57.219153579792,12.994501888219));
#70716=CARTESIAN_POINT('Ctrl Pts',(87.1074198120016,57.214219017657,12.9598198990021));
#70717=CARTESIAN_POINT('Ctrl Pts',(87.073869362273,57.209284455522,12.9231383597958));
#70718=CARTESIAN_POINT('Ctrl Pts',(87.04034089956,57.2043531272124,12.886480859539));
#70719=CARTESIAN_POINT('Ctrl Pts',(87.0089424419052,57.1994217989027,12.8478268082961));
#70720=CARTESIAN_POINT('Ctrl Pts',(86.9799121855865,57.1944904705931,12.8074566197479));
#70721=CARTESIAN_POINT('Ctrl Pts',(86.9508886015368,57.1895602756922,12.7670957098211));
#70722=CARTESIAN_POINT('Ctrl Pts',(86.924232458129,57.1846300807914,12.725019890116));
#70723=CARTESIAN_POINT('Ctrl Pts',(86.900140007665,57.1796998858906,12.6815404758661));
#70724=CARTESIAN_POINT('Ctrl Pts',(86.8760251392384,57.1747651034563,12.6380206041341));
#70725=CARTESIAN_POINT('Ctrl Pts',(86.8544789949268,57.1698303210219,12.593095009375));
#70726=CARTESIAN_POINT('Ctrl Pts',(86.8356520955675,57.1648955385875,12.547100097221));
#70727=CARTESIAN_POINT('Ctrl Pts',(86.8168161701501,57.1599583903025,12.5010831340251));
#70728=CARTESIAN_POINT('Ctrl Pts',(86.8007022656137,57.1550212420174,12.4539963510136));
#70729=CARTESIAN_POINT('Ctrl Pts',(86.7874116183649,57.1500840937324,12.4061932867174));
#70730=CARTESIAN_POINT('Ctrl Pts',(86.7740954976792,57.1451374826926,12.3582986009734));
#70731=CARTESIAN_POINT('Ctrl Pts',(86.763613555933,57.1401908716528,12.3096854290717));
#70732=CARTESIAN_POINT('Ctrl Pts',(86.7560159808755,57.135244260613,12.2607180313741));
#70733=CARTESIAN_POINT('Ctrl Pts',(86.7510039867034,57.1319810634065,12.2284150518008));
#70734=CARTESIAN_POINT('Ctrl Pts',(86.7472461472918,57.1287178662,12.1959580826879));
#70735=CARTESIAN_POINT('Ctrl Pts',(86.7447444544907,57.1254546689935,12.1634520059662));
#70736=CARTESIAN_POINT('Ctrl Pts',(86.7422648212326,57.122220246159,12.1312325628387));
#70737=CARTESIAN_POINT('Ctrl Pts',(86.741014719967,57.1189858233245,12.0989172875295));
#70738=CARTESIAN_POINT('Ctrl Pts',(86.7410001292204,57.11575140049,12.0665729046198));
#70739=CARTESIAN_POINT('',(86.741302287513,57.2853233247604,12.0648429798974));
#70740=CARTESIAN_POINT('Ctrl Pts',(87.1806427720391,57.39301128552,13.0269406193793));
#70741=CARTESIAN_POINT('Ctrl Pts',(87.1553383036075,57.3895120778282,13.0050748059897));
#70742=CARTESIAN_POINT('Ctrl Pts',(87.130897297411,57.3860395939098,12.9822092877968));
#70743=CARTESIAN_POINT('Ctrl Pts',(87.1003752687152,57.3816048880979,12.951303306484));
#70744=CARTESIAN_POINT('Ctrl Pts',(87.0934548898731,57.380592441693,12.9441288852476));
#70745=CARTESIAN_POINT('Ctrl Pts',(87.0827551723581,57.3790170195409,12.932771766008));
#70746=CARTESIAN_POINT('Ctrl Pts',(87.0789182319904,57.3784499909106,12.9286443859873));
#70747=CARTESIAN_POINT('Ctrl Pts',(87.071702328246,57.3773798609861,12.9207779115088));
#70748=CARTESIAN_POINT('Ctrl Pts',(87.0683181018931,57.3768764080165,12.9170442027784));
#70749=CARTESIAN_POINT('Ctrl Pts',(87.0615779363064,57.3758703508852,12.9095184541659));
#70750=CARTESIAN_POINT('Ctrl Pts',(87.0582223626842,57.375367776353,12.9057263926896));
#70751=CARTESIAN_POINT('Ctrl Pts',(87.0470226873618,57.3736841405164,12.8929163134874));
#70752=CARTESIAN_POINT('Ctrl Pts',(87.0392828130171,57.3725102202813,12.8838071868842));
#70753=CARTESIAN_POINT('Ctrl Pts',(87.0161273608067,57.3689608556031,12.8557623299108));
#70754=CARTESIAN_POINT('Ctrl Pts',(87.0011270807996,57.366609459068,12.8364888286805));
#70755=CARTESIAN_POINT('Ctrl Pts',(86.9453243625591,57.3575976606582,12.7603569668231));
#70756=CARTESIAN_POINT('Ctrl Pts',(86.9086895230378,57.3510928680953,12.7005939910778));
#70757=CARTESIAN_POINT('Ctrl Pts',(86.8463003710983,57.3380992105503,12.5769483952262));
#70758=CARTESIAN_POINT('Ctrl Pts',(86.8204429801723,57.3316335620714,12.5133979409689));
#70759=CARTESIAN_POINT('Ctrl Pts',(86.7950974118727,57.3234639864447,12.433054688005));
#70760=CARTESIAN_POINT('Ctrl Pts',(86.7906375339432,57.3219279546698,12.4179426751307));
#70761=CARTESIAN_POINT('Ctrl Pts',(86.7838981927346,57.3194353245459,12.3934362663027));
#70762=CARTESIAN_POINT('Ctrl Pts',(86.7814427149337,57.3184844464329,12.3840915336714));
#70763=CARTESIAN_POINT('Ctrl Pts',(86.7769310749471,57.3166511485781,12.3660884390914));
#70764=CARTESIAN_POINT('Ctrl Pts',(86.7748588212056,57.3157693045291,12.3574346562902));
#70765=CARTESIAN_POINT('Ctrl Pts',(86.7709385374589,57.3140184255622,12.3402689007293));
#70766=CARTESIAN_POINT('Ctrl Pts',(86.7690868004028,57.3131495617903,12.3317582655975));
#70767=CARTESIAN_POINT('Ctrl Pts',(86.7649972548701,57.31112870839,12.3119857512116));
#70768=CARTESIAN_POINT('Ctrl Pts',(86.7628243923142,57.3099747312008,12.3007114416505));
#70769=CARTESIAN_POINT('Ctrl Pts',(86.7564581425606,57.3063219826306,12.2650860617795));
#70770=CARTESIAN_POINT('Ctrl Pts',(86.7528226881776,57.3038063742123,12.2406429863579));
#70771=CARTESIAN_POINT('Ctrl Pts',(86.7439255923012,57.2960797842203,12.1658978510959));
#70772=CARTESIAN_POINT('Ctrl Pts',(86.7409538637996,57.2908087994244,12.1153800774798));
#70773=CARTESIAN_POINT('Ctrl Pts',(86.7410005413785,57.2854959741782,12.0648273530155));
#70774=CARTESIAN_POINT('Ctrl Pts',(86.741302287513,57.2853233247604,12.0648429798974));
#70775=CARTESIAN_POINT('Ctrl Pts',(86.7403266859258,57.2744592453481,11.9555843196995));
#70776=CARTESIAN_POINT('Ctrl Pts',(86.8032502164186,57.2215904177746,11.4249961153898));
#70777=CARTESIAN_POINT('Ctrl Pts',(87.5455254130428,57.1267168420401,10.6389244339282));
#70778=CARTESIAN_POINT('Ctrl Pts',(88.9574435553591,57.0007025975569,10.9009009231395));
#70779=CARTESIAN_POINT('Ctrl Pts',(89.503174214425,56.8746883530736,12.2291789698061));
#70780=CARTESIAN_POINT('Ctrl Pts',(88.6832633409927,56.7486741085905,13.4081152196214));
#70781=CARTESIAN_POINT('Ctrl Pts',(87.6399969614201,56.6570705962878,13.3722260259654));
#70782=CARTESIAN_POINT('Ctrl Pts',(87.2373685545725,56.6074718321463,13.0778629352728));
#70783=CARTESIAN_POINT('Ctrl Pts',(87.1801902653375,56.5998778161658,13.027459163232));
#70784=CARTESIAN_POINT('Origin',(88.011,66.41344859951,12.066));
#70785=CARTESIAN_POINT('',(87.1806428950462,55.6371283284805,13.0269407256708));
#70786=CARTESIAN_POINT('',(87.1806428354183,55.8074024841729,13.0269406741458));
#70787=CARTESIAN_POINT('',(87.1806428354228,66.41344859951,13.0269406741497));
#70788=CARTESIAN_POINT('Ctrl Pts',(87.1806428950461,55.6371283284805,13.0269407256708));
#70789=CARTESIAN_POINT('Ctrl Pts',(87.1966575417485,55.6391162742572,13.0407791189425));
#70790=CARTESIAN_POINT('Ctrl Pts',(87.2130232902582,55.6410993381051,13.0542216369932));
#70791=CARTESIAN_POINT('Ctrl Pts',(87.2478415693537,55.6452363319383,13.081390173289));
#70792=CARTESIAN_POINT('Ctrl Pts',(87.2663373127494,55.6473886266094,13.0950313153536));
#70793=CARTESIAN_POINT('Ctrl Pts',(87.3191680343155,55.6534388570993,13.1318249117389));
#70794=CARTESIAN_POINT('Ctrl Pts',(87.3542771147909,55.657349514506,13.1538091366578));
#70795=CARTESIAN_POINT('Ctrl Pts',(87.4072461824863,55.6631616021996,13.1834768011556));
#70796=CARTESIAN_POINT('Ctrl Pts',(87.4243101697615,55.665021097995,13.192529196605));
#70797=CARTESIAN_POINT('Ctrl Pts',(87.452084004179,55.668033214733,13.2064609551837));
#70798=CARTESIAN_POINT('Ctrl Pts',(87.4626673270561,55.6691776882719,13.2115869844028));
#70799=CARTESIAN_POINT('Ctrl Pts',(87.4830153913326,55.6713732144237,13.2210960066511));
#70800=CARTESIAN_POINT('Ctrl Pts',(87.4927673989274,55.6724233294133,13.2255039825563));
#70801=CARTESIAN_POINT('Ctrl Pts',(87.5028839742889,55.6735110211033,13.2299236311476));
#70802=CARTESIAN_POINT('Ctrl Pts',(87.5031944163985,55.6735443969063,13.2300591067428));
#70803=CARTESIAN_POINT('Ctrl Pts',(87.5038529905149,55.6736151971493,13.2303461920546));
#70804=CARTESIAN_POINT('Ctrl Pts',(87.504201136306,55.6736526226567,13.2304977698301));
#70805=CARTESIAN_POINT('Ctrl Pts',(87.5047096317478,55.673707282742,13.2307188903608));
#70806=CARTESIAN_POINT('Ctrl Pts',(87.5048699282408,55.6737245131886,13.2307885563523));
#70807=CARTESIAN_POINT('Ctrl Pts',(87.5053328579372,55.6737742727883,13.2309896352733));
#70808=CARTESIAN_POINT('Ctrl Pts',(87.5056355276585,55.6738068047807,13.2311209632269));
#70809=CARTESIAN_POINT('Ctrl Pts',(87.506504456366,55.6739001959589,13.2314975878455));
#70810=CARTESIAN_POINT('Ctrl Pts',(87.5070708421007,55.673961065029,13.2317425893548));
#70811=CARTESIAN_POINT('Ctrl Pts',(87.5129785845904,55.6745959121788,13.2342929918363));
#70812=CARTESIAN_POINT('Ctrl Pts',(87.5183354310073,55.6751711027529,13.2365620293644));
#70813=CARTESIAN_POINT('Ctrl Pts',(87.5326730780846,55.6767095635314,13.2425192785805));
#70814=CARTESIAN_POINT('Ctrl Pts',(87.5416806848059,55.6776750176336,13.2461413576657));
#70815=CARTESIAN_POINT('Ctrl Pts',(87.5656139768747,55.6802380967766,13.255447925763));
#70816=CARTESIAN_POINT('Ctrl Pts',(87.5806062949899,55.6818415006664,13.2609545081679));
#70817=CARTESIAN_POINT('Ctrl Pts',(87.663818240602,55.6907340848988,13.289748704159));
#70818=CARTESIAN_POINT('Ctrl Pts',(87.7338059419043,55.6981998836504,13.3074729191307));
#70819=CARTESIAN_POINT('Ctrl Pts',(87.8708204367117,55.7127831599365,13.3300064403415));
#70820=CARTESIAN_POINT('Ctrl Pts',(87.9374904078203,55.7198626315721,13.3356295588604));
#70821=CARTESIAN_POINT('Ctrl Pts',(88.0196803995132,55.7284374411179,13.3360635381995));
#70822=CARTESIAN_POINT('Ctrl Pts',(88.0350676274304,55.7300358253202,13.3358651668414));
#70823=CARTESIAN_POINT('Ctrl Pts',(88.0685363960555,55.7334930915727,13.3348250704445));
#70824=CARTESIAN_POINT('Ctrl Pts',(88.0866121035431,55.7353479619491,13.3338763441794));
#70825=CARTESIAN_POINT('Ctrl Pts',(88.1117501175129,55.7379054957451,13.3320173445547));
#70826=CARTESIAN_POINT('Ctrl Pts',(88.118833086259,55.7386236675221,13.3314337347683));
#70827=CARTESIAN_POINT('Ctrl Pts',(88.1309343977645,55.7398461000161,13.3303342842001));
#70828=CARTESIAN_POINT('Ctrl Pts',(88.1359551297586,55.7403519211687,13.329847958544));
#70829=CARTESIAN_POINT('Ctrl Pts',(88.1465685640516,55.7414182033296,13.328756035346));
#70830=CARTESIAN_POINT('Ctrl Pts',(88.1521603195523,55.7419782607953,13.3281431808919));
#70831=CARTESIAN_POINT('Ctrl Pts',(88.1675980908674,55.7435202059159,13.3263473230968));
#70832=CARTESIAN_POINT('Ctrl Pts',(88.1774349668264,55.7444979234998,13.3250860817073));
#70833=CARTESIAN_POINT('Ctrl Pts',(88.2404439530875,55.7507359644723,13.316255943038));
#70834=CARTESIAN_POINT('Ctrl Pts',(88.2931151631623,55.7558386964992,13.3054344023733));
#70835=CARTESIAN_POINT('Ctrl Pts',(88.4171547747149,55.7679447184983,13.2716279923893));
#70836=CARTESIAN_POINT('Ctrl Pts',(88.4874753148645,55.7748883283417,13.2456065461113));
#70837=CARTESIAN_POINT('Ctrl Pts',(88.5935032145018,55.7860092315872,13.195334685387));
#70838=CARTESIAN_POINT('Ctrl Pts',(88.6309680579838,55.7900762844767,13.1752094502193));
#70839=CARTESIAN_POINT('Ctrl Pts',(88.679175435972,55.7955520454105,13.1461075863678));
#70840=CARTESIAN_POINT('Ctrl Pts',(88.6908832878241,55.7969017051802,13.1387765332332));
#70841=CARTESIAN_POINT('Ctrl Pts',(88.7102365276172,55.7991679157762,13.1262141487104));
#70842=CARTESIAN_POINT('Ctrl Pts',(88.7179487086796,55.800080561094,13.1210873303257));
#70843=CARTESIAN_POINT('Ctrl Pts',(88.7330497004182,55.8018871510145,13.1108087649444));
#70844=CARTESIAN_POINT('Ctrl Pts',(88.7404411439118,55.8027808713713,13.1056618354437));
#70845=CARTESIAN_POINT('Ctrl Pts',(88.7583433574245,55.8049692612826,13.0929109959384));
#70846=CARTESIAN_POINT('Ctrl Pts',(88.7687932849732,55.8062670525804,13.0852240149216));
#70847=CARTESIAN_POINT('Ctrl Pts',(88.8051932460129,55.8108621234631,13.0575789268829));
#70848=CARTESIAN_POINT('Ctrl Pts',(88.8304848261571,55.8141915632259,13.036781029078));
#70849=CARTESIAN_POINT('Ctrl Pts',(88.9201000927007,55.8265210474135,12.9570891838294));
#70850=CARTESIAN_POINT('Ctrl Pts',(88.9791079843614,55.835727146904,12.8925983979044));
#70851=CARTESIAN_POINT('Ctrl Pts',(89.0602621818186,55.8500705710538,12.7831858671924));
#70852=CARTESIAN_POINT('Ctrl Pts',(89.0871844537959,55.8552105447934,12.7421176125316));
#70853=CARTESIAN_POINT('Ctrl Pts',(89.1177991738759,55.8614998146564,12.6889339773645));
#70854=CARTESIAN_POINT('Ctrl Pts',(89.1237780700906,55.8627524967985,12.6781896427754));
#70855=CARTESIAN_POINT('Ctrl Pts',(89.1324950260401,55.8646146869766,12.6619750643581));
#70856=CARTESIAN_POINT('Ctrl Pts',(89.1353508749676,55.865230852365,12.6565696287676));
#70857=CARTESIAN_POINT('Ctrl Pts',(89.1404545385452,55.8663428950501,12.6467383926541));
#70858=CARTESIAN_POINT('Ctrl Pts',(89.1427155291385,55.8668395371269,12.6423198759139));
#70859=CARTESIAN_POINT('Ctrl Pts',(89.1478060136406,55.8679669742596,12.6322263622838));
#70860=CARTESIAN_POINT('Ctrl Pts',(89.1506189912415,55.8685967520716,12.6265432785495));
#70861=CARTESIAN_POINT('Ctrl Pts',(89.1592834587884,55.8705588432015,12.6087035208388));
#70862=CARTESIAN_POINT('Ctrl Pts',(89.1649842067851,55.8718825099257,12.5964738609668));
#70863=CARTESIAN_POINT('Ctrl Pts',(89.2045111413687,55.8813209205935,12.5080233388288));
#70864=CARTESIAN_POINT('Ctrl Pts',(89.2309587827467,55.8890796517984,12.4287111492942));
#70865=CARTESIAN_POINT('Ctrl Pts',(89.2609388073206,55.9017593893021,12.2967526302879));
#70866=CARTESIAN_POINT('Ctrl Pts',(89.2693231612351,55.9066306403825,12.2454876970344));
#70867=CARTESIAN_POINT('Ctrl Pts',(89.2767790551808,55.9136952953303,12.1718048464141));
#70868=CARTESIAN_POINT('Ctrl Pts',(89.2784326683684,55.9158223993223,12.1496994005669));
#70869=CARTESIAN_POINT('Ctrl Pts',(89.2803700289887,55.9196879732769,12.1097802745085));
#70870=CARTESIAN_POINT('Ctrl Pts',(89.2808589836994,55.9214201406924,12.091982102853));
#70871=CARTESIAN_POINT('Ctrl Pts',(89.2810386596975,55.9241522940594,12.0640886772878));
#70872=CARTESIAN_POINT('Ctrl Pts',(89.280983369067,55.9251443728037,12.0539967493361));
#70873=CARTESIAN_POINT('Ctrl Pts',(89.2806545115811,55.9270098537972,12.0350955565668));
#70874=CARTESIAN_POINT('Ctrl Pts',(89.2804094996243,55.9278823119618,12.0262863282272));
#70875=CARTESIAN_POINT('Ctrl Pts',(89.2796518115364,55.9298523695406,12.0064682308919));
#70876=CARTESIAN_POINT('Ctrl Pts',(89.279087478474,55.9309515145273,11.9954622249726));
#70877=CARTESIAN_POINT('Ctrl Pts',(89.2772581722589,55.9338052960521,11.9670273518823));
#70878=CARTESIAN_POINT('Ctrl Pts',(89.2757766239835,55.9355664915871,11.9496154756622));
#70879=CARTESIAN_POINT('Ctrl Pts',(89.2665586479876,55.9444439554479,11.8625805901143));
#70880=CARTESIAN_POINT('Ctrl Pts',(89.2534318267701,55.9517210931723,11.7936653095985));
#70881=CARTESIAN_POINT('Ctrl Pts',(89.2176838792596,55.9657682810975,11.6649301374377));
#70882=CARTESIAN_POINT('Ctrl Pts',(89.1960937041524,55.9725025550085,11.6050267144622));
#70883=CARTESIAN_POINT('Ctrl Pts',(89.1639874814961,55.9806948586644,11.5333236331117));
#70884=CARTESIAN_POINT('Ctrl Pts',(89.1576261640088,55.9822497517298,11.5197649468844));
#70885=CARTESIAN_POINT('Ctrl Pts',(89.1432001287251,55.9856283311879,11.4903801303504));
#70886=CARTESIAN_POINT('Ctrl Pts',(89.1350398737897,55.9874479744314,11.4746034831961));
#70887=CARTESIAN_POINT('Ctrl Pts',(89.1231783327473,55.9899656742618,11.4528041584942));
#70888=CARTESIAN_POINT('Ctrl Pts',(89.1197542832255,55.9906786321525,11.4466344118229));
#70889=CARTESIAN_POINT('Ctrl Pts',(89.1137983987996,55.9918950603745,11.4361102836849));
#70890=CARTESIAN_POINT('Ctrl Pts',(89.1112918188034,55.9924000511409,11.4317419441958));
#70891=CARTESIAN_POINT('Ctrl Pts',(89.1059187905168,55.9934678258761,11.4225058281628));
#70892=CARTESIAN_POINT('Ctrl Pts',(89.1030457675802,55.9940301837883,11.4176421103241));
#70893=CARTESIAN_POINT('Ctrl Pts',(89.0949829953296,55.9955852846546,11.4041983608931));
#70894=CARTESIAN_POINT('Ctrl Pts',(89.0897237492058,55.9965737403957,11.395660056588));
#70895=CARTESIAN_POINT('Ctrl Pts',(89.0508493751088,56.0037029489873,11.3341907235481));
#70896=CARTESIAN_POINT('Ctrl Pts',(89.0134495705617,56.0096269624183,11.283740743919));
#70897=CARTESIAN_POINT('Ctrl Pts',(88.940356290514,56.0201315394287,11.1990441419156));
#70898=CARTESIAN_POINT('Ctrl Pts',(88.9061129501435,56.0247159314429,11.1637315713122));
#70899=CARTESIAN_POINT('Ctrl Pts',(88.8421375310175,56.03289278576,11.1049943529791));
#70900=CARTESIAN_POINT('Ctrl Pts',(88.8132461906574,56.0364629514657,11.0807477235114));
#70901=CARTESIAN_POINT('Ctrl Pts',(88.7624019205083,56.0426038469785,11.0417980652809));
#70902=CARTESIAN_POINT('Ctrl Pts',(88.7409904372697,56.0451502740243,11.0264288462198));
#70903=CARTESIAN_POINT('Ctrl Pts',(88.7094126116907,56.0488627692712,11.005218911422));
#70904=CARTESIAN_POINT('Ctrl Pts',(88.6996179207254,56.0500085255986,10.9988345812159));
#70905=CARTESIAN_POINT('Ctrl Pts',(88.6822262708745,56.0520339942342,10.9878375557018));
#70906=CARTESIAN_POINT('Ctrl Pts',(88.6746662714523,56.0529115307871,10.9831675877452));
#70907=CARTESIAN_POINT('Ctrl Pts',(88.6587437661365,56.0547541911329,10.9735613041863));
#70908=CARTESIAN_POINT('Ctrl Pts',(88.6503724491952,56.0557198219884,10.9686408297783));
#70909=CARTESIAN_POINT('Ctrl Pts',(88.6280779651335,56.0582839079776,10.9558783286952));
#70910=CARTESIAN_POINT('Ctrl Pts',(88.6140623527833,56.0598881502024,10.9482025769741));
#70911=CARTESIAN_POINT('Ctrl Pts',(88.5359858059523,56.0687879623391,10.9073391511682));
#70912=CARTESIAN_POINT('Ctrl Pts',(88.4693458572225,56.0762604648247,10.8793999772346));
#70913=CARTESIAN_POINT('Ctrl Pts',(88.3371893591119,56.090844114938,10.8367909711677));
#70914=CARTESIAN_POINT('Ctrl Pts',(88.2721526629635,56.0979169553746,10.8213498843952));
#70915=CARTESIAN_POINT('Ctrl Pts',(88.1910068747653,56.1064844368024,10.8087275440985));
#70916=CARTESIAN_POINT('Ctrl Pts',(88.1757684170574,56.1080820065607,10.806639875073));
#70917=CARTESIAN_POINT('Ctrl Pts',(88.1425301929175,56.1115378034208,10.8026999260661));
#70918=CARTESIAN_POINT('Ctrl Pts',(88.1245203002804,56.1133920181771,10.8009543376484));
#70919=CARTESIAN_POINT('Ctrl Pts',(88.0993921900853,56.1159488114788,10.7990598631737));
#70920=CARTESIAN_POINT('Ctrl Pts',(88.0923020320993,56.1166668869841,10.7985851200841));
#70921=CARTESIAN_POINT('Ctrl Pts',(88.0801727221825,56.1178892083945,10.7978751737321));
#70922=CARTESIAN_POINT('Ctrl Pts',(88.0751355902273,56.1183950139965,10.7976104417985));
#70923=CARTESIAN_POINT('Ctrl Pts',(88.064477410663,56.1194613226922,10.7971139484841));
#70924=CARTESIAN_POINT('Ctrl Pts',(88.0588562212764,56.120021421833,10.7968895115888));
#70925=CARTESIAN_POINT('Ctrl Pts',(88.0433205130568,56.1215636050123,10.7963725896781));
#70926=CARTESIAN_POINT('Ctrl Pts',(88.03340341165,56.1225415168726,10.79615887364));
#70927=CARTESIAN_POINT('Ctrl Pts',(87.9696194821342,56.1287954453636,10.7955318392073));
#70928=CARTESIAN_POINT('Ctrl Pts',(87.9157651788213,56.1339128960047,10.7984298078159));
#70929=CARTESIAN_POINT('Ctrl Pts',(87.7880484743806,56.1460217478487,10.8134925729129));
#70930=CARTESIAN_POINT('Ctrl Pts',(87.7147674563245,56.1529543306058,10.8287739572073));
#70931=CARTESIAN_POINT('Ctrl Pts',(87.6026022001417,56.164060615678,10.8627065293705));
#70932=CARTESIAN_POINT('Ctrl Pts',(87.5625967117778,56.1681244943999,10.8770350707131));
#70933=CARTESIAN_POINT('Ctrl Pts',(87.5106366817107,56.1735966453727,10.8986409012261));
#70934=CARTESIAN_POINT('Ctrl Pts',(87.4979731099872,56.1749459728426,10.9041505734897));
#70935=CARTESIAN_POINT('Ctrl Pts',(87.4769726029787,56.1772117823192,10.9136977440502));
#70936=CARTESIAN_POINT('Ctrl Pts',(87.4685851766618,56.1781243618353,10.9176220579012));
#70937=CARTESIAN_POINT('Ctrl Pts',(87.452125281242,56.1799309411882,10.9255438703538));
#70938=CARTESIAN_POINT('Ctrl Pts',(87.4440509356029,56.1808247176085,10.9295362378753));
#70939=CARTESIAN_POINT('Ctrl Pts',(87.4244504827272,56.1830134611015,10.9394885585551));
#70940=CARTESIAN_POINT('Ctrl Pts',(87.4129722426007,56.1843115523338,10.9455397672585));
#70941=CARTESIAN_POINT('Ctrl Pts',(87.372845889215,56.188909461235,10.9674861620631));
#70942=CARTESIAN_POINT('Ctrl Pts',(87.3447251315953,56.192241494459,10.9843112155731));
#70943=CARTESIAN_POINT('Ctrl Pts',(87.2442707878701,56.2045714642783,11.0498182880128));
#70944=CARTESIAN_POINT('Ctrl Pts',(87.1763595116153,56.2137752159159,11.1048188063935));
#70945=CARTESIAN_POINT('Ctrl Pts',(87.0889306919784,56.2267700228069,11.1919268355821));
#70946=CARTESIAN_POINT('Ctrl Pts',(87.0643413274314,56.2305754225416,11.2186196204076));
#70947=CARTESIAN_POINT('Ctrl Pts',(87.0271184295518,56.2365499754805,11.262672679929));
#70948=CARTESIAN_POINT('Ctrl Pts',(87.0137238993618,56.2387489214221,11.2793626675136));
#70949=CARTESIAN_POINT('Ctrl Pts',(86.9961736224313,56.2416908311097,11.3024002298551));
#70950=CARTESIAN_POINT('Ctrl Pts',(86.9916446196991,56.2424557987304,11.3084567308875));
#70951=CARTESIAN_POINT('Ctrl Pts',(86.9841382472343,56.2437330227021,11.3186840084514));
#70952=CARTESIAN_POINT('Ctrl Pts',(86.9811316030901,56.244247199545,11.3228328987715));
#70953=CARTESIAN_POINT('Ctrl Pts',(86.9749800803662,56.2453044264436,11.3314304642347));
#70954=CARTESIAN_POINT('Ctrl Pts',(86.971838584719,56.2458472518691,11.3358813562947));
#70955=CARTESIAN_POINT('Ctrl Pts',(86.9635287614173,56.2472914053428,11.3478170618374));
#70956=CARTESIAN_POINT('Ctrl Pts',(86.9584118687584,56.2481893905372,11.355337652707));
#70957=CARTESIAN_POINT('Ctrl Pts',(86.9344966965585,56.2524320379852,11.3913122335962));
#70958=CARTESIAN_POINT('Ctrl Pts',(86.9167662021825,56.2557149288231,11.4204645551366));
#70959=CARTESIAN_POINT('Ctrl Pts',(86.8547707484135,56.2678895556538,11.5323091523519));
#70960=CARTESIAN_POINT('Ctrl Pts',(86.8185328665949,56.2765287208852,11.6191038169872));
#70961=CARTESIAN_POINT('Ctrl Pts',(86.7797200802849,56.2896047084489,11.7516507588071));
#70962=CARTESIAN_POINT('Ctrl Pts',(86.7694989147304,56.2938425203501,11.7948177423543));
#70963=CARTESIAN_POINT('Ctrl Pts',(86.75904840319,56.2995121402973,11.8521939074152));
#70964=CARTESIAN_POINT('Ctrl Pts',(86.7567685632377,56.3008791851863,11.8660017210296));
#70965=CARTESIAN_POINT('Ctrl Pts',(86.7533546557878,56.3031664025184,11.8890406043635));
#70966=CARTESIAN_POINT('Ctrl Pts',(86.7520929406033,56.3040825105391,11.8982518440248));
#70967=CARTESIAN_POINT('Ctrl Pts',(86.7498116281836,56.3058897896291,11.9163854014396));
#70968=CARTESIAN_POINT('Ctrl Pts',(86.7487853113059,56.3067806936629,11.9253063385142));
#70969=CARTESIAN_POINT('Ctrl Pts',(86.7465233004314,56.3089511861853,11.9469911304842));
#70970=CARTESIAN_POINT('Ctrl Pts',(86.7453861951153,56.3102337745337,11.9597639391091));
#70971=CARTESIAN_POINT('Ctrl Pts',(86.7421265891875,56.314686078039,12.003942964004));
#70972=CARTESIAN_POINT('Ctrl Pts',(86.7409785861381,56.3178852264891,12.0354062694396));
#70973=CARTESIAN_POINT('Ctrl Pts',(86.7410352212291,56.3263148445825,12.1174797443888));
#70974=CARTESIAN_POINT('Ctrl Pts',(86.7440945202449,56.331592165542,12.1680288336347));
#70975=CARTESIAN_POINT('Ctrl Pts',(86.7596908493171,56.3452677324998,12.2971843871384));
#70976=CARTESIAN_POINT('Ctrl Pts',(86.7766131019831,56.3537058707465,12.3750492538448));
#70977=CARTESIAN_POINT('Ctrl Pts',(86.8059324309397,56.36369054287,12.467259981848));
#70978=CARTESIAN_POINT('Ctrl Pts',(86.8114928091901,56.3654576267333,12.4835883390532));
#70979=CARTESIAN_POINT('Ctrl Pts',(86.8195930577662,56.3678641805881,12.5058764624462));
#70980=CARTESIAN_POINT('Ctrl Pts',(86.8218480081806,56.3685179406992,12.5119364877091));
#70981=CARTESIAN_POINT('Ctrl Pts',(86.8258027220988,56.3696369763389,12.5223211572607));
#70982=CARTESIAN_POINT('Ctrl Pts',(86.8274800772679,56.3701035024166,12.5266540797633));
#70983=CARTESIAN_POINT('Ctrl Pts',(86.8311038950971,56.3710942489164,12.5358646177411));
#70984=CARTESIAN_POINT('Ctrl Pts',(86.833056920098,56.3716180587509,12.5407395933306));
#70985=CARTESIAN_POINT('Ctrl Pts',(86.8381333998695,56.3729543940538,12.5531868522906));
#70986=CARTESIAN_POINT('Ctrl Pts',(86.8413000584495,56.3737644051926,12.5607414987031));
#70987=CARTESIAN_POINT('Ctrl Pts',(86.8551894874383,56.3772207984287,12.5929982870824));
#70988=CARTESIAN_POINT('Ctrl Pts',(86.8666245069872,56.3798288481463,12.6173893602901));
#70989=CARTESIAN_POINT('Ctrl Pts',(86.9028290931551,56.3874868679531,12.6886262917061));
#70990=CARTESIAN_POINT('Ctrl Pts',(86.9297640290972,56.3924532625638,12.7343084705616));
#70991=CARTESIAN_POINT('Ctrl Pts',(87.0067403310917,56.4053142286159,12.8479630621663));
#70992=CARTESIAN_POINT('Ctrl Pts',(87.0608259367857,56.413184283837,12.9128588107876));
#70993=CARTESIAN_POINT('Ctrl Pts',(87.1332758337077,56.4229920160226,12.9840412066627));
#70994=CARTESIAN_POINT('Ctrl Pts',(87.1458636762144,56.4246722122169,12.9959131372973));
#70995=CARTESIAN_POINT('Ctrl Pts',(87.1659325664215,56.4273180656943,13.0140804229115));
#70996=CARTESIAN_POINT('Ctrl Pts',(87.1732508658231,56.4282763111732,13.0205532091559));
#70997=CARTESIAN_POINT('Ctrl Pts',(87.1806428354357,56.4292380444866,13.0269406741609));
#70998=CARTESIAN_POINT('',(86.7390851620259,56.4915176496327,12.0663168694075));
#70999=CARTESIAN_POINT('Ctrl Pts',(87.1801902653375,56.5998778161658,13.027459163232));
#71000=CARTESIAN_POINT('Ctrl Pts',(86.9210985275164,56.5654670839852,12.7990647662412));
#71001=CARTESIAN_POINT('Ctrl Pts',(86.7455185357409,56.5293656784333,12.4445437149527));
#71002=CARTESIAN_POINT('Ctrl Pts',(86.7389313495616,56.4932642728814,12.0832340865421));
#71003=CARTESIAN_POINT('Ctrl Pts',(86.7389871696286,56.49157359951,12.0663114291823));
#71004=CARTESIAN_POINT('Ctrl Pts',(86.7410000705041,56.490424310788,12.0664231790162));
#71005=CARTESIAN_POINT('Ctrl Pts',(86.7409944767077,56.4887786996571,12.0496356712115));
#71006=CARTESIAN_POINT('Ctrl Pts',(86.7413217419207,56.4871486528724,12.0328482222298));
#71007=CARTESIAN_POINT('Ctrl Pts',(86.7440792033363,56.4803888779874,11.9627636847443));
#71008=CARTESIAN_POINT('Ctrl Pts',(86.749533632266,56.4753729203867,11.9096347422265));
#71009=CARTESIAN_POINT('Ctrl Pts',(86.768349665406,56.4646530658008,11.7968567378609));
#71010=CARTESIAN_POINT('Ctrl Pts',(86.7827018223532,56.4589658482191,11.7375172852167));
#71011=CARTESIAN_POINT('Ctrl Pts',(86.8094982888892,56.4506112304282,11.6536575793795));
#71012=CARTESIAN_POINT('Ctrl Pts',(86.8185584631519,56.4480261107585,11.6281465907376));
#71013=CARTESIAN_POINT('Ctrl Pts',(86.8359784216655,56.4434202088412,11.5836584749831));
#71014=CARTESIAN_POINT('Ctrl Pts',(86.8440010284607,56.4414101030804,11.5645597327873));
#71015=CARTESIAN_POINT('Ctrl Pts',(86.8568603942884,56.438340381375,11.5359285543681));
#71016=CARTESIAN_POINT('Ctrl Pts',(86.861356725083,56.4372922935868,11.526246083597));
#71017=CARTESIAN_POINT('Ctrl Pts',(86.8694073110944,56.4354577264873,11.5094668830204));
#71018=CARTESIAN_POINT('Ctrl Pts',(86.8729070970506,56.4346731649628,11.5023445070938));
#71019=CARTESIAN_POINT('Ctrl Pts',(86.8809816175717,56.4328914891435,11.4862939613533));
#71020=CARTESIAN_POINT('Ctrl Pts',(86.8855957873334,56.4318930404775,11.4773863923023));
#71021=CARTESIAN_POINT('Ctrl Pts',(86.8983429609311,56.4291858788526,11.4534761008689));
#71022=CARTESIAN_POINT('Ctrl Pts',(86.9066732734729,56.427470320509,11.4385817807309));
#71023=CARTESIAN_POINT('Ctrl Pts',(86.9275529782467,56.4232926603611,11.4029541836966));
#71024=CARTESIAN_POINT('Ctrl Pts',(86.940400105792,56.4208205437462,11.3824044521476));
#71025=CARTESIAN_POINT('Ctrl Pts',(87.0020707037576,56.4093774007473,11.2897646095174));
#71026=CARTESIAN_POINT('Ctrl Pts',(87.0576328732422,56.4001850851353,11.2224563229708));
#71027=CARTESIAN_POINT('Ctrl Pts',(87.1545397847391,56.3858605373558,11.1269695469317));
#71028=CARTESIAN_POINT('Ctrl Pts',(87.1914193126317,56.3807253865876,11.0946138270385));
#71029=CARTESIAN_POINT('Ctrl Pts',(87.2369743565261,56.3748050675469,11.0590935056295));
#71030=CARTESIAN_POINT('Ctrl Pts',(87.2439222965438,56.3739130486739,11.0537904385945));
#71031=CARTESIAN_POINT('Ctrl Pts',(87.2566354155185,56.3723012853771,11.0442931510139));
#71032=CARTESIAN_POINT('Ctrl Pts',(87.2623821426932,56.3715801421382,11.0400749910614));
#71033=CARTESIAN_POINT('Ctrl Pts',(87.2682565773948,56.3708506988579,11.0358387402388));
#71034=CARTESIAN_POINT('Ctrl Pts',(87.2683488382733,56.3708392445173,11.0357722266789));
#71035=CARTESIAN_POINT('Ctrl Pts',(87.2685328322327,56.3708164052009,11.0356396176234));
#71036=CARTESIAN_POINT('Ctrl Pts',(87.2686245651208,56.3708050202265,11.0355735220446));
#71037=CARTESIAN_POINT('Ctrl Pts',(87.2688076081209,56.3707823065441,11.0354416726367));
#71038=CARTESIAN_POINT('Ctrl Pts',(87.2688989181502,56.3707709778283,11.0353759186889));
#71039=CARTESIAN_POINT('Ctrl Pts',(87.2690812213319,56.3707483634739,11.0352446757701));
#71040=CARTESIAN_POINT('Ctrl Pts',(87.269172214486,56.3707370778214,11.0351791866634));
#71041=CARTESIAN_POINT('Ctrl Pts',(87.2693539913903,56.3707145362265,11.0350483956949));
#71042=CARTESIAN_POINT('Ctrl Pts',(87.2694447749949,56.370703280293,11.0349830938468));
#71043=CARTESIAN_POINT('Ctrl Pts',(87.26962624206,56.3706807845657,11.0348525985527));
#71044=CARTESIAN_POINT('Ctrl Pts',(87.2697169255604,56.370669544762,11.0347874050308));
#71045=CARTESIAN_POINT('Ctrl Pts',(87.2698983041798,56.3706470674316,11.0346570459229));
#71046=CARTESIAN_POINT('Ctrl Pts',(87.2699889993472,56.3706358298986,11.0345918802997));
#71047=CARTESIAN_POINT('Ctrl Pts',(87.2701705163076,56.3706133428628,11.0344614943715));
#71048=CARTESIAN_POINT('Ctrl Pts',(87.2702613380428,56.3706020933718,11.0343962741517));
#71049=CARTESIAN_POINT('Ctrl Pts',(87.270443226833,56.3705795677358,11.0342656939495));
#71050=CARTESIAN_POINT('Ctrl Pts',(87.2705342939309,56.370568291595,11.0342003340276));
#71051=CARTESIAN_POINT('Ctrl Pts',(87.2707167966334,56.3705456974386,11.0340693863076));
#71052=CARTESIAN_POINT('Ctrl Pts',(87.2708082323319,56.3705343794258,11.0340037985833));
#71053=CARTESIAN_POINT('Ctrl Pts',(87.2709916007978,56.37051168566,11.0338723034888));
#71054=CARTESIAN_POINT('Ctrl Pts',(87.2710835337144,56.3705003099083,11.0338063962052));
#71055=CARTESIAN_POINT('Ctrl Pts',(87.2712680314927,56.3704774840393,11.0336741659072));
#71056=CARTESIAN_POINT('Ctrl Pts',(87.2713605965202,56.370466033927,11.0336078430233));
#71057=CARTESIAN_POINT('Ctrl Pts',(87.2715465008455,56.3704430418132,11.033474680326));
#71058=CARTESIAN_POINT('Ctrl Pts',(87.2716398401792,56.370431499839,11.033407840796));
#71059=CARTESIAN_POINT('Ctrl Pts',(87.2718274438669,56.3704083054605,11.0332735378152));
#71060=CARTESIAN_POINT('Ctrl Pts',(87.2719217083586,56.3703966530776,11.0332060746395));
#71061=CARTESIAN_POINT('Ctrl Pts',(87.2721113228761,56.3703732181611,11.0330704106469));
#71062=CARTESIAN_POINT('Ctrl Pts',(87.2722066732121,56.3703614356347,11.0330022100524));
#71063=CARTESIAN_POINT('Ctrl Pts',(87.2723461567687,56.3703442025296,11.0329024717763));
#71064=CARTESIAN_POINT('Ctrl Pts',(87.2723902822376,56.3703387512953,11.0328709239552));
#71065=CARTESIAN_POINT('Ctrl Pts',(87.2724821732136,56.370327400054,11.0328052347375));
#71066=CARTESIAN_POINT('Ctrl Pts',(87.272529939278,56.3703215000534,11.0327710936755));
#71067=CARTESIAN_POINT('Ctrl Pts',(87.2726295855147,56.3703091929578,11.0326998814097));
#71068=CARTESIAN_POINT('Ctrl Pts',(87.2726814659998,56.3703027859164,11.0326628108804));
#71069=CARTESIAN_POINT('Ctrl Pts',(87.2727899052278,56.3702893953567,11.0325853393688));
#71070=CARTESIAN_POINT('Ctrl Pts',(87.272846464472,56.3702824118908,11.0325449391393));
#71071=CARTESIAN_POINT('Ctrl Pts',(87.2729649386706,56.3702677851928,11.0324603277878));
#71072=CARTESIAN_POINT('Ctrl Pts',(87.2730268543755,56.3702601420111,11.0324161175187));
#71073=CARTESIAN_POINT('Ctrl Pts',(87.2731568638035,56.3702440948194,11.032323303268));
#71074=CARTESIAN_POINT('Ctrl Pts',(87.2732249584165,56.3702356908805,11.0322747004085));
#71075=CARTESIAN_POINT('Ctrl Pts',(87.273368335546,56.3702179981067,11.032172385672));
#71076=CARTESIAN_POINT('Ctrl Pts',(87.2734436190188,56.370208709386,11.0321186753664));
#71077=CARTESIAN_POINT('Ctrl Pts',(87.2736026302837,56.3701890927586,11.0320052564394));
#71078=CARTESIAN_POINT('Ctrl Pts',(87.2736863595989,56.3701787649665,11.0319455496668));
#71079=CARTESIAN_POINT('Ctrl Pts',(87.2738638502754,56.3701568753092,11.0318190148594));
#71080=CARTESIAN_POINT('Ctrl Pts',(87.2739576133625,56.3701453136324,11.0317521894842));
#71081=CARTESIAN_POINT('Ctrl Pts',(87.2741572134408,56.3701207057009,11.0316099745354));
#71082=CARTESIAN_POINT('Ctrl Pts',(87.2742630530015,56.3701076596722,11.0315345883924));
#71083=CARTESIAN_POINT('Ctrl Pts',(87.2744894875351,56.370079754236,11.0313733586743));
#71084=CARTESIAN_POINT('Ctrl Pts',(87.2746100859724,56.3700648951541,11.0312875199213));
#71085=CARTESIAN_POINT('Ctrl Pts',(87.2786299330166,56.3695697142246,11.0284273586923));
#71086=CARTESIAN_POINT('Ctrl Pts',(87.2825447771138,56.3690909217771,11.0256751027829));
#71087=CARTESIAN_POINT('Ctrl Pts',(87.2916750575344,56.3679821814479,11.019333047508));
#71088=CARTESIAN_POINT('Ctrl Pts',(87.2969019151688,56.3673533567395,11.0157600208355));
#71089=CARTESIAN_POINT('Ctrl Pts',(87.3126171974897,56.3654795160996,11.0051887857053));
#71090=CARTESIAN_POINT('Ctrl Pts',(87.3231838553466,56.3642417509356,10.9983071760737));
#71091=CARTESIAN_POINT('Ctrl Pts',(87.382871782273,56.3573616452187,10.9606890214764));
#71092=CARTESIAN_POINT('Ctrl Pts',(87.4339573578284,56.3518890492376,10.9331798210705));
#71093=CARTESIAN_POINT('Ctrl Pts',(87.5324397445668,56.3417366362891,10.8885467312684));
#71094=CARTESIAN_POINT('Ctrl Pts',(87.5793135195015,56.3370584669608,10.8705658431235));
#71095=CARTESIAN_POINT('Ctrl Pts',(87.6625147283791,56.3288380521041,10.844183242201));
#71096=CARTESIAN_POINT('Ctrl Pts',(87.6983739262747,56.3253211888709,10.834520127424));
#71097=CARTESIAN_POINT('Ctrl Pts',(87.7467028267305,56.3205724667023,10.8237437011638));
#71098=CARTESIAN_POINT('Ctrl Pts',(87.7588419473514,56.3193790292513,10.8212229108515));
#71099=CARTESIAN_POINT('Ctrl Pts',(87.7888890615619,56.3164209155193,10.815440916354));
#71100=CARTESIAN_POINT('Ctrl Pts',(87.8068332884153,56.314650741386,10.8123863574094));
#71101=CARTESIAN_POINT('Ctrl Pts',(87.8348987398724,56.3118723908203,10.8082274329291));
#71102=CARTESIAN_POINT('Ctrl Pts',(87.8449787592737,56.3108725810802,10.8068572689973));
#71103=CARTESIAN_POINT('Ctrl Pts',(87.8638099351451,56.3090004349457,10.8045276170071));
#71104=CARTESIAN_POINT('Ctrl Pts',(87.8725567930655,56.3081291091245,10.8035377404462));
#71105=CARTESIAN_POINT('Ctrl Pts',(87.8921596036967,56.3061719822419,10.8015254650013));
#71106=CARTESIAN_POINT('Ctrl Pts',(87.9030196925874,56.3050847224233,10.8005518091968));
#71107=CARTESIAN_POINT('Ctrl Pts',(87.9309162330448,56.3022832651873,10.7984124609382));
#71108=CARTESIAN_POINT('Ctrl Pts',(87.947965421085,56.3005629077477,10.797450376176));
#71109=CARTESIAN_POINT('Ctrl Pts',(88.0549190890686,56.28971301617,10.7935762647113));
#71110=CARTESIAN_POINT('Ctrl Pts',(88.1448803227444,56.2803039770397,10.7998801562732));
#71111=CARTESIAN_POINT('Ctrl Pts',(88.2817750535413,56.2656445958738,10.8242290174473));
#71112=CARTESIAN_POINT('Ctrl Pts',(88.3296144268799,56.2604609850945,10.8356342849448));
#71113=CARTESIAN_POINT('Ctrl Pts',(88.3934232055733,56.2535324835066,10.8548194445523));
#71114=CARTESIAN_POINT('Ctrl Pts',(88.410066468963,56.2517241749087,10.86020072659));
#71115=CARTESIAN_POINT('Ctrl Pts',(88.4386829933462,56.2486181356404,10.870110826045));
#71116=CARTESIAN_POINT('Ctrl Pts',(88.4507084698018,56.2473138857012,10.8744798927133));
#71117=CARTESIAN_POINT('Ctrl Pts',(88.4684695107905,56.2453909386045,10.8812383382198));
#71118=CARTESIAN_POINT('Ctrl Pts',(88.4742562952742,56.2447649545584,10.883489044718));
#71119=CARTESIAN_POINT('Ctrl Pts',(88.484636201945,56.2436433510208,10.8876140900108));
#71120=CARTESIAN_POINT('Ctrl Pts',(88.489235058203,56.2431468869627,10.8894729765329));
#71121=CARTESIAN_POINT('Ctrl Pts',(88.4995905784515,56.2420299721852,10.8937294983982));
#71122=CARTESIAN_POINT('Ctrl Pts',(88.5053406282151,56.2414104544468,10.8961426447587));
#71123=CARTESIAN_POINT('Ctrl Pts',(88.5229617803364,56.2395132372071,10.903690911402));
#71124=CARTESIAN_POINT('Ctrl Pts',(88.5347730205113,56.2382433922188,10.9089653624906));
#71125=CARTESIAN_POINT('Ctrl Pts',(88.6068219341588,56.2304953922296,10.9424692094042));
#71126=CARTESIAN_POINT('Ctrl Pts',(88.6648559092674,56.2242434915549,10.9752200339329));
#71127=CARTESIAN_POINT('Ctrl Pts',(88.7504030762085,56.2145773851178,11.0327912405865));
#71128=CARTESIAN_POINT('Ctrl Pts',(88.7798447966393,56.2111590048738,11.0545085927455));
#71129=CARTESIAN_POINT('Ctrl Pts',(88.8394849889903,56.2039539411864,11.1026117372673));
#71130=CARTESIAN_POINT('Ctrl Pts',(88.869452131769,56.2001672709245,11.1292162744369));
#71131=CARTESIAN_POINT('Ctrl Pts',(88.9177769762932,56.193698887784,11.1763872560628));
#71132=CARTESIAN_POINT('Ctrl Pts',(88.936813711628,56.1910452735105,11.1962160985985));
#71133=CARTESIAN_POINT('Ctrl Pts',(88.9631322565225,56.1872059674732,11.2254732790846));
#71134=CARTESIAN_POINT('Ctrl Pts',(88.9709491471386,56.1860426371561,11.2344119925652));
#71135=CARTESIAN_POINT('Ctrl Pts',(88.9844102301413,56.1839972484038,11.2502476363671));
#71136=CARTESIAN_POINT('Ctrl Pts',(88.9901094240346,56.1831175077262,11.2570969647151));
#71137=CARTESIAN_POINT('Ctrl Pts',(89.0018150857961,56.1812811146627,11.2714698625218));
#71138=CARTESIAN_POINT('Ctrl Pts',(89.0078089888584,56.1803240301923,11.2790028587972));
#71139=CARTESIAN_POINT('Ctrl Pts',(89.0232829717716,56.1778080089371,11.2989105792398));
#71140=CARTESIAN_POINT('Ctrl Pts',(89.0326214958691,56.1762436714983,11.3113925139936));
#71141=CARTESIAN_POINT('Ctrl Pts',(89.0580231221436,56.1718549449632,11.3466804529686));
#71142=CARTESIAN_POINT('Ctrl Pts',(89.0735669327325,56.169011918626,11.3698468267732));
#71143=CARTESIAN_POINT('Ctrl Pts',(89.1342434680561,56.157226054938,11.4670502190186));
#71144=CARTESIAN_POINT('Ctrl Pts',(89.1724942837361,56.1480712647127,11.5450940886237));
#71145=CARTESIAN_POINT('Ctrl Pts',(89.2194158480375,56.1337985244895,11.6722728495075));
#71146=CARTESIAN_POINT('Ctrl Pts',(89.2336773376462,56.1286769272316,11.719083064245));
#71147=CARTESIAN_POINT('Ctrl Pts',(89.2480988191803,56.1224074729185,11.7785331935176));
#71148=CARTESIAN_POINT('Ctrl Pts',(89.250819484923,56.1211568874318,11.7905034693249));
#71149=CARTESIAN_POINT('Ctrl Pts',(89.2546336632738,56.1192972530635,11.8084876224617));
#71150=CARTESIAN_POINT('Ctrl Pts',(89.2558579061516,56.1186815713323,11.8144724424914));
#71151=CARTESIAN_POINT('Ctrl Pts',(89.257902487706,56.117619898294,11.824848313873));
#71152=CARTESIAN_POINT('Ctrl Pts',(89.2587428879161,56.1171728265193,11.8292350583147));
#71153=CARTESIAN_POINT('Ctrl Pts',(89.2606731197801,56.116120025118,11.8396063344473));
#71154=CARTESIAN_POINT('Ctrl Pts',(89.2617431294994,56.1155154130288,11.8455944017373));
#71155=CARTESIAN_POINT('Ctrl Pts',(89.2648200753046,56.1137106482858,11.8635582632988));
#71156=CARTESIAN_POINT('Ctrl Pts',(89.2666984298799,56.1125172850707,11.8755559638125));
#71157=CARTESIAN_POINT('Ctrl Pts',(89.2795355998673,56.1035953756986,11.9660249481598));
#71158=CARTESIAN_POINT('Ctrl Pts',(89.2833035921784,56.0961986007558,12.0453561360594));
#71159=CARTESIAN_POINT('Ctrl Pts',(89.2770664711368,56.0835222915077,12.1805360965278));
#71160=CARTESIAN_POINT('Ctrl Pts',(89.2707776747942,56.0782724249396,12.236300292316));
#71161=CARTESIAN_POINT('Ctrl Pts',(89.2547558179906,56.06967338265,12.3251153867929));
#71162=CARTESIAN_POINT('Ctrl Pts',(89.2473291266059,56.0663858273598,12.3585049471522));
#71163=CARTESIAN_POINT('Ctrl Pts',(89.2352715835483,56.061804731329,12.4039706853961));
#71164=CARTESIAN_POINT('Ctrl Pts',(89.2317897634942,56.0605477335515,12.4163390052111));
#71165=CARTESIAN_POINT('Ctrl Pts',(89.2255301371041,56.0583927257917,12.4373473727942));
#71166=CARTESIAN_POINT('Ctrl Pts',(89.2228462002056,56.0574978078645,12.4460146070116));
#71167=CARTESIAN_POINT('Ctrl Pts',(89.217554885032,56.0557864982736,12.4624755229777));
#71168=CARTESIAN_POINT('Ctrl Pts',(89.2149642574069,56.0549706963618,12.4702741516469));
#71169=CARTESIAN_POINT('Ctrl Pts',(89.2080310740555,56.0528426303544,12.4904874369771));
#71170=CARTESIAN_POINT('Ctrl Pts',(89.2035711594733,56.0515265653442,12.5028603581536));
#71171=CARTESIAN_POINT('Ctrl Pts',(89.1868779270127,56.0467800386114,12.5470098229965));
#71172=CARTESIAN_POINT('Ctrl Pts',(89.1735613511291,56.0433144859927,12.5783572005425));
#71173=CARTESIAN_POINT('Ctrl Pts',(89.1160653065638,56.0294775439033,12.6998858550423));
#71174=CARTESIAN_POINT('Ctrl Pts',(89.0625202196234,56.0188223565737,12.7852215082493));
#71175=CARTESIAN_POINT('Ctrl Pts',(88.9827458789932,56.0055011559645,12.8841212795644));
#71176=CARTESIAN_POINT('Ctrl Pts',(88.9653353061466,56.0027178139118,12.9043655803217));
#71177=CARTESIAN_POINT('Ctrl Pts',(88.9355485917708,55.9981694145393,12.9368687234744));
#71178=CARTESIAN_POINT('Ctrl Pts',(88.923535876726,55.9963880713386,12.9494482506916));
#71179=CARTESIAN_POINT('Ctrl Pts',(88.9063310241698,55.9939138773543,12.9667393295888));
#71180=CARTESIAN_POINT('Ctrl Pts',(88.901353398134,55.993206772056,12.9716598795706));
#71181=CARTESIAN_POINT('Ctrl Pts',(88.8927310836307,55.9919971384544,12.9800435249064));
#71182=CARTESIAN_POINT('Ctrl Pts',(88.8891061361935,55.9914931340657,12.9835265050985));
#71183=CARTESIAN_POINT('Ctrl Pts',(88.8813455108868,55.9904238334908,12.99089506889));
#71184=CARTESIAN_POINT('Ctrl Pts',(88.8772043515741,55.989858988403,12.9947745812247));
#71185=CARTESIAN_POINT('Ctrl Pts',(88.8657776399523,55.9883155705176,13.0053364212366));
#71186=CARTESIAN_POINT('Ctrl Pts',(88.858439589581,55.9873410869101,13.0119618862341));
#71187=CARTESIAN_POINT('Ctrl Pts',(88.8045545513055,55.9802981323048,13.0594838683586));
#71188=CARTESIAN_POINT('Ctrl Pts',(88.7551381270703,55.9744414043534,13.0970191699342));
#71189=CARTESIAN_POINT('Ctrl Pts',(88.6630723378032,55.9641289183963,13.1568660479542));
#71190=CARTESIAN_POINT('Ctrl Pts',(88.6215361272906,55.9596675673528,13.1806446411991));
#71191=CARTESIAN_POINT('Ctrl Pts',(88.543918809118,55.9515036019351,13.2194359510877));
#71192=CARTESIAN_POINT('Ctrl Pts',(88.5083000618796,55.9478186835245,13.2352344147259));
#71193=CARTESIAN_POINT('Ctrl Pts',(88.4468973566905,55.9415038336806,13.2591555280087));
#71194=CARTESIAN_POINT('Ctrl Pts',(88.4214772632858,55.9389001812605,13.2681375936926));
#71195=CARTESIAN_POINT('Ctrl Pts',(88.3845575805572,55.935119990449,13.2798754967061));
#71196=CARTESIAN_POINT('Ctrl Pts',(88.3732737228104,55.9339648463924,13.2832907271699));
#71197=CARTESIAN_POINT('Ctrl Pts',(88.3533927763155,55.9319288335368,13.2890070985774));
#71198=CARTESIAN_POINT('Ctrl Pts',(88.3448158145241,55.9310502166768,13.2913759293645));
#71199=CARTESIAN_POINT('Ctrl Pts',(88.3268740099108,55.9292112565562,13.2961288493208));
#71200=CARTESIAN_POINT('Ctrl Pts',(88.3175054793968,55.9282504474914,13.2984965533198));
#71201=CARTESIAN_POINT('Ctrl Pts',(88.2927871898879,55.9257132122966,13.3044443468397));
#71202=CARTESIAN_POINT('Ctrl Pts',(88.2773968146136,55.9241312153208,13.3078458440097));
#71203=CARTESIAN_POINT('Ctrl Pts',(88.1945481467689,55.9155984151958,13.3245457455559));
#71204=CARTESIAN_POINT('Ctrl Pts',(88.1261718680012,55.9084877933583,13.3326328507286));
#71205=CARTESIAN_POINT('Ctrl Pts',(87.9877614001459,55.893957779421,13.3377030957457));
#71206=CARTESIAN_POINT('Ctrl Pts',(87.9179401969865,55.8865593934954,13.3345065110059));
#71207=CARTESIAN_POINT('Ctrl Pts',(87.8331161611879,55.8776330889125,13.3235791523053));
#71208=CARTESIAN_POINT('Ctrl Pts',(87.8175355910835,55.8759965277639,13.3212766874952));
#71209=CARTESIAN_POINT('Ctrl Pts',(87.7838623231187,55.8724706459469,13.3156586122435));
#71210=CARTESIAN_POINT('Ctrl Pts',(87.7657897880709,55.8705853008424,13.3122384389581));
#71211=CARTESIAN_POINT('Ctrl Pts',(87.7408026231991,55.8679934735267,13.3069449966079));
#71212=CARTESIAN_POINT('Ctrl Pts',(87.7338212475204,55.8672709481157,13.3054043145988));
#71213=CARTESIAN_POINT('Ctrl Pts',(87.7219310811984,55.8660435663198,13.3026748406931));
#71214=CARTESIAN_POINT('Ctrl Pts',(87.7170158058652,55.8655371155654,13.3015156008071));
#71215=CARTESIAN_POINT('Ctrl Pts',(87.7066607861512,55.8644722731719,13.2990081292537));
#71216=CARTESIAN_POINT('Ctrl Pts',(87.7012228719673,55.8639142658272,13.2976531733077));
#71217=CARTESIAN_POINT('Ctrl Pts',(87.6862795906184,55.8623836775207,13.2938245478341));
#71218=CARTESIAN_POINT('Ctrl Pts',(87.6767933294442,55.8614151677584,13.2912764535884));
#71219=CARTESIAN_POINT('Ctrl Pts',(87.6195498995324,55.8555841546172,13.2751860318623));
#71220=CARTESIAN_POINT('Ctrl Pts',(87.572582548947,55.8508556616082,13.258960999801));
#71221=CARTESIAN_POINT('Ctrl Pts',(87.4545392366518,55.8388110971952,13.2102644351407));
#71222=CARTESIAN_POINT('Ctrl Pts',(87.3852977560678,55.8315797142518,13.1739198630397));
#71223=CARTESIAN_POINT('Ctrl Pts',(87.2834501966439,55.8200797552603,13.1078501448482));
#71224=CARTESIAN_POINT('Ctrl Pts',(87.2483078006617,55.815932636649,13.0824055177643));
#71225=CARTESIAN_POINT('Ctrl Pts',(87.2037137403427,55.8103660620342,13.0465009153038));
#71226=CARTESIAN_POINT('Ctrl Pts',(87.193032891288,55.8090082998732,13.037608420261));
#71227=CARTESIAN_POINT('Ctrl Pts',(87.1818808335678,55.8075631810874,13.028009395259));
#71228=CARTESIAN_POINT('Ctrl Pts',(87.181261574703,55.8074828445688,13.027475332124));
#71229=CARTESIAN_POINT('Ctrl Pts',(87.1806428354183,55.8074024841729,13.0269406741458));
#71230=CARTESIAN_POINT('Origin',(88.011,66.41344859951,12.066));
#71231=CARTESIAN_POINT('',(87.1806429093249,54.843673293217,13.0269407380092));
#71232=CARTESIAN_POINT('',(87.180642810782,55.0125145086225,13.0269406528573));
#71233=CARTESIAN_POINT('',(87.1806428354228,66.41344859951,13.0269406741497));
#71234=CARTESIAN_POINT('',(86.7410003566972,55.527636201329,12.0650481540224));
#71235=CARTESIAN_POINT('Ctrl Pts',(87.1806429093249,54.843673293217,13.0269407380092));
#71236=CARTESIAN_POINT('Ctrl Pts',(87.2040859914023,54.8469114146245,13.0471981052538));
#71237=CARTESIAN_POINT('Ctrl Pts',(87.2282722293485,54.8501250084737,13.0665992097863));
#71238=CARTESIAN_POINT('Ctrl Pts',(87.2611973410103,54.854314497518,13.0910836160516));
#71239=CARTESIAN_POINT('Ctrl Pts',(87.269310677785,54.8553326235955,13.096969165162));
#71240=CARTESIAN_POINT('Ctrl Pts',(87.2821036927062,54.8569149544343,13.1060202251068));
#71241=CARTESIAN_POINT('Ctrl Pts',(87.286735958499,54.8574832670097,13.1092514069836));
#71242=CARTESIAN_POINT('Ctrl Pts',(87.295539915687,54.8585544352337,13.1153055970788));
#71243=CARTESIAN_POINT('Ctrl Pts',(87.2997068940555,54.8590576529505,13.1181347288645));
#71244=CARTESIAN_POINT('Ctrl Pts',(87.3097535865277,54.860262129327,13.1248688691191));
#71245=CARTESIAN_POINT('Ctrl Pts',(87.315649241781,54.8609618021117,13.1287498040497));
#71246=CARTESIAN_POINT('Ctrl Pts',(87.3365033096173,54.8634129124974,13.1422295701707));
#71247=CARTESIAN_POINT('Ctrl Pts',(87.3516316689229,54.8651484473797,13.151564089469));
#71248=CARTESIAN_POINT('Ctrl Pts',(87.3798736032326,54.8683211831377,13.1681815786199));
#71249=CARTESIAN_POINT('Ctrl Pts',(87.3929292084119,54.8697622659677,13.1755554562751));
#71250=CARTESIAN_POINT('Ctrl Pts',(87.4621343540991,54.8772855254863,13.2130421631193));
#71251=CARTESIAN_POINT('Ctrl Pts',(87.5203651361938,54.8832252862192,13.239131800875));
#71252=CARTESIAN_POINT('Ctrl Pts',(87.6461155990688,54.895752141195,13.2844629624941));
#71253=CARTESIAN_POINT('Ctrl Pts',(87.7137551658093,54.9023265285547,13.3027035993879));
#71254=CARTESIAN_POINT('Ctrl Pts',(87.7996961509552,54.9107615380978,13.3184195314639));
#71255=CARTESIAN_POINT('Ctrl Pts',(87.8169090661628,54.9124544530802,13.3212022306194));
#71256=CARTESIAN_POINT('Ctrl Pts',(87.8450749501936,54.9152342164259,13.3251624530921));
#71257=CARTESIAN_POINT('Ctrl Pts',(87.8559960872159,54.9163143840079,13.3265534394645));
#71258=CARTESIAN_POINT('Ctrl Pts',(87.8756884630246,54.9182671961108,13.3288018198912));
#71259=CARTESIAN_POINT('Ctrl Pts',(87.8844532954881,54.9191381847808,13.3297102397482));
#71260=CARTESIAN_POINT('Ctrl Pts',(87.9032829363244,54.9210137277207,13.3314639629091));
#71261=CARTESIAN_POINT('Ctrl Pts',(87.9133497104382,54.9220191192657,13.3322805427928));
#71262=CARTESIAN_POINT('Ctrl Pts',(87.9412239486379,54.9248112037378,13.3342072490425));
#71263=CARTESIAN_POINT('Ctrl Pts',(87.9590458507476,54.9266056709485,13.3350622550181));
#71264=CARTESIAN_POINT('Ctrl Pts',(88.0478320843994,54.9355976370358,13.3374485498738));
#71265=CARTESIAN_POINT('Ctrl Pts',(88.1188044344926,54.9429618308533,13.3334036552168));
#71266=CARTESIAN_POINT('Ctrl Pts',(88.2659077508482,54.9585754415624,13.3125741458312));
#71267=CARTESIAN_POINT('Ctrl Pts',(88.3416059800984,54.966812746604,13.2946684021288));
#71268=CARTESIAN_POINT('Ctrl Pts',(88.4336089358017,54.9768506377623,13.2637807879992));
#71269=CARTESIAN_POINT('Ctrl Pts',(88.4518765132657,54.9788442793576,13.2571780600233));
#71270=CARTESIAN_POINT('Ctrl Pts',(88.4769874971889,54.9815796398335,13.2474448867976));
#71271=CARTESIAN_POINT('Ctrl Pts',(88.4839640122219,54.9823390342727,13.2446693435238));
#71272=CARTESIAN_POINT('Ctrl Pts',(88.4956031690392,54.9836045711307,13.2399188217257));
#71273=CARTESIAN_POINT('Ctrl Pts',(88.5002792391161,54.9841126237765,13.2379775860684));
#71274=CARTESIAN_POINT('Ctrl Pts',(88.5099642874028,54.985163954459,13.2338888378009));
#71275=CARTESIAN_POINT('Ctrl Pts',(88.5149712529474,54.9857069652724,13.2317369677214));
#71276=CARTESIAN_POINT('Ctrl Pts',(88.5283055910584,54.9871521663932,13.2259042260816));
#71277=CARTESIAN_POINT('Ctrl Pts',(88.5366077639636,54.9880510053829,13.2221658117659));
#71278=CARTESIAN_POINT('Ctrl Pts',(88.5797176826314,54.9927171849437,13.2021933176134));
#71279=CARTESIAN_POINT('Ctrl Pts',(88.6138211744567,54.9964047768003,13.1844733402355));
#71280=CARTESIAN_POINT('Ctrl Pts',(88.7479775790189,55.0111206640884,13.1068433184347));
#71281=CARTESIAN_POINT('Ctrl Pts',(88.8403578653001,55.021796356782,13.0348431115575));
#71282=CARTESIAN_POINT('Ctrl Pts',(88.9382898473904,55.0352971196386,12.9341044702504));
#71283=CARTESIAN_POINT('Ctrl Pts',(88.954469432111,55.0376118940403,12.9164922634366));
#71284=CARTESIAN_POINT('Ctrl Pts',(88.9775297832324,55.0410483523088,12.889921869592));
#71285=CARTESIAN_POINT('Ctrl Pts',(88.9848044870047,55.0421538151596,12.8813109039671));
#71286=CARTESIAN_POINT('Ctrl Pts',(88.9975750156283,55.0441341502075,12.865779848812));
#71287=CARTESIAN_POINT('Ctrl Pts',(89.0031151475007,55.0450071667658,12.8588969618853));
#71288=CARTESIAN_POINT('Ctrl Pts',(89.0147282203025,55.0468675605707,12.8441569679154));
#71289=CARTESIAN_POINT('Ctrl Pts',(89.0207816784624,55.0478556355033,12.8362853720696));
#71290=CARTESIAN_POINT('Ctrl Pts',(89.0369620343992,55.0505479179782,12.8147267718992));
#71291=CARTESIAN_POINT('Ctrl Pts',(89.046906550162,55.0522589998692,12.8009064035549));
#71292=CARTESIAN_POINT('Ctrl Pts',(89.063004245015,55.0551271093752,12.7775585499622));
#71293=CARTESIAN_POINT('Ctrl Pts',(89.0693133172775,55.0562781059743,12.7681405865538));
#71294=CARTESIAN_POINT('Ctrl Pts',(89.0934511235522,55.0607896549706,12.7310439898861));
#71295=CARTESIAN_POINT('Ctrl Pts',(89.1103251631192,55.064182084285,12.702763440202));
#71296=CARTESIAN_POINT('Ctrl Pts',(89.1524268988841,55.0733265036068,12.6255308062165));
#71297=CARTESIAN_POINT('Ctrl Pts',(89.1756013966874,55.0791247445234,12.5755415970106));
#71298=CARTESIAN_POINT('Ctrl Pts',(89.2172658428356,55.0913000703415,12.4678407324598));
#71299=CARTESIAN_POINT('Ctrl Pts',(89.2350240401574,55.0976639911057,12.4099772236351));
#71300=CARTESIAN_POINT('Ctrl Pts',(89.2514883187243,55.105188282214,12.3384976405336));
#71301=CARTESIAN_POINT('Ctrl Pts',(89.2541909957703,55.1065029004941,12.3258892597207));
#71302=CARTESIAN_POINT('Ctrl Pts',(89.2579139303162,55.1084381263569,12.3071315949462));
#71303=CARTESIAN_POINT('Ctrl Pts',(89.2590815911228,55.1090661496794,12.3010130711218));
#71304=CARTESIAN_POINT('Ctrl Pts',(89.261098392383,55.1101899056476,12.2900058578985));
#71305=CARTESIAN_POINT('Ctrl Pts',(89.2619639481163,55.1106864984279,12.2851205576061));
#71306=CARTESIAN_POINT('Ctrl Pts',(89.2638498696281,55.1118018617394,12.2741006328399));
#71307=CARTESIAN_POINT('Ctrl Pts',(89.2648538389336,55.1124197138887,12.2679634268865));
#71308=CARTESIAN_POINT('Ctrl Pts',(89.2677924644007,55.1143060562481,12.2491326324625));
#71309=CARTESIAN_POINT('Ctrl Pts',(89.2695798417916,55.1155668227158,12.2364162197954));
#71310=CARTESIAN_POINT('Ctrl Pts',(89.2733559097238,55.1185330416817,12.2062368409889));
#71311=CARTESIAN_POINT('Ctrl Pts',(89.2751756738861,55.120230833799,12.1887549367051));
#71312=CARTESIAN_POINT('Ctrl Pts',(89.2807383164286,55.1266703514273,12.1218574915991));
#71313=CARTESIAN_POINT('Ctrl Pts',(89.2819512812683,55.1313252810911,12.0722719978088));
#71314=CARTESIAN_POINT('Ctrl Pts',(89.2772213003621,55.1443406062693,11.933500151439));
#71315=CARTESIAN_POINT('Ctrl Pts',(89.2647782805744,55.152658992987,11.8448455241119));
#71316=CARTESIAN_POINT('Ctrl Pts',(89.2389976417875,55.1629343391081,11.741631882684));
#71317=CARTESIAN_POINT('Ctrl Pts',(89.2345154236301,55.1645965503466,11.7251146433086));
#71318=CARTESIAN_POINT('Ctrl Pts',(89.226629957002,55.1673363120501,11.6982188610567));
#71319=CARTESIAN_POINT('Ctrl Pts',(89.223424014454,55.1684075071326,11.6877842554212));
#71320=CARTESIAN_POINT('Ctrl Pts',(89.2173897708838,55.170350746179,11.6690097568055));
#71321=CARTESIAN_POINT('Ctrl Pts',(89.2146084302668,55.1712212051891,11.6606553698371));
#71322=CARTESIAN_POINT('Ctrl Pts',(89.2084287552842,55.1731030540761,11.6427178802393));
#71323=CARTESIAN_POINT('Ctrl Pts',(89.2050017838382,55.1741153354815,11.6331454035684));
#71324=CARTESIAN_POINT('Ctrl Pts',(89.195131384984,55.1769474419977,11.6065840806115));
#71325=CARTESIAN_POINT('Ctrl Pts',(89.1884380692579,55.1787754158089,11.5896916658243));
#71326=CARTESIAN_POINT('Ctrl Pts',(89.1765836386218,55.1818680123404,11.5615520411776));
#71327=CARTESIAN_POINT('Ctrl Pts',(89.1716160953457,55.1831260198307,11.5502256168485));
#71328=CARTESIAN_POINT('Ctrl Pts',(89.1511294988949,55.1881688028477,11.5053095428946));
#71329=CARTESIAN_POINT('Ctrl Pts',(89.1343128357946,55.1919934642355,11.472336186666));
#71330=CARTESIAN_POINT('Ctrl Pts',(89.0913196407651,55.2010937002782,11.3964220775805));
#71331=CARTESIAN_POINT('Ctrl Pts',(89.0639845346187,55.2063915789275,11.3542078717234));
#71332=CARTESIAN_POINT('Ctrl Pts',(88.9970197160169,55.2183096331906,11.2631240142454));
#71333=CARTESIAN_POINT('Ctrl Pts',(88.956108102467,55.2249155291813,11.2153427114922));
#71334=CARTESIAN_POINT('Ctrl Pts',(88.9047528117866,55.2323544844298,11.1636660906418));
#71335=CARTESIAN_POINT('Ctrl Pts',(88.8975992649569,55.233373254259,11.1566363000158));
#71336=CARTESIAN_POINT('Ctrl Pts',(88.8862870660021,55.2349563597144,11.1457802096424));
#71337=CARTESIAN_POINT('Ctrl Pts',(88.88218514564,55.2355248094521,11.1418959165428));
#71338=CARTESIAN_POINT('Ctrl Pts',(88.8743774057585,55.2365960735772,11.1346006123904));
#71339=CARTESIAN_POINT('Ctrl Pts',(88.8706771723082,55.2370992512437,11.1311842291833));
#71340=CARTESIAN_POINT('Ctrl Pts',(88.8617445346809,55.2383034116671,11.123034724142));
#71341=CARTESIAN_POINT('Ctrl Pts',(88.8564928188597,55.2390028107782,11.1183230104215));
#71342=CARTESIAN_POINT('Ctrl Pts',(88.8378883669359,55.2414518306441,11.1019093186362));
#71343=CARTESIAN_POINT('Ctrl Pts',(88.8243287911994,55.2431855846127,11.0904429254712));
#71344=CARTESIAN_POINT('Ctrl Pts',(88.7989012496192,55.2463544246719,11.0698395164523));
#71345=CARTESIAN_POINT('Ctrl Pts',(88.787104117171,55.2477933961443,11.0606211956387));
#71346=CARTESIAN_POINT('Ctrl Pts',(88.7243940675556,55.2552984193881,11.0133811955402));
#71347=CARTESIAN_POINT('Ctrl Pts',(88.6708394611965,55.2612227105853,10.9790083287027));
#71348=CARTESIAN_POINT('Ctrl Pts',(88.5476886727734,55.2743416357969,10.9124367230199));
#71349=CARTESIAN_POINT('Ctrl Pts',(88.4773127568304,55.28152812068,10.8822381056674));
#71350=CARTESIAN_POINT('Ctrl Pts',(88.3895815172152,55.2904751576018,10.8536355774732));
#71351=CARTESIAN_POINT('Ctrl Pts',(88.3744152027477,55.2920209245925,10.8490033710182));
#71352=CARTESIAN_POINT('Ctrl Pts',(88.3498532946961,55.2945255657283,10.8420015369077));
#71353=CARTESIAN_POINT('Ctrl Pts',(88.340509922056,55.2954786188591,10.8394532249739));
#71354=CARTESIAN_POINT('Ctrl Pts',(88.3225320028196,55.297313602444,10.8347701629403));
#71355=CARTESIAN_POINT('Ctrl Pts',(88.3139023398703,55.2981949379836,10.8326187683016));
#71356=CARTESIAN_POINT('Ctrl Pts',(88.2938228151596,55.3002473441214,10.8278363318714));
#71357=CARTESIAN_POINT('Ctrl Pts',(88.2823578509034,55.3014205101905,10.8252732344519));
#71358=CARTESIAN_POINT('Ctrl Pts',(88.2447302092167,55.3052763938942,10.8174076884091));
#71359=CARTESIAN_POINT('Ctrl Pts',(88.2184378952367,55.3079796710175,10.8127714422844));
#71360=CARTESIAN_POINT('Ctrl Pts',(88.1540095499799,55.3146331498071,10.8034933107744));
#71361=CARTESIAN_POINT('Ctrl Pts',(88.115773537145,55.3186069334515,10.7997469829524));
#71362=CARTESIAN_POINT('Ctrl Pts',(88.0290696715916,55.3276727565817,10.7952054828988));
#71363=CARTESIAN_POINT('Ctrl Pts',(87.9806059548392,55.33277946252,10.7954407251268));
#71364=CARTESIAN_POINT('Ctrl Pts',(87.8701306723697,55.3444479789913,10.8023018827884));
#71365=CARTESIAN_POINT('Ctrl Pts',(87.8083422543417,55.3509954344047,10.8107273917558));
#71366=CARTESIAN_POINT('Ctrl Pts',(87.7376212181031,55.3583769967046,10.8257321911751));
#71367=CARTESIAN_POINT('Ctrl Pts',(87.7278537306123,55.3593938296147,10.827925523675));
#71368=CARTESIAN_POINT('Ctrl Pts',(87.7126198933929,55.3609746043122,10.8315360770151));
#71369=CARTESIAN_POINT('Ctrl Pts',(87.7071356773418,55.3615426412743,10.8328745630933));
#71370=CARTESIAN_POINT('Ctrl Pts',(87.6967745369339,55.362613617301,10.8354766416908));
#71371=CARTESIAN_POINT('Ctrl Pts',(87.691896145026,55.3631169160003,10.8367326943809));
#71372=CARTESIAN_POINT('Ctrl Pts',(87.6801951740616,55.3643220295458,10.8398197271695));
#71373=CARTESIAN_POINT('Ctrl Pts',(87.6733801378873,55.3650222540222,10.8416786648779));
#71374=CARTESIAN_POINT('Ctrl Pts',(87.6494378289595,55.3674775834151,10.8484245389292));
#71375=CARTESIAN_POINT('Ctrl Pts',(87.6323969113525,55.3692167129644,10.853615150129));
#71376=CARTESIAN_POINT('Ctrl Pts',(87.6011797790079,55.3723973164102,10.8638463035105));
#71377=CARTESIAN_POINT('Ctrl Pts',(87.5869737098363,55.3738426652264,10.868783276847));
#71378=CARTESIAN_POINT('Ctrl Pts',(87.512731499737,55.3814029096302,10.8960717571628));
#71379=CARTESIAN_POINT('Ctrl Pts',(87.4543576003053,55.3873740559487,10.9226914621806));
#71380=CARTESIAN_POINT('Ctrl Pts',(87.3318070338228,55.4004864781314,10.9901984704248));
#71381=CARTESIAN_POINT('Ctrl Pts',(87.2687996584706,55.4076191059062,11.0326619362522));
#71382=CARTESIAN_POINT('Ctrl Pts',(87.1976837476851,55.4165053320255,11.0904657628469));
#71383=CARTESIAN_POINT('Ctrl Pts',(87.1855932716191,55.4180478191361,11.1006741205332));
#71384=CARTESIAN_POINT('Ctrl Pts',(87.1664209338989,55.4205484572738,11.1174854483845));
#71385=CARTESIAN_POINT('Ctrl Pts',(87.1592179998855,55.4215008216204,11.1239484807545));
#71386=CARTESIAN_POINT('Ctrl Pts',(87.1458206712316,55.4232972895803,11.136248870789));
#71387=CARTESIAN_POINT('Ctrl Pts',(87.1396096859145,55.4241405625297,11.1420674566059));
#71388=CARTESIAN_POINT('Ctrl Pts',(87.1255300537694,55.4260767146025,11.1555258105711));
#71389=CARTESIAN_POINT('Ctrl Pts',(87.117701088193,55.4271712929331,11.1632058318453));
#71390=CARTESIAN_POINT('Ctrl Pts',(87.0932318038231,55.4306511313656,11.1878395116583));
#71391=CARTESIAN_POINT('Ctrl Pts',(87.0769684081202,55.4330523134773,11.2051579141156));
#71392=CARTESIAN_POINT('Ctrl Pts',(87.0393535103477,55.438828271075,11.2475342040959));
#71393=CARTESIAN_POINT('Ctrl Pts',(87.0184729813944,55.4422194414489,11.2729849765765));
#71394=CARTESIAN_POINT('Ctrl Pts',(86.9653675261235,55.4513631494686,11.3431006451047));
#71395=CARTESIAN_POINT('Ctrl Pts',(86.9350202891547,55.45716199149,11.3890972209607));
#71396=CARTESIAN_POINT('Ctrl Pts',(86.8778079322664,55.4693395549267,11.4894318498634));
#71397=CARTESIAN_POINT('Ctrl Pts',(86.851645129447,55.4757051118253,11.544029404581));
#71398=CARTESIAN_POINT('Ctrl Pts',(86.8247415664918,55.483230973946,11.6122851503339));
#71399=CARTESIAN_POINT('Ctrl Pts',(86.8201962072513,55.4845456038203,11.6243523923442));
#71400=CARTESIAN_POINT('Ctrl Pts',(86.8137286009386,55.4864808433209,11.642349208719));
#71401=CARTESIAN_POINT('Ctrl Pts',(86.8116651510223,55.4871088688318,11.6482264704523));
#71402=CARTESIAN_POINT('Ctrl Pts',(86.8080359032133,55.488232627002,11.6588120865574));
#71403=CARTESIAN_POINT('Ctrl Pts',(86.8064543751589,55.488729219813,11.6635146512866));
#71404=CARTESIAN_POINT('Ctrl Pts',(86.8029526811489,55.4898445810724,11.6741322361196));
#71405=CARTESIAN_POINT('Ctrl Pts',(86.8010483461148,55.490462431156,11.6800522442026));
#71406=CARTESIAN_POINT('Ctrl Pts',(86.7971388503017,55.491755591094,11.6925190974547));
#71407=CARTESIAN_POINT('Ctrl Pts',(86.7951429817796,55.4924303833304,11.6990686795843));
#71408=CARTESIAN_POINT('Ctrl Pts',(86.7899388940344,55.4942308947352,11.7166550875056));
#71409=CARTESIAN_POINT('Ctrl Pts',(86.7868272490698,55.4953518070467,11.727720235947));
#71410=CARTESIAN_POINT('Ctrl Pts',(86.7554955425682,55.5071464108204,11.8452365619051));
#71411=CARTESIAN_POINT('Ctrl Pts',(86.7410829143962,55.5172338869301,11.9548956180338));
#71412=CARTESIAN_POINT('Ctrl Pts',(86.7410003566972,55.527636201329,12.0650481540224));
#71413=CARTESIAN_POINT('Ctrl Pts',(86.7410003556522,55.5276363331034,12.0650495494126));
#71414=CARTESIAN_POINT('Ctrl Pts',(86.7409762743704,55.5306750427983,12.0972271498695));
#71415=CARTESIAN_POINT('Ctrl Pts',(86.7421751037416,55.5337325688994,12.1293919897642));
#71416=CARTESIAN_POINT('Ctrl Pts',(86.7461044628181,55.5387526504158,12.1815121376383));
#71417=CARTESIAN_POINT('Ctrl Pts',(86.7480903153629,55.5406944456528,12.201509414993));
#71418=CARTESIAN_POINT('Ctrl Pts',(86.7517745285109,55.5436247217039,12.2313824890764));
#71419=CARTESIAN_POINT('Ctrl Pts',(86.7531168155513,55.544602413178,12.2412998468796));
#71420=CARTESIAN_POINT('Ctrl Pts',(86.7557867378001,55.5463977939441,12.2594129926097));
#71421=CARTESIAN_POINT('Ctrl Pts',(86.7570778223769,55.5472143111321,12.2676136990852));
#71422=CARTESIAN_POINT('Ctrl Pts',(86.7599037053006,55.5489020927059,12.2844847499268));
#71423=CARTESIAN_POINT('Ctrl Pts',(86.7614484569822,55.5497736266679,12.2931529352528));
#71424=CARTESIAN_POINT('Ctrl Pts',(86.7651086574365,55.5517314974193,12.3125233620957));
#71425=CARTESIAN_POINT('Ctrl Pts',(86.7672720985356,55.552819295837,12.3232156557579));
#71426=CARTESIAN_POINT('Ctrl Pts',(86.7740470906868,55.5560354678659,12.3546129645832));
#71427=CARTESIAN_POINT('Ctrl Pts',(86.7790396688936,55.5581757116014,12.3752305726424));
#71428=CARTESIAN_POINT('Ctrl Pts',(86.8029216734197,55.5675285441556,12.4640662498715));
#71429=CARTESIAN_POINT('Ctrl Pts',(86.8269758864899,55.5748982163994,12.5307504349586));
#71430=CARTESIAN_POINT('Ctrl Pts',(86.891365947548,55.5911638822733,12.6712633640904));
#71431=CARTESIAN_POINT('Ctrl Pts',(86.933740207904,55.6000562040281,12.7438189421686));
#71432=CARTESIAN_POINT('Ctrl Pts',(86.9893733214197,55.6097541951035,12.8205185549781));
#71433=CARTESIAN_POINT('Ctrl Pts',(86.9959011505201,55.6108662837773,12.8292782420139));
#71434=CARTESIAN_POINT('Ctrl Pts',(87.0062550229444,55.6125893391099,12.8428042573247));
#71435=CARTESIAN_POINT('Ctrl Pts',(87.0100035587952,55.6132051040285,12.8476287184431));
#71436=CARTESIAN_POINT('Ctrl Pts',(87.0165532918571,55.6142669539492,12.8559339862698));
#71437=CARTESIAN_POINT('Ctrl Pts',(87.0193381633471,55.6147141194907,12.859427225468));
#71438=CARTESIAN_POINT('Ctrl Pts',(87.0259595389537,55.6157672058953,12.8676435066403));
#71439=CARTESIAN_POINT('Ctrl Pts',(87.029811639287,55.6163720082429,12.8723537859249));
#71440=CARTESIAN_POINT('Ctrl Pts',(87.0414556854975,55.6181775484707,12.8863849129415));
#71441=CARTESIAN_POINT('Ctrl Pts',(87.0493480404108,55.6193714896878,12.8956222824675));
#71442=CARTESIAN_POINT('Ctrl Pts',(87.0956383874749,55.6262151565257,12.9482529719988));
#71443=CARTESIAN_POINT('Ctrl Pts',(87.1368265374621,55.6316892735561,12.9890786360942));
#71444=CARTESIAN_POINT('Ctrl Pts',(87.1806428950461,55.6371283284805,13.0269407256708));
#71445=CARTESIAN_POINT('Ctrl Pts',(87.1806428354183,55.8074024841729,13.0269406741458));
#71446=CARTESIAN_POINT('Ctrl Pts',(87.1742426907308,55.806571248508,13.0214102536541));
#71447=CARTESIAN_POINT('Ctrl Pts',(87.1678981387326,55.8057374559431,13.015816187997));
#71448=CARTESIAN_POINT('Ctrl Pts',(87.1549254284368,55.8040118150213,13.0041456057867));
#71449=CARTESIAN_POINT('Ctrl Pts',(87.1483050232558,55.8031196747329,12.9980612727825));
#71450=CARTESIAN_POINT('Ctrl Pts',(87.1323477367404,55.8009405552997,12.9830804311961));
#71451=CARTESIAN_POINT('Ctrl Pts',(87.1230809352282,55.7996505157731,12.974111237607));
#71452=CARTESIAN_POINT('Ctrl Pts',(87.0912541366452,55.7951311148999,12.9423536738375));
#71453=CARTESIAN_POINT('Ctrl Pts',(87.0694241995254,55.7918710630158,12.9188556513527));
#71454=CARTESIAN_POINT('Ctrl Pts',(86.9912294539478,55.7795550695985,12.8280212070575));
#71455=CARTESIAN_POINT('Ctrl Pts',(86.9410128016627,55.7702866727908,12.7557322484035));
#71456=CARTESIAN_POINT('Ctrl Pts',(86.8810716336288,55.7572073513683,12.6469390278745));
#71457=CARTESIAN_POINT('Ctrl Pts',(86.8648649784342,55.7533834806886,12.614272950054));
#71458=CARTESIAN_POINT('Ctrl Pts',(86.8413834412009,55.7473839179663,12.5613358715389));
#71459=CARTESIAN_POINT('Ctrl Pts',(86.833179765032,55.7451781626739,12.5414999493231));
#71460=CARTESIAN_POINT('Ctrl Pts',(86.8227673631107,55.7422288238544,12.5143977006385));
#71461=CARTESIAN_POINT('Ctrl Pts',(86.8201157952495,55.741463096499,12.5073072836044));
#71462=CARTESIAN_POINT('Ctrl Pts',(86.8157757990795,55.7401850495687,12.495377883066));
#71463=CARTESIAN_POINT('Ctrl Pts',(86.8140530169991,55.7396708031507,12.4905517419504));
#71464=CARTESIAN_POINT('Ctrl Pts',(86.8105604530218,55.7386139239542,12.4805775255028));
#71465=CARTESIAN_POINT('Ctrl Pts',(86.8087944811187,55.73807151245,12.4754282905537));
#71466=CARTESIAN_POINT('Ctrl Pts',(86.804171467344,55.7366293603664,12.4616606212));
#71467=CARTESIAN_POINT('Ctrl Pts',(86.8013735518153,55.7357329475437,12.4530223607614));
#71468=CARTESIAN_POINT('Ctrl Pts',(86.7885731014044,55.7315129327186,12.4120068692531));
#71469=CARTESIAN_POINT('Ctrl Pts',(86.7797750485167,55.7282502967681,12.379263553727));
#71470=CARTESIAN_POINT('Ctrl Pts',(86.7515634702555,55.7160746554525,12.2545475702932));
#71471=CARTESIAN_POINT('Ctrl Pts',(86.7410660618885,55.7074172420535,12.1608707216829));
#71472=CARTESIAN_POINT('Ctrl Pts',(86.7409697010484,55.6943772943106,12.0231361436092));
#71473=CARTESIAN_POINT('Ctrl Pts',(86.7432000208007,55.6901959042556,11.9794171160793));
#71474=CARTESIAN_POINT('Ctrl Pts',(86.7491444094718,55.6845569953527,11.921692688553));
#71475=CARTESIAN_POINT('Ctrl Pts',(86.750847627602,55.6831618261989,11.9075068137284));
#71476=CARTESIAN_POINT('Ctrl Pts',(86.7540615337585,55.6808406807999,11.884084580041));
#71477=CARTESIAN_POINT('Ctrl Pts',(86.7554356972621,55.6799190312747,11.8748304471702));
#71478=CARTESIAN_POINT('Ctrl Pts',(86.7583385394581,55.6781003474421,11.8566653464927));
#71479=CARTESIAN_POINT('Ctrl Pts',(86.7598603862993,55.6772035809256,11.8477538359257));
#71480=CARTESIAN_POINT('Ctrl Pts',(86.7637428491864,55.6750428498231,11.8263960044005));
#71481=CARTESIAN_POINT('Ctrl Pts',(86.7661947521036,55.6737760704334,11.8139675817289));
#71482=CARTESIAN_POINT('Ctrl Pts',(86.7756699159317,55.6692034389198,11.7694562837635));
#71483=CARTESIAN_POINT('Ctrl Pts',(86.7837503728528,55.6658648468416,11.7376154001105));
#71484=CARTESIAN_POINT('Ctrl Pts',(86.8079302954473,55.6570951543037,11.6557814773996));
#71485=CARTESIAN_POINT('Ctrl Pts',(86.8259113657069,55.6516144725774,11.6064138376836));
#71486=CARTESIAN_POINT('Ctrl Pts',(86.8810744508484,55.6370988190487,11.4799285130019));
#71487=CARTESIAN_POINT('Ctrl Pts',(86.9230879715157,55.6280207865556,11.4051959960656));
#71488=CARTESIAN_POINT('Ctrl Pts',(86.9788828632682,55.618093704215,11.3258884163083));
#71489=CARTESIAN_POINT('Ctrl Pts',(86.9855936752824,55.6169287270587,11.3166183598834));
#71490=CARTESIAN_POINT('Ctrl Pts',(86.9960217540745,55.6151632803129,11.3026158663387));
#71491=CARTESIAN_POINT('Ctrl Pts',(86.9996485730698,55.614557239594,11.2978174227993));
#71492=CARTESIAN_POINT('Ctrl Pts',(87.0063041866729,55.6134596926859,11.2891405961505));
#71493=CARTESIAN_POINT('Ctrl Pts',(87.0093215168426,55.6129674713452,11.2852539275462));
#71494=CARTESIAN_POINT('Ctrl Pts',(87.0163328431421,55.6118358563024,11.2763300901002));
#71495=CARTESIAN_POINT('Ctrl Pts',(87.0203426012824,55.6111975800186,11.2713055653412));
#71496=CARTESIAN_POINT('Ctrl Pts',(87.0331885262414,55.6091798680469,11.255457004686));
#71497=CARTESIAN_POINT('Ctrl Pts',(87.0421657495625,55.6078097918092,11.2447476151732));
#71498=CARTESIAN_POINT('Ctrl Pts',(87.0642164520096,55.6045323564112,11.2193071985131));
#71499=CARTESIAN_POINT('Ctrl Pts',(87.0774597481987,55.6026350127563,11.2047273880955));
#71500=CARTESIAN_POINT('Ctrl Pts',(87.1332602744334,55.5948940046685,11.1460956961943));
#71501=CARTESIAN_POINT('Ctrl Pts',(87.1786407943541,55.5891773623421,11.1048389347805));
#71502=CARTESIAN_POINT('Ctrl Pts',(87.2842425587871,55.5765995191281,11.0219446131959));
#71503=CARTESIAN_POINT('Ctrl Pts',(87.3454292036532,55.5697487153235,10.9819146564514));
#71504=CARTESIAN_POINT('Ctrl Pts',(87.4251268937649,55.5610136695561,10.9390753592568));
#71505=CARTESIAN_POINT('Ctrl Pts',(87.4407148192381,55.5593140832851,10.9311074124511));
#71506=CARTESIAN_POINT('Ctrl Pts',(87.4663830358684,55.556525752762,10.9186491441039));
#71507=CARTESIAN_POINT('Ctrl Pts',(87.4763664114891,55.5554437618659,10.9139633116163));
#71508=CARTESIAN_POINT('Ctrl Pts',(87.494433914038,55.5534891598212,10.9057685044401));
#71509=CARTESIAN_POINT('Ctrl Pts',(87.5024960676586,55.5526182200004,10.9022124827278));
#71510=CARTESIAN_POINT('Ctrl Pts',(87.5198614278259,55.5507444504161,10.8947679283834));
#71511=CARTESIAN_POINT('Ctrl Pts',(87.5291751701245,55.5497407957872,10.8909057565745));
#71512=CARTESIAN_POINT('Ctrl Pts',(87.555023959982,55.5469581441455,10.8805458825034));
#71513=CARTESIAN_POINT('Ctrl Pts',(87.5716500965028,55.5451714577499,10.8742839289602));
#71514=CARTESIAN_POINT('Ctrl Pts',(87.6092450208936,55.5411357282,10.8610180476422));
#71515=CARTESIAN_POINT('Ctrl Pts',(87.6302757887951,55.5388810400453,10.854208972585));
#71516=CARTESIAN_POINT('Ctrl Pts',(87.7240536883532,55.5288349419768,10.8265287804316));
#71517=CARTESIAN_POINT('Ctrl Pts',(87.7983936782144,55.5208784789874,10.8116388117117));
#71518=CARTESIAN_POINT('Ctrl Pts',(87.93391375377,55.5065057028491,10.7968907971071));
#71519=CARTESIAN_POINT('Ctrl Pts',(87.9946253038751,55.5001175917607,10.7946565124833));
#71520=CARTESIAN_POINT('Ctrl Pts',(88.068156867777,55.4925702114449,10.7972213210792));
#71521=CARTESIAN_POINT('Ctrl Pts',(88.0810358988616,55.4912555506162,10.7978670169152));
#71522=CARTESIAN_POINT('Ctrl Pts',(88.1001183802775,55.4893203529465,10.7991153559433));
#71523=CARTESIAN_POINT('Ctrl Pts',(88.1063301887382,55.4886923992545,10.7995676298504));
#71524=CARTESIAN_POINT('Ctrl Pts',(88.1174830587634,55.4875688192735,10.8004621844496));
#71525=CARTESIAN_POINT('Ctrl Pts',(88.1224250866354,55.4870723326713,10.800887729211));
#71526=CARTESIAN_POINT('Ctrl Pts',(88.1335549875207,55.4859572877434,10.8019118236752));
#71527=CARTESIAN_POINT('Ctrl Pts',(88.1397411212455,55.4853396467555,10.8025268613153));
#71528=CARTESIAN_POINT('Ctrl Pts',(88.158682648607,55.4834542227593,10.8045506314272));
#71529=CARTESIAN_POINT('Ctrl Pts',(88.1714220728153,55.4821941541104,10.8061073541215));
#71530=CARTESIAN_POINT('Ctrl Pts',(88.2015334496605,55.479229805268,10.8102510655707));
#71531=CARTESIAN_POINT('Ctrl Pts',(88.2188801142066,55.4775331734065,10.8130058522676));
#71532=CARTESIAN_POINT('Ctrl Pts',(88.2848761166757,55.4711002424619,10.8248950022527));
#71533=CARTESIAN_POINT('Ctrl Pts',(88.3330375722939,55.4664505605265,10.8365112492117));
#71534=CARTESIAN_POINT('Ctrl Pts',(88.4659205023589,55.453431763719,10.8769093455519));
#71535=CARTESIAN_POINT('Ctrl Pts',(88.5484422552698,55.4451050334358,10.9118588672234));
#71536=CARTESIAN_POINT('Ctrl Pts',(88.641569196846,55.4348212070188,10.9634687499155));
#71537=CARTESIAN_POINT('Ctrl Pts',(88.6563626355999,55.4331595936727,10.9720623086464));
#71538=CARTESIAN_POINT('Ctrl Pts',(88.6803008697219,55.4304207292695,10.9866226618151));
#71539=CARTESIAN_POINT('Ctrl Pts',(88.6895507011338,55.4293498282405,10.9924134780315));
#71540=CARTESIAN_POINT('Ctrl Pts',(88.7061252976115,55.4274070730296,11.0030896936527));
#71541=CARTESIAN_POINT('Ctrl Pts',(88.7134761742902,55.4265368025766,11.0079335023704));
#71542=CARTESIAN_POINT('Ctrl Pts',(88.7292058128093,55.4246553110747,11.0185346053922));
#71543=CARTESIAN_POINT('Ctrl Pts',(88.7375669132263,55.4236431984878,11.024316819932));
#71544=CARTESIAN_POINT('Ctrl Pts',(88.7606746721042,55.4208114428163,11.0407107994589));
#71545=CARTESIAN_POINT('Ctrl Pts',(88.7752636493158,55.4189836520927,11.0515390370486));
#71546=CARTESIAN_POINT('Ctrl Pts',(88.7993845043506,55.4158913333416,11.0702576572477));
#71547=CARTESIAN_POINT('Ctrl Pts',(88.8090428748285,55.4146334189762,11.0779815370658));
#71548=CARTESIAN_POINT('Ctrl Pts',(88.8471412925432,55.4095909467583,11.1093722502589));
#71549=CARTESIAN_POINT('Ctrl Pts',(88.8746509048974,55.405766506366,11.1341333708096));
#71550=CARTESIAN_POINT('Ctrl Pts',(88.9368848617311,55.3966663165167,11.1952747129193));
#71551=CARTESIAN_POINT('Ctrl Pts',(88.9706077975009,55.3913682524108,11.2325868244853));
#71552=CARTESIAN_POINT('Ctrl Pts',(89.0413098159751,55.3794494169718,11.3208106873007));
#71553=CARTESIAN_POINT('Ctrl Pts',(89.0769058912529,55.3728429243946,11.3726801033294));
#71554=CARTESIAN_POINT('Ctrl Pts',(89.1135662794786,55.3654035246424,11.4356444259484));
#71555=CARTESIAN_POINT('Ctrl Pts',(89.1185092522852,55.3643848682818,11.4443700221243));
#71556=CARTESIAN_POINT('Ctrl Pts',(89.1260740897032,55.3628019725235,11.4581006053044));
#71557=CARTESIAN_POINT('Ctrl Pts',(89.1287666216006,55.362233619658,11.463065771579));
#71558=CARTESIAN_POINT('Ctrl Pts',(89.1337966887918,55.3611625705363,11.4724909877047));
#71559=CARTESIAN_POINT('Ctrl Pts',(89.1361408579918,55.3606595109032,11.4769470281411));
#71560=CARTESIAN_POINT('Ctrl Pts',(89.1417050304948,55.3594556943809,11.4876783970367));
#71561=CARTESIAN_POINT('Ctrl Pts',(89.1448993854837,55.3587565198449,11.4939668413559));
#71562=CARTESIAN_POINT('Ctrl Pts',(89.1559457301189,55.3563086390901,11.5161689752502));
#71563=CARTESIAN_POINT('Ctrl Pts',(89.1635170235174,55.3545757823827,11.532221482241));
#71564=CARTESIAN_POINT('Ctrl Pts',(89.176846448266,55.3514088117629,11.5620894551549));
#71565=CARTESIAN_POINT('Ctrl Pts',(89.1827013978177,55.3499708120719,11.5758575051926));
#71566=CARTESIAN_POINT('Ctrl Pts',(89.2121126492015,55.3424738820711,11.6485599062844));
#71567=CARTESIAN_POINT('Ctrl Pts',(89.2314720252821,55.3365564301679,11.7091002578572));
#71568=CARTESIAN_POINT('Ctrl Pts',(89.2639912469591,55.3234442438341,11.8451908335917));
#71569=CARTESIAN_POINT('Ctrl Pts',(89.2750056182029,55.3162576590329,11.9209813796044));
#71570=CARTESIAN_POINT('Ctrl Pts',(89.2800006411937,55.3073059920968,12.0131760118662));
#71571=CARTESIAN_POINT('Ctrl Pts',(89.2805626469994,55.3057555702018,12.0290726077536));
#71572=CARTESIAN_POINT('Ctrl Pts',(89.2809864284081,55.3032453774918,12.0546669871657));
#71573=CARTESIAN_POINT('Ctrl Pts',(89.2810359303341,55.3022914774543,12.0643604180708));
#71574=CARTESIAN_POINT('Ctrl Pts',(89.2809181040722,55.3004561840916,12.08294154406));
#71575=CARTESIAN_POINT('Ctrl Pts',(89.2807684311442,55.2995753954288,12.091828821345));
#71576=CARTESIAN_POINT('Ctrl Pts',(89.28020511378,55.2975262485786,12.112430187171));
#71577=CARTESIAN_POINT('Ctrl Pts',(89.2797225635363,55.2963558143991,12.1241413468149));
#71578=CARTESIAN_POINT('Ctrl Pts',(89.277618482419,55.2925183263846,12.1623429421642));
#71579=CARTESIAN_POINT('Ctrl Pts',(89.2753288161302,55.2898309829731,12.188787290903));
#71580=CARTESIAN_POINT('Ctrl Pts',(89.2677401360237,55.2832266061911,12.2529623153027));
#71581=CARTESIAN_POINT('Ctrl Pts',(89.2615687161592,55.2792864589947,12.2905615789233));
#71582=CARTESIAN_POINT('Ctrl Pts',(89.2436656760791,55.2702208523047,12.3755367917411));
#71583=CARTESIAN_POINT('Ctrl Pts',(89.230873951759,55.2650792159383,12.4226295924784));
#71584=CARTESIAN_POINT('Ctrl Pts',(89.1955935016051,55.2533546611971,12.5281036600316));
#71585=CARTESIAN_POINT('Ctrl Pts',(89.1714329956013,55.2467860221635,12.5858069028569));
#71586=CARTESIAN_POINT('Ctrl Pts',(89.1385808577845,55.2393838216216,12.6504328111946));
#71587=CARTESIAN_POINT('Ctrl Pts',(89.1339367853736,55.238366444452,12.6593070878795));
#71588=CARTESIAN_POINT('Ctrl Pts',(89.1265114177256,55.2367850879517,12.6730964887112));
#71589=CARTESIAN_POINT('Ctrl Pts',(89.1238016768983,55.2362170076618,12.678049264468));
#71590=CARTESIAN_POINT('Ctrl Pts',(89.1186123770424,55.2351461490309,12.6873856956811));
#71591=CARTESIAN_POINT('Ctrl Pts',(89.1161397446226,55.2346430097185,12.6917727282085));
#71592=CARTESIAN_POINT('Ctrl Pts',(89.1101387096611,55.2334385649127,12.7022734617776));
#71593=CARTESIAN_POINT('Ctrl Pts',(89.1065853045363,55.2327388462045,12.7083726880008));
#71594=CARTESIAN_POINT('Ctrl Pts',(89.0939019621382,55.2302868082073,12.7297315218877));
#71595=CARTESIAN_POINT('Ctrl Pts',(89.0845019083017,55.2285504098872,12.7448298469503));
#71596=CARTESIAN_POINT('Ctrl Pts',(89.0665912226597,55.2253756918107,12.7722947592354));
#71597=CARTESIAN_POINT('Ctrl Pts',(89.0581729216091,55.2239334930981,12.7847169412609));
#71598=CARTESIAN_POINT('Ctrl Pts',(89.0128106847907,55.2164002903223,12.8491644170682));
#71599=CARTESIAN_POINT('Ctrl Pts',(88.9722019895771,55.2104520684762,12.8985043311548));
#71600=CARTESIAN_POINT('Ctrl Pts',(88.8797238794693,55.197924516813,12.9950313099526));
#71601=CARTESIAN_POINT('Ctrl Pts',(88.8273225951367,55.191358018066,13.0413950201957));
#71602=CARTESIAN_POINT('Ctrl Pts',(88.757429170904,55.1829328304002,13.0936414471728));
#71603=CARTESIAN_POINT('Ctrl Pts',(88.7432643871098,55.181241416312,13.1037823710239));
#71604=CARTESIAN_POINT('Ctrl Pts',(88.7198194208111,55.1784637255298,13.1198482373213));
#71605=CARTESIAN_POINT('Ctrl Pts',(88.7106624332172,55.1773841144651,13.1259497815893));
#71606=CARTESIAN_POINT('Ctrl Pts',(88.6940335493441,55.1754320684973,13.1367206831172));
#71607=CARTESIAN_POINT('Ctrl Pts',(88.6865900351724,55.174561286132,13.1414327990515));
#71608=CARTESIAN_POINT('Ctrl Pts',(88.6705087778154,55.172685927221,13.1513802021207));
#71609=CARTESIAN_POINT('Ctrl Pts',(88.6618564685076,55.1716805118497,13.1565905984606));
#71610=CARTESIAN_POINT('Ctrl Pts',(88.6377439880494,55.1688876621025,13.1707219375318));
#71611=CARTESIAN_POINT('Ctrl Pts',(88.6221572253211,55.1670924441391,13.1794205622875));
#71612=CARTESIAN_POINT('Ctrl Pts',(88.5414031664841,55.1578366459231,13.2222811190804));
#71613=CARTESIAN_POINT('Ctrl Pts',(88.4735533902345,55.1501956800951,13.2510541277681));
#71614=CARTESIAN_POINT('Ctrl Pts',(88.3251768370904,55.1337886744991,13.2992861847797));
#71615=CARTESIAN_POINT('Ctrl Pts',(88.2444405521378,55.1250339102652,13.317083399324));
#71616=CARTESIAN_POINT('Ctrl Pts',(88.1496223296431,55.1152170520254,13.3284789871405));
#71617=CARTESIAN_POINT('Ctrl Pts',(88.1366781178288,55.1138871386668,13.3298332168037));
#71618=CARTESIAN_POINT('Ctrl Pts',(88.1173784652334,55.1119214474161,13.3315528777645));
#71619=CARTESIAN_POINT('Ctrl Pts',(88.111038016509,55.1112784213846,13.3320698502638));
#71620=CARTESIAN_POINT('Ctrl Pts',(88.0996299317929,55.1101266946505,13.3329137766099));
#71621=CARTESIAN_POINT('Ctrl Pts',(88.0945637425395,55.1096170851142,13.3332580193756));
#71622=CARTESIAN_POINT('Ctrl Pts',(88.0840856217954,55.1085670854476,13.333906885253));
#71623=CARTESIAN_POINT('Ctrl Pts',(88.078673579823,55.108026932576,13.3342072655776));
#71624=CARTESIAN_POINT('Ctrl Pts',(88.0642980489005,55.1065975417128,13.3349128499314));
#71625=CARTESIAN_POINT('Ctrl Pts',(88.0553316254386,55.10571152923,13.3352577463317));
#71626=CARTESIAN_POINT('Ctrl Pts',(88.0099968123367,55.1012561373778,13.3365205367272));
#71627=CARTESIAN_POINT('Ctrl Pts',(87.973599452576,55.0977581144267,13.3359706459247));
#71628=CARTESIAN_POINT('Ctrl Pts',(87.8341536538382,55.0844775103858,13.3278615020794));
#71629=CARTESIAN_POINT('Ctrl Pts',(87.7321525664578,55.0749877735975,13.3093080343236));
#71630=CARTESIAN_POINT('Ctrl Pts',(87.600567667142,55.0618650497292,13.2683462474039));
#71631=CARTESIAN_POINT('Ctrl Pts',(87.5680491518291,55.058549161303,13.2567498776087));
#71632=CARTESIAN_POINT('Ctrl Pts',(87.5237892189435,55.0539041175254,13.238902517896));
#71633=CARTESIAN_POINT('Ctrl Pts',(87.5116107164062,55.0526118503887,13.2337692295014));
#71634=CARTESIAN_POINT('Ctrl Pts',(87.4919832333254,55.0505045495865,13.2251329982411));
#71635=CARTESIAN_POINT('Ctrl Pts',(87.48448400245,55.0496934762607,13.221745909812));
#71636=CARTESIAN_POINT('Ctrl Pts',(87.4707144379843,55.0481929128675,13.2153649490223));
#71637=CARTESIAN_POINT('Ctrl Pts',(87.4644346847937,55.0475041670229,13.2123920035873));
#71638=CARTESIAN_POINT('Ctrl Pts',(87.4500943428532,55.0459209956294,13.2054584245364));
#71639=CARTESIAN_POINT('Ctrl Pts',(87.4420508550704,55.0450254120678,13.2014635693395));
#71640=CARTESIAN_POINT('Ctrl Pts',(87.4239617918976,55.0429936471862,13.1922390496625));
#71641=CARTESIAN_POINT('Ctrl Pts',(87.4139426093247,55.0418557866997,13.1869597252703));
#71642=CARTESIAN_POINT('Ctrl Pts',(87.3879970054156,55.0388755238957,13.1728419100577));
#71643=CARTESIAN_POINT('Ctrl Pts',(87.3721884418009,55.0370259961618,13.1637939024786));
#71644=CARTESIAN_POINT('Ctrl Pts',(87.3242346711514,55.0313083839228,13.1349611345074));
#71645=CARTESIAN_POINT('Ctrl Pts',(87.2927754174569,55.0274048953664,13.1140826914261));
#71646=CARTESIAN_POINT('Ctrl Pts',(87.2341947981403,55.0198358239701,13.0713277928951));
#71647=CARTESIAN_POINT('Ctrl Pts',(87.2069545388486,55.0161792082546,13.0496768462902));
#71648=CARTESIAN_POINT('Ctrl Pts',(87.180642810782,55.0125145086225,13.0269406528573));
#71649=CARTESIAN_POINT('Origin',(88.011,66.41344859951,12.066));
#71650=CARTESIAN_POINT('',(87.1806428502938,54.0480645842206,13.0269406869999));
#71651=CARTESIAN_POINT('',(87.1806428209146,54.2176482202995,13.026940661613));
#71652=CARTESIAN_POINT('',(87.1806428354228,66.41344859951,13.0269406741497));
#71653=CARTESIAN_POINT('Ctrl Pts',(87.1806428502938,54.0480645842206,13.0269406869999));
#71654=CARTESIAN_POINT('Ctrl Pts',(87.2477090573159,54.0570744662908,13.0848931759078));
#71655=CARTESIAN_POINT('Ctrl Pts',(87.3206512326996,54.0663624465791,13.1356597057593));
#71656=CARTESIAN_POINT('Ctrl Pts',(87.4397015010786,54.0806929260796,13.2012334320204));
#71657=CARTESIAN_POINT('Ctrl Pts',(87.4823742143646,54.0856792126345,13.2217215612789));
#71658=CARTESIAN_POINT('Ctrl Pts',(87.5419104595419,54.0923744890811,13.2463168583588));
#71659=CARTESIAN_POINT('Ctrl Pts',(87.5578593301287,54.0941433137765,13.2525312891203));
#71660=CARTESIAN_POINT('Ctrl Pts',(87.5857486242469,54.0971889307359,13.2627538226797));
#71661=CARTESIAN_POINT('Ctrl Pts',(87.5976317664102,54.0984719261204,13.2669101512775));
#71662=CARTESIAN_POINT('Ctrl Pts',(87.6154292872799,54.1003699080812,13.2728396252423));
#71663=CARTESIAN_POINT('Ctrl Pts',(87.6212973935762,54.1009919187595,13.2747472664732));
#71664=CARTESIAN_POINT('Ctrl Pts',(87.6314405749286,54.1020603194275,13.2779631288489));
#71665=CARTESIAN_POINT('Ctrl Pts',(87.6357088691582,54.102507837008,13.2792916188988));
#71666=CARTESIAN_POINT('Ctrl Pts',(87.645748951861,54.1035556761566,13.2823585010867));
#71667=CARTESIAN_POINT('Ctrl Pts',(87.6515262348226,54.1041549256366,13.2840783837553));
#71668=CARTESIAN_POINT('Ctrl Pts',(87.6683613237701,54.105891043989,13.288959933899));
#71669=CARTESIAN_POINT('Ctrl Pts',(87.6794505902244,54.1070220041077,13.2920127590006));
#71670=CARTESIAN_POINT('Ctrl Pts',(87.7728223244483,54.1164519402811,13.3163579178208));
#71671=CARTESIAN_POINT('Ctrl Pts',(87.8570265830251,54.1243628567864,13.3294958211391));
#71672=CARTESIAN_POINT('Ctrl Pts',(88.0172320519737,54.1393950326146,13.3382219947221));
#71673=CARTESIAN_POINT('Ctrl Pts',(88.0927404322202,54.1464753687877,13.3356075382403));
#71674=CARTESIAN_POINT('Ctrl Pts',(88.185228383494,54.1554897126628,13.3241181799552));
#71675=CARTESIAN_POINT('Ctrl Pts',(88.2028446655056,54.1572216152083,13.3215526408394));
#71676=CARTESIAN_POINT('Ctrl Pts',(88.2303535972828,54.159953445597,13.3169539712056));
#71677=CARTESIAN_POINT('Ctrl Pts',(88.240286444847,54.1609454693887,13.3151715456174));
#71678=CARTESIAN_POINT('Ctrl Pts',(88.2588516753012,54.1628109023192,13.3116111799338));
#71679=CARTESIAN_POINT('Ctrl Pts',(88.2674889089172,54.1636833678406,13.3098613645371));
#71680=CARTESIAN_POINT('Ctrl Pts',(88.286885439905,54.1656535159112,13.3057212156918));
#71681=CARTESIAN_POINT('Ctrl Pts',(88.2976330668623,54.1667527446516,13.3032804588634));
#71682=CARTESIAN_POINT('Ctrl Pts',(88.3253383064679,54.1696068989774,13.2966083343203));
#71683=CARTESIAN_POINT('Ctrl Pts',(88.342242070599,54.1713683864569,13.2921664064197));
#71684=CARTESIAN_POINT('Ctrl Pts',(88.4258372616374,54.1801851679883,13.2683448435993));
#71685=CARTESIAN_POINT('Ctrl Pts',(88.4909387049016,54.1873983060972,13.2438701369153));
#71686=CARTESIAN_POINT('Ctrl Pts',(88.611610003777,54.2014292398099,13.1868345685225));
#71687=CARTESIAN_POINT('Ctrl Pts',(88.6673656328176,54.2082135193037,13.1551221611906));
#71688=CARTESIAN_POINT('Ctrl Pts',(88.7329627406893,54.2164613650735,13.1109382157457));
#71689=CARTESIAN_POINT('Ctrl Pts',(88.7452839299954,54.218022698036,13.1023171489562));
#71690=CARTESIAN_POINT('Ctrl Pts',(88.7718578539834,54.2214129576133,13.0830115454234));
#71691=CARTESIAN_POINT('Ctrl Pts',(88.7860454957718,54.2232378451739,13.0722413974713));
#71692=CARTESIAN_POINT('Ctrl Pts',(88.805537979194,54.2257614811753,13.0567872076999));
#71693=CARTESIAN_POINT('Ctrl Pts',(88.8110363952888,54.2264752206026,13.0523527087603));
#71694=CARTESIAN_POINT('Ctrl Pts',(88.8203922634826,54.2276925472771,13.0446774435839));
#71695=CARTESIAN_POINT('Ctrl Pts',(88.8242678630225,54.2281976609557,13.0414592572267));
#71696=CARTESIAN_POINT('Ctrl Pts',(88.8324458507645,54.2292652046441,13.0345858663922));
#71697=CARTESIAN_POINT('Ctrl Pts',(88.8367431547146,54.2298272120113,13.0309249262644));
#71698=CARTESIAN_POINT('Ctrl Pts',(88.8485926096838,54.231380306168,13.0206930530893));
#71699=CARTESIAN_POINT('Ctrl Pts',(88.8560919817911,54.2323671237043,13.0140610585623));
#71700=CARTESIAN_POINT('Ctrl Pts',(88.9096270001363,54.2394471597219,12.9655777873724));
#71701=CARTESIAN_POINT('Ctrl Pts',(88.9526197939588,54.2453270079938,12.9204740678232));
#71702=CARTESIAN_POINT('Ctrl Pts',(89.0228343171692,54.2557114919477,12.8350437681715));
#71703=CARTESIAN_POINT('Ctrl Pts',(89.0513718490613,54.2602210338976,12.7959749153529));
#71704=CARTESIAN_POINT('Ctrl Pts',(89.0984998871026,54.2683917568101,12.7230575812023));
#71705=CARTESIAN_POINT('Ctrl Pts',(89.1179057383543,54.2720335301538,12.6898107771316));
#71706=CARTESIAN_POINT('Ctrl Pts',(89.1481839480766,54.2782831438371,12.6320628993527));
#71707=CARTESIAN_POINT('Ctrl Pts',(89.1598450576781,54.2808654590492,12.608004921635));
#71708=CARTESIAN_POINT('Ctrl Pts',(89.1755280676174,54.2846205137263,12.5728654024179));
#71709=CARTESIAN_POINT('Ctrl Pts',(89.180169063428,54.2857722665396,12.5620663614418));
#71710=CARTESIAN_POINT('Ctrl Pts',(89.1880575489933,54.2878045607757,12.542984949286));
#71711=CARTESIAN_POINT('Ctrl Pts',(89.1913692147343,54.2886828784394,12.5347297966354));
#71712=CARTESIAN_POINT('Ctrl Pts',(89.19810400506,54.2905234442968,12.5174175688706));
#71713=CARTESIAN_POINT('Ctrl Pts',(89.201510790377,54.2914861738261,12.5083548180015));
#71714=CARTESIAN_POINT('Ctrl Pts',(89.2102187977816,54.2940337345027,12.4843602808558));
#71715=CARTESIAN_POINT('Ctrl Pts',(89.2153445605503,54.2956242180375,12.4693672899858));
#71716=CARTESIAN_POINT('Ctrl Pts',(89.2418364409257,54.3043735642727,12.3868665002708));
#71717=CARTESIAN_POINT('Ctrl Pts',(89.2578037375673,54.3117025925848,12.3177732913356));
#71718=CARTESIAN_POINT('Ctrl Pts',(89.2762633668814,54.3252455634622,12.1900940851957));
#71719=CARTESIAN_POINT('Ctrl Pts',(89.2806219968887,54.3314088549626,12.1319594085346));
#71720=CARTESIAN_POINT('Ctrl Pts',(89.2811379697643,54.3402940178449,12.0472015834006));
#71721=CARTESIAN_POINT('Ctrl Pts',(89.2804681481531,54.3430600981869,12.0206711824044));
#71722=CARTESIAN_POINT('Ctrl Pts',(89.2779882561083,54.3475837970607,11.9768897239188));
#71723=CARTESIAN_POINT('Ctrl Pts',(89.2766553304923,54.3493574972562,11.9596206247205));
#71724=CARTESIAN_POINT('Ctrl Pts',(89.2742892334432,54.3518231016048,11.9354276097054));
#71725=CARTESIAN_POINT('Ctrl Pts',(89.2735515921043,54.3525291317395,11.9284779217565));
#71726=CARTESIAN_POINT('Ctrl Pts',(89.2721848463212,54.3537376210803,11.9165408217073));
#71727=CARTESIAN_POINT('Ctrl Pts',(89.2715834478049,54.3542415475622,11.9115505312625));
#71728=CARTESIAN_POINT('Ctrl Pts',(89.2702391389431,54.3553114882047,11.9009270749086));
#71729=CARTESIAN_POINT('Ctrl Pts',(89.2694880371334,54.3558770454214,11.895295153289));
#71730=CARTESIAN_POINT('Ctrl Pts',(89.267322496146,54.3574240559171,11.8798492725788));
#71731=CARTESIAN_POINT('Ctrl Pts',(89.2658308382263,54.358401389945,11.8700461854474));
#71732=CARTESIAN_POINT('Ctrl Pts',(89.2540512127098,54.3655289610195,11.7982925755796));
#71733=CARTESIAN_POINT('Ctrl Pts',(89.2392936034383,54.3714616685136,11.7371511551096));
#71734=CARTESIAN_POINT('Ctrl Pts',(89.2046897822339,54.3820784468765,11.629502809415));
#71735=CARTESIAN_POINT('Ctrl Pts',(89.1864861846156,54.3867649475019,11.5826189477322));
#71736=CARTESIAN_POINT('Ctrl Pts',(89.1501395232306,54.3949826696573,11.5033010402599));
#71737=CARTESIAN_POINT('Ctrl Pts',(89.1332648476761,54.3984880830722,11.4703573622825));
#71738=CARTESIAN_POINT('Ctrl Pts',(89.1088639433914,54.4032222577977,11.427448732369));
#71739=CARTESIAN_POINT('Ctrl Pts',(89.1025937278335,54.4044128434394,11.4167881158779));
#71740=CARTESIAN_POINT('Ctrl Pts',(89.0867299602863,54.4073650364963,11.3906962371979));
#71741=CARTESIAN_POINT('Ctrl Pts',(89.0769593875125,54.4091321316522,11.3753766406835));
#71742=CARTESIAN_POINT('Ctrl Pts',(89.0612142031055,54.4119068604515,11.3518196977023));
#71743=CARTESIAN_POINT('Ctrl Pts',(89.0554631582905,54.412906165915,11.3434350737097));
#71744=CARTESIAN_POINT('Ctrl Pts',(89.0445448853187,54.414778064243,11.3279197180957));
#71745=CARTESIAN_POINT('Ctrl Pts',(89.0394029138504,54.415649652086,11.3207718675617));
#71746=CARTESIAN_POINT('Ctrl Pts',(89.0277207864666,54.4176082869813,11.3048837136517));
#71747=CARTESIAN_POINT('Ctrl Pts',(89.0211415235751,54.4186968009592,11.2961732388358));
#71748=CARTESIAN_POINT('Ctrl Pts',(89.0039609977495,54.421503398391,11.274026929334));
#71749=CARTESIAN_POINT('Ctrl Pts',(88.9931993615528,54.4232276788463,11.2607191615827));
#71750=CARTESIAN_POINT('Ctrl Pts',(88.9246385638887,54.4340146355097,11.1793565966288));
#71751=CARTESIAN_POINT('Ctrl Pts',(88.8600784429745,54.4433521928657,11.1173534650959));
#71752=CARTESIAN_POINT('Ctrl Pts',(88.7504133965323,54.4579864547707,11.0322570435867));
#71753=CARTESIAN_POINT('Ctrl Pts',(88.7095071795635,54.4632161236954,11.0041878525694));
#71754=CARTESIAN_POINT('Ctrl Pts',(88.6520138762113,54.4701989999536,10.9695009808637));
#71755=CARTESIAN_POINT('Ctrl Pts',(88.636777377736,54.4720164575826,10.9607345787409));
#71756=CARTESIAN_POINT('Ctrl Pts',(88.6101020486744,54.4751365349092,10.9461153524475));
#71757=CARTESIAN_POINT('Ctrl Pts',(88.5987476183028,54.476445747223,10.940114716542));
#71758=CARTESIAN_POINT('Ctrl Pts',(88.5817618113023,54.4783746130096,10.9314650174533));
#71759=CARTESIAN_POINT('Ctrl Pts',(88.5761994081254,54.4790016146174,10.9286837260942));
#71760=CARTESIAN_POINT('Ctrl Pts',(88.5661628659973,54.4801243441433,10.9237571154769));
#71761=CARTESIAN_POINT('Ctrl Pts',(88.5616963848108,54.4806209240297,10.9215970508617));
#71762=CARTESIAN_POINT('Ctrl Pts',(88.5515941464856,54.4817372519929,10.9167842840366));
#71763=CARTESIAN_POINT('Ctrl Pts',(88.5459513877859,54.482356073601,10.9141467924438));
#71764=CARTESIAN_POINT('Ctrl Pts',(88.5285702088604,54.4842485033881,10.9061779090582));
#71765=CARTESIAN_POINT('Ctrl Pts',(88.516769221134,54.4855143155939,10.9009833710567));
#71766=CARTESIAN_POINT('Ctrl Pts',(88.4493852184585,54.4926468783066,10.8725394146499));
#71767=CARTESIAN_POINT('Ctrl Pts',(88.3922729607955,54.4983296620278,10.8530847994365));
#71768=CARTESIAN_POINT('Ctrl Pts',(88.2389483893888,54.5132076613164,10.8127657149742));
#71769=CARTESIAN_POINT('Ctrl Pts',(88.1413461511993,54.5223294742203,10.7988919380768));
#71770=CARTESIAN_POINT('Ctrl Pts',(88.0253755463014,54.5335505100894,10.7959572057265));
#71771=CARTESIAN_POINT('Ctrl Pts',(88.0076165950491,54.5352782998689,10.7958803859647));
#71772=CARTESIAN_POINT('Ctrl Pts',(87.979781669207,54.5380051150081,10.7963437177765));
#71773=CARTESIAN_POINT('Ctrl Pts',(87.9697031728523,54.5389962852452,10.7966315677761));
#71774=CARTESIAN_POINT('Ctrl Pts',(87.9508229866988,54.540860973131,10.7973958815655));
#71775=CARTESIAN_POINT('Ctrl Pts',(87.9420206846636,54.5417335544161,10.7978440449414));
#71776=CARTESIAN_POINT('Ctrl Pts',(87.9222106291433,54.5437051153804,10.7990595122792));
#71777=CARTESIAN_POINT('Ctrl Pts',(87.9112069527115,54.5448056509134,10.7998787262813));
#71778=CARTESIAN_POINT('Ctrl Pts',(87.8827611864052,54.5476656242003,10.802369592879));
#71779=CARTESIAN_POINT('Ctrl Pts',(87.8653412464594,54.5494316691465,10.8042589615149));
#71780=CARTESIAN_POINT('Ctrl Pts',(87.7756934509989,54.5586012203498,10.8158632782155));
#71781=CARTESIAN_POINT('Ctrl Pts',(87.7043752054558,54.5661800643612,10.8314199710698));
#71782=CARTESIAN_POINT('Ctrl Pts',(87.5762308265137,54.5802955222117,10.871162843861));
#71783=CARTESIAN_POINT('Ctrl Pts',(87.5190543661515,54.586786710843,10.8935452778004));
#71784=CARTESIAN_POINT('Ctrl Pts',(87.4459356331277,54.5952329774468,10.9284629505517));
#71785=CARTESIAN_POINT('Ctrl Pts',(87.4283530001038,54.5972752479509,10.9373676994321));
#71786=CARTESIAN_POINT('Ctrl Pts',(87.3986626946154,54.6007360908112,10.9532833038118));
#71787=CARTESIAN_POINT('Ctrl Pts',(87.3864509019732,54.6021631879937,10.9600913673934));
#71788=CARTESIAN_POINT('Ctrl Pts',(87.3687893437143,54.6042301136872,10.9703235792519));
#71789=CARTESIAN_POINT('Ctrl Pts',(87.3632498850711,54.6048788254373,10.973589298295));
#71790=CARTESIAN_POINT('Ctrl Pts',(87.3535147989339,54.6060193467266,10.9794285890256));
#71791=CARTESIAN_POINT('Ctrl Pts',(87.3493090530997,54.6065122107802,10.9819846332971));
#71792=CARTESIAN_POINT('Ctrl Pts',(87.3399956660237,54.6076039313844,10.9877192527519));
#71793=CARTESIAN_POINT('Ctrl Pts',(87.3348956173438,54.6082020059995,10.9909097455034));
#71794=CARTESIAN_POINT('Ctrl Pts',(87.3201599119126,54.6099313795194,11.0002744580347));
#71795=CARTESIAN_POINT('Ctrl Pts',(87.3105843686005,54.6110568386429,11.0065430943592));
#71796=CARTESIAN_POINT('Ctrl Pts',(87.2302069682482,54.6205309982767,11.0607284363416));
#71797=CARTESIAN_POINT('Ctrl Pts',(87.1643108997441,54.6284864121256,11.1155620438226));
#71798=CARTESIAN_POINT('Ctrl Pts',(87.0676533366749,54.6414183348221,11.2140886685929));
#71799=CARTESIAN_POINT('Ctrl Pts',(87.0332521205014,54.6463437503981,11.2538028991818));
#71800=CARTESIAN_POINT('Ctrl Pts',(86.9814839304115,54.6544823065815,11.3216376320076));
#71801=CARTESIAN_POINT('Ctrl Pts',(86.9625813372398,54.657642476021,11.3485067503935));
#71802=CARTESIAN_POINT('Ctrl Pts',(86.937860065441,54.6620758210487,11.3867127256944));
#71803=CARTESIAN_POINT('Ctrl Pts',(86.9311371766234,54.6633155937145,11.3974517408704));
#71804=CARTESIAN_POINT('Ctrl Pts',(86.9198934952538,54.6654503273698,11.4160243397901));
#71805=CARTESIAN_POINT('Ctrl Pts',(86.9152935351916,54.6663423429489,11.4238091436931));
#71806=CARTESIAN_POINT('Ctrl Pts',(86.9061030147647,54.6681637309044,11.4397490737935));
#71807=CARTESIAN_POINT('Ctrl Pts',(86.9015186985972,54.6690932614997,11.4479071263924));
#71808=CARTESIAN_POINT('Ctrl Pts',(86.8901617304365,54.6714507760458,11.4686509938695));
#71809=CARTESIAN_POINT('Ctrl Pts',(86.8835108308186,54.6728829474553,11.4813014519466));
#71810=CARTESIAN_POINT('Ctrl Pts',(86.8573580728529,54.6787335095887,11.5331518263962));
#71811=CARTESIAN_POINT('Ctrl Pts',(86.8396787641963,54.6832126176885,11.5732299737906));
#71812=CARTESIAN_POINT('Ctrl Pts',(86.7909831271674,54.6973977977161,11.7011366842082));
#71813=CARTESIAN_POINT('Ctrl Pts',(86.767529211037,54.7072893198655,11.7915124924679));
#71814=CARTESIAN_POINT('Ctrl Pts',(86.749121452133,54.720699356509,11.9183681160973));
#71815=CARTESIAN_POINT('Ctrl Pts',(86.7455219099128,54.7243414510373,11.9533122849575));
#71816=CARTESIAN_POINT('Ctrl Pts',(86.7428319437241,54.7288247137774,11.997234203389));
#71817=CARTESIAN_POINT('Ctrl Pts',(86.7423818345657,54.7297257640732,12.0061090960341));
#71818=CARTESIAN_POINT('Ctrl Pts',(86.7418079148009,54.7311667993958,12.0203860522273));
#71819=CARTESIAN_POINT('Ctrl Pts',(86.7416253688206,54.731709810395,12.0257851877751));
#71820=CARTESIAN_POINT('Ctrl Pts',(86.7413377252564,54.7327607548558,12.0362742121381));
#71821=CARTESIAN_POINT('Ctrl Pts',(86.7412287726824,54.7332688610319,12.041363705589));
#71822=CARTESIAN_POINT('Ctrl Pts',(86.7410518012606,54.7344128290737,12.0528610200948));
#71823=CARTESIAN_POINT('Ctrl Pts',(86.7410016692145,54.7350477107754,12.0592689933539));
#71824=CARTESIAN_POINT('Ctrl Pts',(86.7409954393869,54.737467659951,12.0837882439003));
#71825=CARTESIAN_POINT('Ctrl Pts',(86.7413782462323,54.7392356099123,12.1018988784228));
#71826=CARTESIAN_POINT('Ctrl Pts',(86.7428033295998,54.7424795095499,12.1353864192012));
#71827=CARTESIAN_POINT('Ctrl Pts',(86.7437382177276,54.7439592720158,12.1507638011839));
#71828=CARTESIAN_POINT('Ctrl Pts',(86.7502296530399,54.7518249398589,12.2328488985241));
#71829=CARTESIAN_POINT('Ctrl Pts',(86.7607741707956,54.7580558745846,12.2990610896158));
#71830=CARTESIAN_POINT('Ctrl Pts',(86.7933757143798,54.7710769329224,12.4340550311957));
#71831=CARTESIAN_POINT('Ctrl Pts',(86.816166671103,54.7778528761339,12.5023988119153));
#71832=CARTESIAN_POINT('Ctrl Pts',(86.8509282599534,54.7863711478374,12.5830959713173));
#71833=CARTESIAN_POINT('Ctrl Pts',(86.857517285119,54.7879266373817,12.5976316934127));
#71834=CARTESIAN_POINT('Ctrl Pts',(86.8685512176222,54.7904431456659,12.6208017543951));
#71835=CARTESIAN_POINT('Ctrl Pts',(86.8728245161467,54.7913982411413,12.6295164256622));
#71836=CARTESIAN_POINT('Ctrl Pts',(86.8812012190041,54.7932345964088,12.6461152471569));
#71837=CARTESIAN_POINT('Ctrl Pts',(86.8852883481446,54.7941152418322,12.6540070171199));
#71838=CARTESIAN_POINT('Ctrl Pts',(86.8949476552359,54.7961622143243,12.6721881523995));
#71839=CARTESIAN_POINT('Ctrl Pts',(86.9005797756989,54.7973306010337,12.6824444940606));
#71840=CARTESIAN_POINT('Ctrl Pts',(86.9193827947974,54.8011528229406,12.7155916481902));
#71841=CARTESIAN_POINT('Ctrl Pts',(86.9331250331379,54.8038267187554,12.7381478433711));
#71842=CARTESIAN_POINT('Ctrl Pts',(86.9682326824704,54.8103894049703,12.7919246111992));
#71843=CARTESIAN_POINT('Ctrl Pts',(86.9903080281129,54.8143009102124,12.8226488418689));
#71844=CARTESIAN_POINT('Ctrl Pts',(87.0440791960149,54.8233651467671,12.8908445856383));
#71845=CARTESIAN_POINT('Ctrl Pts',(87.0766427135866,54.8285353338819,12.9275569074693));
#71846=CARTESIAN_POINT('Ctrl Pts',(87.1335701734923,54.8370389051246,12.984704319067));
#71847=CARTESIAN_POINT('Ctrl Pts',(87.1567195825001,54.8403688370676,13.0062683871806));
#71848=CARTESIAN_POINT('Ctrl Pts',(87.1806429093249,54.843673293217,13.0269407380092));
#71849=CARTESIAN_POINT('',(86.7410003619504,54.90489047952,12.0650595732259));
#71850=CARTESIAN_POINT('Ctrl Pts',(87.180642810782,55.0125145086225,13.0269406528573));
#71851=CARTESIAN_POINT('Ctrl Pts',(87.1698106884351,55.0110058097381,13.0175805215751));
#71852=CARTESIAN_POINT('Ctrl Pts',(87.1591359293049,55.0094958279517,13.0080364534887));
#71853=CARTESIAN_POINT('Ctrl Pts',(87.102604711212,55.0013776670237,12.9557458148336));
#71854=CARTESIAN_POINT('Ctrl Pts',(87.0597937052197,54.9947847952294,12.9098238037927));
#71855=CARTESIAN_POINT('Ctrl Pts',(87.0142711780043,54.9873587895733,12.8531036237434));
#71856=CARTESIAN_POINT('Ctrl Pts',(87.0080900050372,54.9863406024284,12.8452124382936));
#71857=CARTESIAN_POINT('Ctrl Pts',(86.9985732413489,54.9847582712658,12.8327619884891));
#71858=CARTESIAN_POINT('Ctrl Pts',(86.9951737557381,54.9841900183706,12.828252539949));
#71859=CARTESIAN_POINT('Ctrl Pts',(86.9888000763443,54.9831190391899,12.8196794220616));
#71860=CARTESIAN_POINT('Ctrl Pts',(86.985819930942,54.9826159504102,12.8156206928221));
#71861=CARTESIAN_POINT('Ctrl Pts',(86.9787223153728,54.9814119038054,12.8058327872665));
#71862=CARTESIAN_POINT('Ctrl Pts',(86.9746282856707,54.9807125299567,12.8000868133862));
#71863=CARTESIAN_POINT('Ctrl Pts',(86.9612526646347,54.9784101933249,12.7809791584609));
#71864=CARTESIAN_POINT('Ctrl Pts',(86.9521793093724,54.9768200701466,12.7674723798383));
#71865=CARTESIAN_POINT('Ctrl Pts',(86.890023481675,54.9656912590456,12.670990567327));
#71866=CARTESIAN_POINT('Ctrl Pts',(86.8464848539477,54.9566150649677,12.5822489567285));
#71867=CARTESIAN_POINT('Ctrl Pts',(86.7940489582253,54.9418198833297,12.4339455362181));
#71868=CARTESIAN_POINT('Ctrl Pts',(86.7783309794268,54.9362472325153,12.3772539443391));
#71869=CARTESIAN_POINT('Ctrl Pts',(86.7635088573466,54.9290486303741,12.3045467181843));
#71870=CARTESIAN_POINT('Ctrl Pts',(86.7606994424445,54.9275419707352,12.2893543233547));
#71871=CARTESIAN_POINT('Ctrl Pts',(86.7565952360157,54.9250851736239,12.2646474290017));
#71872=CARTESIAN_POINT('Ctrl Pts',(86.7551299125376,54.924140453901,12.255162426993));
#71873=CARTESIAN_POINT('Ctrl Pts',(86.7525739206633,54.9223554465787,12.2372762686541));
#71874=CARTESIAN_POINT('Ctrl Pts',(86.7514595327371,54.9215159572235,12.2288789729665));
#71875=CARTESIAN_POINT('Ctrl Pts',(86.7493741882523,54.9198113628102,12.2118614279721));
#71876=CARTESIAN_POINT('Ctrl Pts',(86.748407387461,54.9189461736336,12.2032411388734));
#71877=CARTESIAN_POINT('Ctrl Pts',(86.7463769813185,54.9169398262956,12.1832946222166));
#71878=CARTESIAN_POINT('Ctrl Pts',(86.7453771269305,54.9157967451473,12.1719628677395));
#71879=CARTESIAN_POINT('Ctrl Pts',(86.7421536702233,54.9114308722007,12.1288173779079));
#71880=CARTESIAN_POINT('Ctrl Pts',(86.7409767013054,54.9081768245373,12.0969410458204));
#71881=CARTESIAN_POINT('Ctrl Pts',(86.741000349337,54.904890341317,12.0650580255078));
#71882=CARTESIAN_POINT('Ctrl Pts',(86.7410003481916,54.9048905006295,12.0650595710399));
#71883=CARTESIAN_POINT('Ctrl Pts',(86.7410934640266,54.8919284719138,11.9393115527867));
#71884=CARTESIAN_POINT('Ctrl Pts',(86.7598596542112,54.8784526712305,11.8142941249287));
#71885=CARTESIAN_POINT('Ctrl Pts',(86.8000461907814,54.8643085503561,11.6830861840034));
#71886=CARTESIAN_POINT('Ctrl Pts',(86.8035615683117,54.8631294965894,11.672141418893));
#71887=CARTESIAN_POINT('Ctrl Pts',(86.8094072797689,54.8612592606878,11.65475577855));
#71888=CARTESIAN_POINT('Ctrl Pts',(86.8116418267275,54.8605636417918,11.648283763229));
#71889=CARTESIAN_POINT('Ctrl Pts',(86.816005498673,54.8592415412436,11.6359688302902));
#71890=CARTESIAN_POINT('Ctrl Pts',(86.8181254029523,54.8586145936132,11.6301228764736));
#71891=CARTESIAN_POINT('Ctrl Pts',(86.8220134337675,54.8574920245916,11.619641904184));
#71892=CARTESIAN_POINT('Ctrl Pts',(86.8237658511113,54.8569955509263,11.6150014597488));
#71893=CARTESIAN_POINT('Ctrl Pts',(86.8277792241609,54.8558795571868,11.6045594730795));
#71894=CARTESIAN_POINT('Ctrl Pts',(86.8300557092215,54.8552609624051,11.598764136273));
#71895=CARTESIAN_POINT('Ctrl Pts',(86.8371734589993,54.8533695505927,11.581028612118));
#71896=CARTESIAN_POINT('Ctrl Pts',(86.8421541185608,54.8521045189239,11.5691445403283));
#71897=CARTESIAN_POINT('Ctrl Pts',(86.8711897508726,54.845034940732,11.5027187163825));
#71898=CARTESIAN_POINT('Ctrl Pts',(86.898884545489,54.8394103086718,11.4498385398354));
#71899=CARTESIAN_POINT('Ctrl Pts',(86.957438505406,54.828944563975,11.3549450153583));
#71900=CARTESIAN_POINT('Ctrl Pts',(86.9873580027247,54.8241067814038,11.3125095054062));
#71901=CARTESIAN_POINT('Ctrl Pts',(87.0417871436568,54.8158976085815,11.2445594063387));
#71902=CARTESIAN_POINT('Ctrl Pts',(87.0649160702189,54.8125593532128,11.2180241628412));
#71903=CARTESIAN_POINT('Ctrl Pts',(87.1010909933119,54.807510928794,11.1798460780079));
#71904=CARTESIAN_POINT('Ctrl Pts',(87.1133250067429,54.8058307642166,11.1674552232407));
#71905=CARTESIAN_POINT('Ctrl Pts',(87.1361804189124,54.8027357380138,11.1452395062453));
#71906=CARTESIAN_POINT('Ctrl Pts',(87.1467225318601,54.8013243501708,11.1353370087123));
#71907=CARTESIAN_POINT('Ctrl Pts',(87.1577545313864,54.7998624769916,11.1253234555548));
#71908=CARTESIAN_POINT('Ctrl Pts',(87.1580782715222,54.7998195907075,11.1250299069215));
#71909=CARTESIAN_POINT('Ctrl Pts',(87.1587262028293,54.7997337847073,11.1244430097918));
#71910=CARTESIAN_POINT('Ctrl Pts',(87.1590503940878,54.7996908649918,11.1241496614968));
#71911=CARTESIAN_POINT('Ctrl Pts',(87.1597029878005,54.7996044944453,11.1235597669833));
#71912=CARTESIAN_POINT('Ctrl Pts',(87.1600313938301,54.7995610434592,11.1232632249135));
#71913=CARTESIAN_POINT('Ctrl Pts',(87.1606965707766,54.79947306186,11.1226632182742));
#71914=CARTESIAN_POINT('Ctrl Pts',(87.1610333493052,54.7994285309049,11.1223597622975));
#71915=CARTESIAN_POINT('Ctrl Pts',(87.1678875392284,54.7985225122609,11.1161904064832));
#71916=CARTESIAN_POINT('Ctrl Pts',(87.1744651567851,54.7976582896785,11.1103921662719));
#71917=CARTESIAN_POINT('Ctrl Pts',(87.1879067299265,54.7959022483479,11.0987884000115));
#71918=CARTESIAN_POINT('Ctrl Pts',(87.1947733284507,54.7950103352439,11.0929867316224));
#71919=CARTESIAN_POINT('Ctrl Pts',(87.2100650496211,54.7930348550631,11.0803423503396));
#71920=CARTESIAN_POINT('Ctrl Pts',(87.2185173591802,54.7919499913962,11.0735338583841));
#71921=CARTESIAN_POINT('Ctrl Pts',(87.2481870943528,54.7881649774426,11.0502550012664));
#71922=CARTESIAN_POINT('Ctrl Pts',(87.2698371283267,54.7854432180522,11.034351439843));
#71923=CARTESIAN_POINT('Ctrl Pts',(87.3686244663003,54.7731854466729,10.9664996947126));
#71924=CARTESIAN_POINT('Ctrl Pts',(87.4508128749438,54.763381774003,10.9224393986443));
#71925=CARTESIAN_POINT('Ctrl Pts',(87.5721714171492,54.749603050082,10.8736231944838));
#71926=CARTESIAN_POINT('Ctrl Pts',(87.6079083186902,54.7456284260851,10.8610723900173));
#71927=CARTESIAN_POINT('Ctrl Pts',(87.6652083914254,54.7394248306864,10.8437840851159));
#71928=CARTESIAN_POINT('Ctrl Pts',(87.6864251036473,54.7371635848832,10.8379792689086));
#71929=CARTESIAN_POINT('Ctrl Pts',(87.7151996095432,54.7341530222537,10.8309046820618));
#71930=CARTESIAN_POINT('Ctrl Pts',(87.7226318520593,54.7333804158651,10.8291482961644));
#71931=CARTESIAN_POINT('Ctrl Pts',(87.7350895739684,54.7320942028469,10.8263226929633));
#71932=CARTESIAN_POINT('Ctrl Pts',(87.7401063850147,54.7315786160972,10.825216762339));
#71933=CARTESIAN_POINT('Ctrl Pts',(87.7504317359373,54.7305225095385,10.8230062041882));
#71934=CARTESIAN_POINT('Ctrl Pts',(87.7557408629402,54.7299821877035,10.8219050785012));
#71935=CARTESIAN_POINT('Ctrl Pts',(87.7698617672608,54.7285518422606,10.8190705717059));
#71936=CARTESIAN_POINT('Ctrl Pts',(87.7786854314441,54.7276650517673,10.8173965382823));
#71937=CARTESIAN_POINT('Ctrl Pts',(87.81957034491,54.7235849506805,10.8100882597403));
#71938=CARTESIAN_POINT('Ctrl Pts',(87.8518270409986,54.7204477333111,10.8055936472637));
#71939=CARTESIAN_POINT('Ctrl Pts',(87.9514931432954,54.7108998143063,10.7955947677734));
#71940=CARTESIAN_POINT('Ctrl Pts',(88.0191979091881,54.704612275786,10.7942276895338));
#71941=CARTESIAN_POINT('Ctrl Pts',(88.1514390326683,54.6921835303043,10.802123545547));
#71942=CARTESIAN_POINT('Ctrl Pts',(88.2157824777618,54.686064924414,10.8109426972517));
#71943=CARTESIAN_POINT('Ctrl Pts',(88.2965679504061,54.6780710247587,10.8283942569459));
#71944=CARTESIAN_POINT('Ctrl Pts',(88.3138897576757,54.6763387324865,10.8325192545325));
#71945=CARTESIAN_POINT('Ctrl Pts',(88.3408833471298,54.6736065565357,10.8395503245772));
#71946=CARTESIAN_POINT('Ctrl Pts',(88.350617538802,54.672614582483,10.8422100908025));
#71947=CARTESIAN_POINT('Ctrl Pts',(88.3687895050635,54.6707494059505,10.8474088880152));
#71948=CARTESIAN_POINT('Ctrl Pts',(88.377234624666,54.6698771480351,10.8499203077494));
#71949=CARTESIAN_POINT('Ctrl Pts',(88.3961788519711,54.6679076927656,10.8557691896448));
#71950=CARTESIAN_POINT('Ctrl Pts',(88.4066618709041,54.6668089517301,10.8591557571115));
#71951=CARTESIAN_POINT('Ctrl Pts',(88.4336466123747,54.6639565542522,10.8682626131104));
#71952=CARTESIAN_POINT('Ctrl Pts',(88.4500760831121,54.6621963476232,10.8741874633724));
#71953=CARTESIAN_POINT('Ctrl Pts',(88.5354174710193,54.65292354661,10.9069675898494));
#71954=CARTESIAN_POINT('Ctrl Pts',(88.6019939977865,54.6452297135823,10.9394604562044));
#71955=CARTESIAN_POINT('Ctrl Pts',(88.7172631204084,54.6310766496725,11.0087578628638));
#71956=CARTESIAN_POINT('Ctrl Pts',(88.7668756677696,54.624666052473,11.0436394730726));
#71957=CARTESIAN_POINT('Ctrl Pts',(88.8289828577866,54.616312114149,11.0943069292513));
#71958=CARTESIAN_POINT('Ctrl Pts',(88.8438675644932,54.6142830231231,11.1070343507949));
#71959=CARTESIAN_POINT('Ctrl Pts',(88.8688158653228,54.61084206221,11.1293861378105));
#71960=CARTESIAN_POINT('Ctrl Pts',(88.8790261743421,54.6094217857296,11.1388407884696));
#71961=CARTESIAN_POINT('Ctrl Pts',(88.8937161291832,54.6073628928174,11.1528990099708));
#71962=CARTESIAN_POINT('Ctrl Pts',(88.898318983797,54.6067154848059,11.1573712473022));
#71963=CARTESIAN_POINT('Ctrl Pts',(88.9063902915822,54.6055764465913,11.1653333417676));
#71964=CARTESIAN_POINT('Ctrl Pts',(88.9098725923055,54.6050837713722,11.1688086770513));
#71965=CARTESIAN_POINT('Ctrl Pts',(88.9175733017625,54.6039914894095,11.1765838281908));
#71966=CARTESIAN_POINT('Ctrl Pts',(88.9217814276838,54.6033926717779,11.1808935235751));
#71967=CARTESIAN_POINT('Ctrl Pts',(88.9339226836329,54.6016586842055,11.1935061124505));
#71968=CARTESIAN_POINT('Ctrl Pts',(88.9417744173397,54.6005294024667,11.2018872286319));
#71969=CARTESIAN_POINT('Ctrl Pts',(89.0068712655435,54.5910865180717,11.2732901338863));
#71970=CARTESIAN_POINT('Ctrl Pts',(89.0577709229527,54.5831625132236,11.3418279581042));
#71971=CARTESIAN_POINT('Ctrl Pts',(89.1284424505854,54.5702460281034,11.4601961620565));
#71972=CARTESIAN_POINT('Ctrl Pts',(89.1526079268061,54.5653032155488,11.5070666754943));
#71973=CARTESIAN_POINT('Ctrl Pts',(89.187028315973,54.557139897787,11.585436898572));
#71974=CARTESIAN_POINT('Ctrl Pts',(89.1990868389286,54.5539728128097,11.6160747414578));
#71975=CARTESIAN_POINT('Ctrl Pts',(89.2141222022973,54.5495315761257,11.6591121774551));
#71976=CARTESIAN_POINT('Ctrl Pts',(89.2181238957757,54.5482909954441,11.6711422966348));
#71977=CARTESIAN_POINT('Ctrl Pts',(89.2246699800244,54.5461554480458,11.6918517079031));
#71978=CARTESIAN_POINT('Ctrl Pts',(89.2273030520984,54.5452634344613,11.7005022028386));
#71979=CARTESIAN_POINT('Ctrl Pts',(89.2321612988465,54.5435517554946,11.7170972335822));
#71980=CARTESIAN_POINT('Ctrl Pts',(89.2344018803436,54.5427326399951,11.7250368213773));
#71981=CARTESIAN_POINT('Ctrl Pts',(89.2394974019756,54.5407970350535,11.7437901076697));
#71982=CARTESIAN_POINT('Ctrl Pts',(89.2422870999899,54.5396785065264,11.7546205880538));
#71983=CARTESIAN_POINT('Ctrl Pts',(89.2517401826652,54.535666199873,11.7934356705659));
#71984=CARTESIAN_POINT('Ctrl Pts',(89.2575947509803,54.5327473167474,11.8216054367845));
#71985=CARTESIAN_POINT('Ctrl Pts',(89.2779626443844,54.5204791434414,11.9395864339998));
#71986=CARTESIAN_POINT('Ctrl Pts',(89.2837593992223,54.5108837227244,12.0306143038151));
#71987=CARTESIAN_POINT('Ctrl Pts',(89.2775894085617,54.4960029016111,12.1717695457315));
#71988=CARTESIAN_POINT('Ctrl Pts',(89.2723996171966,54.4907233301621,12.2219112243757));
#71989=CARTESIAN_POINT('Ctrl Pts',(89.2622305298388,54.4842847338275,12.2838918446784));
#71990=CARTESIAN_POINT('Ctrl Pts',(89.2600364952113,54.4830172366291,12.2961359821706));
#71991=CARTESIAN_POINT('Ctrl Pts',(89.2564910524735,54.481137620085,12.3143741967708));
#71992=CARTESIAN_POINT('Ctrl Pts',(89.2552755897611,54.4805186646489,12.3203933291233));
#71993=CARTESIAN_POINT('Ctrl Pts',(89.2531003768096,54.4794535699923,12.3307765386684));
#71994=CARTESIAN_POINT('Ctrl Pts',(89.2521612141287,54.4790063256276,12.3351445791839));
#71995=CARTESIAN_POINT('Ctrl Pts',(89.2498955399249,54.4779563316691,12.3454180938682));
#71996=CARTESIAN_POINT('Ctrl Pts',(89.248549837746,54.4773546749522,12.3513191803497));
#71997=CARTESIAN_POINT('Ctrl Pts',(89.2444972534445,54.4756043450149,12.3685220216944));
#71998=CARTESIAN_POINT('Ctrl Pts',(89.2416772565029,54.4744617284442,12.3797970254614));
#71999=CARTESIAN_POINT('Ctrl Pts',(89.2172317356977,54.4651293178242,12.4721319029169));
#72000=CARTESIAN_POINT('Ctrl Pts',(89.1877731304621,54.4573162747194,12.5509215426156));
#72001=CARTESIAN_POINT('Ctrl Pts',(89.1272113055187,54.4444544097837,12.6741278069826));
#72002=CARTESIAN_POINT('Ctrl Pts',(89.1006806900123,54.4394504502596,12.7204786401932));
#72003=CARTESIAN_POINT('Ctrl Pts',(89.0589178918515,54.4322155310729,12.7838269091795));
#72004=CARTESIAN_POINT('Ctrl Pts',(89.0460225595952,54.4300546750574,12.802298548022));
#72005=CARTESIAN_POINT('Ctrl Pts',(89.0219367227628,54.4261339902829,12.8349160033659));
#72006=CARTESIAN_POINT('Ctrl Pts',(89.0109229389182,54.4243807461337,12.8491851099382));
#72007=CARTESIAN_POINT('Ctrl Pts',(88.9932470705487,54.421623027223,12.8711046122149));
#72008=CARTESIAN_POINT('Ctrl Pts',(88.9867902432503,54.4206267134841,12.8789182804297));
#72009=CARTESIAN_POINT('Ctrl Pts',(88.974550504583,54.4187577041039,12.8933741421176));
#72010=CARTESIAN_POINT('Ctrl Pts',(88.9687906385924,54.417885989702,12.9000351483223));
#72011=CARTESIAN_POINT('Ctrl Pts',(88.9557122213166,54.4159234963693,12.9148455603578));
#72012=CARTESIAN_POINT('Ctrl Pts',(88.9483566833082,54.4148312215729,12.9229611399494));
#72013=CARTESIAN_POINT('Ctrl Pts',(88.9291519674401,54.4120075519794,12.9436071780924));
#72014=CARTESIAN_POINT('Ctrl Pts',(88.9171513393755,54.4102698283627,12.9559927357421));
#72015=CARTESIAN_POINT('Ctrl Pts',(88.8436968601303,54.3997841687521,13.0287773962269));
#72016=CARTESIAN_POINT('Ctrl Pts',(88.7764921301597,54.3907823443872,13.0830247520019));
#72017=CARTESIAN_POINT('Ctrl Pts',(88.6610408754983,54.3762572511149,13.1582531509457));
#72018=CARTESIAN_POINT('Ctrl Pts',(88.6160639346775,54.3708013832918,13.1837962122567));
#72019=CARTESIAN_POINT('Ctrl Pts',(88.5534992295892,54.363552929103,13.2144416161539));
#72020=CARTESIAN_POINT('Ctrl Pts',(88.5371777433677,54.3616919650728,13.2220106560987));
#72021=CARTESIAN_POINT('Ctrl Pts',(88.5087332694371,54.3585055580064,13.2344743403046));
#72022=CARTESIAN_POINT('Ctrl Pts',(88.4966856901262,54.3571731644325,13.2395331907957));
#72023=CARTESIAN_POINT('Ctrl Pts',(88.4787524777634,54.3552171244259,13.2467399425524));
#72024=CARTESIAN_POINT('Ctrl Pts',(88.472926195591,54.3545858374817,13.2490314401169));
#72025=CARTESIAN_POINT('Ctrl Pts',(88.4624533947451,54.3534588873235,13.2530612616414));
#72026=CARTESIAN_POINT('Ctrl Pts',(88.4578134106997,54.3529623372208,13.2548155390403));
#72027=CARTESIAN_POINT('Ctrl Pts',(88.4473652911451,54.3518503447489,13.25869593022));
#72028=CARTESIAN_POINT('Ctrl Pts',(88.4415517546531,54.3512357938772,13.2608068637843));
#72029=CARTESIAN_POINT('Ctrl Pts',(88.4237852353928,54.3493696895176,13.267111485281));
#72030=CARTESIAN_POINT('Ctrl Pts',(88.4117841241153,54.3481256235145,13.271169108979));
#72031=CARTESIAN_POINT('Ctrl Pts',(88.3096035819413,54.3376549887867,13.3040214162474));
#72032=CARTESIAN_POINT('Ctrl Pts',(88.2165082314341,54.3288988436078,13.3228351911097));
#72033=CARTESIAN_POINT('Ctrl Pts',(88.0583346645404,54.3139999131475,13.3367343967961));
#72034=CARTESIAN_POINT('Ctrl Pts',(87.9941756024205,54.3079526973779,13.3375035803119));
#72035=CARTESIAN_POINT('Ctrl Pts',(87.9124589523599,54.3000330499152,13.3322966064627));
#72036=CARTESIAN_POINT('Ctrl Pts',(87.894705251123,54.298299672508,13.3307896623789));
#72037=CARTESIAN_POINT('Ctrl Pts',(87.8669531057224,54.2955661733847,13.327844827497));
#72038=CARTESIAN_POINT('Ctrl Pts',(87.8569294897768,54.2945739742299,13.3266601999583));
#72039=CARTESIAN_POINT('Ctrl Pts',(87.8381848255181,54.2927086006077,13.3242180013995));
#72040=CARTESIAN_POINT('Ctrl Pts',(87.8294606070769,54.2918363726147,13.3229888871672));
#72041=CARTESIAN_POINT('Ctrl Pts',(87.8098613366899,54.2898672869698,13.320019348486));
#72042=CARTESIAN_POINT('Ctrl Pts',(87.7989948880798,54.2887688881668,13.3182280547628));
#72043=CARTESIAN_POINT('Ctrl Pts',(87.7709715095677,54.2859180136631,13.313233307976));
#72044=CARTESIAN_POINT('Ctrl Pts',(87.753855569142,54.2841589995986,13.3098172152271));
#72045=CARTESIAN_POINT('Ctrl Pts',(87.6687843221247,54.2753219228958,13.2910073802815));
#72046=CARTESIAN_POINT('Ctrl Pts',(87.6021200901101,54.2680848228393,13.2703952751904));
#72047=CARTESIAN_POINT('Ctrl Pts',(87.4781922404125,54.254044161759,13.2205996898477));
#72048=CARTESIAN_POINT('Ctrl Pts',(87.420772204561,54.247274937073,13.1923286053936));
#72049=CARTESIAN_POINT('Ctrl Pts',(87.3527888283091,54.2390438609256,13.1522244542174));
#72050=CARTESIAN_POINT('Ctrl Pts',(87.33999023972,54.2374845061477,13.1443651804191));
#72051=CARTESIAN_POINT('Ctrl Pts',(87.3123387923966,54.234097917353,13.1267021711953));
#72052=CARTESIAN_POINT('Ctrl Pts',(87.2975457726233,54.2322747226001,13.1168090964369));
#72053=CARTESIAN_POINT('Ctrl Pts',(87.2771794563364,54.2297530917471,13.1025602992714));
#72054=CARTESIAN_POINT('Ctrl Pts',(87.2714282191832,54.2290396927658,13.0984647373534));
#72055=CARTESIAN_POINT('Ctrl Pts',(87.2616335438753,54.2278228412966,13.0913659227947));
#72056=CARTESIAN_POINT('Ctrl Pts',(87.2575733652529,54.2273178644425,13.0883862636069));
#72057=CARTESIAN_POINT('Ctrl Pts',(87.2490001081318,54.2262505054806,13.082015760578));
#72058=CARTESIAN_POINT('Ctrl Pts',(87.2444917672516,54.2256885465556,13.0786188792675));
#72059=CARTESIAN_POINT('Ctrl Pts',(87.2320505764725,54.2241353851996,13.0691141632968));
#72060=CARTESIAN_POINT('Ctrl Pts',(87.2241667767994,54.223148453758,13.0629421903661));
#72061=CARTESIAN_POINT('Ctrl Pts',(87.2042690256248,54.2206480225701,13.046981774004));
#72062=CARTESIAN_POINT('Ctrl Pts',(87.1923625943332,54.2191427597545,13.0370678197031));
#72063=CARTESIAN_POINT('Ctrl Pts',(87.1806428209146,54.2176482202995,13.026940661613));
#72064=CARTESIAN_POINT('Origin',(88.011,66.41344859951,12.066));
#72065=CARTESIAN_POINT('',(87.180642873398,53.2551312395179,13.0269407069644));
#72066=CARTESIAN_POINT('',(87.1806428308131,53.4258009314892,13.0269406701664));
#72067=CARTESIAN_POINT('',(87.1806428354228,66.41344859951,13.0269406741497));
#72068=CARTESIAN_POINT('',(86.7410006142678,53.9404808773293,12.0671672720113));
#72069=CARTESIAN_POINT('Ctrl Pts',(87.180642873398,53.2551312395179,13.0269407069644));
#72070=CARTESIAN_POINT('Ctrl Pts',(87.227200822058,53.2609129875801,13.0671718306847));
#72071=CARTESIAN_POINT('Ctrl Pts',(87.2766258799977,53.2667392828233,13.1039705488038));
#72072=CARTESIAN_POINT('Ctrl Pts',(87.3419097202082,53.2742449419896,13.1455692719022));
#72073=CARTESIAN_POINT('Ctrl Pts',(87.3554449324859,53.2757911838897,13.1538414935601));
#72074=CARTESIAN_POINT('Ctrl Pts',(87.3774884242731,53.2782964046547,13.1667528771713));
#72075=CARTESIAN_POINT('Ctrl Pts',(87.3859014717742,53.2792495575271,13.1715521834217));
#72076=CARTESIAN_POINT('Ctrl Pts',(87.4021431627526,53.2810846073721,13.1805727640856));
#72077=CARTESIAN_POINT('Ctrl Pts',(87.4099629095553,53.281965908476,13.1848089650934));
#72078=CARTESIAN_POINT('Ctrl Pts',(87.4282119803334,53.2840180455739,13.1944485293537));
#72079=CARTESIAN_POINT('Ctrl Pts',(87.438672854058,53.2851909752648,13.1997899159215));
#72080=CARTESIAN_POINT('Ctrl Pts',(87.4731334037261,53.2890451883397,13.2167872697744));
#72081=CARTESIAN_POINT('Ctrl Pts',(87.4974244754101,53.2917470063026,13.2278311941146));
#72082=CARTESIAN_POINT('Ctrl Pts',(87.5574596915302,53.2983959634044,13.2528756537902));
#72083=CARTESIAN_POINT('Ctrl Pts',(87.5935234971836,53.3023666408844,13.2660355517333));
#72084=CARTESIAN_POINT('Ctrl Pts',(87.6763517669119,53.3114324930981,13.2920745537359));
#72085=CARTESIAN_POINT('Ctrl Pts',(87.7233712346569,53.3165424736692,13.3039488656055));
#72086=CARTESIAN_POINT('Ctrl Pts',(87.8321118113701,53.3282161234439,13.3248797660017));
#72087=CARTESIAN_POINT('Ctrl Pts',(87.8940655349541,53.3347654443521,13.3321389991874));
#72088=CARTESIAN_POINT('Ctrl Pts',(87.9663115815308,53.3421488353369,13.3352529899925));
#72089=CARTESIAN_POINT('Ctrl Pts',(87.9763179798554,53.343165726688,13.3355658264261));
#72090=CARTESIAN_POINT('Ctrl Pts',(87.9919715713423,53.3447465717136,13.3358699876128));
#72091=CARTESIAN_POINT('Ctrl Pts',(87.9976164228162,53.3453146211337,13.3359420266138));
#72092=CARTESIAN_POINT('Ctrl Pts',(88.0082991920578,53.3463856058333,13.3360071189668));
#72093=CARTESIAN_POINT('Ctrl Pts',(88.0133366499035,53.3468889008576,13.3360078419431));
#72094=CARTESIAN_POINT('Ctrl Pts',(88.0254374930207,53.3480939855365,13.3359375770154));
#72095=CARTESIAN_POINT('Ctrl Pts',(88.0325005487673,53.3487941850249,13.3358376375378));
#72096=CARTESIAN_POINT('Ctrl Pts',(88.0573668062436,53.3512493231859,13.3352782459652));
#72097=CARTESIAN_POINT('Ctrl Pts',(88.0751621460975,53.3529882897881,13.3345032445289));
#72098=CARTESIAN_POINT('Ctrl Pts',(88.1079409181058,53.3561685364609,13.3323840333867));
#72099=CARTESIAN_POINT('Ctrl Pts',(88.1229274231113,53.3576136917733,13.331147567277));
#72100=CARTESIAN_POINT('Ctrl Pts',(88.2016123289715,53.3651722545157,13.3232463992466));
#72101=CARTESIAN_POINT('Ctrl Pts',(88.2647662196606,53.3711419734209,13.3120360571269));
#72102=CARTESIAN_POINT('Ctrl Pts',(88.3940981054705,53.3836557428268,13.2788322085525));
#72103=CARTESIAN_POINT('Ctrl Pts',(88.4598453548579,53.3901865239372,13.2560679273938));
#72104=CARTESIAN_POINT('Ctrl Pts',(88.539374841443,53.3985779470414,13.2210000080367));
#72105=CARTESIAN_POINT('Ctrl Pts',(88.5552063716418,53.4002735747,13.2136255257334));
#72106=CARTESIAN_POINT('Ctrl Pts',(88.5807690891419,53.4030568699978,13.2010702936736));
#72107=CARTESIAN_POINT('Ctrl Pts',(88.5905942179696,53.4041378277624,13.196084912859));
#72108=CARTESIAN_POINT('Ctrl Pts',(88.608158994077,53.4060914880882,13.186883042628));
#72109=CARTESIAN_POINT('Ctrl Pts',(88.6159220864767,53.4069625285583,13.1827125497895));
#72110=CARTESIAN_POINT('Ctrl Pts',(88.6324828838084,53.4088375414358,13.173592396239));
#72111=CARTESIAN_POINT('Ctrl Pts',(88.641266159136,53.4098423464701,13.1686179957836));
#72112=CARTESIAN_POINT('Ctrl Pts',(88.6653836757304,53.4126310330154,13.1545767484904));
#72113=CARTESIAN_POINT('Ctrl Pts',(88.6805871360927,53.4144226573814,13.1452915810143));
#72114=CARTESIAN_POINT('Ctrl Pts',(88.7057337470706,53.417445128256,13.1291980435367));
#72115=CARTESIAN_POINT('Ctrl Pts',(88.7157848461693,53.418669540422,13.1225620450246));
#72116=CARTESIAN_POINT('Ctrl Pts',(88.7418933031712,53.4218938618913,13.1047862530261));
#72117=CARTESIAN_POINT('Ctrl Pts',(88.7577898985557,53.4239015101202,13.0934174663456));
#72118=CARTESIAN_POINT('Ctrl Pts',(88.8327674971458,53.4335891531515,13.0371361729708));
#72119=CARTESIAN_POINT('Ctrl Pts',(88.8880919137604,53.441417514281,12.9874739654833));
#72120=CARTESIAN_POINT('Ctrl Pts',(88.977981698057,53.4552869895173,12.8913154341149));
#72121=CARTESIAN_POINT('Ctrl Pts',(89.014320546775,53.4613141201742,12.8467362553351));
#72122=CARTESIAN_POINT('Ctrl Pts',(89.0532635774611,53.4681945067787,12.7917309572362));
#72123=CARTESIAN_POINT('Ctrl Pts',(89.0589116240661,53.4692040610727,12.7835514181491));
#72124=CARTESIAN_POINT('Ctrl Pts',(89.067607674981,53.470776074706,12.770636016785));
#72125=CARTESIAN_POINT('Ctrl Pts',(89.0707210090841,53.4713425583696,12.7659450567098));
#72126=CARTESIAN_POINT('Ctrl Pts',(89.0765635827895,53.4724124640642,12.7570135152552));
#72127=CARTESIAN_POINT('Ctrl Pts',(89.0792987988567,53.4729162319831,12.7527773332959));
#72128=CARTESIAN_POINT('Ctrl Pts',(89.0858223890336,53.4741249947116,12.7425406009205));
#72129=CARTESIAN_POINT('Ctrl Pts',(89.0895858520266,53.4748283734369,12.7365243628437));
#72130=CARTESIAN_POINT('Ctrl Pts',(89.1027301802048,53.4773079483199,12.7151148948363));
#72131=CARTESIAN_POINT('Ctrl Pts',(89.1118342568701,53.4790677482175,12.6995526749275));
#72132=CARTESIAN_POINT('Ctrl Pts',(89.1280472963119,53.4822937092311,12.6704331355535));
#72133=CARTESIAN_POINT('Ctrl Pts',(89.1352481784326,53.4837637017494,12.6569316091449));
#72134=CARTESIAN_POINT('Ctrl Pts',(89.1722531185891,53.4915413443748,12.5844217391698));
#72135=CARTESIAN_POINT('Ctrl Pts',(89.1976622421734,53.4976972963418,12.5232792095373));
#72136=CARTESIAN_POINT('Ctrl Pts',(89.2409203861896,53.510754763041,12.3908832282285));
#72137=CARTESIAN_POINT('Ctrl Pts',(89.2575877956678,53.5176441922671,12.3195137660679));
#72138=CARTESIAN_POINT('Ctrl Pts',(89.2702811037403,53.5262742114309,12.2314166371873));
#72139=CARTESIAN_POINT('Ctrl Pts',(89.272248599468,53.5278202924326,12.2156779167385));
#72140=CARTESIAN_POINT('Ctrl Pts',(89.2749419691799,53.5303253168196,12.1902759223732));
#72141=CARTESIAN_POINT('Ctrl Pts',(89.2758529362929,53.5312784358993,12.1806335158943));
#72142=CARTESIAN_POINT('Ctrl Pts',(89.2773886760471,53.533113463287,12.1621187693856));
#72143=CARTESIAN_POINT('Ctrl Pts',(89.278030703806,53.5339947760492,12.1532483926499));
#72144=CARTESIAN_POINT('Ctrl Pts',(89.2793043736349,53.5360470042544,12.1326482825649));
#72145=CARTESIAN_POINT('Ctrl Pts',(89.2798665269275,53.5372200139954,12.1209153052308));
#72146=CARTESIAN_POINT('Ctrl Pts',(89.2811730491244,53.5410747927666,12.082507475488));
#72147=CARTESIAN_POINT('Ctrl Pts',(89.2812394047926,53.5437771048086,12.0558189759272));
#72148=CARTESIAN_POINT('Ctrl Pts',(89.279351549044,53.5504275928278,11.9907820758287));
#72149=CARTESIAN_POINT('Ctrl Pts',(89.2764990454405,53.554399321915,11.9524884125613));
#72150=CARTESIAN_POINT('Ctrl Pts',(89.2661339457825,53.5634651656053,11.8662851949888));
#72151=CARTESIAN_POINT('Ctrl Pts',(89.2576027577796,53.5685740388597,11.8185565934819));
#72152=CARTESIAN_POINT('Ctrl Pts',(89.2319222088054,53.5802459506783,11.7108556917915));
#72153=CARTESIAN_POINT('Ctrl Pts',(89.2130387189582,53.5867946386327,11.651411261068));
#72154=CARTESIAN_POINT('Ctrl Pts',(89.1861418964584,53.5941774091248,11.5842929036424));
#72155=CARTESIAN_POINT('Ctrl Pts',(89.182308366679,53.595194280619,11.5750448732928));
#72156=CARTESIAN_POINT('Ctrl Pts',(89.1761425240416,53.5967751017487,11.5606538169309));
#72157=CARTESIAN_POINT('Ctrl Pts',(89.1738847311767,53.5973431469358,11.5554797039982));
#72158=CARTESIAN_POINT('Ctrl Pts',(89.1695469582974,53.5984141286884,11.545717074907));
#72159=CARTESIAN_POINT('Ctrl Pts',(89.1674741567402,53.5989174249613,11.54112582131));
#72160=CARTESIAN_POINT('Ctrl Pts',(89.1624292812693,53.6001225194474,11.5301264121205));
#72161=CARTESIAN_POINT('Ctrl Pts',(89.159430956467,53.6008227274255,11.523730474059));
#72162=CARTESIAN_POINT('Ctrl Pts',(89.1486857207714,53.6032779305565,11.5012979832534));
#72163=CARTESIAN_POINT('Ctrl Pts',(89.1406544459258,53.6050169525187,11.4853984879923));
#72164=CARTESIAN_POINT('Ctrl Pts',(89.1252304480136,53.6081973204011,11.4563963653593));
#72165=CARTESIAN_POINT('Ctrl Pts',(89.1179346531099,53.6096425414535,11.4432465898851));
#72166=CARTESIAN_POINT('Ctrl Pts',(89.0783432864674,53.6172016754727,11.3747832724085));
#72167=CARTESIAN_POINT('Ctrl Pts',(89.0421284568892,53.6231718792804,11.3218374218185));
#72168=CARTESIAN_POINT('Ctrl Pts',(88.9586340692464,53.6356853680847,11.217640040739));
#72169=CARTESIAN_POINT('Ctrl Pts',(88.9108310694222,53.6422153736724,11.1670969481297));
#72170=CARTESIAN_POINT('Ctrl Pts',(88.8461424890644,53.6506060544648,11.1090558822231));
#72171=CARTESIAN_POINT('Ctrl Pts',(88.8329046808739,53.6523017639449,11.0976624308889));
#72172=CARTESIAN_POINT('Ctrl Pts',(88.8109397090098,53.6550851657703,11.0795326391947));
#72173=CARTESIAN_POINT('Ctrl Pts',(88.8023519489175,53.6561661473626,11.0726302469969));
#72174=CARTESIAN_POINT('Ctrl Pts',(88.7867357361356,53.6581198332789,11.0604097616439));
#72175=CARTESIAN_POINT('Ctrl Pts',(88.779739556562,53.6589908753236,11.0550513642729));
#72176=CARTESIAN_POINT('Ctrl Pts',(88.7646113938964,53.6608658722791,11.0437124892815));
#72177=CARTESIAN_POINT('Ctrl Pts',(88.7564628059474,53.6618706596769,11.0377553416448));
#72178=CARTESIAN_POINT('Ctrl Pts',(88.7337400591966,53.6646592440665,11.0215555977138));
#72179=CARTESIAN_POINT('Ctrl Pts',(88.7190207791399,53.6664507829694,11.0115220266858));
#72180=CARTESIAN_POINT('Ctrl Pts',(88.6855108820365,53.6704992528545,10.9896975309784));
#72181=CARTESIAN_POINT('Ctrl Pts',(88.6666130533864,53.67276188235,10.9780830417959));
#72182=CARTESIAN_POINT('Ctrl Pts',(88.602455349279,53.6803799305159,10.9409308300515));
#72183=CARTESIAN_POINT('Ctrl Pts',(88.5559389544959,53.6858031451973,10.9176794012558));
#72184=CARTESIAN_POINT('Ctrl Pts',(88.4312121177589,53.7000586730948,10.8646217120435));
#72185=CARTESIAN_POINT('Ctrl Pts',(88.3512396705861,53.7089328416846,10.8395712402414));
#72186=CARTESIAN_POINT('Ctrl Pts',(88.2576175200656,53.7187474075095,10.8201171399385));
#72187=CARTESIAN_POINT('Ctrl Pts',(88.2458213257682,53.7199735538201,10.8178400407036));
#72188=CARTESIAN_POINT('Ctrl Pts',(88.2279678130038,53.7218119895713,10.8146557482068));
#72189=CARTESIAN_POINT('Ctrl Pts',(88.2219338513308,53.7224303527924,10.8136245034682));
#72190=CARTESIAN_POINT('Ctrl Pts',(88.2109382800165,53.7235515169876,10.8118270119901));
#72191=CARTESIAN_POINT('Ctrl Pts',(88.2059791600429,53.7240550771237,10.8110464823259));
#72192=CARTESIAN_POINT('Ctrl Pts',(88.1955383257625,53.7251107239863,10.8094665582754));
#72193=CARTESIAN_POINT('Ctrl Pts',(88.1900558198364,53.7256624524202,10.8086735898869));
#72194=CARTESIAN_POINT('Ctrl Pts',(88.1751391518321,53.7271569958738,10.8066156519063));
#72195=CARTESIAN_POINT('Ctrl Pts',(88.165695350603,53.7280960512637,10.8054207815989));
#72196=CARTESIAN_POINT('Ctrl Pts',(88.110183777952,53.7335790675027,10.7990304967894));
#72197=CARTESIAN_POINT('Ctrl Pts',(88.0638650818169,53.738005843388,10.7962535985385));
#72198=CARTESIAN_POINT('Ctrl Pts',(87.9203700546664,53.7515648895685,10.7955202181334));
#72199=CARTESIAN_POINT('Ctrl Pts',(87.8235171925083,53.7605208532554,10.8061656460052));
#72200=CARTESIAN_POINT('Ctrl Pts',(87.6987427862446,53.7727394791197,10.8345994491986));
#72201=CARTESIAN_POINT('Ctrl Pts',(87.668924110744,53.7757102978226,10.8425476629295));
#72202=CARTESIAN_POINT('Ctrl Pts',(87.6272754210389,53.7799532090743,10.8552907325108));
#72203=CARTESIAN_POINT('Ctrl Pts',(87.6151809256083,53.7811966276637,10.8591906882591));
#72204=CARTESIAN_POINT('Ctrl Pts',(87.5946628477819,53.7833268368108,10.8661484911236));
#72205=CARTESIAN_POINT('Ctrl Pts',(87.5862091529078,53.7842105935675,10.8691152964586));
#72206=CARTESIAN_POINT('Ctrl Pts',(87.5701273551783,53.7859039369664,10.8749509997062));
#72207=CARTESIAN_POINT('Ctrl Pts',(87.5624940540122,53.7867129697123,10.8778043853999));
#72208=CARTESIAN_POINT('Ctrl Pts',(87.5429750969172,53.7887957477423,10.885315601271));
#72209=CARTESIAN_POINT('Ctrl Pts',(87.5311316064293,53.7900729717251,10.8900794016814));
#72210=CARTESIAN_POINT('Ctrl Pts',(87.505759343155,53.7928394602801,10.9007319866757));
#72211=CARTESIAN_POINT('Ctrl Pts',(87.4922575138148,53.7943305434619,10.9066795737546));
#72212=CARTESIAN_POINT('Ctrl Pts',(87.4540644936607,53.7986043003359,10.9243044321128));
#72213=CARTESIAN_POINT('Ctrl Pts',(87.4296439162768,53.8014048315963,10.9365440420089));
#72214=CARTESIAN_POINT('Ctrl Pts',(87.338102664363,53.8121704423523,10.9861799518255));
#72215=CARTESIAN_POINT('Ctrl Pts',(87.274036090704,53.8202832533066,11.0288484074807));
#72216=CARTESIAN_POINT('Ctrl Pts',(87.1721700492341,53.8340593509287,11.1109182916318));
#72217=CARTESIAN_POINT('Ctrl Pts',(87.1323115452117,53.8397179275001,11.1474548667143));
#72218=CARTESIAN_POINT('Ctrl Pts',(87.088025414481,53.8462457087994,11.193580191624));
#72219=CARTESIAN_POINT('Ctrl Pts',(87.0812386734784,53.8472532929789,11.2008166058618));
#72220=CARTESIAN_POINT('Ctrl Pts',(87.0707369416348,53.84882293458,11.212280473454));
#72221=CARTESIAN_POINT('Ctrl Pts',(87.0669643006591,53.849388997233,11.2164540908107));
#72222=CARTESIAN_POINT('Ctrl Pts',(87.059862004756,53.8504586166493,11.2244169944347));
#72223=CARTESIAN_POINT('Ctrl Pts',(87.0565271452581,53.8509625155647,11.2282010905067));
#72224=CARTESIAN_POINT('Ctrl Pts',(87.0498840262776,53.8519698519427,11.2358302524024));
#72225=CARTESIAN_POINT('Ctrl Pts',(87.0465761672355,53.8524732570309,11.2396753671932));
#72226=CARTESIAN_POINT('Ctrl Pts',(87.0355052617916,53.8541646747381,11.2527014296199));
#72227=CARTESIAN_POINT('Ctrl Pts',(87.0278491601786,53.8553454513114,11.2619732509114));
#72228=CARTESIAN_POINT('Ctrl Pts',(86.9931989627852,53.8607493197772,11.3051711380689));
#72229=CARTESIAN_POINT('Ctrl Pts',(86.9678177390817,53.8648799917736,11.3403613686492));
#72230=CARTESIAN_POINT('Ctrl Pts',(86.8978245348265,53.8770552709313,11.4486919645222));
#72231=CARTESIAN_POINT('Ctrl Pts',(86.858756279572,53.8849730260875,11.5251088653218));
#72232=CARTESIAN_POINT('Ctrl Pts',(86.8138425110357,53.8967233255252,11.6403654185521));
#72233=CARTESIAN_POINT('Ctrl Pts',(86.8016176322635,53.9003750519474,11.6764560070783));
#72234=CARTESIAN_POINT('Ctrl Pts',(86.787231252252,53.9054097134905,11.7261805659641));
#72235=CARTESIAN_POINT('Ctrl Pts',(86.7836415410765,53.9067467444399,11.7393834450648));
#72236=CARTESIAN_POINT('Ctrl Pts',(86.7782150904638,53.9089070967039,11.7606961253094));
#72237=CARTESIAN_POINT('Ctrl Pts',(86.7762433873895,53.9097260516932,11.7687708148808));
#72238=CARTESIAN_POINT('Ctrl Pts',(86.7723033992911,53.9114365702296,11.7856223395694));
#72239=CARTESIAN_POINT('Ctrl Pts',(86.7703488253289,53.912328520507,11.7944018533713));
#72240=CARTESIAN_POINT('Ctrl Pts',(86.7666474487188,53.9141084381533,11.8119019490776));
#72241=CARTESIAN_POINT('Ctrl Pts',(86.7648986721547,53.914996287898,11.8206215947707));
#72242=CARTESIAN_POINT('Ctrl Pts',(86.7610045829513,53.9170897039602,11.8411542756627));
#72243=CARTESIAN_POINT('Ctrl Pts',(86.7589349747071,53.9182975815157,11.8529805420042));
#72244=CARTESIAN_POINT('Ctrl Pts',(86.7462970460061,53.9263601260066,11.9317589099448));
#72245=CARTESIAN_POINT('Ctrl Pts',(86.7409382294059,53.9333728463356,11.999419128777));
#72246=CARTESIAN_POINT('Ctrl Pts',(86.7410005370969,53.9404808185598,12.0671680007619));
#72247=CARTESIAN_POINT('Ctrl Pts',(86.7410005364398,53.9404807435815,12.0671672861144));
#72248=CARTESIAN_POINT('Ctrl Pts',(86.7410774089203,53.9492556144373,12.1508040292818));
#72249=CARTESIAN_POINT('Ctrl Pts',(86.7494157570709,53.9581444962025,12.2342329466652));
#72250=CARTESIAN_POINT('Ctrl Pts',(86.7688445984371,53.968341402801,12.330902980819));
#72251=CARTESIAN_POINT('Ctrl Pts',(86.7720501381706,53.969878990606,12.345511955724));
#72252=CARTESIAN_POINT('Ctrl Pts',(86.7771489511873,53.9721258255758,12.3669343715233));
#72253=CARTESIAN_POINT('Ctrl Pts',(86.7788420704812,53.9728440139614,12.3737933580615));
#72254=CARTESIAN_POINT('Ctrl Pts',(86.7818560468689,53.9740756904126,12.3855796582954));
#72255=CARTESIAN_POINT('Ctrl Pts',(86.7831494855596,53.9745905597395,12.3905136868546));
#72256=CARTESIAN_POINT('Ctrl Pts',(86.785784663883,53.9756126975312,12.4003246352557));
#72257=CARTESIAN_POINT('Ctrl Pts',(86.7871258895036,53.9761199808866,12.4052016333851));
#72258=CARTESIAN_POINT('Ctrl Pts',(86.7900098943165,53.9771839811387,12.4154486725062));
#72259=CARTESIAN_POINT('Ctrl Pts',(86.7915590183176,53.9777403313606,12.420816726675));
#72260=CARTESIAN_POINT('Ctrl Pts',(86.7959055217669,53.9792611371941,12.4355135363661));
#72261=CARTESIAN_POINT('Ctrl Pts',(86.7987749560635,53.9802216080124,12.4448209455089));
#72262=CARTESIAN_POINT('Ctrl Pts',(86.8161707011016,53.9858048695619,12.4990236134905));
#72263=CARTESIAN_POINT('Ctrl Pts',(86.8330853920197,53.9903068880614,12.5431218244563));
#72264=CARTESIAN_POINT('Ctrl Pts',(86.8820836768189,54.0016038173732,12.6522535615841));
#72265=CARTESIAN_POINT('Ctrl Pts',(86.9173456295729,54.0083221859697,12.7156659144132));
#72266=CARTESIAN_POINT('Ctrl Pts',(86.9854956949888,54.0198335403661,12.8167951369301));
#72267=CARTESIAN_POINT('Ctrl Pts',(87.0155449349726,54.0245513528329,12.8562027721401));
#72268=CARTESIAN_POINT('Ctrl Pts',(87.0573017404777,54.0307715628485,12.9047917088545));
#72269=CARTESIAN_POINT('Ctrl Pts',(87.0669781102026,54.032191910796,12.9156673059788));
#72270=CARTESIAN_POINT('Ctrl Pts',(87.0771017205844,54.0336580390481,12.926659139456));
#72271=CARTESIAN_POINT('Ctrl Pts',(87.077364775672,54.0336961218725,12.9269444921234));
#72272=CARTESIAN_POINT('Ctrl Pts',(87.0778940974583,54.033772725348,12.927518153414));
#72273=CARTESIAN_POINT('Ctrl Pts',(87.0781603670495,54.0338112461138,12.9278064592564));
#72274=CARTESIAN_POINT('Ctrl Pts',(87.0786989203184,54.0338891298909,12.9283890407244));
#72275=CARTESIAN_POINT('Ctrl Pts',(87.0789712097866,54.0339284931401,12.9286833109255));
#72276=CARTESIAN_POINT('Ctrl Pts',(87.0795249682822,54.0340085175775,12.9292812037212));
#72277=CARTESIAN_POINT('Ctrl Pts',(87.0798064465256,54.0340491791475,12.9295848177096));
#72278=CARTESIAN_POINT('Ctrl Pts',(87.0803822894288,54.0341323327005,12.9302053366248));
#72279=CARTESIAN_POINT('Ctrl Pts',(87.0806766675609,54.0341748252385,12.9305222288629));
#72280=CARTESIAN_POINT('Ctrl Pts',(87.0812828050402,54.0342622851492,12.9311740557667));
#72281=CARTESIAN_POINT('Ctrl Pts',(87.081594583547,54.0343072533134,12.9315089723637));
#72282=CARTESIAN_POINT('Ctrl Pts',(87.0822411605697,54.0344004715382,12.9322027817289));
#72283=CARTESIAN_POINT('Ctrl Pts',(87.0825759862102,54.0344487227287,12.9325616489964));
#72284=CARTESIAN_POINT('Ctrl Pts',(87.0832759761026,54.0345495528775,12.9333110291756));
#72285=CARTESIAN_POINT('Ctrl Pts',(87.0836411789779,54.0346021334467,12.9337015056552));
#72286=CARTESIAN_POINT('Ctrl Pts',(87.0844117616438,54.0347130262685,12.9345243737721));
#72287=CARTESIAN_POINT('Ctrl Pts',(87.0848171976186,54.0347713408721,12.9349567123087));
#72288=CARTESIAN_POINT('Ctrl Pts',(87.0856819839576,54.0348956592984,12.9358775884344));
#72289=CARTESIAN_POINT('Ctrl Pts',(87.08614141865,54.0349616666589,12.9363660460818));
#72290=CARTESIAN_POINT('Ctrl Pts',(87.0871342276459,54.0351042199292,12.9374198981166));
#72291=CARTESIAN_POINT('Ctrl Pts',(87.0876677342188,54.0351807714096,12.9379851668015));
#72292=CARTESIAN_POINT('Ctrl Pts',(87.088720540459,54.0353317328197,12.9390986019172));
#72293=CARTESIAN_POINT('Ctrl Pts',(87.0892398107883,54.0354061414805,12.9396467957585));
#72294=CARTESIAN_POINT('Ctrl Pts',(87.0905308512817,54.0355910187751,12.941007315263));
#72295=CARTESIAN_POINT('Ctrl Pts',(87.0913032064837,54.0357015122499,12.9418190814783));
#72296=CARTESIAN_POINT('Ctrl Pts',(87.0981508446169,54.0366801881847,12.9489970881405));
#72297=CARTESIAN_POINT('Ctrl Pts',(87.1042908739419,54.037551123617,12.9553008427873));
#72298=CARTESIAN_POINT('Ctrl Pts',(87.118128539811,54.039499851941,12.969215214179));
#72299=CARTESIAN_POINT('Ctrl Pts',(87.1258588598495,54.0405790426804,12.9767921337576));
#72300=CARTESIAN_POINT('Ctrl Pts',(87.1458321042446,54.043344475069,12.9958745931005));
#72301=CARTESIAN_POINT('Ctrl Pts',(87.1582077453494,54.0450366054679,13.0072372431507));
#72302=CARTESIAN_POINT('Ctrl Pts',(87.174069591308,54.0471802137722,13.0212310982307));
#72303=CARTESIAN_POINT('Ctrl Pts',(87.1773491320214,54.0476220959016,13.0240945565846));
#72304=CARTESIAN_POINT('Ctrl Pts',(87.1806428502938,54.0480645842206,13.0269406869999));
#72305=CARTESIAN_POINT('Ctrl Pts',(87.1806428209146,54.2176482202995,13.026940661613));
#72306=CARTESIAN_POINT('Ctrl Pts',(87.1452504011479,54.2131348764096,12.996357764029));
#72307=CARTESIAN_POINT('Ctrl Pts',(87.1115603032837,54.2087186693022,12.9638305417161));
#72308=CARTESIAN_POINT('Ctrl Pts',(87.0467713246626,54.1997705438192,12.8939570940156));
#72309=CARTESIAN_POINT('Ctrl Pts',(87.0158741148475,54.1952486465662,12.8565531707686));
#72310=CARTESIAN_POINT('Ctrl Pts',(86.9644944811698,54.1870763956072,12.7865535725928));
#72311=CARTESIAN_POINT('Ctrl Pts',(86.9432127007455,54.1834459049798,12.7546225877747));
#72312=CARTESIAN_POINT('Ctrl Pts',(86.9096381452467,54.1772134858484,12.6989402662999));
#72313=CARTESIAN_POINT('Ctrl Pts',(86.8965905957655,54.174636889643,12.6756743072217));
#72314=CARTESIAN_POINT('Ctrl Pts',(86.8788676274429,54.1708887549885,12.6415989755517));
#72315=CARTESIAN_POINT('Ctrl Pts',(86.8735941890102,54.1697380961456,12.6311069706101));
#72316=CARTESIAN_POINT('Ctrl Pts',(86.8645847070452,54.1677072020006,12.612544633227));
#72317=CARTESIAN_POINT('Ctrl Pts',(86.8607864545929,54.1668291826751,12.6045051994745));
#72318=CARTESIAN_POINT('Ctrl Pts',(86.8530285148853,54.1649887233119,12.587628043773));
#72319=CARTESIAN_POINT('Ctrl Pts',(86.8490848963894,54.1640257985537,12.5787836337886));
#72320=CARTESIAN_POINT('Ctrl Pts',(86.8389503302454,54.1614765140877,12.5553374099452));
#72321=CARTESIAN_POINT('Ctrl Pts',(86.8329313494374,54.1598844859821,12.5406638022288));
#72322=CARTESIAN_POINT('Ctrl Pts',(86.8006921590715,54.1508945143421,12.4576749218825));
#72323=CARTESIAN_POINT('Ctrl Pts',(86.7801458233677,54.1433138737863,12.3873216522661));
#72324=CARTESIAN_POINT('Ctrl Pts',(86.7527767831557,54.1286851747907,12.2507841957157));
#72325=CARTESIAN_POINT('Ctrl Pts',(86.744864362002,54.121679725967,12.1850450812428));
#72326=CARTESIAN_POINT('Ctrl Pts',(86.7414675389801,54.113186815787,12.1037015291466));
#72327=CARTESIAN_POINT('Ctrl Pts',(86.7411054460214,54.1115976140026,12.0884042004117));
#72328=CARTESIAN_POINT('Ctrl Pts',(86.7409190489905,54.1081570085854,12.0550785338904));
#72329=CARTESIAN_POINT('Ctrl Pts',(86.741201971086,54.1063096229264,12.0370520622072));
#72330=CARTESIAN_POINT('Ctrl Pts',(86.7421310113146,54.1037606345058,12.011946066198));
#72331=CARTESIAN_POINT('Ctrl Pts',(86.7424527987386,54.1030436523913,12.0048579929283));
#72332=CARTESIAN_POINT('Ctrl Pts',(86.7431048214481,54.1018226752449,11.9927386083271));
#72333=CARTESIAN_POINT('Ctrl Pts',(86.7434056364446,54.1013171283638,11.987706005492));
#72334=CARTESIAN_POINT('Ctrl Pts',(86.7441057043148,54.1002507981529,11.9770588902709));
#72335=CARTESIAN_POINT('Ctrl Pts',(86.7445123191759,54.0996904225213,11.9714450620343));
#72336=CARTESIAN_POINT('Ctrl Pts',(86.7457398629063,54.0981463162111,11.9559295892261));
#72337=CARTESIAN_POINT('Ctrl Pts',(86.7466397088983,54.0971667758778,11.9460342270354));
#72338=CARTESIAN_POINT('Ctrl Pts',(86.753462231243,54.0906247524847,11.8796561964146));
#72339=CARTESIAN_POINT('Ctrl Pts',(86.7630528461093,54.0852392204285,11.8236043980689));
#72340=CARTESIAN_POINT('Ctrl Pts',(86.7938720768371,54.0728695065694,11.6957581542139));
#72341=CARTESIAN_POINT('Ctrl Pts',(86.8177483610913,54.0659350576208,11.6248317152101));
#72342=CARTESIAN_POINT('Ctrl Pts',(86.8585329065731,54.0562880486032,11.5317285163744));
#72343=CARTESIAN_POINT('Ctrl Pts',(86.8701297135073,54.0537136447811,11.5073935156067));
#72344=CARTESIAN_POINT('Ctrl Pts',(86.8919621904196,54.0491248629058,11.4651000828709));
#72345=CARTESIAN_POINT('Ctrl Pts',(86.9018787347758,54.0471210451209,11.4469876943142));
#72346=CARTESIAN_POINT('Ctrl Pts',(86.9175787775237,54.0440589315388,11.4199011502146));
#72347=CARTESIAN_POINT('Ctrl Pts',(86.9230416266576,54.0430120750963,11.410744130681));
#72348=CARTESIAN_POINT('Ctrl Pts',(86.9327696084529,54.041178843936,11.3948948051827));
#72349=CARTESIAN_POINT('Ctrl Pts',(86.93698345927,54.0403943776376,11.3881715388263));
#72350=CARTESIAN_POINT('Ctrl Pts',(86.946672078271,54.0386118204885,11.3730303725156));
#72351=CARTESIAN_POINT('Ctrl Pts',(86.9521841608399,54.0376123875257,11.3646371598997));
#72352=CARTESIAN_POINT('Ctrl Pts',(86.9673556778885,54.0348997894766,11.3421220773424));
#72353=CARTESIAN_POINT('Ctrl Pts',(86.9772014826095,54.033179731932,11.3281292321384));
#72354=CARTESIAN_POINT('Ctrl Pts',(87.049229071842,54.020867390024,11.2300359650397));
#72355=CARTESIAN_POINT('Ctrl Pts',(87.1212936806378,54.0098816986994,11.1537224746171));
#72356=CARTESIAN_POINT('Ctrl Pts',(87.233316938063,53.9945638770265,11.0611248684566));
#72357=CARTESIAN_POINT('Ctrl Pts',(87.2660047324878,53.9902734837296,11.036656733222));
#72358=CARTESIAN_POINT('Ctrl Pts',(87.3189208879931,53.983647056243,11.000890510969));
#72359=CARTESIAN_POINT('Ctrl Pts',(87.3383755947283,53.9812739783418,10.9884990219838));
#72360=CARTESIAN_POINT('Ctrl Pts',(87.3648208636924,53.978140601786,10.9726506307202));
#72361=CARTESIAN_POINT('Ctrl Pts',(87.3715195148245,53.9773546256594,10.9687192520859));
#72362=CARTESIAN_POINT('Ctrl Pts',(87.3827303395892,53.9760524813875,10.9622772602455));
#72363=CARTESIAN_POINT('Ctrl Pts',(87.3872223883075,53.9755342291853,10.9597323342925));
#72364=CARTESIAN_POINT('Ctrl Pts',(87.3958519078256,53.9745454739766,10.954912643268));
#72365=CARTESIAN_POINT('Ctrl Pts',(87.3999867131435,53.974074679926,10.9526334585611));
#72366=CARTESIAN_POINT('Ctrl Pts',(87.411285725228,53.9727959279774,10.9464871301954));
#72367=CARTESIAN_POINT('Ctrl Pts',(87.4184747782267,53.9719907666679,10.9426656101503));
#72368=CARTESIAN_POINT('Ctrl Pts',(87.4471279635553,53.9688128720373,10.9277859233527));
#72369=CARTESIAN_POINT('Ctrl Pts',(87.4688709215971,53.9664702359408,10.9172705776264));
#72370=CARTESIAN_POINT('Ctrl Pts',(87.5582283065022,53.9570613150049,10.8771586054341));
#72371=CARTESIAN_POINT('Ctrl Pts',(87.6280679556381,53.9501984395087,10.8528587190258));
#72372=CARTESIAN_POINT('Ctrl Pts',(87.770028122764,53.9364695387322,10.816958237326));
#72373=CARTESIAN_POINT('Ctrl Pts',(87.8418107444953,53.9296293366728,10.8052284554274));
#72374=CARTESIAN_POINT('Ctrl Pts',(87.9298719804741,53.9210645337955,10.7984963534869));
#72375=CARTESIAN_POINT('Ctrl Pts',(87.9455704471089,53.9195315420915,10.7975891159698));
#72376=CARTESIAN_POINT('Ctrl Pts',(87.9709288032017,53.9170426217436,10.7965956025956));
#72377=CARTESIAN_POINT('Ctrl Pts',(87.980580366757,53.9160923817299,10.7963276572004));
#72378=CARTESIAN_POINT('Ctrl Pts',(87.9991331974031,53.9142594960961,10.7960242518575));
#72379=CARTESIAN_POINT('Ctrl Pts',(88.0080336641173,53.9133774200005,10.7959722788624));
#72380=CARTESIAN_POINT('Ctrl Pts',(88.0285381315914,53.9113384330585,10.7960680802873));
#72381=CARTESIAN_POINT('Ctrl Pts',(88.0401408087626,53.9101795529397,10.7962813472911));
#72382=CARTESIAN_POINT('Ctrl Pts',(88.0783240644833,53.9063476655699,10.7975068019968));
#72383=CARTESIAN_POINT('Ctrl Pts',(88.1048736211317,53.9036541536336,10.7991949652328));
#72384=CARTESIAN_POINT('Ctrl Pts',(88.2247184448708,53.891349956566,10.8106030784746));
#72385=CARTESIAN_POINT('Ctrl Pts',(88.3167996224409,53.8814639459333,10.8298056266883));
#72386=CARTESIAN_POINT('Ctrl Pts',(88.4546734630524,53.8661827805205,10.8749136740534));
#72387=CARTESIAN_POINT('Ctrl Pts',(88.5024354813102,53.8608008338611,10.8938117165615));
#72388=CARTESIAN_POINT('Ctrl Pts',(88.5602894635928,53.8542529043565,10.9208631636009));
#72389=CARTESIAN_POINT('Ctrl Pts',(88.5715718353867,53.8529746664114,10.9263436706061));
#72390=CARTESIAN_POINT('Ctrl Pts',(88.5882726868535,53.8510823733531,10.9347643057762));
#72391=CARTESIAN_POINT('Ctrl Pts',(88.5937534190231,53.8504613516962,10.9375779117248));
#72392=CARTESIAN_POINT('Ctrl Pts',(88.6036103921725,53.8493446754645,10.9427290915909));
#72393=CARTESIAN_POINT('Ctrl Pts',(88.6079935926367,53.848848216146,10.9450525150588));
#72394=CARTESIAN_POINT('Ctrl Pts',(88.6178998857648,53.8477263606179,10.9503781818722));
#72395=CARTESIAN_POINT('Ctrl Pts',(88.6234144524948,53.8471019381096,10.9533958219668));
#72396=CARTESIAN_POINT('Ctrl Pts',(88.6404393225424,53.845173682006,10.9628769821767));
#72397=CARTESIAN_POINT('Ctrl Pts',(88.6518720409121,53.8438780778468,10.9694794435844));
#72398=CARTESIAN_POINT('Ctrl Pts',(88.7350119539368,53.8344341155836,11.0192379815106));
#72399=CARTESIAN_POINT('Ctrl Pts',(88.8024136019785,53.8266470684094,11.069218188806));
#72400=CARTESIAN_POINT('Ctrl Pts',(88.9029230042319,53.8139301878386,11.1604189644734));
#72401=CARTESIAN_POINT('Ctrl Pts',(88.9392446499283,53.8090502815021,11.1976885705281));
#72402=CARTESIAN_POINT('Ctrl Pts',(88.9876594990274,53.8019745890153,11.2538863906094));
#72403=CARTESIAN_POINT('Ctrl Pts',(89.0016973148835,53.7998453505486,11.271071702612));
#72404=CARTESIAN_POINT('Ctrl Pts',(89.0261832243833,53.795976350256,11.3027042000749));
#72405=CARTESIAN_POINT('Ctrl Pts',(89.0367910905204,53.7942429093751,11.3170206805782));
#72406=CARTESIAN_POINT('Ctrl Pts',(89.0529308143438,53.7915093328552,11.3397892473091));
#72407=CARTESIAN_POINT('Ctrl Pts',(89.0586693440849,53.7905171205344,11.3480927566082));
#72408=CARTESIAN_POINT('Ctrl Pts',(89.0692303822464,53.7886517353787,11.3637706347628));
#72409=CARTESIAN_POINT('Ctrl Pts',(89.0740763391676,53.7877795091298,11.3711285655024));
#72410=CARTESIAN_POINT('Ctrl Pts',(89.0848065919618,53.7858104450746,11.3877959842441));
#72411=CARTESIAN_POINT('Ctrl Pts',(89.0906470392867,53.7847120662646,11.3971326477929));
#72412=CARTESIAN_POINT('Ctrl Pts',(89.1054272420102,53.7818612807239,11.4214586212093));
#72413=CARTESIAN_POINT('Ctrl Pts',(89.1141803847152,53.7801023363195,11.4365577561931));
#72414=CARTESIAN_POINT('Ctrl Pts',(89.1563168367608,53.7712647232938,11.512822959893));
#72415=CARTESIAN_POINT('Ctrl Pts',(89.1849305820884,53.7640269853221,11.5764710535249));
#72416=CARTESIAN_POINT('Ctrl Pts',(89.2295070319227,53.7499860653472,11.7023728720982));
#72417=CARTESIAN_POINT('Ctrl Pts',(89.2462591447343,53.7432172414619,11.7641401883981));
#72418=CARTESIAN_POINT('Ctrl Pts',(89.2611180185048,53.7349866104183,11.8416555402151));
#72419=CARTESIAN_POINT('Ctrl Pts',(89.2636834239061,53.7334273071814,11.8564533809709));
#72420=CARTESIAN_POINT('Ctrl Pts',(89.2687136535559,53.7300408118499,11.8888759465607));
#72421=CARTESIAN_POINT('Ctrl Pts',(89.2710718879255,53.7282176590526,11.9065148451159));
#72422=CARTESIAN_POINT('Ctrl Pts',(89.2738471033515,53.7256960756864,11.9312148486454));
#72423=CARTESIAN_POINT('Ctrl Pts',(89.2745768999791,53.7249826829541,11.9382374474331));
#72424=CARTESIAN_POINT('Ctrl Pts',(89.2757268741141,53.7237658386703,11.9502792369806));
#72425=CARTESIAN_POINT('Ctrl Pts',(89.2761758197216,53.7232608628,11.9552953882759));
#72426=CARTESIAN_POINT('Ctrl Pts',(89.277064663548,53.7221935019962,11.9659393734273));
#72427=CARTESIAN_POINT('Ctrl Pts',(89.2774968993691,53.7216315402728,11.9715676446691));
#72428=CARTESIAN_POINT('Ctrl Pts',(89.2785916406405,53.7200783628997,11.9871858877048));
#72429=CARTESIAN_POINT('Ctrl Pts',(89.2791735938267,53.7190914183823,11.9971814655512));
#72430=CARTESIAN_POINT('Ctrl Pts',(89.282522263607,53.7120035476859,12.0694102439732));
#72431=CARTESIAN_POINT('Ctrl Pts',(89.2808255258396,53.7061165425557,12.13177786816));
#72432=CARTESIAN_POINT('Ctrl Pts',(89.2696773275139,53.6957116902284,12.2420169720675));
#72433=CARTESIAN_POINT('Ctrl Pts',(89.2620411319101,53.6911891213685,12.289934433655));
#72434=CARTESIAN_POINT('Ctrl Pts',(89.2434919432652,53.6830167976973,12.3747625981709));
#72435=CARTESIAN_POINT('Ctrl Pts',(89.2336075385662,53.6793869309998,12.4118338791707));
#72436=CARTESIAN_POINT('Ctrl Pts',(89.2140325740849,53.6731554580471,12.473828108739));
#72437=CARTESIAN_POINT('Ctrl Pts',(89.2052047983294,53.670579173345,12.4989963113444));
#72438=CARTESIAN_POINT('Ctrl Pts',(89.1913588844973,53.6668314079365,12.5348184944832));
#72439=CARTESIAN_POINT('Ctrl Pts',(89.1869740556626,53.6656808009468,12.5457112411131));
#72440=CARTESIAN_POINT('Ctrl Pts',(89.1790046389428,53.6636499659003,12.564742641155));
#72441=CARTESIAN_POINT('Ctrl Pts',(89.17548435024,53.6627719534045,12.5729075326067));
#72442=CARTESIAN_POINT('Ctrl Pts',(89.1679514675653,53.6609314763122,12.5898865170836));
#72443=CARTESIAN_POINT('Ctrl Pts',(89.1639232254399,53.6599685267739,12.5986929734983));
#72444=CARTESIAN_POINT('Ctrl Pts',(89.153032704143,53.6574191011774,12.6217993058069));
#72445=CARTESIAN_POINT('Ctrl Pts',(89.1460028308883,53.6558269555751,12.6360176146151));
#72446=CARTESIAN_POINT('Ctrl Pts',(89.1051197283574,53.6468510496238,12.7149497508105));
#72447=CARTESIAN_POINT('Ctrl Pts',(89.0660073902115,53.6392853545012,12.7767661248979));
#72448=CARTESIAN_POINT('Ctrl Pts',(88.9880434050264,53.6257575059081,12.8792634541353));
#72449=CARTESIAN_POINT('Ctrl Pts',(88.9513868087343,53.6198554004453,12.9213852368911));
#72450=CARTESIAN_POINT('Ctrl Pts',(88.8932991622785,53.6112137878877,12.9798700489183));
#72451=CARTESIAN_POINT('Ctrl Pts',(88.873926140145,53.6084348393591,12.9981850649468));
#72452=CARTESIAN_POINT('Ctrl Pts',(88.8409965628351,53.6038927425522,13.0274091130975));
#72453=CARTESIAN_POINT('Ctrl Pts',(88.8277672466565,53.6021133600738,13.0386731966241));
#72454=CARTESIAN_POINT('Ctrl Pts',(88.8088912648143,53.5996413918402,13.0540882914258));
#72455=CARTESIAN_POINT('Ctrl Pts',(88.8034359992838,53.5989345843782,13.0584687085611));
#72456=CARTESIAN_POINT('Ctrl Pts',(88.7939994124706,53.5977252914003,13.0659185892293));
#72457=CARTESIAN_POINT('Ctrl Pts',(88.7900356548054,53.5972213320852,13.0690098295977));
#72458=CARTESIAN_POINT('Ctrl Pts',(88.7815572245223,53.5961519352171,13.0755413695585));
#72459=CARTESIAN_POINT('Ctrl Pts',(88.7770377095485,53.5955869501071,13.0789750467331));
#72460=CARTESIAN_POINT('Ctrl Pts',(88.7645785600711,53.5940427624159,13.0883097411461));
#72461=CARTESIAN_POINT('Ctrl Pts',(88.7565924790065,53.5930676556945,13.0941486908534));
#72462=CARTESIAN_POINT('Ctrl Pts',(88.6979295637554,53.5860039232337,13.1359964606998));
#72463=CARTESIAN_POINT('Ctrl Pts',(88.6447275843761,53.5801284639822,13.1683416361379));
#72464=CARTESIAN_POINT('Ctrl Pts',(88.5464070672245,53.5697574741116,13.2186347797761));
#72465=CARTESIAN_POINT('Ctrl Pts',(88.5022377493295,53.5652569076127,13.2381403916589));
#72466=CARTESIAN_POINT('Ctrl Pts',(88.4209541155103,53.5570872098767,13.2686326186366));
#72467=CARTESIAN_POINT('Ctrl Pts',(88.384246949572,53.5534371585868,13.280526176888));
#72468=CARTESIAN_POINT('Ctrl Pts',(88.3212393590593,53.5471750903146,13.2978150639335));
#72469=CARTESIAN_POINT('Ctrl Pts',(88.2952050747479,53.5445887437386,13.3040807929702));
#72470=CARTESIAN_POINT('Ctrl Pts',(88.2574800375832,53.5408290533537,13.3119076518311));
#72471=CARTESIAN_POINT('Ctrl Pts',(88.2459336004037,53.5396767739187,13.3141363974276));
#72472=CARTESIAN_POINT('Ctrl Pts',(88.2256030552416,53.5376440318289,13.317768601019));
#72473=CARTESIAN_POINT('Ctrl Pts',(88.2168318620694,53.5367657981367,13.3192407335524));
#72474=CARTESIAN_POINT('Ctrl Pts',(88.1984871034593,53.5349258882757,13.3221218955505));
#72475=CARTESIAN_POINT('Ctrl Pts',(88.1889114993275,53.5339637342582,13.323513862975));
#72476=CARTESIAN_POINT('Ctrl Pts',(88.1636369979451,53.5314188393498,13.3268934694608));
#72477=CARTESIAN_POINT('Ctrl Pts',(88.1479158546044,53.5298304656738,13.3286972658015));
#72478=CARTESIAN_POINT('Ctrl Pts',(88.0619889765172,53.5211146086696,13.3369327989064));
#72479=CARTESIAN_POINT('Ctrl Pts',(87.9913901625712,53.5138185211745,13.3378023642957));
#72480=CARTESIAN_POINT('Ctrl Pts',(87.8626381848231,53.5002697111586,13.3286652738885));
#72481=CARTESIAN_POINT('Ctrl Pts',(87.8045361113477,53.4940661992991,13.3204749509714));
#72482=CARTESIAN_POINT('Ctrl Pts',(87.7212732943293,53.4851434214448,13.3027947902325));
#72483=CARTESIAN_POINT('Ctrl Pts',(87.6955154855073,53.4823791994417,13.296476605255));
#72484=CARTESIAN_POINT('Ctrl Pts',(87.6532995552846,53.4778582397883,13.2847083222531));
#72485=CARTESIAN_POINT('Ctrl Pts',(87.6367220638024,53.4760854407113,13.2797197839208));
#72486=CARTESIAN_POINT('Ctrl Pts',(87.6136031291482,53.4736209479673,13.2722439772814));
#72487=CARTESIAN_POINT('Ctrl Pts',(87.6069734770703,53.4729151425032,13.2700396101214));
#72488=CARTESIAN_POINT('Ctrl Pts',(87.5956069833166,53.4717069948256,13.2661557784235));
#72489=CARTESIAN_POINT('Ctrl Pts',(87.5908614189479,53.4712031865013,13.264502744347));
#72490=CARTESIAN_POINT('Ctrl Pts',(87.580772298154,53.4701334626688,13.2609210823057));
#72491=CARTESIAN_POINT('Ctrl Pts',(87.5754317070703,53.4695680041429,13.2589847170942));
#72492=CARTESIAN_POINT('Ctrl Pts',(87.5608068928572,53.4680212129953,13.2535708187436));
#72493=CARTESIAN_POINT('Ctrl Pts',(87.5515497785602,53.4670439988229,13.2500201854786));
#72494=CARTESIAN_POINT('Ctrl Pts',(87.4839673931964,53.4599163535982,13.2231864349197));
#72495=CARTESIAN_POINT('Ctrl Pts',(87.4273873336932,53.4539834716108,13.1957093548275));
#72496=CARTESIAN_POINT('Ctrl Pts',(87.3296137954752,53.4433666361083,13.1389109049242));
#72497=CARTESIAN_POINT('Ctrl Pts',(87.2877010223443,53.4386802496924,13.1111140975397));
#72498=CARTESIAN_POINT('Ctrl Pts',(87.2246387717377,53.431247716195,13.0636761329904));
#72499=CARTESIAN_POINT('Ctrl Pts',(87.202325301845,53.4285357509339,13.0456766814791));
#72500=CARTESIAN_POINT('Ctrl Pts',(87.1806428308131,53.4258009314892,13.0269406701664));
#72501=CARTESIAN_POINT('Origin',(88.011,66.41344859951,12.066));
#72502=CARTESIAN_POINT('',(87.1806428354249,52.4628656574377,13.0269406741515));
#72503=CARTESIAN_POINT('',(87.1806428293121,52.6319631729084,13.0269406688694));
#72504=CARTESIAN_POINT('',(87.1806428354228,66.41344859951,13.0269406741497));
#72505=CARTESIAN_POINT('Ctrl Pts',(87.1806428354249,52.4628656574377,13.0269406741515));
#72506=CARTESIAN_POINT('Ctrl Pts',(87.1823742791358,52.4630959657415,13.0284368296678));
#72507=CARTESIAN_POINT('Ctrl Pts',(87.1841097925396,52.463325945256,13.0299283280082));
#72508=CARTESIAN_POINT('Ctrl Pts',(87.1894085350898,52.464025434346,13.0344572198663));
#72509=CARTESIAN_POINT('Ctrl Pts',(87.1929844642713,52.4644938131071,13.0374795455676));
#72510=CARTESIAN_POINT('Ctrl Pts',(87.201458071945,52.4655951445308,13.0445613565417));
#72511=CARTESIAN_POINT('Ctrl Pts',(87.2063696616142,52.4662268852427,13.0486039317712));
#72512=CARTESIAN_POINT('Ctrl Pts',(87.2218771673402,52.468201630086,13.0611734145365));
#72513=CARTESIAN_POINT('Ctrl Pts',(87.2325803858327,52.4695358283367,13.0695676005866));
#72514=CARTESIAN_POINT('Ctrl Pts',(87.3096735956759,52.4789615863688,13.1280535433542));
#72515=CARTESIAN_POINT('Ctrl Pts',(87.3807201693157,52.4867000534846,13.1716984530809));
#72516=CARTESIAN_POINT('Ctrl Pts',(87.5022452525584,52.4993623578523,13.2308030983649));
#72517=CARTESIAN_POINT('Ctrl Pts',(87.5502984157015,52.5042369908387,13.2506311297707));
#72518=CARTESIAN_POINT('Ctrl Pts',(87.6204046098024,52.5113059949499,13.2746467373196));
#72519=CARTESIAN_POINT('Ctrl Pts',(87.6415653099816,52.5134339706799,13.2812816877559));
#72520=CARTESIAN_POINT('Ctrl Pts',(87.6800151641187,52.5173009710025,13.2922406880998));
#72521=CARTESIAN_POINT('Ctrl Pts',(87.6972425256221,52.519033685865,13.2967612925169));
#72522=CARTESIAN_POINT('Ctrl Pts',(87.724372709713,52.5217665067826,13.3032738866751));
#72523=CARTESIAN_POINT('Ctrl Pts',(87.7342145487322,52.5227586991067,13.3055126758526));
#72524=CARTESIAN_POINT('Ctrl Pts',(87.7526973989221,52.524624279486,13.3094859980572));
#72525=CARTESIAN_POINT('Ctrl Pts',(87.7613318818579,52.525496722493,13.3112483615455));
#72526=CARTESIAN_POINT('Ctrl Pts',(87.7808022491705,52.5274665932623,13.3150117727668));
#72527=CARTESIAN_POINT('Ctrl Pts',(87.7916470715518,52.5285655653177,13.3169619043391));
#72528=CARTESIAN_POINT('Ctrl Pts',(87.8197466933412,52.5314185771291,13.3216382087006));
#72529=CARTESIAN_POINT('Ctrl Pts',(87.8370341115358,52.533179169902,13.3241498044262));
#72530=CARTESIAN_POINT('Ctrl Pts',(87.9233754684778,52.542004222068,13.3348804914783));
#72531=CARTESIAN_POINT('Ctrl Pts',(87.9929571080323,52.5492270024747,13.3377729134239));
#72532=CARTESIAN_POINT('Ctrl Pts',(88.1263516045711,52.5632616172065,13.3323684303559));
#72533=CARTESIAN_POINT('Ctrl Pts',(88.1900050836201,52.5700396018162,13.3249490044845));
#72534=CARTESIAN_POINT('Ctrl Pts',(88.2675827476387,52.5782804582478,13.3099015786419));
#72535=CARTESIAN_POINT('Ctrl Pts',(88.2822847477183,52.5798409831681,13.3067781746664));
#72536=CARTESIAN_POINT('Ctrl Pts',(88.3142741597248,52.5832297777446,13.2993862803844));
#72537=CARTESIAN_POINT('Ctrl Pts',(88.3315350822376,52.5850540078219,13.2950135501902));
#72538=CARTESIAN_POINT('Ctrl Pts',(88.3555080030124,52.587576899724,13.2884009627456));
#72539=CARTESIAN_POINT('Ctrl Pts',(88.3623006858114,52.5882905412783,13.2864661873842));
#72540=CARTESIAN_POINT('Ctrl Pts',(88.3739099895328,52.5895077554112,13.2830545233475));
#72541=CARTESIAN_POINT('Ctrl Pts',(88.3787344945672,52.5900128536705,13.2816054950424));
#72542=CARTESIAN_POINT('Ctrl Pts',(88.3889476423061,52.5910804261593,13.278471628976));
#72543=CARTESIAN_POINT('Ctrl Pts',(88.3943338421549,52.5916424773191,13.2767795180905));
#72544=CARTESIAN_POINT('Ctrl Pts',(88.409240642247,52.5931958221268,13.2719869976482));
#72545=CARTESIAN_POINT('Ctrl Pts',(88.4187364879145,52.5941828442802,13.268809721904));
#72546=CARTESIAN_POINT('Ctrl Pts',(88.4870166062117,52.6012693017236,13.2450618313528));
#72547=CARTESIAN_POINT('Ctrl Pts',(88.5442665422542,52.6071549270674,13.2203000051829));
#72548=CARTESIAN_POINT('Ctrl Pts',(88.6424211426496,52.6175562367526,13.1689758392418));
#72549=CARTESIAN_POINT('Ctrl Pts',(88.6840438071263,52.6220766717097,13.1440817922037));
#72550=CARTESIAN_POINT('Ctrl Pts',(88.7558918978885,52.630248660336,13.09532422512));
#72551=CARTESIAN_POINT('Ctrl Pts',(88.7866463255951,52.633880404465,13.0723521302925));
#72552=CARTESIAN_POINT('Ctrl Pts',(88.8369403570209,52.640114813673,13.0311084119627));
#72553=CARTESIAN_POINT('Ctrl Pts',(88.857029163468,52.6426921267512,13.0135474341148));
#72554=CARTESIAN_POINT('Ctrl Pts',(88.8851436743173,52.6464412526736,12.9873635491724));
#72555=CARTESIAN_POINT('Ctrl Pts',(88.8936269322807,52.647592173582,12.9792401814132));
#72556=CARTESIAN_POINT('Ctrl Pts',(88.9083334550585,52.6496235194173,12.9647612388746));
#72557=CARTESIAN_POINT('Ctrl Pts',(88.9146050211638,52.6505017272515,12.958455628959));
#72558=CARTESIAN_POINT('Ctrl Pts',(88.9275675017931,52.6523425762586,12.9451460800595));
#72559=CARTESIAN_POINT('Ctrl Pts',(88.9342455087131,52.6533057023011,12.9381304562682));
#72560=CARTESIAN_POINT('Ctrl Pts',(88.9516471836922,52.6558555212838,12.9194251634223));
#72561=CARTESIAN_POINT('Ctrl Pts',(88.9622327786363,52.657447884948,12.9076102280764));
#72562=CARTESIAN_POINT('Ctrl Pts',(89.0202758209102,52.6664201791749,12.8403322986654));
#72563=CARTESIAN_POINT('Ctrl Pts',(89.0630929910157,52.6739818345908,12.7810691260865));
#72564=CARTESIAN_POINT('Ctrl Pts',(89.1346129647296,52.6886052203436,12.6616362905329));
#72565=CARTESIAN_POINT('Ctrl Pts',(89.1641489655427,52.6956251131005,12.6022242664629));
#72566=CARTESIAN_POINT('Ctrl Pts',(89.1946418421869,52.7041340548743,12.5265720308245));
#72567=CARTESIAN_POINT('Ctrl Pts',(89.2001107648329,52.7057250924005,12.5122625312404));
#72568=CARTESIAN_POINT('Ctrl Pts',(89.2114541684645,52.7091690983356,12.4808918312051));
#72569=CARTESIAN_POINT('Ctrl Pts',(89.2172269717008,52.7110180491254,12.4637964956962));
#72570=CARTESIAN_POINT('Ctrl Pts',(89.2247611033712,52.7135688958206,12.4398106023941));
#72571=CARTESIAN_POINT('Ctrl Pts',(89.2268314715854,52.7142861973132,12.4330207403978));
#72572=CARTESIAN_POINT('Ctrl Pts',(89.2302751574187,52.7155076259154,12.4213779947144));
#72573=CARTESIAN_POINT('Ctrl Pts',(89.2316766654725,52.716013306784,12.4165337527103));
#72574=CARTESIAN_POINT('Ctrl Pts',(89.2345814793649,52.7170798301912,12.4062646726259));
#72575=CARTESIAN_POINT('Ctrl Pts',(89.2360776264963,52.7176402654713,12.4008380170699));
#72576=CARTESIAN_POINT('Ctrl Pts',(89.2401144566424,52.7191843691226,12.3858067380316));
#72577=CARTESIAN_POINT('Ctrl Pts',(89.2425786941156,52.7201638482998,12.3761816241583));
#72578=CARTESIAN_POINT('Ctrl Pts',(89.2582601139588,52.7266608149601,12.3117957102351));
#72579=CARTESIAN_POINT('Ctrl Pts',(89.2679366369789,52.7320043117928,12.2562262810163));
#72580=CARTESIAN_POINT('Ctrl Pts',(89.2818195819148,52.7443650466693,12.1255689132522));
#72581=CARTESIAN_POINT('Ctrl Pts',(89.2831190812652,52.751330386456,12.0503969934082));
#72582=CARTESIAN_POINT('Ctrl Pts',(89.2758512804784,52.7610151567976,11.9486079547546));
#72583=CARTESIAN_POINT('Ctrl Pts',(89.2730685294822,52.7635951417093,11.9217347057547));
#72584=CARTESIAN_POINT('Ctrl Pts',(89.2666460818684,52.7681929154307,11.8744779410276));
#72585=CARTESIAN_POINT('Ctrl Pts',(89.2633607333884,52.770200084597,11.8540559961083));
#72586=CARTESIAN_POINT('Ctrl Pts',(89.2576268216648,52.7732663856689,11.8232337839553));
#72587=CARTESIAN_POINT('Ctrl Pts',(89.2555431097102,52.7743140319397,11.8127682896456));
#72588=CARTESIAN_POINT('Ctrl Pts',(89.251680037624,52.7761482684735,11.794566695118));
#72589=CARTESIAN_POINT('Ctrl Pts',(89.2499595264022,52.776932945165,11.7868185545899));
#72590=CARTESIAN_POINT('Ctrl Pts',(89.2458985632029,52.7787154791357,11.7693076974282));
#72591=CARTESIAN_POINT('Ctrl Pts',(89.2435147782696,52.7797146755448,11.7595557305063));
#72592=CARTESIAN_POINT('Ctrl Pts',(89.2367605029523,52.7824253855073,11.7332788724281));
#72593=CARTESIAN_POINT('Ctrl Pts',(89.2321717875719,52.7841437730606,11.7168130136821));
#72594=CARTESIAN_POINT('Ctrl Pts',(89.1971120622441,52.7964665985134,11.6001641702151));
#72595=CARTESIAN_POINT('Ctrl Pts',(89.1546922661271,52.807465525127,11.5040202504589));
#72596=CARTESIAN_POINT('Ctrl Pts',(89.0800702195963,52.8227892616701,11.3792332701759));
#72597=CARTESIAN_POINT('Ctrl Pts',(89.0574896753962,52.8270726976908,11.3452923142248));
#72598=CARTESIAN_POINT('Ctrl Pts',(89.0196466282889,52.8336899689284,11.2939490414931));
#72599=CARTESIAN_POINT('Ctrl Pts',(89.0054749532874,52.8360607374529,11.2757781974143));
#72600=CARTESIAN_POINT('Ctrl Pts',(88.9858750436903,52.8391916859008,11.2520104772819));
#72601=CARTESIAN_POINT('Ctrl Pts',(88.9808797849678,52.839977491618,11.2460649368586));
#72602=CARTESIAN_POINT('Ctrl Pts',(88.972472747039,52.8412795081493,11.2362429189353));
#72603=CARTESIAN_POINT('Ctrl Pts',(88.9690913900066,52.8417978012411,11.2323408670968));
#72604=CARTESIAN_POINT('Ctrl Pts',(88.9625714739324,52.8427867725853,11.2249090201569));
#72605=CARTESIAN_POINT('Ctrl Pts',(88.9594368952985,52.8432577411085,11.2213759624957));
#72606=CARTESIAN_POINT('Ctrl Pts',(88.9508418827735,52.8445372385156,11.2117965072618));
#72607=CARTESIAN_POINT('Ctrl Pts',(88.9453426962689,52.8453429660223,11.2057848464429));
#72608=CARTESIAN_POINT('Ctrl Pts',(88.9232910610307,52.8485253607497,11.1821391926004));
#72609=CARTESIAN_POINT('Ctrl Pts',(88.9062925921666,52.8508718261795,11.1649248931283));
#72610=CARTESIAN_POINT('Ctrl Pts',(88.8355028162124,52.860281101975,11.0972191223858));
#72611=CARTESIAN_POINT('Ctrl Pts',(88.7778475790417,52.8671409590051,11.0509686130264));
#72612=CARTESIAN_POINT('Ctrl Pts',(88.6593817268734,52.8804987430598,10.9718249073616));
#72613=CARTESIAN_POINT('Ctrl Pts',(88.5992748881181,52.8869671663661,10.9383705084544));
#72614=CARTESIAN_POINT('Ctrl Pts',(88.5205318119235,52.8953336506621,10.9025588223497));
#72615=CARTESIAN_POINT('Ctrl Pts',(88.5041453972314,52.8970686588304,10.8955190803493));
#72616=CARTESIAN_POINT('Ctrl Pts',(88.4782570129851,52.8998042760683,10.8850373172108));
#72617=CARTESIAN_POINT('Ctrl Pts',(88.4688523560557,52.9007969440513,10.8813594723269));
#72618=CARTESIAN_POINT('Ctrl Pts',(88.451160703031,52.9026629411226,10.8746829947548));
#72619=CARTESIAN_POINT('Ctrl Pts',(88.4428843429044,52.903535321127,10.8716576889786));
#72620=CARTESIAN_POINT('Ctrl Pts',(88.4241962894727,52.9055044119707,10.86504617782));
#72621=CARTESIAN_POINT('Ctrl Pts',(88.4137682499115,52.9066026617624,10.8615088319652));
#72622=CARTESIAN_POINT('Ctrl Pts',(88.3867053417737,52.9094524596944,10.8527194151114));
#72623=CARTESIAN_POINT('Ctrl Pts',(88.3700065812749,52.9112105359099,10.8476739029728));
#72624=CARTESIAN_POINT('Ctrl Pts',(88.2800974423266,52.9206800557911,10.8225167652175));
#72625=CARTESIAN_POINT('Ctrl Pts',(88.2053140600595,52.9285834933689,10.808661086677));
#72626=CARTESIAN_POINT('Ctrl Pts',(88.0579048758485,52.9441695733533,10.7948161707603));
#72627=CARTESIAN_POINT('Ctrl Pts',(87.9856023694152,52.9518147146446,10.7942040359902));
#72628=CARTESIAN_POINT('Ctrl Pts',(87.8954880800442,52.9611473823246,10.8011331170657));
#72629=CARTESIAN_POINT('Ctrl Pts',(87.8773721915217,52.9630129813771,10.802918465057));
#72630=CARTESIAN_POINT('Ctrl Pts',(87.8522285098102,52.965582628126,10.805943519324));
#72631=CARTESIAN_POINT('Ctrl Pts',(87.845164635058,52.9663023712236,10.8068537173674));
#72632=CARTESIAN_POINT('Ctrl Pts',(87.8331090616176,52.9675266179231,10.8085103259716));
#72633=CARTESIAN_POINT('Ctrl Pts',(87.8281135894133,52.9680326940156,10.8092271359246));
#72634=CARTESIAN_POINT('Ctrl Pts',(87.8175660245862,52.9690985484034,10.8108048520815));
#72635=CARTESIAN_POINT('Ctrl Pts',(87.8120151923191,52.9696579298235,10.8116728444997));
#72636=CARTESIAN_POINT('Ctrl Pts',(87.7967150855748,52.9711960145643,10.8141694724645));
#72637=CARTESIAN_POINT('Ctrl Pts',(87.7869784265711,52.9721705819194,10.8158751857984));
#72638=CARTESIAN_POINT('Ctrl Pts',(87.7262729961519,52.9782262386956,10.82724192125));
#72639=CARTESIAN_POINT('Ctrl Pts',(87.6759070930623,52.9831606259344,10.8399062997474));
#72640=CARTESIAN_POINT('Ctrl Pts',(87.553773073519,52.9952364751671,10.8787096118044));
#72641=CARTESIAN_POINT('Ctrl Pts',(87.4833261242387,53.0023077546989,10.908297493803));
#72642=CARTESIAN_POINT('Ctrl Pts',(87.3780644970398,53.0135974124284,10.9641231634466));
#72643=CARTESIAN_POINT('Ctrl Pts',(87.3412172364548,53.0177006555736,10.9861249541763));
#72644=CARTESIAN_POINT('Ctrl Pts',(87.2940382427846,53.0232175586522,11.0176404554194));
#72645=CARTESIAN_POINT('Ctrl Pts',(87.2826464542447,53.0245709832951,11.0255227191019));
#72646=CARTESIAN_POINT('Ctrl Pts',(87.2638516843255,53.0268417395692,11.0389871944164));
#72647=CARTESIAN_POINT('Ctrl Pts',(87.2563765442531,53.0277551314488,11.0444671629876));
#72648=CARTESIAN_POINT('Ctrl Pts',(87.241761787677,53.0295618480941,11.0554290778574));
#72649=CARTESIAN_POINT('Ctrl Pts',(87.2346191387781,53.0304549392476,11.0609060921191));
#72650=CARTESIAN_POINT('Ctrl Pts',(87.2173516827805,53.0326393539961,11.0744407342887));
#72651=CARTESIAN_POINT('Ctrl Pts',(87.2072909123284,53.0339337721917,11.0825778630921));
#72652=CARTESIAN_POINT('Ctrl Pts',(87.1723812219749,53.0385042600995,11.1117062314311));
#72653=CARTESIAN_POINT('Ctrl Pts',(87.1482186488439,53.0418120395344,11.1334948218912));
#72654=CARTESIAN_POINT('Ctrl Pts',(87.0623102930519,53.0541387940927,11.2171618134637));
#72655=CARTESIAN_POINT('Ctrl Pts',(87.0061700679373,53.0633659433336,11.2844309088616));
#72656=CARTESIAN_POINT('Ctrl Pts',(86.9299582166029,53.0777384268249,11.3976720114085));
#72657=CARTESIAN_POINT('Ctrl Pts',(86.9049121616993,53.0828859921942,11.4399930945454));
#72658=CARTESIAN_POINT('Ctrl Pts',(86.8767379270176,53.0891833996016,11.4945974306205));
#72659=CARTESIAN_POINT('Ctrl Pts',(86.8712557038719,53.0904369016935,11.505612342601));
#72660=CARTESIAN_POINT('Ctrl Pts',(86.8632893563129,53.092300061176,11.522219099191));
#72661=CARTESIAN_POINT('Ctrl Pts',(86.8606844009173,53.0929163857274,11.5277515277105));
#72662=CARTESIAN_POINT('Ctrl Pts',(86.8562454710126,53.0939788184756,11.5373584034222));
#72663=CARTESIAN_POINT('Ctrl Pts',(86.8543929468679,53.094426011435,11.5414238978997));
#72664=CARTESIAN_POINT('Ctrl Pts',(86.850070254946,53.095478607935,11.5510445799515));
#72665=CARTESIAN_POINT('Ctrl Pts',(86.8476184599334,53.0960828972349,11.5566078569078));
#72666=CARTESIAN_POINT('Ctrl Pts',(86.8403979450442,53.097885302517,11.5733157574695));
#72667=CARTESIAN_POINT('Ctrl Pts',(86.8357485000002,53.0990766566255,11.5845118016098));
#72668=CARTESIAN_POINT('Ctrl Pts',(86.8017584495209,53.1080404802805,11.6697886326248));
#72669=CARTESIAN_POINT('Ctrl Pts',(86.7792818949578,53.1154771514103,11.746431270888));
#72670=CARTESIAN_POINT('Ctrl Pts',(86.7487691137389,53.1305199686773,11.9040920530442));
#72671=CARTESIAN_POINT('Ctrl Pts',(86.7410239596817,53.1380967716393,11.9847682564807));
#72672=CARTESIAN_POINT('Ctrl Pts',(86.7409950052116,53.1475755416504,12.0827072230892));
#72673=CARTESIAN_POINT('Ctrl Pts',(86.7413346216635,53.149238241815,12.0997872587707));
#72674=CARTESIAN_POINT('Ctrl Pts',(86.7424204882589,53.1518947598353,12.1268831867411));
#72675=CARTESIAN_POINT('Ctrl Pts',(86.742941254752,53.1528815493602,12.1369065886768));
#72676=CARTESIAN_POINT('Ctrl Pts',(86.7440864916012,53.1546553940199,12.1548434636506));
#72677=CARTESIAN_POINT('Ctrl Pts',(86.7446664669981,53.1554410169951,12.1627593650907));
#72678=CARTESIAN_POINT('Ctrl Pts',(86.7462002829072,53.1572886816428,12.1813065724569));
#72679=CARTESIAN_POINT('Ctrl Pts',(86.7472140159564,53.1583525422592,12.1919321193083));
#72680=CARTESIAN_POINT('Ctrl Pts',(86.7505868315951,53.1614919958295,12.2231211225857));
#72681=CARTESIAN_POINT('Ctrl Pts',(86.7533146938287,53.1635788800465,12.2436399273561));
#72682=CARTESIAN_POINT('Ctrl Pts',(86.7607596324566,53.1684278405857,12.2907890205622));
#72683=CARTESIAN_POINT('Ctrl Pts',(86.7658282467243,53.1711996524057,12.3173525847148));
#72684=CARTESIAN_POINT('Ctrl Pts',(86.7881848887099,53.1817656008263,12.4171095530073));
#72685=CARTESIAN_POINT('Ctrl Pts',(86.811112449967,53.1897012770843,12.4888731918023));
#72686=CARTESIAN_POINT('Ctrl Pts',(86.8620017324087,53.2035347978097,12.6099246723796));
#72687=CARTESIAN_POINT('Ctrl Pts',(86.8871665725444,53.2094217686278,12.6601813295732));
#72688=CARTESIAN_POINT('Ctrl Pts',(86.9206056157081,53.2161683758425,12.7171825919518));
#72689=CARTESIAN_POINT('Ctrl Pts',(86.9257327438217,53.2171773812698,12.7256921148064));
#72690=CARTESIAN_POINT('Ctrl Pts',(86.9339207137207,53.2187487340921,12.738927851421));
#72691=CARTESIAN_POINT('Ctrl Pts',(86.9369138375728,53.219315100488,12.7436950659087));
#72692=CARTESIAN_POINT('Ctrl Pts',(86.9426485136075,53.2203849262764,12.7526953710659));
#72693=CARTESIAN_POINT('Ctrl Pts',(86.9453836131954,53.2208887305173,12.7569320872768));
#72694=CARTESIAN_POINT('Ctrl Pts',(86.9520294677,53.2220977728255,12.7670932887489));
#72695=CARTESIAN_POINT('Ctrl Pts',(86.9559648042419,53.2228013928399,12.7730015079374));
#72696=CARTESIAN_POINT('Ctrl Pts',(86.9700772545258,53.2252828311546,12.7938086074734));
#72697=CARTESIAN_POINT('Ctrl Pts',(86.9805228532394,53.2270442206058,12.80852441132));
#72698=CARTESIAN_POINT('Ctrl Pts',(87.0004112541684,53.2302736778544,12.8353146849463));
#72699=CARTESIAN_POINT('Ctrl Pts',(87.0097653911286,53.2317455734891,12.847449941906));
#72700=CARTESIAN_POINT('Ctrl Pts',(87.0607361913128,53.2395402786966,12.9111567310743));
#72701=CARTESIAN_POINT('Ctrl Pts',(87.1061251458202,53.2457107582171,12.9595851144826));
#72702=CARTESIAN_POINT('Ctrl Pts',(87.163508176764,53.2529925397285,13.011932042438));
#72703=CARTESIAN_POINT('Ctrl Pts',(87.1720264167175,53.2540612142451,13.0194951526666));
#72704=CARTESIAN_POINT('Ctrl Pts',(87.180642873398,53.2551312395179,13.0269407069644));
#72705=CARTESIAN_POINT('Ctrl Pts',(87.1806428308131,53.4258009314892,13.0269406701664));
#72706=CARTESIAN_POINT('Ctrl Pts',(87.1743362995706,53.4250054859773,13.021491141811));
#72707=CARTESIAN_POINT('Ctrl Pts',(87.1680831488515,53.4242081263248,13.0159792999802));
#72708=CARTESIAN_POINT('Ctrl Pts',(87.1526872726662,53.4222224618141,13.0021368621377));
#72709=CARTESIAN_POINT('Ctrl Pts',(87.1436118734228,53.4210318639093,12.9937342173096));
#72710=CARTESIAN_POINT('Ctrl Pts',(87.1215109639658,53.4180797241952,12.9726638567472));
#72711=CARTESIAN_POINT('Ctrl Pts',(87.1086323299979,53.4163126955017,12.9598470804606));
#72712=CARTESIAN_POINT('Ctrl Pts',(87.0889835770527,53.4135381775367,12.9394352080008));
#72713=CARTESIAN_POINT('Ctrl Pts',(87.0820218227003,53.4125390165741,12.9320270653993));
#72714=CARTESIAN_POINT('Ctrl Pts',(87.0691988395837,53.4106674557414,12.918049336971));
#72715=CARTESIAN_POINT('Ctrl Pts',(87.0633154884272,53.4097960610142,12.9115007717413));
#72716=CARTESIAN_POINT('Ctrl Pts',(87.0502925727587,53.4078379539761,12.8966986971728));
#72717=CARTESIAN_POINT('Ctrl Pts',(87.0431904664282,53.4067497761132,12.8884133838061));
#72718=CARTESIAN_POINT('Ctrl Pts',(87.0252313496684,53.4039442570272,12.8669074889071));
#72719=CARTESIAN_POINT('Ctrl Pts',(87.0145335404841,53.4022207250683,12.8535577183681));
#72720=CARTESIAN_POINT('Ctrl Pts',(86.9496254954417,53.3914231563109,12.7691189825988));
#72721=CARTESIAN_POINT('Ctrl Pts',(86.9027909286916,53.3820734526397,12.692703495933));
#72722=CARTESIAN_POINT('Ctrl Pts',(86.8430929950701,53.3674346628164,12.5673411062292));
#72723=CARTESIAN_POINT('Ctrl Pts',(86.824442372871,53.3622125720084,12.521446286182));
#72724=CARTESIAN_POINT('Ctrl Pts',(86.8028678730855,53.3552387132727,12.4579504163095));
#72725=CARTESIAN_POINT('Ctrl Pts',(86.7975635046663,53.3534228278343,12.4412070441592));
#72726=CARTESIAN_POINT('Ctrl Pts',(86.7889868668633,53.3503052046175,12.4120470621341));
#72727=CARTESIAN_POINT('Ctrl Pts',(86.785552508179,53.3489968862542,12.3996812210068));
#72728=CARTESIAN_POINT('Ctrl Pts',(86.7807334664907,53.3470691505736,12.3812505326128));
#72729=CARTESIAN_POINT('Ctrl Pts',(86.7792050926382,53.3464423956993,12.3752247628335));
#72730=CARTESIAN_POINT('Ctrl Pts',(86.7765367977728,53.3453200200336,12.3643709214399));
#72731=CARTESIAN_POINT('Ctrl Pts',(86.7753808583461,53.3448235485095,12.3595471757687));
#72732=CARTESIAN_POINT('Ctrl Pts',(86.772837291566,53.343707371493,12.3486515437848));
#72733=CARTESIAN_POINT('Ctrl Pts',(86.7714660254179,53.3430885928258,12.3425760648276));
#72734=CARTESIAN_POINT('Ctrl Pts',(86.76739326784,53.3411960252479,12.323892510249));
#72735=CARTESIAN_POINT('Ctrl Pts',(86.7648388967869,53.3399300354423,12.3112525290357));
#72736=CARTESIAN_POINT('Ctrl Pts',(86.7513700162843,53.3327578184018,12.2389480823466));
#72737=CARTESIAN_POINT('Ctrl Pts',(86.7445464424472,53.3270381670947,12.1785910719884));
#72738=CARTESIAN_POINT('Ctrl Pts',(86.7389670051514,53.3142432876107,12.0423534299551));
#72739=CARTESIAN_POINT('Ctrl Pts',(86.742635134136,53.3072033728407,11.9666197628864));
#72740=CARTESIAN_POINT('Ctrl Pts',(86.7560566600149,53.2978758065233,11.8697709449612));
#72741=CARTESIAN_POINT('Ctrl Pts',(86.7596619502016,53.2957543189757,11.8479596572584));
#72742=CARTESIAN_POINT('Ctrl Pts',(86.7671881734674,53.2918980023108,11.8088078804139));
#72743=CARTESIAN_POINT('Ctrl Pts',(86.7709075752303,53.2901694303619,11.7914342521375));
#72744=CARTESIAN_POINT('Ctrl Pts',(86.7773070816809,53.2874417910367,11.7643322192337));
#72745=CARTESIAN_POINT('Ctrl Pts',(86.7797409192025,53.2864505890083,11.7545473902702));
#72746=CARTESIAN_POINT('Ctrl Pts',(86.7845195335236,53.2845860869579,11.7362678217));
#72747=CARTESIAN_POINT('Ctrl Pts',(86.7868367415506,53.2837137249435,11.7277664257047));
#72748=CARTESIAN_POINT('Ctrl Pts',(86.7922528064276,53.2817429947288,11.7086809604643));
#72749=CARTESIAN_POINT('Ctrl Pts',(86.7954013963993,53.2806430741272,11.6981119286266));
#72750=CARTESIAN_POINT('Ctrl Pts',(86.8039028215265,53.277785425259,11.6708762075711));
#72751=CARTESIAN_POINT('Ctrl Pts',(86.8094631084701,53.2760211059665,11.6542774845786));
#72752=CARTESIAN_POINT('Ctrl Pts',(86.8400105828043,53.2668309478734,11.568981708683));
#72753=CARTESIAN_POINT('Ctrl Pts',(86.8705468156836,53.2592285556787,11.5024349977368));
#72754=CARTESIAN_POINT('Ctrl Pts',(86.9368333641795,53.2451044765989,11.3856998462628));
#72755=CARTESIAN_POINT('Ctrl Pts',(86.9708449156313,53.2386288866275,11.33475436133));
#72756=CARTESIAN_POINT('Ctrl Pts',(87.0204768562574,53.2302005573834,11.2709206285754));
#72757=CARTESIAN_POINT('Ctrl Pts',(87.0329171919717,53.2281608980847,11.255665844093));
#72758=CARTESIAN_POINT('Ctrl Pts',(87.0547835720146,53.224704037964,11.2300902031486));
#72759=CARTESIAN_POINT('Ctrl Pts',(87.0640342951544,53.2232783350877,11.2196247538526));
#72760=CARTESIAN_POINT('Ctrl Pts',(87.0777917420912,53.2212131152558,11.204568835072));
#72761=CARTESIAN_POINT('Ctrl Pts',(87.0821631471431,53.2205647333298,11.1998571642833));
#72762=CARTESIAN_POINT('Ctrl Pts',(87.0899440778987,53.2194246594765,11.19159723377));
#72763=CARTESIAN_POINT('Ctrl Pts',(87.0933386676946,53.2189319149457,11.188035369674));
#72764=CARTESIAN_POINT('Ctrl Pts',(87.100929468367,53.2178403121735,11.1801626481716));
#72765=CARTESIAN_POINT('Ctrl Pts',(87.1051357102015,53.2172422366549,11.1758617633376));
#72766=CARTESIAN_POINT('Ctrl Pts',(87.1174343768849,53.2155125088264,11.1634638412944));
#72767=CARTESIAN_POINT('Ctrl Pts',(87.1256062680018,53.2143867011865,11.1554457657749));
#72768=CARTESIAN_POINT('Ctrl Pts',(87.1956854808461,53.2049159360581,11.088521372613));
#72769=CARTESIAN_POINT('Ctrl Pts',(87.2632970299013,53.1969638755544,11.0358793469521));
#72770=CARTESIAN_POINT('Ctrl Pts',(87.3801771608586,53.1840333805324,10.9624961337654));
#72771=CARTESIAN_POINT('Ctrl Pts',(87.4263416165389,53.1791058824947,10.9373583323227));
#72772=CARTESIAN_POINT('Ctrl Pts',(87.4941503445692,53.1719690393177,10.9057136033897));
#72773=CARTESIAN_POINT('Ctrl Pts',(87.5146182916453,53.1698275950103,10.896810895419));
#72774=CARTESIAN_POINT('Ctrl Pts',(87.5519033764804,53.1659386317299,10.88174892614));
#72775=CARTESIAN_POINT('Ctrl Pts',(87.5686366863371,53.1641975348209,10.8753972373276));
#72776=CARTESIAN_POINT('Ctrl Pts',(87.5950233905697,53.1614546236232,10.8660143026159));
#72777=CARTESIAN_POINT('Ctrl Pts',(87.6045888929747,53.160460824184,10.8627410041958));
#72778=CARTESIAN_POINT('Ctrl Pts',(87.6225597507285,53.1585940439212,10.8568301340054));
#72779=CARTESIAN_POINT('Ctrl Pts',(87.6309555187496,53.1577220231255,10.8541651208067));
#72780=CARTESIAN_POINT('Ctrl Pts',(87.6498864610458,53.1557555380268,10.8483720687597));
#72781=CARTESIAN_POINT('Ctrl Pts',(87.6604357180292,53.1546595503998,10.8452930607038));
#72782=CARTESIAN_POINT('Ctrl Pts',(87.6877601302789,53.151819397866,10.8377012838283));
#72783=CARTESIAN_POINT('Ctrl Pts',(87.7045896201895,53.15006877755,10.8333952976683));
#72784=CARTESIAN_POINT('Ctrl Pts',(87.8006196166402,53.1400662759991,10.8109131766325));
#72785=CARTESIAN_POINT('Ctrl Pts',(87.8813147875154,53.1315914198,10.8000305166795));
#72786=CARTESIAN_POINT('Ctrl Pts',(88.0175852036541,53.1172239105759,10.7948202513751));
#72787=CARTESIAN_POINT('Ctrl Pts',(88.0727745163799,53.1113950628162,10.7963048142722));
#72788=CARTESIAN_POINT('Ctrl Pts',(88.146254503647,53.1037117947099,10.8030852748142));
#72789=CARTESIAN_POINT('Ctrl Pts',(88.1647753570916,53.1017821873963,10.8052063503584));
#72790=CARTESIAN_POINT('Ctrl Pts',(88.1965351239592,53.0984914775908,10.8095539492406));
#72791=CARTESIAN_POINT('Ctrl Pts',(88.2097974223791,53.0971228444555,10.8115839616569));
#72792=CARTESIAN_POINT('Ctrl Pts',(88.2292631079569,53.0951243033126,10.8148800086814));
#72793=CARTESIAN_POINT('Ctrl Pts',(88.2354924915123,53.0944862887158,10.8159827423222));
#72794=CARTESIAN_POINT('Ctrl Pts',(88.2465929146709,53.0933524448222,10.8180334144628));
#72795=CARTESIAN_POINT('Ctrl Pts',(88.2514669066145,53.092855675258,10.8189633965339));
#72796=CARTESIAN_POINT('Ctrl Pts',(88.2623440776884,53.0917494404576,10.8211049621593));
#72797=CARTESIAN_POINT('Ctrl Pts',(88.2683440995254,53.0911408168332,10.8223314264609));
#72798=CARTESIAN_POINT('Ctrl Pts',(88.2864194141755,53.0893114371129,10.8261626179787));
#72799=CARTESIAN_POINT('Ctrl Pts',(88.298466398465,53.0880977465207,10.8289002873616));
#72800=CARTESIAN_POINT('Ctrl Pts',(88.3847382968194,53.0794328010571,10.849833952263));
#72801=CARTESIAN_POINT('Ctrl Pts',(88.4572412975141,53.0722879195457,10.8745246671426));
#72802=CARTESIAN_POINT('Ctrl Pts',(88.6031961230309,53.0573242846725,10.9394385622575));
#72803=CARTESIAN_POINT('Ctrl Pts',(88.6757708175089,53.0495325654057,10.9806828417891));
#72804=CARTESIAN_POINT('Ctrl Pts',(88.758114356599,53.0397782748239,11.0388543638781));
#72805=CARTESIAN_POINT('Ctrl Pts',(88.7722363912794,53.0380703642393,11.0492762890238));
#72806=CARTESIAN_POINT('Ctrl Pts',(88.7940887735301,53.0353679252044,11.06611363734));
#72807=CARTESIAN_POINT('Ctrl Pts',(88.8019671879608,53.0343810181749,11.0723342318931));
#72808=CARTESIAN_POINT('Ctrl Pts',(88.8166255014765,53.0325202257917,11.0841928440842));
#72809=CARTESIAN_POINT('Ctrl Pts',(88.8234220811331,53.0316472417752,11.0898093976243));
#72810=CARTESIAN_POINT('Ctrl Pts',(88.8386373397229,53.0296692076657,11.1026519242035));
#72811=CARTESIAN_POINT('Ctrl Pts',(88.8470207791278,53.0285625554123,11.1099182472026));
#72812=CARTESIAN_POINT('Ctrl Pts',(88.8685552350983,53.0256748717389,11.1290829718841));
#72813=CARTESIAN_POINT('Ctrl Pts',(88.8815535628568,53.0238870134857,11.1411481676868));
#72814=CARTESIAN_POINT('Ctrl Pts',(88.9124633002674,53.0195220834512,11.1710679673297));
#72815=CARTESIAN_POINT('Ctrl Pts',(88.9301014311276,53.0169341977256,11.1891922870389));
#72816=CARTESIAN_POINT('Ctrl Pts',(88.9916209429204,53.0075433220139,11.2563044355828));
#72817=CARTESIAN_POINT('Ctrl Pts',(89.0322184093449,53.0006319543569,11.3081510593211));
#72818=CARTESIAN_POINT('Ctrl Pts',(89.1041642543375,52.9869299370977,11.4163730820691));
#72819=CARTESIAN_POINT('Ctrl Pts',(89.1356115581439,52.9801598257506,11.4724730876544));
#72820=CARTESIAN_POINT('Ctrl Pts',(89.1680855505055,52.9722572636082,11.5423423466759));
#72821=CARTESIAN_POINT('Ctrl Pts',(89.1733123175282,52.9709503881399,11.5540484093683));
#72822=CARTESIAN_POINT('Ctrl Pts',(89.1808084034402,52.9690243505817,11.5715438260489));
#72823=CARTESIAN_POINT('Ctrl Pts',(89.1832136657773,52.9683978689227,11.5772733520239));
#72824=CARTESIAN_POINT('Ctrl Pts',(89.1874632619129,52.9672757671348,11.5876081126859));
#72825=CARTESIAN_POINT('Ctrl Pts',(89.1893227576895,52.966779298458,11.592206704995));
#72826=CARTESIAN_POINT('Ctrl Pts',(89.1934572169716,52.9656628608343,11.6026062676374));
#72827=CARTESIAN_POINT('Ctrl Pts',(89.1957164976753,52.9650438208894,11.6084132351972));
#72828=CARTESIAN_POINT('Ctrl Pts',(89.2025246358033,52.9631496103649,11.6263004921114));
#72829=CARTESIAN_POINT('Ctrl Pts',(89.2069323771307,52.9618822584453,11.6384343191065));
#72830=CARTESIAN_POINT('Ctrl Pts',(89.2169432469068,52.9588974548337,11.6673596396495));
#72831=CARTESIAN_POINT('Ctrl Pts',(89.2223820315127,52.9571877953838,11.684205655217));
#72832=CARTESIAN_POINT('Ctrl Pts',(89.2418856285817,52.9506762649702,11.7492356995046));
#72833=CARTESIAN_POINT('Ctrl Pts',(89.2534430343471,52.9459632329482,11.7981279600959));
#72834=CARTESIAN_POINT('Ctrl Pts',(89.2772681025976,52.9329794250132,11.9345948434656));
#72835=CARTESIAN_POINT('Ctrl Pts',(89.2833384199377,52.9247468114159,12.0229431818811));
#72836=CARTESIAN_POINT('Ctrl Pts',(89.2795847020413,52.9145602018262,12.1283485130167));
#72837=CARTESIAN_POINT('Ctrl Pts',(89.2786264699751,52.9128935361273,12.1454830166634));
#72838=CARTESIAN_POINT('Ctrl Pts',(89.2764902721414,52.9101480862054,12.173488603561));
#72839=CARTESIAN_POINT('Ctrl Pts',(89.2755185174059,52.9090757050422,12.1843736862948));
#72840=CARTESIAN_POINT('Ctrl Pts',(89.273510459982,52.9071313783768,12.2040030975057));
#72841=CARTESIAN_POINT('Ctrl Pts',(89.2725234395056,52.9062610283024,12.2127518933196));
#72842=CARTESIAN_POINT('Ctrl Pts',(89.2702023512373,52.9043806150649,12.2315673532507));
#72843=CARTESIAN_POINT('Ctrl Pts',(89.2688383586928,52.9033696695075,12.2416296041543));
#72844=CARTESIAN_POINT('Ctrl Pts',(89.2647059530782,52.9005447071138,12.2695913144076));
#72845=CARTESIAN_POINT('Ctrl Pts',(89.2616751975165,52.8987226067386,12.2874486474905));
#72846=CARTESIAN_POINT('Ctrl Pts',(89.2539937456106,52.8945928600967,12.3274964690376));
#72847=CARTESIAN_POINT('Ctrl Pts',(89.2491287026293,52.892279158034,12.3496388724209));
#72848=CARTESIAN_POINT('Ctrl Pts',(89.2306913532324,52.8844019954083,12.4239989880257));
#72849=CARTESIAN_POINT('Ctrl Pts',(89.2143872341998,52.8787654563511,12.4754727203919));
#72850=CARTESIAN_POINT('Ctrl Pts',(89.1648757976314,52.8643716092896,12.6029661035577));
#72851=CARTESIAN_POINT('Ctrl Pts',(89.1274025669483,52.8555840413405,12.6770729622982));
#72852=CARTESIAN_POINT('Ctrl Pts',(89.0766828758596,52.8458963161823,12.7569107348018));
#72853=CARTESIAN_POINT('Ctrl Pts',(89.0702546409967,52.8447014861323,12.7667262492174));
#72854=CARTESIAN_POINT('Ctrl Pts',(89.0602921451754,52.8429002529548,12.7814878802534));
#72855=CARTESIAN_POINT('Ctrl Pts',(89.0568571737377,52.8422879459457,12.7864996116957));
#72856=CARTESIAN_POINT('Ctrl Pts',(89.0508345918231,52.8412296338958,12.7951529152225));
#72857=CARTESIAN_POINT('Ctrl Pts',(89.0482636307569,52.8407825747008,12.7988056459588));
#72858=CARTESIAN_POINT('Ctrl Pts',(89.0421269240648,52.8397265336142,12.8074274532702));
#72859=CARTESIAN_POINT('Ctrl Pts',(89.0385444757098,52.8391186952639,12.8123844573347));
#72860=CARTESIAN_POINT('Ctrl Pts',(89.0276429985925,52.8372941490059,12.8272414742837));
#72861=CARTESIAN_POINT('Ctrl Pts',(89.0202153337361,52.8360844519654,12.8370616189461));
#72862=CARTESIAN_POINT('Ctrl Pts',(88.9823875275384,52.8300783294306,12.8855905255051));
#72863=CARTESIAN_POINT('Ctrl Pts',(88.9498934610293,52.8254036125229,12.9226230338728));
#72864=CARTESIAN_POINT('Ctrl Pts',(88.853791285557,52.8125125897115,13.0200880685693));
#72865=CARTESIAN_POINT('Ctrl Pts',(88.7859656525664,52.804400662786,13.0759547566736));
#72866=CARTESIAN_POINT('Ctrl Pts',(88.686067098715,52.7929676115575,13.1422078952438));
#72867=CARTESIAN_POINT('Ctrl Pts',(88.6585382890826,52.789866493102,13.1589925856943));
#72868=CARTESIAN_POINT('Ctrl Pts',(88.6191324948814,52.7854708056106,13.1810074223256));
#72869=CARTESIAN_POINT('Ctrl Pts',(88.607766703452,52.7842078810806,13.1871316404283));
#72870=CARTESIAN_POINT('Ctrl Pts',(88.5883279549346,52.7820547193353,13.1972264709698));
#72871=CARTESIAN_POINT('Ctrl Pts',(88.5803023389341,52.7811676829258,13.2012866301586));
#72872=CARTESIAN_POINT('Ctrl Pts',(88.563916170857,52.7793599788299,13.2093589531419));
#72873=CARTESIAN_POINT('Ctrl Pts',(88.5555534662902,52.7784391781227,13.2133654598325));
#72874=CARTESIAN_POINT('Ctrl Pts',(88.5345647854469,52.7761319350997,13.223139831433));
#72875=CARTESIAN_POINT('Ctrl Pts',(88.5218870900371,52.7747416667695,13.2287927656928));
#72876=CARTESIAN_POINT('Ctrl Pts',(88.4693883834337,52.768995601822,13.2511774899006));
#72877=CARTESIAN_POINT('Ctrl Pts',(88.4288248404821,52.764580372948,13.2660778717099));
#72878=CARTESIAN_POINT('Ctrl Pts',(88.313684937213,52.7520945759315,13.3018276019312));
#72879=CARTESIAN_POINT('Ctrl Pts',(88.2378473576537,52.7439134533325,13.3179686969941));
#72880=CARTESIAN_POINT('Ctrl Pts',(88.110910077758,52.7304611387984,13.3330694253974));
#72881=CARTESIAN_POINT('Ctrl Pts',(88.0604773065984,52.7251820375424,13.3360395713598));
#72882=CARTESIAN_POINT('Ctrl Pts',(88.0001483484465,52.7190241107554,13.335991806336));
#72883=CARTESIAN_POINT('Ctrl Pts',(87.9903020752933,52.7180241434539,13.3358695067524));
#72884=CARTESIAN_POINT('Ctrl Pts',(87.9748501246574,52.7164637481889,13.3354977941489));
#72885=CARTESIAN_POINT('Ctrl Pts',(87.969243327152,52.7158993880113,13.3353257452641));
#72886=CARTESIAN_POINT('Ctrl Pts',(87.9585929779854,52.7148310610893,13.3349282833395));
#72887=CARTESIAN_POINT('Ctrl Pts',(87.9535495675135,52.7143267663684,13.3347099487096));
#72888=CARTESIAN_POINT('Ctrl Pts',(87.9413788672194,52.7131134379033,13.3341103405441));
#72889=CARTESIAN_POINT('Ctrl Pts',(87.9342532101594,52.7124060534704,13.3336990482815));
#72890=CARTESIAN_POINT('Ctrl Pts',(87.9088621077425,52.7098947822123,13.3320185893685));
#72891=CARTESIAN_POINT('Ctrl Pts',(87.8906196938915,52.708107853037,13.3304144592637));
#72892=CARTESIAN_POINT('Ctrl Pts',(87.8568620913763,52.7048219610243,13.3267086760515));
#72893=CARTESIAN_POINT('Ctrl Pts',(87.8413394460499,52.703319233422,13.3247137149969));
#72894=CARTESIAN_POINT('Ctrl Pts',(87.7576549415357,52.6952419761042,13.3123822712204));
#72895=CARTESIAN_POINT('Ctrl Pts',(87.6903785885725,52.6888304194108,13.2967949164672));
#72896=CARTESIAN_POINT('Ctrl Pts',(87.5586013782521,52.6758550212628,13.2547174752188));
#72897=CARTESIAN_POINT('Ctrl Pts',(87.4943593346212,52.6693112279041,13.2282364520719));
#72898=CARTESIAN_POINT('Ctrl Pts',(87.4186656291913,52.6610687245653,13.1895146846946));
#72899=CARTESIAN_POINT('Ctrl Pts',(87.4048573173293,52.6595424937634,13.1821255530731));
#72900=CARTESIAN_POINT('Ctrl Pts',(87.3826525252733,52.6570484483686,13.1697097105431));
#72901=CARTESIAN_POINT('Ctrl Pts',(87.3741709190312,52.6560861534063,13.1648377416535));
#72902=CARTESIAN_POINT('Ctrl Pts',(87.3585851005065,52.6542992563279,13.1556439483817));
#72903=CARTESIAN_POINT('Ctrl Pts',(87.3514653592732,52.6534756785054,13.1513493376085));
#72904=CARTESIAN_POINT('Ctrl Pts',(87.3371111111189,52.6517999688757,13.1424974992895));
#72905=CARTESIAN_POINT('Ctrl Pts',(87.329879447325,52.6509477332218,13.1379365112114));
#72906=CARTESIAN_POINT('Ctrl Pts',(87.3134618915067,52.6489941427409,13.1273488035069));
#72907=CARTESIAN_POINT('Ctrl Pts',(87.3043072047548,52.6478911000812,13.1212753049212));
#72908=CARTESIAN_POINT('Ctrl Pts',(87.255383607329,52.6419203044738,13.0878958009803));
#72909=CARTESIAN_POINT('Ctrl Pts',(87.2171260935039,52.6369746254133,13.0584661740469));
#72910=CARTESIAN_POINT('Ctrl Pts',(87.1806428293121,52.6319631729084,13.0269406688694));
#72911=CARTESIAN_POINT('Origin',(88.011,66.41344859951,12.066));
#72912=CARTESIAN_POINT('',(87.1806428357067,51.6672833294972,13.026940674395));
#72913=CARTESIAN_POINT('',(87.1792973239246,51.8375066538898,13.0285052387874));
#72914=CARTESIAN_POINT('',(87.1806428354228,66.41344859951,13.0269406741497));
#72915=CARTESIAN_POINT('',(86.7410001453939,52.3539891800374,12.0650476267737));
#72916=CARTESIAN_POINT('Ctrl Pts',(87.1806428357067,51.6672833294972,13.026940674395));
#72917=CARTESIAN_POINT('Ctrl Pts',(87.1817392149757,51.6674344362791,13.0278880652227));
#72918=CARTESIAN_POINT('Ctrl Pts',(87.1828372304032,51.6675855942185,13.0288335924603));
#72919=CARTESIAN_POINT('Ctrl Pts',(87.2213438210188,51.6728804841237,13.0618779302639));
#72920=CARTESIAN_POINT('Ctrl Pts',(87.2605856494101,51.6780774533418,13.0917716257743));
#72921=CARTESIAN_POINT('Ctrl Pts',(87.3535931839974,51.6898996608408,13.1544241286476));
#72922=CARTESIAN_POINT('Ctrl Pts',(87.4082672543514,51.6965107849232,13.1856278242971));
#72923=CARTESIAN_POINT('Ctrl Pts',(87.4739873489515,51.7039430767255,13.2169195082281));
#72924=CARTESIAN_POINT('Ctrl Pts',(87.4829892692356,51.7049503422229,13.2210770503001));
#72925=CARTESIAN_POINT('Ctrl Pts',(87.4972249153891,51.7065254537571,13.2274505763393));
#72926=CARTESIAN_POINT('Ctrl Pts',(87.5024260803381,51.7070972484085,13.2297374496546));
#72927=CARTESIAN_POINT('Ctrl Pts',(87.5122573403788,51.7081709014651,13.2339816026196));
#72928=CARTESIAN_POINT('Ctrl Pts',(87.5168837642477,51.7086731525451,13.2359463287323));
#72929=CARTESIAN_POINT('Ctrl Pts',(87.5279705418267,51.7098698347381,13.2405771072161));
#72930=CARTESIAN_POINT('Ctrl Pts',(87.5344414706581,51.7105627350852,13.2432174033289));
#72931=CARTESIAN_POINT('Ctrl Pts',(87.5570221378625,51.712962567406,13.2522141505839));
#72932=CARTESIAN_POINT('Ctrl Pts',(87.573241005222,51.7146544656587,13.2582948797009));
#72933=CARTESIAN_POINT('Ctrl Pts',(87.6146089505715,51.7189030076769,13.2728463288263));
#72934=CARTESIAN_POINT('Ctrl Pts',(87.6399094313916,51.7214399748708,13.2808645944262));
#72935=CARTESIAN_POINT('Ctrl Pts',(87.7214345733798,51.7294789526008,13.3039165351732));
#72936=CARTESIAN_POINT('Ctrl Pts',(87.7784492768445,51.7349007854946,13.3158825738163));
#72937=CARTESIAN_POINT('Ctrl Pts',(87.9062412190162,51.7470004134378,13.3336523343811));
#72938=CARTESIAN_POINT('Ctrl Pts',(87.9770770967976,51.7536772256821,13.3375200956158));
#72939=CARTESIAN_POINT('Ctrl Pts',(88.0637009184863,51.7620798466425,13.3350050560877));
#72940=CARTESIAN_POINT('Ctrl Pts',(88.0795332609607,51.7636248911654,13.334248539426));
#72941=CARTESIAN_POINT('Ctrl Pts',(88.1050081914213,51.7661286509612,13.3325528896491));
#72942=CARTESIAN_POINT('Ctrl Pts',(88.1146618962562,51.7670815527957,13.3317993366585));
#72943=CARTESIAN_POINT('Ctrl Pts',(88.1331645870808,51.7689164368705,13.3301419710605));
#72944=CARTESIAN_POINT('Ctrl Pts',(88.1420145876308,51.7697978256503,13.3292554282161));
#72945=CARTESIAN_POINT('Ctrl Pts',(88.1625342767225,51.7718506439428,13.3269819429118));
#72946=CARTESIAN_POINT('Ctrl Pts',(88.1741952464939,51.7730241716353,13.3255258572246));
#72947=CARTESIAN_POINT('Ctrl Pts',(88.2122951475645,51.7768826095321,13.3202304376413));
#72948=CARTESIAN_POINT('Ctrl Pts',(88.2386311296509,51.7795881173133,13.315718977328));
#72949=CARTESIAN_POINT('Ctrl Pts',(88.3024759949519,51.7862485109085,13.3026972344534));
#72950=CARTESIAN_POINT('Ctrl Pts',(88.3397761485748,51.7902270454978,13.2933075706572));
#72951=CARTESIAN_POINT('Ctrl Pts',(88.4229203949389,51.7992927949267,13.2683153262318));
#72952=CARTESIAN_POINT('Ctrl Pts',(88.4684155811112,51.804394462812,13.2517533452652));
#72953=CARTESIAN_POINT('Ctrl Pts',(88.5700267689911,51.8160551147531,13.2080433012511));
#72954=CARTESIAN_POINT('Ctrl Pts',(88.6253249693706,51.8225997333426,13.1792749187157));
#72955=CARTESIAN_POINT('Ctrl Pts',(88.6868133522788,51.8299785158323,13.1413029767386));
#72956=CARTESIAN_POINT('Ctrl Pts',(88.6952673438125,51.8309952606904,13.1359431778764));
#72957=CARTESIAN_POINT('Ctrl Pts',(88.7083888441128,51.8325759297479,13.1274050420334));
#72958=CARTESIAN_POINT('Ctrl Pts',(88.713099726916,51.8331439482561,13.1242947799039));
#72959=CARTESIAN_POINT('Ctrl Pts',(88.7219752823662,51.8342149117723,13.118349526282));
#72960=CARTESIAN_POINT('Ctrl Pts',(88.7261438787201,51.8347182162491,13.1155211347422));
#72961=CARTESIAN_POINT('Ctrl Pts',(88.7361175492315,51.8359233741614,13.1086669840792));
#72962=CARTESIAN_POINT('Ctrl Pts',(88.7419060867106,51.8366236369168,13.1046174468439));
#72963=CARTESIAN_POINT('Ctrl Pts',(88.7621708584317,51.8390792589787,13.0901873075785));
#72964=CARTESIAN_POINT('Ctrl Pts',(88.7764632817917,51.8408186378754,13.0795498901577));
#72965=CARTESIAN_POINT('Ctrl Pts',(88.8024023463741,51.843999787252,13.0593823757239));
#72966=CARTESIAN_POINT('Ctrl Pts',(88.8141120330593,51.8454454321576,13.0499397004182));
#72967=CARTESIAN_POINT('Ctrl Pts',(88.8748140165075,51.8530082505001,12.9991838161022));
#72968=CARTESIAN_POINT('Ctrl Pts',(88.9207990569598,51.8589815816981,12.9544109119908));
#72969=CARTESIAN_POINT('Ctrl Pts',(89.0091377830331,51.8714932992909,12.854313642337));
#72970=CARTESIAN_POINT('Ctrl Pts',(89.0507144980876,51.8780183416019,12.798604190185));
#72971=CARTESIAN_POINT('Ctrl Pts',(89.0967978004155,51.8864042547085,12.7249752222019));
#72972=CARTESIAN_POINT('Ctrl Pts',(89.1057592992095,51.8881004701978,12.7099776503915));
#72973=CARTESIAN_POINT('Ctrl Pts',(89.1198640045623,51.8908845307619,12.6852269738495));
#72974=CARTESIAN_POINT('Ctrl Pts',(89.1251948337624,51.8919656596498,12.6755828732984));
#72975=CARTESIAN_POINT('Ctrl Pts',(89.1345618343001,51.8939195037024,12.6581034254008));
#72976=CARTESIAN_POINT('Ctrl Pts',(89.1386432734137,51.8947905554241,12.6502929914847));
#72977=CARTESIAN_POINT('Ctrl Pts',(89.1472240298164,51.8966654537922,12.6334476363894));
#72978=CARTESIAN_POINT('Ctrl Pts',(89.1516975435629,51.8976701320607,12.6244003626394));
#72979=CARTESIAN_POINT('Ctrl Pts',(89.1637648405395,51.9004580846247,12.5992451039592));
#72980=CARTESIAN_POINT('Ctrl Pts',(89.1711280119999,51.9022490949957,12.5830300103371));
#72981=CARTESIAN_POINT('Ctrl Pts',(89.2068749783876,51.9114287868335,12.4996971376571));
#72982=CARTESIAN_POINT('Ctrl Pts',(89.2297789064264,51.9189941700965,12.4303948988274));
#72983=CARTESIAN_POINT('Ctrl Pts',(89.2653190483963,51.935161767403,12.2807872587821));
#72984=CARTESIAN_POINT('Ctrl Pts',(89.276456050109,51.9437521262372,12.2004349617768));
#72985=CARTESIAN_POINT('Ctrl Pts',(89.2805289953162,51.9536989766017,12.1039514713849));
#72986=CARTESIAN_POINT('Ctrl Pts',(89.2808999066288,51.9552978033713,12.0883268779407));
#72987=CARTESIAN_POINT('Ctrl Pts',(89.2810153078521,51.9575168102198,12.0664467473331));
#72988=CARTESIAN_POINT('Ctrl Pts',(89.2810021214388,51.9581485716723,12.0601948973341));
#72989=CARTESIAN_POINT('Ctrl Pts',(89.2808948176609,51.959286291433,12.048892622697));
#72990=CARTESIAN_POINT('Ctrl Pts',(89.2808167375596,51.959793090378,12.0438422031532));
#72991=CARTESIAN_POINT('Ctrl Pts',(89.2805912850935,51.9608454063165,12.0333210223533));
#72992=CARTESIAN_POINT('Ctrl Pts',(89.2804386828509,51.9613906324065,12.0278505381235));
#72993=CARTESIAN_POINT('Ctrl Pts',(89.2799344176376,51.962848356043,12.0131771325673));
#72994=CARTESIAN_POINT('Ctrl Pts',(89.2795179978313,51.9637574004397,12.0039764644561));
#72995=CARTESIAN_POINT('Ctrl Pts',(89.2767486519361,51.9686063171211,11.9546705563998));
#72996=CARTESIAN_POINT('Ctrl Pts',(89.2725935187751,51.972458744986,11.9146833579683));
#72997=CARTESIAN_POINT('Ctrl Pts',(89.2581369648283,51.9815722209583,11.8196751289201));
#72998=CARTESIAN_POINT('Ctrl Pts',(89.2460835817811,51.9867853967364,11.7650086279144));
#72999=CARTESIAN_POINT('Ctrl Pts',(89.2103850981192,51.998770218907,11.6422724191995));
#73000=CARTESIAN_POINT('Ctrl Pts',(89.1844816080507,52.0055438242668,11.5750745540258));
#73001=CARTESIAN_POINT('Ctrl Pts',(89.146057339155,52.0140592987613,11.4960882375117));
#73002=CARTESIAN_POINT('Ctrl Pts',(89.1388081664462,52.0156144717272,11.4818739303158));
#73003=CARTESIAN_POINT('Ctrl Pts',(89.12672209458,52.0181305935031,11.4592394202074));
#73004=CARTESIAN_POINT('Ctrl Pts',(89.1220528317171,52.0190856223875,11.4507311273435));
#73005=CARTESIAN_POINT('Ctrl Pts',(89.1129218042035,52.0209219322914,11.4345355698235));
#73006=CARTESIAN_POINT('Ctrl Pts',(89.1084759294346,52.0218025995724,11.4268399549019));
#73007=CARTESIAN_POINT('Ctrl Pts',(89.0979897575588,52.023849746178,11.4091208523541));
#73008=CARTESIAN_POINT('Ctrl Pts',(89.0918910682549,52.0250182862934,11.3991331297484));
#73009=CARTESIAN_POINT('Ctrl Pts',(89.0715776151549,52.0288415853856,11.3668769521485));
#73010=CARTESIAN_POINT('Ctrl Pts',(89.0568070661922,52.031516420849,11.3449693284727));
#73011=CARTESIAN_POINT('Ctrl Pts',(89.0192456406346,52.0380820025928,11.2928426036675));
#73012=CARTESIAN_POINT('Ctrl Pts',(88.9957675525294,52.04199549108,11.2631526609964));
#73013=CARTESIAN_POINT('Ctrl Pts',(88.938912261982,52.0510598404315,11.1975062318521));
#73014=CARTESIAN_POINT('Ctrl Pts',(88.9047061400356,52.0562280683231,11.1623455640425));
#73015=CARTESIAN_POINT('Ctrl Pts',(88.8223671330295,52.0679963130974,11.0869674223922));
#73016=CARTESIAN_POINT('Ctrl Pts',(88.7731064762636,52.0745821144528,11.0481505325354));
#73017=CARTESIAN_POINT('Ctrl Pts',(88.7128667057587,52.0820013128468,11.0075182732179));
#73018=CARTESIAN_POINT('Ctrl Pts',(88.7044916479797,52.0830193939742,11.0020123141498));
#73019=CARTESIAN_POINT('Ctrl Pts',(88.6912963709355,52.0846016706885,10.9935594459112));
#73020=CARTESIAN_POINT('Ctrl Pts',(88.6865204887862,52.0851699736504,10.9905447623639));
#73021=CARTESIAN_POINT('Ctrl Pts',(88.6774474793814,52.0862411351503,10.9849018888959));
#73022=CARTESIAN_POINT('Ctrl Pts',(88.6731547776891,52.0867443556721,10.9822673664916));
#73023=CARTESIAN_POINT('Ctrl Pts',(88.6628088303405,52.087948854134,10.9760022633703));
#73024=CARTESIAN_POINT('Ctrl Pts',(88.6567407659716,52.0886485460433,10.9723964663112));
#73025=CARTESIAN_POINT('Ctrl Pts',(88.6352875561016,52.09109980242,10.9598892612214));
#73026=CARTESIAN_POINT('Ctrl Pts',(88.6197447734738,52.09283546166,10.9512597453841));
#73027=CARTESIAN_POINT('Ctrl Pts',(88.5907659230636,52.0960084694772,10.9359573979586));
#73028=CARTESIAN_POINT('Ctrl Pts',(88.5773835830163,52.0974496997681,10.929191089982));
#73029=CARTESIAN_POINT('Ctrl Pts',(88.5065152751818,52.1049742345317,10.8949212841805));
#73030=CARTESIAN_POINT('Ctrl Pts',(88.4471346030256,52.1109150771811,10.8715340416709));
#73031=CARTESIAN_POINT('Ctrl Pts',(88.3194247811908,52.1234425699354,10.8320364591742));
#73032=CARTESIAN_POINT('Ctrl Pts',(88.2510227557726,52.1300165013664,10.8169289013674));
#73033=CARTESIAN_POINT('Ctrl Pts',(88.1644602816992,52.1384505340385,10.8051852809591));
#73034=CARTESIAN_POINT('Ctrl Pts',(88.1471428636284,52.1401429410943,10.8031980101817));
#73035=CARTESIAN_POINT('Ctrl Pts',(88.1188314603923,52.1429220431208,10.8005382077332));
#73036=CARTESIAN_POINT('Ctrl Pts',(88.1078594361391,52.1440020627525,10.7996511529323));
#73037=CARTESIAN_POINT('Ctrl Pts',(88.0880861390598,52.1459547162005,10.7983110107467));
#73038=CARTESIAN_POINT('Ctrl Pts',(88.0792889162113,52.1468256953351,10.7978066944111));
#73039=CARTESIAN_POINT('Ctrl Pts',(88.0603975765138,52.1487013382048,10.7969208422943));
#73040=CARTESIAN_POINT('Ctrl Pts',(88.0503028159967,52.1497068400885,10.7965681181659));
#73041=CARTESIAN_POINT('Ctrl Pts',(88.0223631474586,52.15249956369,10.7959254394335));
#73042=CARTESIAN_POINT('Ctrl Pts',(88.0045155495054,52.1542945656077,10.7958911939459));
#73043=CARTESIAN_POINT('Ctrl Pts',(87.9142136112086,52.1634384733453,10.7976211637886));
#73044=CARTESIAN_POINT('Ctrl Pts',(87.8420212708799,52.1709618813644,10.8052088877695));
#73045=CARTESIAN_POINT('Ctrl Pts',(87.6920222529483,52.1870212600025,10.8340896915308));
#73046=CARTESIAN_POINT('Ctrl Pts',(87.6147735663741,52.1955454771024,10.8567207812351));
#73047=CARTESIAN_POINT('Ctrl Pts',(87.5250498300873,52.205504249235,10.8925360407141));
#73048=CARTESIAN_POINT('Ctrl Pts',(87.5100406801162,52.207171636112,10.8988645841986));
#73049=CARTESIAN_POINT('Ctrl Pts',(87.4893461591826,52.2094691105509,10.9080631723716));
#73050=CARTESIAN_POINT('Ctrl Pts',(87.4835553417364,52.2101118295174,10.9106894075234));
#73051=CARTESIAN_POINT('Ctrl Pts',(87.4731759129027,52.2112632429076,10.9154909678409));
#73052=CARTESIAN_POINT('Ctrl Pts',(87.4685801877,52.2117728438773,10.9176505176821));
#73053=CARTESIAN_POINT('Ctrl Pts',(87.459201349554,52.2128122315539,10.9221265412529));
#73054=CARTESIAN_POINT('Ctrl Pts',(87.4544196264119,52.2133418568133,10.9244455633442));
#73055=CARTESIAN_POINT('Ctrl Pts',(87.4419250183301,52.2147253718586,10.9306023265188));
#73056=CARTESIAN_POINT('Ctrl Pts',(87.4342361501195,52.2155763581498,10.9344887591395));
#73057=CARTESIAN_POINT('Ctrl Pts',(87.4171542118176,52.2174674879111,10.9433424114163));
#73058=CARTESIAN_POINT('Ctrl Pts',(87.4077825917064,52.2185053836489,10.9483499365597));
#73059=CARTESIAN_POINT('Ctrl Pts',(87.3790508385487,52.2216922329338,10.9641688441136));
#73060=CARTESIAN_POINT('Ctrl Pts',(87.3599089406063,52.2238222973051,10.9753707125273));
#73061=CARTESIAN_POINT('Ctrl Pts',(87.2741762101353,52.2334431137692,11.0286040078826));
#73062=CARTESIAN_POINT('Ctrl Pts',(87.2112866374828,52.2407364630698,11.0762726531749));
#73063=CARTESIAN_POINT('Ctrl Pts',(87.1101825432368,52.2536335600202,11.1688751991031));
#73064=CARTESIAN_POINT('Ctrl Pts',(87.0699257814049,52.2591677577206,11.2112003035933));
#73065=CARTESIAN_POINT('Ctrl Pts',(87.0228737148715,52.2663259016114,11.2680369056587));
#73066=CARTESIAN_POINT('Ctrl Pts',(87.013240899309,52.2678324615083,11.2801149050149));
#73067=CARTESIAN_POINT('Ctrl Pts',(86.9979841374338,52.2702892673875,11.2999771567767));
#73068=CARTESIAN_POINT('Ctrl Pts',(86.992223699199,52.2712340975289,11.307655111123));
#73069=CARTESIAN_POINT('Ctrl Pts',(86.9812771966769,52.2730638955885,11.3225952839969));
#73070=CARTESIAN_POINT('Ctrl Pts',(86.9760795392654,52.2739483488278,11.3298483491408));
#73071=CARTESIAN_POINT('Ctrl Pts',(86.9641005325154,52.2760243390254,11.3469420593605));
#73072=CARTESIAN_POINT('Ctrl Pts',(86.9573809473203,52.2772181268517,11.3568246452856));
#73073=CARTESIAN_POINT('Ctrl Pts',(86.9357029531295,52.2811692641687,11.3896950240199));
#73074=CARTESIAN_POINT('Ctrl Pts',(86.921350949421,52.2839483983011,11.4130705927901));
#73075=CARTESIAN_POINT('Ctrl Pts',(86.8698084939175,52.2945927301042,11.5034574774526));
#73076=CARTESIAN_POINT('Ctrl Pts',(86.8379586335781,52.3026265416557,11.5733116096807));
#73077=CARTESIAN_POINT('Ctrl Pts',(86.7942977908676,52.316532262508,11.6977704280845));
#73078=CARTESIAN_POINT('Ctrl Pts',(86.7794197358012,52.3223659474705,11.7510898798021));
#73079=CARTESIAN_POINT('Ctrl Pts',(86.7638460209407,52.3302189440268,11.8253158809965));
#73080=CARTESIAN_POINT('Ctrl Pts',(86.7601161365846,52.3323294997758,11.845519574348));
#73081=CARTESIAN_POINT('Ctrl Pts',(86.7556706550292,52.335194929833,11.8733685560581));
#73082=CARTESIAN_POINT('Ctrl Pts',(86.7545319422459,52.3359696994726,11.8809414468146));
#73083=CARTESIAN_POINT('Ctrl Pts',(86.7527503274679,52.3372534279904,11.8935654368501));
#73084=CARTESIAN_POINT('Ctrl Pts',(86.7520691931819,52.3377644162333,11.8986107973947));
#73085=CARTESIAN_POINT('Ctrl Pts',(86.7508275297589,52.3387360334251,11.9082447740154));
#73086=CARTESIAN_POINT('Ctrl Pts',(86.7502616868218,52.3391969666742,11.9128325285457));
#73087=CARTESIAN_POINT('Ctrl Pts',(86.7490890935347,52.3401934796134,11.9227867709244));
#73088=CARTESIAN_POINT('Ctrl Pts',(86.7484914940307,52.3407285578998,11.9281542854903));
#73089=CARTESIAN_POINT('Ctrl Pts',(86.7471097786466,52.3420366875703,11.9413281979347));
#73090=CARTESIAN_POINT('Ctrl Pts',(86.7463637057939,52.3428077976718,11.9491385266829));
#73091=CARTESIAN_POINT('Ctrl Pts',(86.7425923982012,52.3471061903767,11.992899355873));
#73092=CARTESIAN_POINT('Ctrl Pts',(86.7410273681016,52.3505653341981,12.0289633647895));
#73093=CARTESIAN_POINT('Ctrl Pts',(86.7410003558112,52.3539897096227,12.0650493369797));
#73094=CARTESIAN_POINT('Ctrl Pts',(86.7410003571183,52.3539895440703,12.0650475923927));
#73095=CARTESIAN_POINT('Ctrl Pts',(86.7409228830868,52.3637930183023,12.1683562929114));
#73096=CARTESIAN_POINT('Ctrl Pts',(86.753450462588,52.373289701593,12.2712934287686));
#73097=CARTESIAN_POINT('Ctrl Pts',(86.7836604081648,52.3852655112793,12.3931567335967));
#73098=CARTESIAN_POINT('Ctrl Pts',(86.7895734438675,52.3873983575918,12.4145843449426));
#73099=CARTESIAN_POINT('Ctrl Pts',(86.7997968819516,52.3907937032765,12.4481687713019));
#73100=CARTESIAN_POINT('Ctrl Pts',(86.8037356630307,52.3920449995578,12.4604347292532));
#73101=CARTESIAN_POINT('Ctrl Pts',(86.8116063344157,52.3944439929493,12.4837220629807));
#73102=CARTESIAN_POINT('Ctrl Pts',(86.8155053163813,52.3955905420546,12.4947532228195));
#73103=CARTESIAN_POINT('Ctrl Pts',(86.8226331246346,52.3976169116452,12.5140660134888));
#73104=CARTESIAN_POINT('Ctrl Pts',(86.8257975972196,52.3984945500352,12.5223707234641));
#73105=CARTESIAN_POINT('Ctrl Pts',(86.8326000892366,52.4003369262407,12.5396748536933));
#73106=CARTESIAN_POINT('Ctrl Pts',(86.8362546314832,52.4013021676833,12.5486670927795));
#73107=CARTESIAN_POINT('Ctrl Pts',(86.8461903537524,52.4038640355043,12.5723331414491));
#73108=CARTESIAN_POINT('Ctrl Pts',(86.8526454676223,52.4054664308222,12.586931358009));
#73109=CARTESIAN_POINT('Ctrl Pts',(86.8897303060332,52.4143501938584,12.6666990502503));
#73110=CARTESIAN_POINT('Ctrl Pts',(86.925577989438,52.4218077958084,12.7292794558702));
#73111=CARTESIAN_POINT('Ctrl Pts',(86.9962646864695,52.4348574983519,12.831470748392));
#73112=CARTESIAN_POINT('Ctrl Pts',(87.0286317927001,52.4403866717277,12.8725890138752));
#73113=CARTESIAN_POINT('Ctrl Pts',(87.0829805272465,52.4489575970268,12.9334912719663));
#73114=CARTESIAN_POINT('Ctrl Pts',(87.1032752829178,52.4520235824041,12.9547054532518));
#73115=CARTESIAN_POINT('Ctrl Pts',(87.1334325348802,52.4563751143607,12.9841168135056));
#73116=CARTESIAN_POINT('Ctrl Pts',(87.1427110633365,52.4576878722564,12.992896704501));
#73117=CARTESIAN_POINT('Ctrl Pts',(87.1592318409866,52.4599780164577,13.0080637897263));
#73118=CARTESIAN_POINT('Ctrl Pts',(87.1664172467258,52.460958909738,13.0145110299053));
#73119=CARTESIAN_POINT('Ctrl Pts',(87.1759907852523,52.4622452888258,13.022905998961));
#73120=CARTESIAN_POINT('Ctrl Pts',(87.1783131263503,52.4625557707564,13.0249275523496));
#73121=CARTESIAN_POINT('Ctrl Pts',(87.1806428354249,52.4628656574377,13.0269406741515));
#73122=CARTESIAN_POINT('',(86.7429214405097,52.5228781632973,12.0657516006032));
#73123=CARTESIAN_POINT('Ctrl Pts',(87.1806428293121,52.6319631729084,13.0269406688694));
#73124=CARTESIAN_POINT('Ctrl Pts',(87.1768365540776,52.6314403313266,13.0236516334097));
#73125=CARTESIAN_POINT('Ctrl Pts',(87.1730495891386,52.630916799465,13.0203397830469));
#73126=CARTESIAN_POINT('Ctrl Pts',(87.1308342248737,52.6250431480985,12.9829757150102));
#73127=CARTESIAN_POINT('Ctrl Pts',(87.0944880664598,52.6196322981951,12.9466482670422));
#73128=CARTESIAN_POINT('Ctrl Pts',(87.0209437915815,52.6079403163833,12.8636441858104));
#73129=CARTESIAN_POINT('Ctrl Pts',(86.98462435003,52.6016712815446,12.8163348878005));
#73130=CARTESIAN_POINT('Ctrl Pts',(86.9446491424354,52.594238554194,12.7558998571834));
#73131=CARTESIAN_POINT('Ctrl Pts',(86.9377052946905,52.5929250144058,12.7450467481082));
#73132=CARTESIAN_POINT('Ctrl Pts',(86.927652198721,52.5909911353728,12.7287943141345));
#73133=CARTESIAN_POINT('Ctrl Pts',(86.9244159069601,52.5903633933194,12.723475304578));
#73134=CARTESIAN_POINT('Ctrl Pts',(86.9186716855218,52.5892400262526,12.7138761129677));
#73135=CARTESIAN_POINT('Ctrl Pts',(86.9161495931388,52.5887435426158,12.7096048432044));
#73136=CARTESIAN_POINT('Ctrl Pts',(86.9105220974512,52.5876282991705,12.699945623841));
#73137=CARTESIAN_POINT('Ctrl Pts',(86.9074311557749,52.5870104583669,12.6945495048389));
#73138=CARTESIAN_POINT('Ctrl Pts',(86.8980782401371,52.5851237809178,12.6779396266779));
#73139=CARTESIAN_POINT('Ctrl Pts',(86.8919463018392,52.5838626734678,12.6666528260402));
#73140=CARTESIAN_POINT('Ctrl Pts',(86.8692734898747,52.5790971678405,12.6233669873468));
#73141=CARTESIAN_POINT('Ctrl Pts',(86.853923441756,52.575652527841,12.5907589113411));
#73142=CARTESIAN_POINT('Ctrl Pts',(86.8107868934517,52.5650951835039,12.4879920767538));
#73143=CARTESIAN_POINT('Ctrl Pts',(86.787847405811,52.5581052351373,12.4159820225771));
#73144=CARTESIAN_POINT('Ctrl Pts',(86.7652123732216,52.5482976246684,12.3144562090411));
#73145=CARTESIAN_POINT('Ctrl Pts',(86.759935714398,52.5455886786553,12.2863525667403));
#73146=CARTESIAN_POINT('Ctrl Pts',(86.7511806298997,52.5400552375633,12.2291363832637));
#73147=CARTESIAN_POINT('Ctrl Pts',(86.7477530677977,52.5372312723383,12.2000343623896));
#73148=CARTESIAN_POINT('Ctrl Pts',(86.7443272794877,52.5331868979984,12.1586779702516));
#73149=CARTESIAN_POINT('Ctrl Pts',(86.743495099411,52.5319922188989,12.1465002415837));
#73150=CARTESIAN_POINT('Ctrl Pts',(86.7423624342434,52.5299216426699,12.1254734381258));
#73151=CARTESIAN_POINT('Ctrl Pts',(86.7419787213059,52.5290483877225,12.1166295106733));
#73152=CARTESIAN_POINT('Ctrl Pts',(86.7414406201416,52.5274294647725,12.1002825387802));
#73153=CARTESIAN_POINT('Ctrl Pts',(86.741260223201,52.526684646562,12.0927806738322));
#73154=CARTESIAN_POINT('Ctrl Pts',(86.7410469714205,52.525286242958,12.0787335420508));
#73155=CARTESIAN_POINT('Ctrl Pts',(86.7409982154571,52.5246331820998,12.0721887397098));
#73156=CARTESIAN_POINT('Ctrl Pts',(86.7410000498879,52.5239785351125,12.0656440290264));
#73157=CARTESIAN_POINT('Ctrl Pts',(86.7430172856975,52.522823273187,12.0657569666219));
#73158=CARTESIAN_POINT('Ctrl Pts',(86.7426850306966,52.5032787808449,11.8685299954553));
#73159=CARTESIAN_POINT('Ctrl Pts',(86.8788243097244,52.4417295403419,11.2478608714619));
#73160=CARTESIAN_POINT('Ctrl Pts',(87.847476062713,52.3381755516775,10.5738635505768));
#73161=CARTESIAN_POINT('Ctrl Pts',(89.175880239728,52.2121613071944,11.1192871132785));
#73162=CARTESIAN_POINT('Ctrl Pts',(89.4381831401015,52.086147062711,12.5311446533891));
#73163=CARTESIAN_POINT('Ctrl Pts',(88.4036797289598,51.9612621782764,13.5084625635155));
#73164=CARTESIAN_POINT('Ctrl Pts',(87.489495448972,51.8783820420025,13.2952201808301));
#73165=CARTESIAN_POINT('Ctrl Pts',(87.1792973239246,51.8375066538898,13.0285052387874));
#73166=CARTESIAN_POINT('Origin',(88.011,66.41344859951,12.066));
#73167=CARTESIAN_POINT('',(87.1806428354228,50.8732662532979,13.0269406741497));
#73168=CARTESIAN_POINT('',(87.1806428354228,51.0436650276944,13.0269406741497));
#73169=CARTESIAN_POINT('',(87.1806428354228,66.41344859951,13.0269406741497));
#73170=CARTESIAN_POINT('Ctrl Pts',(87.1806428354228,50.8732662532979,13.0269406741497));
#73171=CARTESIAN_POINT('Ctrl Pts',(87.1806475183611,50.8732668464107,13.0269447207173));
#73172=CARTESIAN_POINT('Ctrl Pts',(87.1806522013294,50.8732674395246,13.026948767251));
#73173=CARTESIAN_POINT('Ctrl Pts',(87.2010075773433,50.8758455061281,13.0445375042818));
#73174=CARTESIAN_POINT('Ctrl Pts',(87.2219099279938,50.8784434310677,13.0614697333693));
#73175=CARTESIAN_POINT('Ctrl Pts',(87.2507103336188,50.8819711428578,13.0833226623144));
#73176=CARTESIAN_POINT('Ctrl Pts',(87.2581491587513,50.8828778254497,13.0888398583794));
#73177=CARTESIAN_POINT('Ctrl Pts',(87.2668241774468,50.8839304024496,13.0951280082915));
#73178=CARTESIAN_POINT('Ctrl Pts',(87.2680023887985,50.8840732588447,13.0959789619348));
#73179=CARTESIAN_POINT('Ctrl Pts',(87.2704084295926,50.8843647843292,13.0977104287168));
#73180=CARTESIAN_POINT('Ctrl Pts',(87.2716363743223,50.8845134593419,13.0985907765699));
#73181=CARTESIAN_POINT('Ctrl Pts',(87.2731954855051,50.884702096019,13.0997043399589));
#73182=CARTESIAN_POINT('Ctrl Pts',(87.2735252026008,50.8847419808244,13.0999395955563));
#73183=CARTESIAN_POINT('Ctrl Pts',(87.2808501879476,50.885627891699,13.1051607406175));
#73184=CARTESIAN_POINT('Ctrl Pts',(87.2878955312112,50.8864765664898,13.1100755293309));
#73185=CARTESIAN_POINT('Ctrl Pts',(87.3029034585386,50.8882776862816,13.1203202035269));
#73186=CARTESIAN_POINT('Ctrl Pts',(87.3108775370951,50.8892307410921,13.1256321661932));
#73187=CARTESIAN_POINT('Ctrl Pts',(87.3320137441215,50.8917473486438,13.1393694052747));
#73188=CARTESIAN_POINT('Ctrl Pts',(87.3452721031549,50.8933163782212,13.1476425135847));
#73189=CARTESIAN_POINT('Ctrl Pts',(87.4189506169962,50.9019883013449,13.1917495479482));
#73190=CARTESIAN_POINT('Ctrl Pts',(87.4820978118385,50.9092586344217,13.2227596055896));
#73191=CARTESIAN_POINT('Ctrl Pts',(87.6020667138533,50.9227845607846,13.2697908767773));
#73192=CARTESIAN_POINT('Ctrl Pts',(87.6580793731078,50.928991823158,13.2873868573782));
#73193=CARTESIAN_POINT('Ctrl Pts',(87.7408897635774,50.9379182683555,13.3072265563895));
#73194=CARTESIAN_POINT('Ctrl Pts',(87.7668618326338,50.9406824759937,13.3125952419291));
#73195=CARTESIAN_POINT('Ctrl Pts',(87.8100368650045,50.9452034581481,13.3201185798864));
#73196=CARTESIAN_POINT('Ctrl Pts',(87.8271491852083,50.9469762946206,13.3227412527986));
#73197=CARTESIAN_POINT('Ctrl Pts',(87.8512374353375,50.9494408784373,13.3259304489418));
#73198=CARTESIAN_POINT('Ctrl Pts',(87.8581713872103,50.9501467390286,13.3267903222324));
#73199=CARTESIAN_POINT('Ctrl Pts',(87.8701048177369,50.951355011114,13.3281702759157));
#73200=CARTESIAN_POINT('Ctrl Pts',(87.8751008088186,50.9518588887623,13.3287179702252));
#73201=CARTESIAN_POINT('Ctrl Pts',(87.8857520150819,50.9529288337518,13.3298216757311));
#73202=CARTESIAN_POINT('Ctrl Pts',(87.8914078800005,50.9534944434384,13.3303694140808));
#73203=CARTESIAN_POINT('Ctrl Pts',(87.9069446667003,50.9550417218643,13.3317688726076));
#73204=CARTESIAN_POINT('Ctrl Pts',(87.9168325429424,50.9560192691645,13.3325428787274));
#73205=CARTESIAN_POINT('Ctrl Pts',(87.9894488021941,50.9631529404859,13.33737198038));
#73206=CARTESIAN_POINT('Ctrl Pts',(88.0524047341841,50.9690911195251,13.3368815752058));
#73207=CARTESIAN_POINT('Ctrl Pts',(88.1652082375716,50.9797181419027,13.327606112865));
#73208=CARTESIAN_POINT('Ctrl Pts',(88.2150498953138,50.9844093451062,13.3205093545668));
#73209=CARTESIAN_POINT('Ctrl Pts',(88.3005304078304,50.9926259398401,13.3031080190138));
#73210=CARTESIAN_POINT('Ctrl Pts',(88.3363801705357,50.9961252892169,13.2941658770595));
#73211=CARTESIAN_POINT('Ctrl Pts',(88.3836293596144,51.0008517473405,13.280166348107));
#73212=CARTESIAN_POINT('Ctrl Pts',(88.3954197416399,51.0020408105421,13.2764850269123));
#73213=CARTESIAN_POINT('Ctrl Pts',(88.4244001382436,51.0049898156787,13.2669703617734));
#73214=CARTESIAN_POINT('Ctrl Pts',(88.4415216933512,51.0067552395283,13.2609395284613));
#73215=CARTESIAN_POINT('Ctrl Pts',(88.4680192946969,51.0095279551601,13.2509627304541));
#73216=CARTESIAN_POINT('Ctrl Pts',(88.4774877682093,51.0105269395311,13.2472673091019));
#73217=CARTESIAN_POINT('Ctrl Pts',(88.4950747915169,51.0123985865962,13.2401589076645));
#73218=CARTESIAN_POINT('Ctrl Pts',(88.5032042416846,51.0132702472347,13.2367743244472));
#73219=CARTESIAN_POINT('Ctrl Pts',(88.5213359187787,51.0152295071382,13.2290032366264));
#73220=CARTESIAN_POINT('Ctrl Pts',(88.531317926608,51.0163185771885,13.2245717563011));
#73221=CARTESIAN_POINT('Ctrl Pts',(88.5568085318832,51.0191275643771,13.2128594303851));
#73222=CARTESIAN_POINT('Ctrl Pts',(88.572228573518,51.020853696034,13.2053927862796));
#73223=CARTESIAN_POINT('Ctrl Pts',(88.6667310003779,51.0316065665054,13.1572493886093));
#73224=CARTESIAN_POINT('Ctrl Pts',(88.7414919890587,51.0409057155117,13.1086803954499));
#73225=CARTESIAN_POINT('Ctrl Pts',(88.8492394954175,51.0555262295804,13.0213711142937));
#73226=CARTESIAN_POINT('Ctrl Pts',(88.8860518416663,51.0607804380291,12.9877723897631));
#73227=CARTESIAN_POINT('Ctrl Pts',(88.9330925070017,51.0677922254182,12.9394734709603));
#73228=CARTESIAN_POINT('Ctrl Pts',(88.9451237139666,51.0696144940624,12.9265948367129));
#73229=CARTESIAN_POINT('Ctrl Pts',(88.9654692388157,51.0727419338406,12.9038866299424));
#73230=CARTESIAN_POINT('Ctrl Pts',(88.9739091574118,51.0740537360569,12.8941736128847));
#73231=CARTESIAN_POINT('Ctrl Pts',(88.9862108198781,51.075985670113,12.8795739613433));
#73232=CARTESIAN_POINT('Ctrl Pts',(88.9901861868078,51.0766131818272,12.8747849846119));
#73233=CARTESIAN_POINT('Ctrl Pts',(88.9972672069768,51.0777364408778,12.8661259983265));
#73234=CARTESIAN_POINT('Ctrl Pts',(89.0003855361722,51.0782330441306,12.8622668401978));
#73235=CARTESIAN_POINT('Ctrl Pts',(89.0073646515024,51.0793489533023,12.8535253762663));
#73236=CARTESIAN_POINT('Ctrl Pts',(89.0112122684,51.0799673365591,12.8486328393164));
#73237=CARTESIAN_POINT('Ctrl Pts',(89.0229039848524,51.0818569883998,12.83353886815));
#73238=CARTESIAN_POINT('Ctrl Pts',(89.0306295454953,51.0831204942264,12.8232458157112));
#73239=CARTESIAN_POINT('Ctrl Pts',(89.0726505548739,51.0900890733903,12.765450170921));
#73240=CARTESIAN_POINT('Ctrl Pts',(89.1037892396832,51.0956206146516,12.7157280493234));
#73241=CARTESIAN_POINT('Ctrl Pts',(89.155273356326,51.105885176255,12.6192736327138));
#73242=CARTESIAN_POINT('Ctrl Pts',(89.1764569382815,51.110616051943,12.5731323794142));
#73243=CARTESIAN_POINT('Ctrl Pts',(89.2080211088673,51.1188293148092,12.4918742429685));
#73244=CARTESIAN_POINT('Ctrl Pts',(89.2197483765835,51.1222837897439,12.4573506732537));
#73245=CARTESIAN_POINT('Ctrl Pts',(89.2334063140848,51.1269530411692,12.4106337177286));
#73246=CARTESIAN_POINT('Ctrl Pts',(89.2366685298787,51.1281307225479,12.3988456536996));
#73247=CARTESIAN_POINT('Ctrl Pts',(89.244314561596,51.1310557365436,12.3695784755436));
#73248=CARTESIAN_POINT('Ctrl Pts',(89.2484974042333,51.1328085065896,12.3520503378366));
#73249=CARTESIAN_POINT('Ctrl Pts',(89.2544482866336,51.1355657781011,12.3245326069871));
#73250=CARTESIAN_POINT('Ctrl Pts',(89.2564720872051,51.1365621252465,12.3146001119612));
#73251=CARTESIAN_POINT('Ctrl Pts',(89.2600318300694,51.1384313750803,12.2959936298492));
#73252=CARTESIAN_POINT('Ctrl Pts',(89.2615968513931,51.1393032976045,12.2873257501095));
#73253=CARTESIAN_POINT('Ctrl Pts',(89.2649062760589,51.1412665006684,12.2678393580063));
#73254=CARTESIAN_POINT('Ctrl Pts',(89.2666010411752,51.1423592796885,12.2570133022467));
#73255=CARTESIAN_POINT('Ctrl Pts',(89.2706037459408,51.1451847713726,12.2290835523616));
#73256=CARTESIAN_POINT('Ctrl Pts',(89.272703408528,51.146923824872,12.2119529915864));
#73257=CARTESIAN_POINT('Ctrl Pts',(89.2831549136372,51.157374972638,12.1094186632909));
#73258=CARTESIAN_POINT('Ctrl Pts',(89.2831802528016,51.1663386329533,12.0234094526222));
#73259=CARTESIAN_POINT('Ctrl Pts',(89.2693112502228,51.1808517088892,11.8864221737266));
#73260=CARTESIAN_POINT('Ctrl Pts',(89.2609190017953,51.18633380876,11.8351352372675));
#73261=CARTESIAN_POINT('Ctrl Pts',(89.2454125038135,51.1936130669747,11.7669163114878));
#73262=CARTESIAN_POINT('Ctrl Pts',(89.2410404169332,51.1954790777445,11.749415176521));
#73263=CARTESIAN_POINT('Ctrl Pts',(89.2328538905988,51.1986732227454,11.7193814029891));
#73264=CARTESIAN_POINT('Ctrl Pts',(89.2292157730967,51.2000083488342,11.7068040085793));
#73265=CARTESIAN_POINT('Ctrl Pts',(89.2235495255271,51.2019676738704,11.6882925572965));
#73266=CARTESIAN_POINT('Ctrl Pts',(89.2216711099963,51.2025995475692,11.6823142774983));
#73267=CARTESIAN_POINT('Ctrl Pts',(89.21822618287,51.2037271941518,11.6716276371158));
#73268=CARTESIAN_POINT('Ctrl Pts',(89.2166762577483,51.2042238579118,11.6669143173981));
#73269=CARTESIAN_POINT('Ctrl Pts',(89.2131331788622,51.2053356875237,11.6563488867037));
#73270=CARTESIAN_POINT('Ctrl Pts',(89.2111248720212,51.2059499648591,11.6505020917065));
#73271=CARTESIAN_POINT('Ctrl Pts',(89.2048776855024,51.2078139831363,11.6327378916362));
#73272=CARTESIAN_POINT('Ctrl Pts',(89.2005031851558,51.2090562621806,11.6208683345868));
#73273=CARTESIAN_POINT('Ctrl Pts',(89.170238728609,51.2172624221028,11.5423846448894));
#73274=CARTESIAN_POINT('Ctrl Pts',(89.138935603695,51.2239623865126,11.4779813141137));
#73275=CARTESIAN_POINT('Ctrl Pts',(89.0561090910428,51.2391383734191,11.3387904389401));
#73276=CARTESIAN_POINT('Ctrl Pts',(89.0016608137928,51.2475847792139,11.2661996161526));
#73277=CARTESIAN_POINT('Ctrl Pts',(88.9289867364727,51.2579154583508,11.1882420656301));
#73278=CARTESIAN_POINT('Ctrl Pts',(88.9177986252339,51.2594827739811,11.1766885601194));
#73279=CARTESIAN_POINT('Ctrl Pts',(88.8994931247381,51.2620137124744,11.1584898468565));
#73280=CARTESIAN_POINT('Ctrl Pts',(88.8925131035788,51.2629712866419,11.1517082818468));
#73281=CARTESIAN_POINT('Ctrl Pts',(88.8790165122139,51.2648093353586,11.1388936491756));
#73282=CARTESIAN_POINT('Ctrl Pts',(88.8725132132093,51.2656891720706,11.1328473734218));
#73283=CARTESIAN_POINT('Ctrl Pts',(88.8574813508069,51.2677101567449,11.1191629535415));
#73284=CARTESIAN_POINT('Ctrl Pts',(88.8489119862787,51.2688531567997,11.1115710864687));
#73285=CARTESIAN_POINT('Ctrl Pts',(88.8215674176925,51.2724732657526,11.0879977762989));
#73286=CARTESIAN_POINT('Ctrl Pts',(88.8024302333195,51.2749674462781,11.0724478584596));
#73287=CARTESIAN_POINT('Ctrl Pts',(88.699655813023,51.2881739062547,10.9937922245773));
#73288=CARTESIAN_POINT('Ctrl Pts',(88.6089125115153,51.2992501117441,10.9406700660958));
#73289=CARTESIAN_POINT('Ctrl Pts',(88.4829718369426,51.3136654021562,10.886512684579));
#73290=CARTESIAN_POINT('Ctrl Pts',(88.4527551870671,51.317053687807,10.8748658944421));
#73291=CARTESIAN_POINT('Ctrl Pts',(88.4033453136906,51.3224553898071,10.8579606479839));
#73292=CARTESIAN_POINT('Ctrl Pts',(88.3844167071596,51.3244927569641,10.8519760975121));
#73293=CARTESIAN_POINT('Ctrl Pts',(88.3582891209898,51.3272551801618,10.844384516329));
#73294=CARTESIAN_POINT('Ctrl Pts',(88.3512064085372,51.3279990629208,10.8423931461976));
#73295=CARTESIAN_POINT('Ctrl Pts',(88.3391987044207,51.329251419441,10.8391293971574));
#73296=CARTESIAN_POINT('Ctrl Pts',(88.3342827609187,51.3297616511068,10.8378248793202));
#73297=CARTESIAN_POINT('Ctrl Pts',(88.3240146246647,51.3308220840184,10.8351660060951));
#73298=CARTESIAN_POINT('Ctrl Pts',(88.3186612444582,51.3313719846676,10.8338169621516));
#73299=CARTESIAN_POINT('Ctrl Pts',(88.3041388757967,51.3328561616506,10.8302578958513));
#73300=CARTESIAN_POINT('Ctrl Pts',(88.2949534791662,51.3337867657434,10.8281149529939));
#73301=CARTESIAN_POINT('Ctrl Pts',(88.2471666561997,51.338590432386,10.8175262773889));
#73302=CARTESIAN_POINT('Ctrl Pts',(88.2082046080001,51.3423797516393,10.8107818300825));
#73303=CARTESIAN_POINT('Ctrl Pts',(88.0808269138722,51.3545554784744,10.7948122457321));
#73304=CARTESIAN_POINT('Ctrl Pts',(87.9917505918072,51.3627570528973,10.7930409782929));
#73305=CARTESIAN_POINT('Ctrl Pts',(87.859973992344,51.3752848362197,10.804265242885));
#73306=CARTESIAN_POINT('Ctrl Pts',(87.8169546560851,51.3794351898445,10.8101620399867));
#73307=CARTESIAN_POINT('Ctrl Pts',(87.7606665597119,51.3850056077569,10.8208387800724));
#73308=CARTESIAN_POINT('Ctrl Pts',(87.7470511953186,51.3863638724029,10.8236537170663));
#73309=CARTESIAN_POINT('Ctrl Pts',(87.7244308013906,51.3886404786809,10.8287190329065));
#73310=CARTESIAN_POINT('Ctrl Pts',(87.7153989849389,51.3895548364401,10.8308457077787));
#73311=CARTESIAN_POINT('Ctrl Pts',(87.6976607825607,51.3913617439212,10.835228122518));
#73312=CARTESIAN_POINT('Ctrl Pts',(87.6889534389196,51.3922540480884,10.8374777651735));
#73313=CARTESIAN_POINT('Ctrl Pts',(87.669782373453,51.3942309325549,10.8426486416162));
#73314=CARTESIAN_POINT('Ctrl Pts',(87.6593309045423,51.3953168147763,10.8456120112212));
#73315=CARTESIAN_POINT('Ctrl Pts',(87.6234042117042,51.3990788443186,10.8562983362493));
#73316=CARTESIAN_POINT('Ctrl Pts',(87.5981367770844,51.4017761319917,10.8646872599623));
#73317=CARTESIAN_POINT('Ctrl Pts',(87.4857161967608,51.4140238234804,10.9059769077466));
#73318=CARTESIAN_POINT('Ctrl Pts',(87.402092817642,51.4238437394858,10.947607468878));
#73319=CARTESIAN_POINT('Ctrl Pts',(87.2808228362238,51.4390337497524,11.0256385787474));
#73320=CARTESIAN_POINT('Ctrl Pts',(87.2395569886027,51.4443923953111,11.0558575977986));
#73321=CARTESIAN_POINT('Ctrl Pts',(87.1905837010173,51.4509155773321,11.0964775279904));
#73322=CARTESIAN_POINT('Ctrl Pts',(87.1810658458023,51.4521914975508,11.1046124248178));
#73323=CARTESIAN_POINT('Ctrl Pts',(87.1670485818414,51.4540811362545,11.1169563176296));
#73324=CARTESIAN_POINT('Ctrl Pts',(87.1624574187888,51.454701792407,11.1210590489672));
#73325=CARTESIAN_POINT('Ctrl Pts',(87.154220216904,51.4558182201388,11.1285283866829));
#73326=CARTESIAN_POINT('Ctrl Pts',(87.1505639191276,51.4563147927477,11.1318831035276));
#73327=CARTESIAN_POINT('Ctrl Pts',(87.1423154210495,51.4574374318566,11.139540772407));
#73328=CARTESIAN_POINT('Ctrl Pts',(87.1377354138947,51.4580625198593,11.143856536677));
#73329=CARTESIAN_POINT('Ctrl Pts',(87.1236246156361,51.4599945921281,11.157352636741));
#73330=CARTESIAN_POINT('Ctrl Pts',(87.1142045750657,51.4612933018189,11.1666485003378));
#73331=CARTESIAN_POINT('Ctrl Pts',(87.0463119314727,51.4707365649291,11.2357739931844));
#73332=CARTESIAN_POINT('Ctrl Pts',(86.993721774966,51.4785204051252,11.3011152185336));
#73333=CARTESIAN_POINT('Ctrl Pts',(86.9194934654134,51.4912329536637,11.4146814228274));
#73334=CARTESIAN_POINT('Ctrl Pts',(86.8937529958692,51.4961117558921,11.4598970818801));
#73335=CARTESIAN_POINT('Ctrl Pts',(86.8564776726467,51.5041836066285,11.5358644190922));
#73336=CARTESIAN_POINT('Ctrl Pts',(86.8432351341186,51.507324868133,11.5657097376064));
#73337=CARTESIAN_POINT('Ctrl Pts',(86.8264795623958,51.5117362128425,11.6077739007571));
#73338=CARTESIAN_POINT('Ctrl Pts',(86.821977084653,51.5129733464209,11.6195872940853));
#73339=CARTESIAN_POINT('Ctrl Pts',(86.8145597080186,51.5151049605263,11.6399573931017));
#73340=CARTESIAN_POINT('Ctrl Pts',(86.8115583567113,51.515996517825,11.6484818460083));
#73341=CARTESIAN_POINT('Ctrl Pts',(86.8059887358412,51.517708698356,11.6648565507218));
#73342=CARTESIAN_POINT('Ctrl Pts',(86.8034055612349,51.5185287806601,11.6727012879839));
#73343=CARTESIAN_POINT('Ctrl Pts',(86.7974945408428,51.5204688244557,11.6912596220072));
#73344=CARTESIAN_POINT('Ctrl Pts',(86.7942318473777,51.5215908472242,11.7019930051687));
#73345=CARTESIAN_POINT('Ctrl Pts',(86.7830220936081,51.5256389372007,11.7407059081105));
#73346=CARTESIAN_POINT('Ctrl Pts',(86.7758953303166,51.5285907381942,11.7689106367472));
#73347=CARTESIAN_POINT('Ctrl Pts',(86.750561903591,51.5408647765453,11.8859521652629));
#73348=CARTESIAN_POINT('Ctrl Pts',(86.7409293229408,51.5504299644905,11.9763568610618));
#73349=CARTESIAN_POINT('Ctrl Pts',(86.7410430757661,51.5657096205168,12.1214365257508));
#73350=CARTESIAN_POINT('Ctrl Pts',(86.7445862925543,51.5714147465689,12.1758269348659));
#73351=CARTESIAN_POINT('Ctrl Pts',(86.7528915680399,51.5779873340751,12.2396711533848));
#73352=CARTESIAN_POINT('Ctrl Pts',(86.7542872187237,51.5789953780693,12.2494979665258));
#73353=CARTESIAN_POINT('Ctrl Pts',(86.7566544540706,51.5805655728232,12.2648690801218));
#73354=CARTESIAN_POINT('Ctrl Pts',(86.7575478766861,51.581131733278,12.2704246528713));
#73355=CARTESIAN_POINT('Ctrl Pts',(86.7593121052029,51.5822014180731,12.2809484866138));
#73356=CARTESIAN_POINT('Ctrl Pts',(86.7601755892262,51.5827052854402,12.2859175600669));
#73357=CARTESIAN_POINT('Ctrl Pts',(86.762326406213,51.5839148162359,12.297872174857));
#73358=CARTESIAN_POINT('Ctrl Pts',(86.7636427848273,51.5846188581633,12.3048523304708));
#73359=CARTESIAN_POINT('Ctrl Pts',(86.7685156466526,51.5871035613752,12.3295511570532));
#73360=CARTESIAN_POINT('Ctrl Pts',(86.7723919341085,51.5888677365882,12.3472059042553));
#73361=CARTESIAN_POINT('Ctrl Pts',(86.7802565610388,51.5921033245222,12.3796979041116));
#73362=CARTESIAN_POINT('Ctrl Pts',(86.784139579768,51.5935785587552,12.394556468848));
#73363=CARTESIAN_POINT('Ctrl Pts',(86.8062828961033,51.6014032959769,12.4734132303857));
#73364=CARTESIAN_POINT('Ctrl Pts',(86.8292843776834,51.6075993535272,12.5359773289825));
#73365=CARTESIAN_POINT('Ctrl Pts',(86.8872910225581,51.6206197714087,12.6621608049326));
#73366=CARTESIAN_POINT('Ctrl Pts',(86.9230474371549,51.6274307846633,12.7251554959279));
#73367=CARTESIAN_POINT('Ctrl Pts',(86.9730248299818,51.6359912189574,12.7979589349563));
#73368=CARTESIAN_POINT('Ctrl Pts',(86.982334295024,51.6375516561407,12.8109853342826));
#73369=CARTESIAN_POINT('Ctrl Pts',(86.9976852581056,51.6400742032395,12.8316289256802));
#73370=CARTESIAN_POINT('Ctrl Pts',(87.0035725913524,51.6410303375728,12.8393591799687));
#73371=CARTESIAN_POINT('Ctrl Pts',(87.0150114201699,51.6428674009647,12.8540264448457));
#73372=CARTESIAN_POINT('Ctrl Pts',(87.0205481762864,51.6437477058152,12.8609742785927));
#73373=CARTESIAN_POINT('Ctrl Pts',(87.0335302257596,51.6457919685805,12.8769187408945));
#73374=CARTESIAN_POINT('Ctrl Pts',(87.0410274803757,51.646957968272,12.885871728769));
#73375=CARTESIAN_POINT('Ctrl Pts',(87.0657872669771,51.650763473949,12.9146241044349));
#73376=CARTESIAN_POINT('Ctrl Pts',(87.0835394131259,51.6534227952322,12.933989965764));
#73377=CARTESIAN_POINT('Ctrl Pts',(87.1270707845374,51.659792555792,12.9786176184718));
#73378=CARTESIAN_POINT('Ctrl Pts',(87.1533498826672,51.6635217203355,13.0033565971518));
#73379=CARTESIAN_POINT('Ctrl Pts',(87.1806428357067,51.6672833294972,13.026940674395));
#73380=CARTESIAN_POINT('',(86.7410004204394,51.72907359951,12.0649665997861));
#73381=CARTESIAN_POINT('Ctrl Pts',(87.1792973239246,51.8375066538898,13.0285052387874));
#73382=CARTESIAN_POINT('Ctrl Pts',(87.1707267540613,51.8363772938414,13.0211360806275));
#73383=CARTESIAN_POINT('Ctrl Pts',(86.8998704527144,51.8002331995894,12.7813463937796));
#73384=CARTESIAN_POINT('Ctrl Pts',(86.7432354015658,51.7640891053375,12.4162822252844));
#73385=CARTESIAN_POINT('Ctrl Pts',(86.7401346566022,51.7290743711339,12.0649736370867));
#73386=CARTESIAN_POINT('Ctrl Pts',(86.7410004204394,51.72907359951,12.0649665997861));
#73387=CARTESIAN_POINT('Ctrl Pts',(86.7410574454711,51.7220838427605,11.9948855554347));
#73388=CARTESIAN_POINT('Ctrl Pts',(86.7469171288941,51.715094086011,11.9250345638552));
#73389=CARTESIAN_POINT('Ctrl Pts',(86.7584556185441,51.7081043292614,11.8561606031191));
#73390=CARTESIAN_POINT('Ctrl Pts',(86.7666237113341,51.7031562829017,11.807404750389));
#73391=CARTESIAN_POINT('Ctrl Pts',(86.7776608791493,51.698208236542,11.759018762359));
#73392=CARTESIAN_POINT('Ctrl Pts',(86.7915187869455,51.6932601901823,11.7113655811865));
#73393=CARTESIAN_POINT('Ctrl Pts',(86.805351196489,51.6883212481217,11.663800080844));
#73394=CARTESIAN_POINT('Ctrl Pts',(86.8219939005199,51.683382306061,11.6169652350239));
#73395=CARTESIAN_POINT('Ctrl Pts',(86.8413475075088,51.6784433640004,11.5712141404515));
#73396=CARTESIAN_POINT('Ctrl Pts',(86.8606814637615,51.6735094367076,11.5255094993744));
#73397=CARTESIAN_POINT('Ctrl Pts',(86.8827206614617,51.6685755094149,11.4808869333989));
#73398=CARTESIAN_POINT('Ctrl Pts',(86.9073164919653,51.6636415821222,11.4376826326671));
#73399=CARTESIAN_POINT('Ctrl Pts',(86.931897815201,51.6587105649896,11.3945038149685));
#73400=CARTESIAN_POINT('Ctrl Pts',(86.9590325132943,51.6537795478569,11.3527420806323));
#73401=CARTESIAN_POINT('Ctrl Pts',(86.9885257684931,51.6488485307243,11.3127095872743));
#73402=CARTESIAN_POINT('Ctrl Pts',(87.0180141771654,51.643918323889,11.2726836723202));
#73403=CARTESIAN_POINT('Ctrl Pts',(87.0498600478677,51.6389881170537,11.234386874561));
#73404=CARTESIAN_POINT('Ctrl Pts',(87.0838264121602,51.6340579102184,11.1981007327965));
#73405=CARTESIAN_POINT('Ctrl Pts',(87.1178259624633,51.6291228864444,11.1617791385394));
#73406=CARTESIAN_POINT('Ctrl Pts',(87.1539497669398,51.6241878626704,11.1274725226636));
#73407=CARTESIAN_POINT('Ctrl Pts',(87.1919231183123,51.6192528388963,11.0954264263413));
#73408=CARTESIAN_POINT('Ctrl Pts',(87.2299169057445,51.6143151592482,11.0633630838208));
#73409=CARTESIAN_POINT('Ctrl Pts',(87.2697617828868,51.6093774796001,11.0335630118872));
#73410=CARTESIAN_POINT('Ctrl Pts',(87.3111518062313,51.6044397999519,11.006229975099));
#73411=CARTESIAN_POINT('Ctrl Pts',(87.3526191203687,51.5994928997925,10.9788458972164));
#73412=CARTESIAN_POINT('Ctrl Pts',(87.3956368650549,51.5945459996332,10.9539383239309));
#73413=CARTESIAN_POINT('Ctrl Pts',(87.4398735480189,51.5895990994738,10.9316655802421));
#73414=CARTESIAN_POINT('Ctrl Pts',(87.462256177663,51.5870960945753,10.9203961418543));
#73415=CARTESIAN_POINT('Ctrl Pts',(87.4849505357424,51.5845930896767,10.9098004835379));
#73416=CARTESIAN_POINT('Ctrl Pts',(87.5079119951131,51.5820900847782,10.8998943189664));
#73417=CARTESIAN_POINT('Ctrl Pts',(87.5533031872588,51.5771420379465,10.8803113903627));
#73418=CARTESIAN_POINT('Ctrl Pts',(87.5999398310792,51.5721939911148,10.8633394471891));
#73419=CARTESIAN_POINT('Ctrl Pts',(87.6474907942364,51.5672459442831,10.8491347415079));
#73420=CARTESIAN_POINT('Ctrl Pts',(87.6949542647047,51.5623070017449,10.8349561721615));
#73421=CARTESIAN_POINT('Ctrl Pts',(87.7433281971118,51.5573680592066,10.8235348974083));
#73422=CARTESIAN_POINT('Ctrl Pts',(87.7922620375085,51.5524291166684,10.814978935523));
#73423=CARTESIAN_POINT('Ctrl Pts',(87.8411461928357,51.547495188895,10.8064316609503));
#73424=CARTESIAN_POINT('Ctrl Pts',(87.890588593523,51.5425612611216,10.8007440337539));
#73425=CARTESIAN_POINT('Ctrl Pts',(87.9402261939047,51.5376273333482,10.7979735537574));
#73426=CARTESIAN_POINT('Ctrl Pts',(87.989834516748,51.5326963157328,10.7952047078614));
#73427=CARTESIAN_POINT('Ctrl Pts',(88.0396372651039,51.5277652981174,10.7953496310471));
#73428=CARTESIAN_POINT('Ctrl Pts',(88.0892665197824,51.522834280502,10.7984139666748));
#73429=CARTESIAN_POINT('Ctrl Pts',(88.1388876190668,51.5179040731827,10.8014777987514));
#73430=CARTESIAN_POINT('Ctrl Pts',(88.1883347346994,51.5129738658635,10.8074600561353));
#73431=CARTESIAN_POINT('Ctrl Pts',(88.2372428085287,51.5080436585442,10.816314362894));
#73432=CARTESIAN_POINT('Ctrl Pts',(88.2861986667775,51.5031086342882,10.8251773205333));
#73433=CARTESIAN_POINT('Ctrl Pts',(88.3346138916304,51.4981736100322,10.8369178313481));
#73434=CARTESIAN_POINT('Ctrl Pts',(88.3821331978085,51.4932385857763,10.8514382891411));
#73435=CARTESIAN_POINT('Ctrl Pts',(88.4296780773711,51.4883009056467,10.8659665613843));
#73436=CARTESIAN_POINT('Ctrl Pts',(88.4763255638781,51.4833632255171,10.8832775689133));
#73437=CARTESIAN_POINT('Ctrl Pts',(88.5217385269754,51.4784255453875,10.903224803729));
#73438=CARTESIAN_POINT('Ctrl Pts',(88.567236293145,51.4734786447531,10.9232092875301));
#73439=CARTESIAN_POINT('Ctrl Pts',(88.6114944466437,51.4685317441187,10.9458395743221));
#73440=CARTESIAN_POINT('Ctrl Pts',(88.6542001742352,51.4635848434842,10.9709230456886));
#73441=CARTESIAN_POINT('Ctrl Pts',(88.6758081444493,51.4610818424212,10.9836146196935));
#73442=CARTESIAN_POINT('Ctrl Pts',(88.6970191400709,51.4585788413581,10.9969335388941));
#73443=CARTESIAN_POINT('Ctrl Pts',(88.7177957541759,51.456075840295,11.0108508342993));
#73444=CARTESIAN_POINT('Ctrl Pts',(88.7588678986207,51.4511277953109,11.0383631692868));
#73445=CARTESIAN_POINT('Ctrl Pts',(88.7984220319169,51.4461797503268,11.0683380283455));
#73446=CARTESIAN_POINT('Ctrl Pts',(88.8361472777453,51.4412317053428,11.1005819713567));
#73447=CARTESIAN_POINT('Ctrl Pts',(88.8738031099641,51.4362927646509,11.132766586233));
#73448=CARTESIAN_POINT('Ctrl Pts',(88.9096363157023,51.4313538239591,11.1672116513664));
#73449=CARTESIAN_POINT('Ctrl Pts',(88.9433660065904,51.4264148832673,11.2036812481718));
#73450=CARTESIAN_POINT('Ctrl Pts',(88.9770614499743,51.421480957338,11.2401138155043));
#73451=CARTESIAN_POINT('Ctrl Pts',(89.008657236395,51.4165470314088,11.2785664447452));
#73452=CARTESIAN_POINT('Ctrl Pts',(89.0379081435998,51.4116131054796,11.3187653215968));
#73453=CARTESIAN_POINT('Ctrl Pts',(89.0671417978915,51.4066820897027,11.3589404881502));
#73454=CARTESIAN_POINT('Ctrl Pts',(89.0940329910739,51.4017510739257,11.4008594196246));
#73455=CARTESIAN_POINT('Ctrl Pts',(89.1183774232072,51.3968200581488,11.4442160804822));
#73456=CARTESIAN_POINT('Ctrl Pts',(89.1427178549522,51.391889852659,11.4875656167752));
#73457=CARTESIAN_POINT('Ctrl Pts',(89.1645120891895,51.3869596471691,11.5323519353977));
#73458=CARTESIAN_POINT('Ctrl Pts',(89.1836010803103,51.3820294416793,11.5782431892274));
#73459=CARTESIAN_POINT('Ctrl Pts',(89.2027087219714,51.3770944192247,11.6241792802448));
#73460=CARTESIAN_POINT('Ctrl Pts',(89.2191056333498,51.3721593967702,11.6712219546057));
#73461=CARTESIAN_POINT('Ctrl Pts',(89.2326811092605,51.3672243743156,11.7190197883509));
#73462=CARTESIAN_POINT('Ctrl Pts',(89.2462638911013,51.3622866959741,11.7668433455137));
#73463=CARTESIAN_POINT('Ctrl Pts',(89.2570220952417,51.3573490176326,11.8154223357806));
#73464=CARTESIAN_POINT('Ctrl Pts',(89.264895947147,51.3524113392911,11.8643940632613));
#73465=CARTESIAN_POINT('Ctrl Pts',(89.272784502565,51.3474644404032,11.91345723981));
#73466=CARTESIAN_POINT('Ctrl Pts',(89.2777779005425,51.3425175415153,11.9629140718333));
#73467=CARTESIAN_POINT('Ctrl Pts',(89.2798682944581,51.3375706426275,12.0123972825424));
#73468=CARTESIAN_POINT('Ctrl Pts',(89.2809259850863,51.3350676270222,12.0374346345097));
#73469=CARTESIAN_POINT('Ctrl Pts',(89.2812413025968,51.332564611417,12.06247875113));
#73470=CARTESIAN_POINT('Ctrl Pts',(89.2808182950789,51.3300615958117,12.087482492471));
#73471=CARTESIAN_POINT('Ctrl Pts',(89.279982079308,51.325113548707,12.136910746011));
#73472=CARTESIAN_POINT('Ctrl Pts',(89.2762536753466,51.3201655016022,12.1863993558836));
#73473=CARTESIAN_POINT('Ctrl Pts',(89.2696269775012,51.3152174544974,12.235582226386));
#73474=CARTESIAN_POINT('Ctrl Pts',(89.2630124726603,51.31027851171,12.2846746012953));
#73475=CARTESIAN_POINT('Ctrl Pts',(89.2535103232701,51.3053395689225,12.3334618139219));
#73476=CARTESIAN_POINT('Ctrl Pts',(89.2411663761222,51.300400626135,12.3815799218239));
#73477=CARTESIAN_POINT('Ctrl Pts',(89.2288349624615,51.2954666981273,12.4296491727693));
#73478=CARTESIAN_POINT('Ctrl Pts',(89.2136675987204,51.2905327701195,12.4770501356944));
#73479=CARTESIAN_POINT('Ctrl Pts',(89.1957613139366,51.2855988421118,12.5234282774371));
#73480=CARTESIAN_POINT('Ctrl Pts',(89.1778655907964,51.2806678242772,12.5697790640134));
#73481=CARTESIAN_POINT('Ctrl Pts',(89.1572343439754,51.2757368064426,12.6151077143118));
#73482=CARTESIAN_POINT('Ctrl Pts',(89.1340138684682,51.270805788608,12.659076598112));
#73483=CARTESIAN_POINT('Ctrl Pts',(89.1107972087694,51.265875581085,12.7030382565289));
#73484=CARTESIAN_POINT('Ctrl Pts',(89.0849924217139,51.2609453735619,12.7456401082241));
#73485=CARTESIAN_POINT('Ctrl Pts',(89.0567920330508,51.2560151660388,12.7865685419219));
#73486=CARTESIAN_POINT('Ctrl Pts',(89.0285640920397,51.2510801416037,12.8275369635243));
#73487=CARTESIAN_POINT('Ctrl Pts',(88.9979361886039,51.2461451171685,12.8668282512264));
#73488=CARTESIAN_POINT('Ctrl Pts',(88.965143515197,51.2412100927333,12.9041587871086));
#73489=CARTESIAN_POINT('Ctrl Pts',(88.9323331939043,51.2362724124382,12.9415094129977));
#73490=CARTESIAN_POINT('Ctrl Pts',(88.897356168362,51.2313347321431,12.9768967956966));
#73491=CARTESIAN_POINT('Ctrl Pts',(88.860484725547,51.226397051848,13.010073991307));
#73492=CARTESIAN_POINT('Ctrl Pts',(88.8235444300621,51.221450151071,13.0433131410564));
#73493=CARTESIAN_POINT('Ctrl Pts',(88.7847030851708,51.216503250294,13.074333524153));
#73494=CARTESIAN_POINT('Ctrl Pts',(88.744264992011,51.211556349517,13.1029293377521));
#73495=CARTESIAN_POINT('Ctrl Pts',(88.7238043991424,51.2090533501208,13.1173980541054));
#73496=CARTESIAN_POINT('Ctrl Pts',(88.7029354661896,51.2065503507247,13.1312467641965));
#73497=CARTESIAN_POINT('Ctrl Pts',(88.6816999912418,51.2040473513286,13.1444533006803));
#73498=CARTESIAN_POINT('Ctrl Pts',(88.6397206804174,51.1990993014309,13.1705606188038));
#73499=CARTESIAN_POINT('Ctrl Pts',(88.5961219425973,51.1941512515332,13.1942708819615));
#73500=CARTESIAN_POINT('Ctrl Pts',(88.5512080313302,51.1892032016355,13.2153803908569));
#73501=CARTESIAN_POINT('Ctrl Pts',(88.5063767603522,51.1842642560055,13.2364510588705));
#73502=CARTESIAN_POINT('Ctrl Pts',(88.4602356072625,51.1793253103755,13.2549302323215));
#73503=CARTESIAN_POINT('Ctrl Pts',(88.4131151955272,51.1743863647455,13.2706590262502));
#73504=CARTESIAN_POINT('Ctrl Pts',(88.3660426274367,51.1694524338672,13.2863718499698));
#73505=CARTESIAN_POINT('Ctrl Pts',(88.3179932863306,51.1645185029888,13.2993396498775));
#73506=CARTESIAN_POINT('Ctrl Pts',(88.2693176518826,51.1595845721104,13.3094516439033));
#73507=CARTESIAN_POINT('Ctrl Pts',(88.2206707274901,51.1546535513827,13.3195576736327));
#73508=CARTESIAN_POINT('Ctrl Pts',(88.1713987770709,51.149722530655,13.3268111231438));
#73509=CARTESIAN_POINT('Ctrl Pts',(88.1218648015373,51.1447915099273,13.331151767884));
#73510=CARTESIAN_POINT('Ctrl Pts',(88.0723389657214,51.1398612994943,13.3354916993437));
#73511=CARTESIAN_POINT('Ctrl Pts',(88.0225517359407,51.1349310890612,13.3369197294466));
#73512=CARTESIAN_POINT('Ctrl Pts',(87.9728710097596,51.1300008786282,13.3354275009244));
#73513=CARTESIAN_POINT('Ctrl Pts',(87.9231417445166,51.1250658512811,13.3339338144652));
#73514=CARTESIAN_POINT('Ctrl Pts',(87.8735197393815,51.120130823934,13.3295141902602));
#73515=CARTESIAN_POINT('Ctrl Pts',(87.8243708362133,51.1151957965869,13.3222123846007));
#73516=CARTESIAN_POINT('Ctrl Pts',(87.7751954827628,51.1102581133745,13.3149066493557));
#73517=CARTESIAN_POINT('Ctrl Pts',(87.7264942751833,51.105320430162,13.3047157563041));
#73518=CARTESIAN_POINT('Ctrl Pts',(87.6786223647281,51.1003827469496,13.2917345175735));
#73519=CARTESIAN_POINT('Ctrl Pts',(87.6306610599554,51.0954358432817,13.2787290381353));
#73520=CARTESIAN_POINT('Ctrl Pts',(87.5835326629146,51.0904889396138,13.2629229877022));
#73521=CARTESIAN_POINT('Ctrl Pts',(87.5375751258267,51.0855420359458,13.2444603890305));
#73522=CARTESIAN_POINT('Ctrl Pts',(87.5143220695857,51.083039059579,13.2351188996368));
#73523=CARTESIAN_POINT('Ctrl Pts',(87.4913684052438,51.0805360832122,13.2250980770676));
#73524=CARTESIAN_POINT('Ctrl Pts',(87.4687554261298,51.0780331068453,13.2144210125683));
#73525=CARTESIAN_POINT('Ctrl Pts',(87.4240553196919,51.0730853593838,13.1933151725478));
#73526=CARTESIAN_POINT('Ctrl Pts',(87.3804905119902,51.0681376119222,13.1695489817321));
#73527=CARTESIAN_POINT('Ctrl Pts',(87.3383971025424,51.0631898644607,13.1432675351702));
#73528=CARTESIAN_POINT('Ctrl Pts',(87.2963761237482,51.0582506306497,13.1170313114205));
#73529=CARTESIAN_POINT('Ctrl Pts',(87.2558219855198,51.0533113968388,13.0882886988727));
#73530=CARTESIAN_POINT('Ctrl Pts',(87.217047557413,51.0483721630279,13.0572313145326));
#73531=CARTESIAN_POINT('Ctrl Pts',(87.204730094991,51.0468031179167,13.047365323383));
#73532=CARTESIAN_POINT('Ctrl Pts',(87.1925920371449,51.0452340728055,13.0372660829162));
#73533=CARTESIAN_POINT('Ctrl Pts',(87.1806428354228,51.0436650276944,13.0269406741497));
#73534=CARTESIAN_POINT('Origin',(88.011,66.41344859951,12.066));
#73535=CARTESIAN_POINT('',(87.1806428554372,50.081424866233,13.0269406914443));
#73536=CARTESIAN_POINT('',(87.1806428354216,50.251127131729,13.0269406741487));
#73537=CARTESIAN_POINT('',(87.1806428354228,66.41344859951,13.0269406741497));
#73538=CARTESIAN_POINT('',(86.7410003813397,50.764592782682,12.066337079236));
#73539=CARTESIAN_POINT('Ctrl Pts',(87.1806428554372,50.081424866233,13.0269406914443));
#73540=CARTESIAN_POINT('Ctrl Pts',(87.2137718936792,50.0856223393657,13.0555677792986));
#73541=CARTESIAN_POINT('Ctrl Pts',(87.2483726174281,50.0897447031932,13.0824741104664));
#73542=CARTESIAN_POINT('Ctrl Pts',(87.3456350912355,50.1008674491368,13.1503343910258));
#73543=CARTESIAN_POINT('Ctrl Pts',(87.4106144382412,50.1078244608523,13.1876182254033));
#73544=CARTESIAN_POINT('Ctrl Pts',(87.4983872052244,50.1170475336888,13.2281567654651));
#73545=CARTESIAN_POINT('Ctrl Pts',(87.5185150137556,50.1191506355758,13.2368281867314));
#73546=CARTESIAN_POINT('Ctrl Pts',(87.5552212134029,50.1229749750837,13.2515279314804));
#73547=CARTESIAN_POINT('Ctrl Pts',(87.5717202782133,50.1246900545637,13.2577399177896));
#73548=CARTESIAN_POINT('Ctrl Pts',(87.5977901198249,50.1273977183724,13.2669404535801));
#73549=CARTESIAN_POINT('Ctrl Pts',(87.6072766813256,50.1283825320622,13.270162715654));
#73550=CARTESIAN_POINT('Ctrl Pts',(87.6251287290019,50.1302355876166,13.275991787139));
#73551=CARTESIAN_POINT('Ctrl Pts',(87.6334850659694,50.1311029029523,13.2786249327349));
#73552=CARTESIAN_POINT('Ctrl Pts',(87.6523647345522,50.1330627636406,13.2843600048799));
#73553=CARTESIAN_POINT('Ctrl Pts',(87.6629021951891,50.1341568571783,13.2874124012293));
#73554=CARTESIAN_POINT('Ctrl Pts',(87.6902678589796,50.1369997060255,13.2949565643126));
#73555=CARTESIAN_POINT('Ctrl Pts',(87.7071505878643,50.1387550291535,13.2992391497411));
#73556=CARTESIAN_POINT('Ctrl Pts',(87.8012166371657,50.1485491745357,13.3210518959149));
#73557=CARTESIAN_POINT('Ctrl Pts',(87.8798028110497,50.1567998306994,13.3316800951234));
#73558=CARTESIAN_POINT('Ctrl Pts',(88.037212816016,50.1734006869207,13.3381494395508));
#73559=CARTESIAN_POINT('Ctrl Pts',(88.1157153056916,50.1817133060103,13.3341044272359));
#73560=CARTESIAN_POINT('Ctrl Pts',(88.2054129762427,50.1910027028717,13.3210904968183));
#73561=CARTESIAN_POINT('Ctrl Pts',(88.2174502242791,50.1922446102772,13.3191667508069));
#73562=CARTESIAN_POINT('Ctrl Pts',(88.2354356132192,50.1940914731074,13.3160261870327));
#73563=CARTESIAN_POINT('Ctrl Pts',(88.2414051997936,50.194703023341,13.3149396551745));
#73564=CARTESIAN_POINT('Ctrl Pts',(88.2517411489544,50.1957591244495,13.3129817636831));
#73565=CARTESIAN_POINT('Ctrl Pts',(88.2561108748048,50.1962047344619,13.3121302022032));
#73566=CARTESIAN_POINT('Ctrl Pts',(88.2664365600203,50.197255703035,13.3100615396305));
#73567=CARTESIAN_POINT('Ctrl Pts',(88.272388399797,50.1978599361106,13.3088246298879));
#73568=CARTESIAN_POINT('Ctrl Pts',(88.2901766777976,50.1996618109895,13.3049944308104));
#73569=CARTESIAN_POINT('Ctrl Pts',(88.3019856901424,50.2008526981427,13.3022743160909));
#73570=CARTESIAN_POINT('Ctrl Pts',(88.3223155981013,50.2028967355451,13.2972840055971));
#73571=CARTESIAN_POINT('Ctrl Pts',(88.3308546986669,50.2037533971276,13.2950934418673));
#73572=CARTESIAN_POINT('Ctrl Pts',(88.3543248069187,50.2061046294642,13.288811402005));
#73573=CARTESIAN_POINT('Ctrl Pts',(88.369205431299,50.2075916242958,13.2845354219099));
#73574=CARTESIAN_POINT('Ctrl Pts',(88.4485676820369,50.2155215360091,13.2601509023413));
#73575=CARTESIAN_POINT('Ctrl Pts',(88.5114509015288,50.2218070896741,13.2351930726608));
#73576=CARTESIAN_POINT('Ctrl Pts',(88.6361172212039,50.2348375539543,13.173803030499));
#73577=CARTESIAN_POINT('Ctrl Pts',(88.697393610511,50.2415669420926,13.1369155606738));
#73578=CARTESIAN_POINT('Ctrl Pts',(88.7681344113431,50.2500313385099,13.0857552260132));
#73579=CARTESIAN_POINT('Ctrl Pts',(88.7808519435079,50.2515825183522,13.0761886797807));
#73580=CARTESIAN_POINT('Ctrl Pts',(88.801032685155,50.254094886571,13.0604056514914));
#73581=CARTESIAN_POINT('Ctrl Pts',(88.8086105592416,50.2550502122455,13.0543378097216));
#73582=CARTESIAN_POINT('Ctrl Pts',(88.8230076339551,50.2568889399281,13.0425362090783));
#73583=CARTESIAN_POINT('Ctrl Pts',(88.829837552629,50.2577717407301,13.036816366452));
#73584=CARTESIAN_POINT('Ctrl Pts',(88.8455418105376,50.259826715194,13.0233809287976));
#73585=CARTESIAN_POINT('Ctrl Pts',(88.8543701089196,50.2610009800321,13.015613138003));
#73586=CARTESIAN_POINT('Ctrl Pts',(88.8828804560114,50.2648575740096,12.9898164663151));
#73587=CARTESIAN_POINT('Ctrl Pts',(88.9021005560537,50.267560399581,12.9712910691408));
#73588=CARTESIAN_POINT('Ctrl Pts',(88.9475185412699,50.2742130459336,12.9246663443893));
#73589=CARTESIAN_POINT('Ctrl Pts',(88.9730511129631,50.2781863677068,12.8959589471802));
#73590=CARTESIAN_POINT('Ctrl Pts',(89.0275875235413,50.2872232905143,12.8287383279579));
#73591=CARTESIAN_POINT('Ctrl Pts',(89.0557794851644,50.2923008789926,12.7896402722075));
#73592=CARTESIAN_POINT('Ctrl Pts',(89.1150213422399,50.3039088817162,12.6967770470786));
#73593=CARTESIAN_POINT('Ctrl Pts',(89.1444953983897,50.3104250348099,12.6421365601638));
#73594=CARTESIAN_POINT('Ctrl Pts',(89.1739587002637,50.3177777033157,12.5764187309047));
#73595=CARTESIAN_POINT('Ctrl Pts',(89.1779462390541,50.3187945622113,12.567235191552));
#73596=CARTESIAN_POINT('Ctrl Pts',(89.1840160766264,50.320376443516,12.5527907890431));
#73597=CARTESIAN_POINT('Ctrl Pts',(89.186172396088,50.3209455401553,12.5475618676405));
#73598=CARTESIAN_POINT('Ctrl Pts',(89.1901873145122,50.3220186595176,12.5376383853029));
#73599=CARTESIAN_POINT('Ctrl Pts',(89.1920528796724,50.3225230402024,12.5329470918492));
#73600=CARTESIAN_POINT('Ctrl Pts',(89.1964714553114,50.3237319166861,12.5216398916832));
#73601=CARTESIAN_POINT('Ctrl Pts',(89.1989971312686,50.3244348074499,12.5150134819995));
#73602=CARTESIAN_POINT('Ctrl Pts',(89.2077239958939,50.3269076760321,12.4915282971825));
#73603=CARTESIAN_POINT('Ctrl Pts',(89.2136233642303,50.3286614086111,12.4745582167289));
#73604=CARTESIAN_POINT('Ctrl Pts',(89.2238518716219,50.3318736059311,12.4429905968366));
#73605=CARTESIAN_POINT('Ctrl Pts',(89.2282822533412,50.3333359160257,12.4284300529639));
#73606=CARTESIAN_POINT('Ctrl Pts',(89.2503729914404,50.3410440870511,12.3508472103654));
#73607=CARTESIAN_POINT('Ctrl Pts',(89.2634051054318,50.3471410737372,12.2866046673119));
#73608=CARTESIAN_POINT('Ctrl Pts',(89.2804878682751,50.3602086205882,12.1482610693548));
#73609=CARTESIAN_POINT('Ctrl Pts',(89.2831223930948,50.3671683498128,12.0742453011175));
#73610=CARTESIAN_POINT('Ctrl Pts',(89.2784875672266,50.3758726795263,11.9845958574865));
#73611=CARTESIAN_POINT('Ctrl Pts',(89.2773726110597,50.3774182246551,11.9687800233279));
#73612=CARTESIAN_POINT('Ctrl Pts',(89.2750999486658,50.3799229114105,11.9433412818497));
#73613=CARTESIAN_POINT('Ctrl Pts',(89.2741276050075,50.3808762400798,11.933703054076));
#73614=CARTESIAN_POINT('Ctrl Pts',(89.2720506654689,50.3827120398874,11.9152339159228));
#73615=CARTESIAN_POINT('Ctrl Pts',(89.2709633065944,50.3835939179016,11.9064016016141));
#73616=CARTESIAN_POINT('Ctrl Pts',(89.2682238289021,50.3856480307401,11.8859263375));
#73617=CARTESIAN_POINT('Ctrl Pts',(89.2665026666512,50.3868223663914,11.8742936881538));
#73618=CARTESIAN_POINT('Ctrl Pts',(89.2603393668592,50.390684237341,11.8362909932978));
#73619=CARTESIAN_POINT('Ctrl Pts',(89.255226247977,50.3933924052873,11.810039356906));
#73620=CARTESIAN_POINT('Ctrl Pts',(89.240741393767,50.4000599490987,11.7464415016833));
#73621=CARTESIAN_POINT('Ctrl Pts',(89.2304931157282,50.4040430247816,11.7093245290532));
#73622=CARTESIAN_POINT('Ctrl Pts',(89.2035935531212,50.4131144433267,11.6267257177769));
#73623=CARTESIAN_POINT('Ctrl Pts',(89.1859939151048,50.4182171604065,11.5816137574962));
#73624=CARTESIAN_POINT('Ctrl Pts',(89.1399589598822,50.4298819883382,11.4809967120988));
#73625=CARTESIAN_POINT('Ctrl Pts',(89.1099196617483,50.4364297026322,11.4263476385792));
#73626=CARTESIAN_POINT('Ctrl Pts',(89.0705327381305,50.4438116426284,11.3657210545662));
#73627=CARTESIAN_POINT('Ctrl Pts',(89.0649793304309,50.444828641422,11.3573902213326));
#73628=CARTESIAN_POINT('Ctrl Pts',(89.0561409434015,50.4464096525536,11.3444653296272));
#73629=CARTESIAN_POINT('Ctrl Pts',(89.0529230629831,50.4469777618668,11.3398263241406));
#73630=CARTESIAN_POINT('Ctrl Pts',(89.0467769061642,50.4480485729273,11.3310907859019));
#73631=CARTESIAN_POINT('Ctrl Pts',(89.0438551719068,50.4485516360892,11.3269901569517));
#73632=CARTESIAN_POINT('Ctrl Pts',(89.0367791852879,50.449755976069,11.3171830134152));
#73633=CARTESIAN_POINT('Ctrl Pts',(89.0326015969653,50.4504556648391,11.3114935374574));
#73634=CARTESIAN_POINT('Ctrl Pts',(89.017727967652,50.4529085512158,11.2915871209789));
#73635=CARTESIAN_POINT('Ctrl Pts',(89.0067800549273,50.4546457966983,11.2775593199254));
#73636=CARTESIAN_POINT('Ctrl Pts',(88.9860543362218,50.4578225300462,11.2521237586053));
#73637=CARTESIAN_POINT('Ctrl Pts',(88.9763624170447,50.4592658959712,11.240651012034));
#73638=CARTESIAN_POINT('Ctrl Pts',(88.9243675354584,50.4668098088022,11.1812718042929));
#73639=CARTESIAN_POINT('Ctrl Pts',(88.8786931270231,50.47276705523,11.1364331914181));
#73640=CARTESIAN_POINT('Ctrl Pts',(88.7765492036836,50.4852895618523,11.0502768623177));
#73641=CARTESIAN_POINT('Ctrl Pts',(88.7196639181814,50.491841812351,11.0098029501408));
#73642=CARTESIAN_POINT('Ctrl Pts',(88.6447652973133,50.5002531834599,10.9652977413729));
#73643=CARTESIAN_POINT('Ctrl Pts',(88.629597446969,50.5019458217325,10.9567024548141));
#73644=CARTESIAN_POINT('Ctrl Pts',(88.6045745914689,50.5047248157208,10.9431953406822));
#73645=CARTESIAN_POINT('Ctrl Pts',(88.5948236951881,50.5058044861767,10.9380944308729));
#73646=CARTESIAN_POINT('Ctrl Pts',(88.5771532202644,50.5077561733276,10.9291411387469));
#73647=CARTESIAN_POINT('Ctrl Pts',(88.5692573981834,50.5086265332205,10.9252431430309));
#73648=CARTESIAN_POINT('Ctrl Pts',(88.5522284441692,50.5105004471694,10.917055449912));
#73649=CARTESIAN_POINT('Ctrl Pts',(88.5430835214305,50.5115048359098,10.9127919012208));
#73650=CARTESIAN_POINT('Ctrl Pts',(88.5176535060523,50.5142932829565,10.9013027759149));
#73651=CARTESIAN_POINT('Ctrl Pts',(88.5012664623239,50.5160850951454,10.8943105735418));
#73652=CARTESIAN_POINT('Ctrl Pts',(88.4641530742585,50.5201346310081,10.8793894650232));
#73653=CARTESIAN_POINT('Ctrl Pts',(88.4433556405824,50.522398066054,10.8716546901673));
#73654=CARTESIAN_POINT('Ctrl Pts',(88.373170963431,50.530020994298,10.8476255774668));
#73655=CARTESIAN_POINT('Ctrl Pts',(88.3229928274774,50.5354484554071,10.8338218043469));
#73656=CARTESIAN_POINT('Ctrl Pts',(88.1902441127786,50.5497156973191,10.8059323301311));
#73657=CARTESIAN_POINT('Ctrl Pts',(88.1068658778822,50.5585974207116,10.7968620043451));
#73658=CARTESIAN_POINT('Ctrl Pts',(88.0112103798305,50.5684156491252,10.7959434690102));
#73659=CARTESIAN_POINT('Ctrl Pts',(87.9992242987896,50.5696389376938,10.7959980292704));
#73660=CARTESIAN_POINT('Ctrl Pts',(87.9811292404922,50.5714735958391,10.7963366223104));
#73661=CARTESIAN_POINT('Ctrl Pts',(87.9750191195292,50.5720910150153,10.7964950820435));
#73662=CARTESIAN_POINT('Ctrl Pts',(87.9638473666615,50.5732158282852,10.7968655354197));
#73663=CARTESIAN_POINT('Ctrl Pts',(87.9587854314221,50.5737239444895,10.7970637117246));
#73664=CARTESIAN_POINT('Ctrl Pts',(87.9481710785332,50.574786056042,10.7975428937645));
#73665=CARTESIAN_POINT('Ctrl Pts',(87.9426191316844,50.5753397099833,10.7978300725215));
#73666=CARTESIAN_POINT('Ctrl Pts',(87.9274763089576,50.5768450851812,10.7987130843112));
#73667=CARTESIAN_POINT('Ctrl Pts',(87.9178896893916,50.5777929552151,10.7993813422276));
#73668=CARTESIAN_POINT('Ctrl Pts',(87.8599047605607,50.583500309318,10.8040852573779));
#73669=CARTESIAN_POINT('Ctrl Pts',(87.8117546841063,50.5881309514798,10.8107862428404));
#73670=CARTESIAN_POINT('Ctrl Pts',(87.656578052346,50.6030622271736,10.8415409595869));
#73671=CARTESIAN_POINT('Ctrl Pts',(87.552277979746,50.6131514530036,10.8766778297455));
#73672=CARTESIAN_POINT('Ctrl Pts',(87.4350904074372,50.6257165006223,10.9338953159463));
#73673=CARTESIAN_POINT('Ctrl Pts',(87.416622740002,50.6277343804381,10.9434812112058));
#73674=CARTESIAN_POINT('Ctrl Pts',(87.3890177082363,50.6308148341375,10.9586821824363));
#73675=CARTESIAN_POINT('Ctrl Pts',(87.3797014794857,50.6318658009791,10.9639669328338));
#73676=CARTESIAN_POINT('Ctrl Pts',(87.3629927282394,50.6337722495248,10.9737265768937));
#73677=CARTESIAN_POINT('Ctrl Pts',(87.355576812171,50.6346262081228,10.9781603562039));
#73678=CARTESIAN_POINT('Ctrl Pts',(87.3398463128581,50.6364548397345,10.987784440479));
#73679=CARTESIAN_POINT('Ctrl Pts',(87.3315454862454,50.6374302453875,10.9929959858024));
#73680=CARTESIAN_POINT('Ctrl Pts',(87.3145643725677,50.6394478998342,11.0039333651496));
#73681=CARTESIAN_POINT('Ctrl Pts',(87.3058924631122,50.6404905207432,11.0096707592265));
#73682=CARTESIAN_POINT('Ctrl Pts',(87.2626117579527,50.6457575760369,11.0390759731378));
#73683=CARTESIAN_POINT('Ctrl Pts',(87.2291246874004,50.6500407490533,11.0643374292269));
#73684=CARTESIAN_POINT('Ctrl Pts',(87.1410672345652,50.661911715154,11.1378738561848));
#73685=CARTESIAN_POINT('Ctrl Pts',(87.0893051868982,50.6695952362075,11.1892575459361));
#73686=CARTESIAN_POINT('Ctrl Pts',(87.0057996198002,50.6831997367175,11.2877665315057));
#73687=CARTESIAN_POINT('Ctrl Pts',(86.9722584683398,50.6891095307555,11.3331336162015));
#73688=CARTESIAN_POINT('Ctrl Pts',(86.9364755486907,50.6958781514125,11.3889505702609));
#73689=CARTESIAN_POINT('Ctrl Pts',(86.9312110986664,50.6968873805576,11.3973785243914));
#73690=CARTESIAN_POINT('Ctrl Pts',(86.9231190805357,50.6984591494907,11.4106780874535));
#73691=CARTESIAN_POINT('Ctrl Pts',(86.9202242573422,50.6990257076263,11.4155078880149));
#73692=CARTESIAN_POINT('Ctrl Pts',(86.9147971950766,50.7000958460839,11.4247006517141));
#73693=CARTESIAN_POINT('Ctrl Pts',(86.9122587913744,50.7005997714842,11.4290594988228));
#73694=CARTESIAN_POINT('Ctrl Pts',(86.9062093966164,50.7018091830133,11.4395910708417));
#73695=CARTESIAN_POINT('Ctrl Pts',(86.9027240679784,50.7025130499213,11.4457783532729));
#73696=CARTESIAN_POINT('Ctrl Pts',(86.8905610885781,50.7049960698484,11.4678004760827));
#73697=CARTESIAN_POINT('Ctrl Pts',(86.8821687623422,50.7067587701328,11.4837919770318));
#73698=CARTESIAN_POINT('Ctrl Pts',(86.871357951743,50.7091064374567,11.5055052232116));
#73699=CARTESIAN_POINT('Ctrl Pts',(86.8686368482392,50.7097043859978,11.5110722331004));
#73700=CARTESIAN_POINT('Ctrl Pts',(86.857612617095,50.7121572463431,11.534051085486));
#73701=CARTESIAN_POINT('Ctrl Pts',(86.8496654974237,50.7139980522281,11.5516320662685));
#73702=CARTESIAN_POINT('Ctrl Pts',(86.8129648770841,50.7229039802973,11.638014589817));
#73703=CARTESIAN_POINT('Ctrl Pts',(86.7899072459362,50.7298164424287,11.7090780399915));
#73704=CARTESIAN_POINT('Ctrl Pts',(86.7665956722931,50.739623894063,11.810592140147));
#73705=CARTESIAN_POINT('Ctrl Pts',(86.7609840665396,50.7424225527554,11.8396479177557));
#73706=CARTESIAN_POINT('Ctrl Pts',(86.7515192764045,50.7482422335109,11.89988575983));
#73707=CARTESIAN_POINT('Ctrl Pts',(86.7477983743734,50.7512643137505,11.931066976616));
#73708=CARTESIAN_POINT('Ctrl Pts',(86.7442145865341,50.7555415829047,11.974832357443));
#73709=CARTESIAN_POINT('Ctrl Pts',(86.7433772602529,50.7567667183457,11.9873273528142));
#73710=CARTESIAN_POINT('Ctrl Pts',(86.7422604385822,50.7588738081213,12.0087340827899));
#73711=CARTESIAN_POINT('Ctrl Pts',(86.7418897624083,50.7597528742209,12.0176403612404));
#73712=CARTESIAN_POINT('Ctrl Pts',(86.7413908361932,50.7613422019641,12.0336941723447));
#73713=CARTESIAN_POINT('Ctrl Pts',(86.7412291216526,50.7620513840103,12.040840379757));
#73714=CARTESIAN_POINT('Ctrl Pts',(86.7410409837832,50.76337102007,12.0541039224022));
#73715=CARTESIAN_POINT('Ctrl Pts',(86.7409984184484,50.7639809463774,12.0602208479458));
#73716=CARTESIAN_POINT('Ctrl Pts',(86.7410000448951,50.7645922586327,12.0663376885773));
#73717=CARTESIAN_POINT('Ctrl Pts',(86.7410000447486,50.7645922035288,12.0663371372026));
#73718=CARTESIAN_POINT('Ctrl Pts',(86.7410023456166,50.7654584163238,12.0750045347553));
#73719=CARTESIAN_POINT('Ctrl Pts',(86.7410933751595,50.7663273812323,12.0836714430582));
#73720=CARTESIAN_POINT('Ctrl Pts',(86.7415718652515,50.7686481774774,12.1067402439223));
#73721=CARTESIAN_POINT('Ctrl Pts',(86.7421156803795,50.7701047204387,12.1211370738178));
#73722=CARTESIAN_POINT('Ctrl Pts',(86.7468349430576,50.7788657526092,12.2072188902602));
#73723=CARTESIAN_POINT('Ctrl Pts',(86.7568383137963,50.7863417879925,12.2784392447491));
#73724=CARTESIAN_POINT('Ctrl Pts',(86.7892680712375,50.8016896527302,12.4206198309249));
#73725=CARTESIAN_POINT('Ctrl Pts',(86.8120207969228,50.8095380783809,12.4912466070921));
#73726=CARTESIAN_POINT('Ctrl Pts',(86.8477272851518,50.8190228295637,12.5759159671575));
#73727=CARTESIAN_POINT('Ctrl Pts',(86.8549989752535,50.8208493164447,12.5921933549002));
#73728=CARTESIAN_POINT('Ctrl Pts',(86.8656287469066,50.8233747536019,12.6147026656477));
#73729=CARTESIAN_POINT('Ctrl Pts',(86.868699284808,50.8240887231853,12.6210666692601));
#73730=CARTESIAN_POINT('Ctrl Pts',(86.8740497445912,50.8253062984407,12.6319235754041));
#73731=CARTESIAN_POINT('Ctrl Pts',(86.876303523269,50.8258114325395,12.6364290376006));
#73732=CARTESIAN_POINT('Ctrl Pts',(86.8811389028331,50.8268788338796,12.6459532297317));
#73733=CARTESIAN_POINT('Ctrl Pts',(86.8837272229446,50.827440679765,12.6509683224287));
#73734=CARTESIAN_POINT('Ctrl Pts',(86.8909961472493,50.8289929786911,12.6648250543686));
#73735=CARTESIAN_POINT('Ctrl Pts',(86.8957480900361,50.829979168734,12.6736292259547));
#73736=CARTESIAN_POINT('Ctrl Pts',(86.9307070500633,50.8370401017552,12.7366074123193));
#73737=CARTESIAN_POINT('Ctrl Pts',(86.964748915361,50.8429027571994,12.788571029944));
#73738=CARTESIAN_POINT('Ctrl Pts',(87.0316113988497,50.8532345390526,12.8759374488599));
#73739=CARTESIAN_POINT('Ctrl Pts',(87.0628969375233,50.8577090726089,12.9123458238389));
#73740=CARTESIAN_POINT('Ctrl Pts',(87.1230896966267,50.8658744272791,12.9748574814305));
#73741=CARTESIAN_POINT('Ctrl Pts',(87.1512780495804,50.8695470862058,13.0015663082118));
#73742=CARTESIAN_POINT('Ctrl Pts',(87.1806428354228,50.8732662532979,13.0269406741497));
#73743=CARTESIAN_POINT('',(86.7410003148723,50.93532359951,12.0668943017129));
#73744=CARTESIAN_POINT('Ctrl Pts',(87.1806428354228,51.0436650276944,13.0269406741497));
#73745=CARTESIAN_POINT('Ctrl Pts',(87.1430769411697,51.0387322644776,12.9944796593588));
#73746=CARTESIAN_POINT('Ctrl Pts',(87.1073801397486,51.0337995012609,12.9597803455295));
#73747=CARTESIAN_POINT('Ctrl Pts',(87.0738248751965,51.0288667380441,12.9230897184365));
#73748=CARTESIAN_POINT('Ctrl Pts',(87.0402848627672,51.0239362169528,12.8864157686058));
#73749=CARTESIAN_POINT('Ctrl Pts',(87.0088848274002,51.0190056958614,12.8477527031886));
#73750=CARTESIAN_POINT('Ctrl Pts',(86.9798597720419,51.01407517477,12.8073837267478));
#73751=CARTESIAN_POINT('Ctrl Pts',(86.9494169468044,51.0089038154027,12.7650428705588));
#73752=CARTESIAN_POINT('Ctrl Pts',(86.9215875510066,51.0037324560354,12.7208256290176));
#73753=CARTESIAN_POINT('Ctrl Pts',(86.8965925656136,50.998561096668,12.6750944673729));
#73754=CARTESIAN_POINT('Ctrl Pts',(86.8727362769691,50.9936253289606,12.6314466806232));
#73755=CARTESIAN_POINT('Ctrl Pts',(86.8514618982502,50.9886895612531,12.5864204923266));
#73756=CARTESIAN_POINT('Ctrl Pts',(86.8329135745309,50.9837537935456,12.5403546923193));
#73757=CARTESIAN_POINT('Ctrl Pts',(86.8143526726114,50.9788146787392,12.4942576536479));
#73758=CARTESIAN_POINT('Ctrl Pts',(86.798521676003,50.9738755639328,12.4471201205344));
#73759=CARTESIAN_POINT('Ctrl Pts',(86.7855151215509,50.9689364491264,12.3992968837125));
#73760=CARTESIAN_POINT('Ctrl Pts',(86.7724856954086,50.9639886490141,12.3513895509634));
#73761=CARTESIAN_POINT('Ctrl Pts',(86.7622907226357,50.9590408489019,12.3027946460171));
#73762=CARTESIAN_POINT('Ctrl Pts',(86.7549735022767,50.9540930487896,12.2538761214657));
#73763=CARTESIAN_POINT('Ctrl Pts',(86.753951008858,50.9534016533138,12.2470403468198));
#73764=CARTESIAN_POINT('Ctrl Pts',(86.7529846253408,50.9527102578379,12.2401982568247));
#73765=CARTESIAN_POINT('Ctrl Pts',(86.752074388931,50.9520188623621,12.2333508464107));
#73766=CARTESIAN_POINT('Ctrl Pts',(86.7447478362555,50.9464537747447,12.1782355900387));
#73767=CARTESIAN_POINT('Ctrl Pts',(86.7410395617865,50.9408886871273,12.1226289244708));
#73768=CARTESIAN_POINT('Ctrl Pts',(86.7410003148723,50.93532359951,12.0668943017129));
#73769=CARTESIAN_POINT('Ctrl Pts',(87.1806428354213,50.2511271317289,13.0269406741484));
#73770=CARTESIAN_POINT('Ctrl Pts',(87.1933607595619,50.2528272069875,13.0379303426189));
#73771=CARTESIAN_POINT('Ctrl Pts',(87.2062963695742,50.2545169653573,13.0486671138574));
#73772=CARTESIAN_POINT('Ctrl Pts',(87.2272751080988,50.2571971502778,13.0653876246349));
#73773=CARTESIAN_POINT('Ctrl Pts',(87.2351819200797,50.2581941239906,13.0715379913703));
#73774=CARTESIAN_POINT('Ctrl Pts',(87.2494778044442,50.2599738176597,13.0823891171531));
#73775=CARTESIAN_POINT('Ctrl Pts',(87.2558395914037,50.2607578654046,13.0871247016414));
#73776=CARTESIAN_POINT('Ctrl Pts',(87.2708688789396,50.2625920355324,13.0980949111228));
#73777=CARTESIAN_POINT('Ctrl Pts',(87.279571595843,50.2636402346878,13.1042805442905));
#73778=CARTESIAN_POINT('Ctrl Pts',(87.3054085375234,50.2667130527024,13.12215857191));
#73779=CARTESIAN_POINT('Ctrl Pts',(87.322753138677,50.2687260882595,13.1335423244838));
#73780=CARTESIAN_POINT('Ctrl Pts',(87.3634020759689,50.2733403115177,13.1588186109842));
#73781=CARTESIAN_POINT('Ctrl Pts',(87.3868884976003,50.2759307516124,13.1723998501801));
#73782=CARTESIAN_POINT('Ctrl Pts',(87.4775169115569,50.2856889010736,13.2210013593576));
#73783=CARTESIAN_POINT('Ctrl Pts',(87.547306137468,50.2927144311646,13.250745019563));
#73784=CARTESIAN_POINT('Ctrl Pts',(87.6721704028295,50.3050655083306,13.291226520702));
#73785=CARTESIAN_POINT('Ctrl Pts',(87.7260675111065,50.3103349249922,13.3048691044664));
#73786=CARTESIAN_POINT('Ctrl Pts',(87.7904358936943,50.316752025255,13.3167397925055));
#73787=CARTESIAN_POINT('Ctrl Pts',(87.8002188967009,50.3177306749078,13.3184255896165));
#73788=CARTESIAN_POINT('Ctrl Pts',(87.8155731595856,50.3192734131746,13.3208864405542));
#73789=CARTESIAN_POINT('Ctrl Pts',(87.8211318773399,50.3198333154589,13.3217395112493));
#73790=CARTESIAN_POINT('Ctrl Pts',(87.8316835314354,50.3208990876806,13.3232871652754));
#73791=CARTESIAN_POINT('Ctrl Pts',(87.8366752082008,50.3214045524627,13.3239889800932));
#73792=CARTESIAN_POINT('Ctrl Pts',(87.8487027672629,50.3226254259054,13.325607062744));
#73793=CARTESIAN_POINT('Ctrl Pts',(87.8557422917161,50.3233423875154,13.3264941013898));
#73794=CARTESIAN_POINT('Ctrl Pts',(87.8806906429315,50.3258910450536,13.3294256529803));
#73795=CARTESIAN_POINT('Ctrl Pts',(87.8986338907768,50.3277381139815,13.3311476790901));
#73796=CARTESIAN_POINT('Ctrl Pts',(87.9318608953387,50.3311779743658,13.3336241578025));
#73797=CARTESIAN_POINT('Ctrl Pts',(87.9471342247533,50.3327667472074,13.3344853623832));
#73798=CARTESIAN_POINT('Ctrl Pts',(88.0284505978251,50.3412555789819,13.3375982472763));
#73799=CARTESIAN_POINT('Ctrl Pts',(88.0945772527446,50.3482573087147,13.3349685354004));
#73800=CARTESIAN_POINT('Ctrl Pts',(88.2328883340389,50.3628884955099,13.3186066593674));
#73801=CARTESIAN_POINT('Ctrl Pts',(88.3047143759776,50.3704751140489,13.303737636321));
#73802=CARTESIAN_POINT('Ctrl Pts',(88.3900694645436,50.3794710610343,13.2782119837858));
#73803=CARTESIAN_POINT('Ctrl Pts',(88.4051793312595,50.3810633500663,13.2733832307786));
#73804=CARTESIAN_POINT('Ctrl Pts',(88.4293645216141,50.3836131183543,13.2651517557138));
#73805=CARTESIAN_POINT('Ctrl Pts',(88.4384976915128,50.384576265869,13.2619262281776));
#73806=CARTESIAN_POINT('Ctrl Pts',(88.4559449078257,50.3864172019866,13.2555390385792));
#73807=CARTESIAN_POINT('Ctrl Pts',(88.4642643365153,50.3872954750221,13.2523939255929));
#73808=CARTESIAN_POINT('Ctrl Pts',(88.4834931184777,50.38932704548,13.2448927943395));
#73809=CARTESIAN_POINT('Ctrl Pts',(88.4943766143245,50.3904781255635,13.2404722384276));
#73810=CARTESIAN_POINT('Ctrl Pts',(88.5297762194812,50.3942281918976,13.2255184943305));
#73811=CARTESIAN_POINT('Ctrl Pts',(88.5540233730338,50.396806280095,13.2143630766783));
#73812=CARTESIAN_POINT('Ctrl Pts',(88.6122499809643,50.4030432885563,13.1853175258539));
#73813=CARTESIAN_POINT('Ctrl Pts',(88.6458049051743,50.4066768378064,13.1666345729477));
#73814=CARTESIAN_POINT('Ctrl Pts',(88.7196479063812,50.4148459089605,13.1210172811799));
#73815=CARTESIAN_POINT('Ctrl Pts',(88.7593428157943,50.419361764589,13.0932421292802));
#73816=CARTESIAN_POINT('Ctrl Pts',(88.8462452540176,50.4297546781969,13.0247187708921));
#73817=CARTESIAN_POINT('Ctrl Pts',(88.8922245497247,50.4356365261322,12.9826332529987));
#73818=CARTESIAN_POINT('Ctrl Pts',(88.9417149479889,50.4427073732877,12.9301571805777));
#73819=CARTESIAN_POINT('Ctrl Pts',(88.9484204601546,50.4436828371823,12.9228785245358));
#73820=CARTESIAN_POINT('Ctrl Pts',(88.9588381586419,50.4452276053274,12.9113017616408));
#73821=CARTESIAN_POINT('Ctrl Pts',(88.9626079806121,50.4457928126501,12.9070555806854));
#73822=CARTESIAN_POINT('Ctrl Pts',(88.9696619846618,50.446862547954,12.8990020891879));
#73823=CARTESIAN_POINT('Ctrl Pts',(88.9729522124265,50.447366622778,12.895200348363));
#73824=CARTESIAN_POINT('Ctrl Pts',(88.9807679078606,50.4485762172832,12.8860604741242));
#73825=CARTESIAN_POINT('Ctrl Pts',(88.985271910514,50.4492832111768,12.8807043711685));
#73826=CARTESIAN_POINT('Ctrl Pts',(89.0008089867568,50.4517562628244,12.8619147941696));
#73827=CARTESIAN_POINT('Ctrl Pts',(89.0116095675138,50.4535365558507,12.8482931531908));
#73828=CARTESIAN_POINT('Ctrl Pts',(89.0382663290889,50.4580815023244,12.8132184416301));
#73829=CARTESIAN_POINT('Ctrl Pts',(89.0537319998744,50.4608624108807,12.7914800106823));
#73830=CARTESIAN_POINT('Ctrl Pts',(89.1247048533258,50.4742988958354,12.6847592195526));
#73831=CARTESIAN_POINT('Ctrl Pts',(89.1705868038097,50.4850736822582,12.5937940156327));
#73832=CARTESIAN_POINT('Ctrl Pts',(89.2145924637585,50.4983692545979,12.4722447051878));
#73833=CARTESIAN_POINT('Ctrl Pts',(89.2231797260878,50.5011973652224,12.4458554832027));
#73834=CARTESIAN_POINT('Ctrl Pts',(89.2352430399156,50.5055758519852,12.4041911337756));
#73835=CARTESIAN_POINT('Ctrl Pts',(89.2393124030434,50.5071445229759,12.3890989946561));
#73836=CARTESIAN_POINT('Ctrl Pts',(89.2454385857783,50.5096657737448,12.3645870303443));
#73837=CARTESIAN_POINT('Ctrl Pts',(89.2476684392079,50.5106237952912,12.3552127613446));
#73838=CARTESIAN_POINT('Ctrl Pts',(89.251753924701,50.5124608699196,12.337125495374));
#73839=CARTESIAN_POINT('Ctrl Pts',(89.2536249877953,50.5133403633046,12.3284166263606));
#73840=CARTESIAN_POINT('Ctrl Pts',(89.2577720109134,50.5153835175523,12.3080744613313));
#73841=CARTESIAN_POINT('Ctrl Pts',(89.2599770783257,50.5165448767635,12.296427370355));
#73842=CARTESIAN_POINT('Ctrl Pts',(89.2667295387395,50.5203696949251,12.2578105425165));
#73843=CARTESIAN_POINT('Ctrl Pts',(89.2705691621717,50.523011032483,12.2307232108686));
#73844=CARTESIAN_POINT('Ctrl Pts',(89.277838373264,50.5294413936635,12.16399184886));
#73845=CARTESIAN_POINT('Ctrl Pts',(89.2802860215701,50.5332027767716,12.1242697655643));
#73846=CARTESIAN_POINT('Ctrl Pts',(89.2813758046904,50.5402405372658,12.0494452071396));
#73847=CARTESIAN_POINT('Ctrl Pts',(89.2804349581069,50.543518450964,12.0143889623366));
#73848=CARTESIAN_POINT('Ctrl Pts',(89.2733458687954,50.5532633789349,11.9106491614456));
#73849=CARTESIAN_POINT('Ctrl Pts',(89.2630569744751,50.5597314506678,11.8423915764317));
#73850=CARTESIAN_POINT('Ctrl Pts',(89.2443826145806,50.5676905537196,11.762968136109));
#73851=CARTESIAN_POINT('Ctrl Pts',(89.2412938357436,50.568936485229,11.7506620586212));
#73852=CARTESIAN_POINT('Ctrl Pts',(89.2364250819374,50.5708048354054,11.7324259174487));
#73853=CARTESIAN_POINT('Ctrl Pts',(89.2347850929626,50.5714197401356,11.7264586323839));
#73854=CARTESIAN_POINT('Ctrl Pts',(89.2317521452105,50.5725320533066,11.7157303801249));
#73855=CARTESIAN_POINT('Ctrl Pts',(89.230374804627,50.5730285670758,11.7109652282235));
#73856=CARTESIAN_POINT('Ctrl Pts',(89.2271971618092,50.5741550208695,11.7002082487243));
#73857=CARTESIAN_POINT('Ctrl Pts',(89.2253804954412,50.5747858442692,11.6942216414149));
#73858=CARTESIAN_POINT('Ctrl Pts',(89.2196398336134,50.5767391296854,11.6757950466257));
#73859=CARTESIAN_POINT('Ctrl Pts',(89.2155685485842,50.5780692034371,11.6634025372838));
#73860=CARTESIAN_POINT('Ctrl Pts',(89.2054431682607,50.581249000772,11.6341114772262));
#73861=CARTESIAN_POINT('Ctrl Pts',(89.1992203433359,50.583105639662,11.617274583164));
#73862=CARTESIAN_POINT('Ctrl Pts',(89.1737815846719,50.590327535794,11.5526892374117));
#73863=CARTESIAN_POINT('Ctrl Pts',(89.1520274808799,50.5957607627426,11.5059959026813));
#73864=CARTESIAN_POINT('Ctrl Pts',(89.0863105150756,50.6102964936842,11.3847672435156));
#73865=CARTESIAN_POINT('Ctrl Pts',(89.0374596709513,50.6193315366198,11.3131665459124));
#73866=CARTESIAN_POINT('Ctrl Pts',(88.9705877513366,50.6298472415509,11.2339012736109));
#73867=CARTESIAN_POINT('Ctrl Pts',(88.9592085198891,50.6315838450733,11.2209570303957));
#73868=CARTESIAN_POINT('Ctrl Pts',(88.9401741325998,50.6344060316017,11.2001736327621));
#73869=CARTESIAN_POINT('Ctrl Pts',(88.9326752626552,50.6354979334889,11.1921953328077));
#73870=CARTESIAN_POINT('Ctrl Pts',(88.9189614076943,50.6374599564657,11.1779777022235));
#73871=CARTESIAN_POINT('Ctrl Pts',(88.9127830440334,50.6383315712694,11.1717042599807));
#73872=CARTESIAN_POINT('Ctrl Pts',(88.8993522803582,50.640200580341,11.1583475461461));
#73873=CARTESIAN_POINT('Ctrl Pts',(88.8920792528265,50.641196991888,11.1512857735986));
#73874=CARTESIAN_POINT('Ctrl Pts',(88.8716371367725,50.6439555543264,11.1319074999547));
#73875=CARTESIAN_POINT('Ctrl Pts',(88.8582886754994,50.6457095340881,11.1197827639675));
#73876=CARTESIAN_POINT('Ctrl Pts',(88.827685685288,50.6496321805462,11.0931524624263));
#73877=CARTESIAN_POINT('Ctrl Pts',(88.8102938984672,50.6517942513949,11.0788134761274));
#73878=CARTESIAN_POINT('Ctrl Pts',(88.7504328539674,50.6590354612147,11.0320797101052));
#73879=CARTESIAN_POINT('Ctrl Pts',(88.7063036785166,50.6640443439526,11.0019014526015));
#73880=CARTESIAN_POINT('Ctrl Pts',(88.5883545841602,50.6769025714163,10.9317203834137));
#73881=CARTESIAN_POINT('Ctrl Pts',(88.512254065804,50.6847074000522,10.8960995081019));
#73882=CARTESIAN_POINT('Ctrl Pts',(88.4222478726026,50.6940316630985,10.8643717289543));
#73883=CARTESIAN_POINT('Ctrl Pts',(88.4112251605279,50.6951752405397,10.8606556092584));
#73884=CARTESIAN_POINT('Ctrl Pts',(88.39439041845,50.6969267161178,10.8552364210392));
#73885=CARTESIAN_POINT('Ctrl Pts',(88.3886141778352,50.6975285445198,10.8534225038224));
#73886=CARTESIAN_POINT('Ctrl Pts',(88.3785533584201,50.6985786807131,10.8503419517906));
#73887=CARTESIAN_POINT('Ctrl Pts',(88.3742746963736,50.6990258940004,10.8490565115931));
#73888=CARTESIAN_POINT('Ctrl Pts',(88.3641013667044,50.7000907055486,10.8460585654577));
#73889=CARTESIAN_POINT('Ctrl Pts',(88.3582011108808,50.7007094072312,10.8443662325694));
#73890=CARTESIAN_POINT('Ctrl Pts',(88.3403197923637,50.7025874454875,10.8393774465212));
#73891=CARTESIAN_POINT('Ctrl Pts',(88.3283029698728,50.7038536018419,10.8362141658418));
#73892=CARTESIAN_POINT('Ctrl Pts',(88.2674624978797,50.7102785868745,10.8211496635686));
#73893=CARTESIAN_POINT('Ctrl Pts',(88.2180150528518,50.7155454192613,10.8119789597148));
#73894=CARTESIAN_POINT('Ctrl Pts',(88.0782726214735,50.7303768945394,10.7945519608485));
#73895=CARTESIAN_POINT('Ctrl Pts',(87.9874236354046,50.7399365560761,10.7929894504075));
#73896=CARTESIAN_POINT('Ctrl Pts',(87.8681451949257,50.7522120735621,10.8037235797317));
#73897=CARTESIAN_POINT('Ctrl Pts',(87.8392161648363,50.7551702834468,10.8073340702816));
#73898=CARTESIAN_POINT('Ctrl Pts',(87.7993527411348,50.7592251288385,10.8137095501827));
#73899=CARTESIAN_POINT('Ctrl Pts',(87.7882951149303,50.7603476224732,10.8156286600132));
#73900=CARTESIAN_POINT('Ctrl Pts',(87.7691461853345,50.762288154719,10.8192141562275));
#73901=CARTESIAN_POINT('Ctrl Pts',(87.7610432345023,50.7631082581969,10.8208133346681));
#73902=CARTESIAN_POINT('Ctrl Pts',(87.7441107979463,50.7648201708318,10.824327030018));
#73903=CARTESIAN_POINT('Ctrl Pts',(87.7352849389046,50.7657114411779,10.8262569515287));
#73904=CARTESIAN_POINT('Ctrl Pts',(87.7141703174142,50.7678417775888,10.8311106614747));
#73905=CARTESIAN_POINT('Ctrl Pts',(87.7019028786637,50.769077928063,10.8341239768997));
#73906=CARTESIAN_POINT('Ctrl Pts',(87.6581701957626,50.7734820319056,10.8455607238672));
#73907=CARTESIAN_POINT('Ctrl Pts',(87.6269844028073,50.7766171820344,10.8550114260545));
#73908=CARTESIAN_POINT('Ctrl Pts',(87.5472197120588,50.7846678443899,10.8825758630856));
#73909=CARTESIAN_POINT('Ctrl Pts',(87.4993246728235,50.7895319408776,10.902482063593));
#73910=CARTESIAN_POINT('Ctrl Pts',(87.3783376234381,50.8021533318055,10.9616873993773));
#73911=CARTESIAN_POINT('Ctrl Pts',(87.307657228934,50.8098615479298,11.0053059913324));
#73912=CARTESIAN_POINT('Ctrl Pts',(87.2317311902766,50.8191515321603,11.0631049954354));
#73913=CARTESIAN_POINT('Ctrl Pts',(87.2218356063798,50.8203841734155,11.0708729803637));
#73914=CARTESIAN_POINT('Ctrl Pts',(87.2071927750937,50.8222442295094,11.0827232770878));
#73915=CARTESIAN_POINT('Ctrl Pts',(87.2023571983565,50.8228645204907,11.0866961748154));
#73916=CARTESIAN_POINT('Ctrl Pts',(87.1936715635788,50.823990096353,11.0939404589562));
#73917=CARTESIAN_POINT('Ctrl Pts',(87.1898112996983,50.8244944943799,11.0971993802937));
#73918=CARTESIAN_POINT('Ctrl Pts',(87.1818559772851,50.8255428392805,11.1039971514426));
#73919=CARTESIAN_POINT('Ctrl Pts',(87.1777640663151,50.8260869821424,11.1075391683529));
#73920=CARTESIAN_POINT('Ctrl Pts',(87.1675202616545,50.8274613913342,11.1165215246915));
#73921=CARTESIAN_POINT('Ctrl Pts',(87.16139841877,50.8282939675565,11.1219954532139));
#73922=CARTESIAN_POINT('Ctrl Pts',(87.1475748063007,50.8301989646515,11.1345993949217));
#73923=CARTESIAN_POINT('Ctrl Pts',(87.1399075858775,50.8312736297951,11.1417661902698));
#73924=CARTESIAN_POINT('Ctrl Pts',(87.1166108724021,50.8345930437667,11.1640897565982));
#73925=CARTESIAN_POINT('Ctrl Pts',(87.1012824287929,50.8368536336616,11.1795532795196));
#73926=CARTESIAN_POINT('Ctrl Pts',(87.0346016725022,50.8470131674831,11.250373181455));
#73927=CARTESIAN_POINT('Ctrl Pts',(86.9878484774379,50.855025435301,11.309850435194));
#73928=CARTESIAN_POINT('Ctrl Pts',(86.9128489266427,50.8694115247047,11.4250602058156));
#73929=CARTESIAN_POINT('Ctrl Pts',(86.8828829344972,50.875805445719,11.4794043279298));
#73930=CARTESIAN_POINT('Ctrl Pts',(86.8504864413318,50.8836373421491,11.5499072950956));
#73931=CARTESIAN_POINT('Ctrl Pts',(86.8442337816867,50.8852031886813,11.5642031810678));
#73932=CARTESIAN_POINT('Ctrl Pts',(86.8345504019281,50.887721023568,11.5875033294502));
#73933=CARTESIAN_POINT('Ctrl Pts',(86.8309561373216,50.8886784270204,11.596437207851));
#73934=CARTESIAN_POINT('Ctrl Pts',(86.8242327904738,50.8905150375786,11.6137136350366));
#73935=CARTESIAN_POINT('Ctrl Pts',(86.8210892210585,50.8913946796686,11.6220498745539));
#73936=CARTESIAN_POINT('Ctrl Pts',(86.8139637432605,50.8934392516797,11.6415650776602));
#73937=CARTESIAN_POINT('Ctrl Pts',(86.810050207516,50.8946018695847,11.6527683187081));
#73938=CARTESIAN_POINT('Ctrl Pts',(86.8021406192779,50.8970399120771,11.6764731092283));
#73939=CARTESIAN_POINT('Ctrl Pts',(86.7981801392068,50.8983141025145,11.6889851253288));
#73940=CARTESIAN_POINT('Ctrl Pts',(86.7878534175345,50.9017929641555,11.7234578347432));
#73941=CARTESIAN_POINT('Ctrl Pts',(86.7818848923609,50.9039857019889,11.7455333348979));
#73942=CARTESIAN_POINT('Ctrl Pts',(86.7528442359326,50.9157727302543,11.865739128937));
#73943=CARTESIAN_POINT('Ctrl Pts',(86.7409239715871,50.9250457026798,11.9661780945622));
#73944=CARTESIAN_POINT('Ctrl Pts',(86.7410003648342,50.9346029221184,12.0669626415845));
#73945=CARTESIAN_POINT('Origin',(88.011,65.0896,12.066));
#73946=CARTESIAN_POINT('',(86.3066601088578,64.6798399153869,12.0666091481311));
#73947=CARTESIAN_POINT('',(88.8060699928714,64.9396,13.5735272939604));
#73948=CARTESIAN_POINT('Ctrl Pts',(86.306660108858,64.6798399154298,12.0666091487058));
#73949=CARTESIAN_POINT('Ctrl Pts',(86.3066704464735,64.6819963896155,12.095532809473));
#73950=CARTESIAN_POINT('Ctrl Pts',(86.3074170166427,64.6841528638012,12.1244434963871));
#73951=CARTESIAN_POINT('Ctrl Pts',(86.3088981128696,64.6863093379869,12.1533155279848));
#73952=CARTESIAN_POINT('Ctrl Pts',(86.3120611916116,64.6909147765331,12.214975606324));
#73953=CARTESIAN_POINT('Ctrl Pts',(86.3185854995964,64.6955202150793,12.2765881435167));
#73954=CARTESIAN_POINT('Ctrl Pts',(86.3284654841818,64.7001256536254,12.3377580517307));
#73955=CARTESIAN_POINT('Ctrl Pts',(86.3384945128726,64.7048005673273,12.399850736105));
#73956=CARTESIAN_POINT('Ctrl Pts',(86.3519813709746,64.7094754810292,12.461486795159));
#73957=CARTESIAN_POINT('Ctrl Pts',(86.3688652169034,64.714150394731,12.5222545229849));
#73958=CARTESIAN_POINT('Ctrl Pts',(86.3854521571814,64.7187430991839,12.5819536387276));
#73959=CARTESIAN_POINT('Ctrl Pts',(86.4053174346001,64.7233358036367,12.6408142071515));
#73960=CARTESIAN_POINT('Ctrl Pts',(86.4283517349835,64.7279285080896,12.6984549824615));
#73961=CARTESIAN_POINT('Ctrl Pts',(86.4513717033921,64.7325183549551,12.7560598935981));
#73962=CARTESIAN_POINT('Ctrl Pts',(86.4775565967264,64.7371082018206,12.8124460468413));
#73963=CARTESIAN_POINT('Ctrl Pts',(86.506747924809,64.7416980486861,12.8672493556213));
#73964=CARTESIAN_POINT('Ctrl Pts',(86.5359317104231,64.7462867096249,12.9220385042976));
#73965=CARTESIAN_POINT('Ctrl Pts',(86.5681201503177,64.7508753705637,12.975245173118));
#73966=CARTESIAN_POINT('Ctrl Pts',(86.6031083773965,64.7554640315025,13.0265290285061));
#73967=CARTESIAN_POINT('Ctrl Pts',(86.6392375609678,64.7602023274165,13.0794852363583));
#73968=CARTESIAN_POINT('Ctrl Pts',(86.6783520305866,64.7649406233304,13.1303905425967));
#73969=CARTESIAN_POINT('Ctrl Pts',(86.720178601905,64.7696789192444,13.1789038385324));
#73970=CARTESIAN_POINT('Ctrl Pts',(86.760733202724,64.774273120808,13.2259418167618));
#73971=CARTESIAN_POINT('Ctrl Pts',(86.8038368845309,64.7788673223717,13.2707308699209));
#73972=CARTESIAN_POINT('Ctrl Pts',(86.8492022623125,64.7834615239353,13.3129967330768));
#73973=CARTESIAN_POINT('Ctrl Pts',(86.8967019265033,64.7882718670245,13.3572510610425));
#73974=CARTESIAN_POINT('Ctrl Pts',(86.946680901022,64.7930822101136,13.398738486692));
#73975=CARTESIAN_POINT('Ctrl Pts',(86.9987718552393,64.7978925532027,13.43719255342));
#73976=CARTESIAN_POINT('Ctrl Pts',(87.0508628094566,64.8027028962919,13.475646620148));
#73977=CARTESIAN_POINT('Ctrl Pts',(87.1050651763733,64.807513239381,13.5110670434374));
#73978=CARTESIAN_POINT('Ctrl Pts',(87.1609813508699,64.8123235824701,13.543241730974));
#73979=CARTESIAN_POINT('Ctrl Pts',(87.2144523232767,64.8169235703073,13.5740094264566));
#73980=CARTESIAN_POINT('Ctrl Pts',(87.2697035984548,64.8215235581445,13.6019321206037));
#73981=CARTESIAN_POINT('Ctrl Pts',(87.3264006550764,64.8261235459817,13.6268006190831));
#73982=CARTESIAN_POINT('Ctrl Pts',(87.3840296067459,64.8307991410222,13.6520778659519));
#73983=CARTESIAN_POINT('Ctrl Pts',(87.4431518843408,64.8354747360627,13.6741992645683));
#73984=CARTESIAN_POINT('Ctrl Pts',(87.5033875661512,64.8401503311031,13.6929924562216));
#73985=CARTESIAN_POINT('Ctrl Pts',(87.5624893325295,64.8447379097186,13.7114318726807));
#73986=CARTESIAN_POINT('Ctrl Pts',(87.6226624393423,64.8493254883341,13.726667145479));
#73987=CARTESIAN_POINT('Ctrl Pts',(87.6835277454027,64.8539130669496,13.7385838568123));
#73988=CARTESIAN_POINT('Ctrl Pts',(87.7443569176477,64.8584979220641,13.7504934935693));
#73989=CARTESIAN_POINT('Ctrl Pts',(87.8058769765099,64.8630827771787,13.7590883781332));
#73990=CARTESIAN_POINT('Ctrl Pts',(87.8676965928791,64.8676676322932,13.7643047338766));
#73991=CARTESIAN_POINT('Ctrl Pts',(87.9295021218816,64.8722514426175,13.7695199009242));
#73992=CARTESIAN_POINT('Ctrl Pts',(87.9916065666705,64.8768352529417,13.7713580249794));
#73993=CARTESIAN_POINT('Ctrl Pts',(88.0536134849601,64.881419063266,13.769807185834));
#73994=CARTESIAN_POINT('Ctrl Pts',(88.1177769370419,64.8861622935732,13.7682024101745));
#73995=CARTESIAN_POINT('Ctrl Pts',(88.1818353744046,64.8909055238805,13.7629685434884));
#73996=CARTESIAN_POINT('Ctrl Pts',(88.2453521333063,64.8956487541878,13.7541510338873));
#73997=CARTESIAN_POINT('Ctrl Pts',(88.3068136763909,64.9002385074897,13.7456188330066));
#73998=CARTESIAN_POINT('Ctrl Pts',(88.3677675604565,64.9048282607915,13.7337315525005));
#73999=CARTESIAN_POINT('Ctrl Pts',(88.4278283183883,64.9094180140933,13.7185825209621));
#74000=CARTESIAN_POINT('Ctrl Pts',(88.4909016386516,64.9142379829033,13.7026736355134));
#74001=CARTESIAN_POINT('Ctrl Pts',(88.5529892627615,64.9190579517134,13.6831673404478));
#74002=CARTESIAN_POINT('Ctrl Pts',(88.6136655192791,64.9238779205234,13.6602299418441));
#74003=CARTESIAN_POINT('Ctrl Pts',(88.6743417757967,64.9286978893333,13.6372925432403));
#74004=CARTESIAN_POINT('Ctrl Pts',(88.7336061107467,64.9335178581434,13.6109243717016));
#74005=CARTESIAN_POINT('Ctrl Pts',(88.7910626927788,64.9383378269534,13.5813471651522));
#74006=CARTESIAN_POINT('Ctrl Pts',(88.7960779499343,64.9387585513022,13.5787654366271));
#74007=CARTESIAN_POINT('Ctrl Pts',(88.8010804362425,64.9391792756511,13.5761587864509));
#74008=CARTESIAN_POINT('Ctrl Pts',(88.8060699928714,64.9396,13.5735272939604));
#74009=CARTESIAN_POINT('',(87.2157910724421,64.9396,13.5734540116143));
#74010=CARTESIAN_POINT('Origin',(88.011,64.9396,12.066));
#74011=CARTESIAN_POINT('',(86.306311228203,64.8024850845702,12.0672964986124));
#74012=CARTESIAN_POINT('Ctrl Pts',(87.2157910724421,64.9396,13.5734540116144));
#74013=CARTESIAN_POINT('Ctrl Pts',(86.7145593062453,64.8975952518389,13.309045298523));
#74014=CARTESIAN_POINT('Ctrl Pts',(86.3287535439272,64.851890280029,12.7301966984418));
#74015=CARTESIAN_POINT('Ctrl Pts',(86.3044108940433,64.8061853082191,12.1169819374226));
#74016=CARTESIAN_POINT('Ctrl Pts',(86.3047298421322,64.8024850845702,12.0672977013333));
#74017=CARTESIAN_POINT('',(86.3066602867323,64.0087350846259,12.0669886246394));
#74018=CARTESIAN_POINT('Ctrl Pts',(86.306660492924,64.8024850845702,12.0672962329796));
#74019=CARTESIAN_POINT('Ctrl Pts',(86.3066145342196,64.7979795717007,12.0068678711104));
#74020=CARTESIAN_POINT('Ctrl Pts',(86.309786550778,64.7934740588313,11.9462894264899));
#74021=CARTESIAN_POINT('Ctrl Pts',(86.3161980195603,64.7889685459618,11.8859414464744));
#74022=CARTESIAN_POINT('Ctrl Pts',(86.3225985529314,64.7844707177022,11.8256963960686));
#74023=CARTESIAN_POINT('Ctrl Pts',(86.3322275268003,64.7799728894426,11.7656815533077));
#74024=CARTESIAN_POINT('Ctrl Pts',(86.3450544185545,64.7754750611829,11.7062776692192));
#74025=CARTESIAN_POINT('Ctrl Pts',(86.3578692724028,64.7709814540889,11.6469295350653));
#74026=CARTESIAN_POINT('Ctrl Pts',(86.3738759928126,64.7664878469948,11.5881917405843));
#74027=CARTESIAN_POINT('Ctrl Pts',(86.3929924649126,64.7619942399008,11.5304381903082));
#74028=CARTESIAN_POINT('Ctrl Pts',(86.4120986283622,64.7575030560062,11.4727157839144));
#74029=CARTESIAN_POINT('Ctrl Pts',(86.4343110558028,64.7530118721116,11.4159770732769));
#74030=CARTESIAN_POINT('Ctrl Pts',(86.45949751305,64.748520688217,11.3605817775334));
#74031=CARTESIAN_POINT('Ctrl Pts',(86.4846804398158,64.7440301338687,11.3051942467589));
#74032=CARTESIAN_POINT('Ctrl Pts',(86.5128363483428,64.7395395795204,11.2511502394488));
#74033=CARTESIAN_POINT('Ctrl Pts',(86.5437854254147,64.7350490251721,11.1987882451646));
#74034=CARTESIAN_POINT('Ctrl Pts',(86.5747636162918,64.7305542465581,11.1463769939383));
#74035=CARTESIAN_POINT('Ctrl Pts',(86.6085399490278,64.7260594679441,11.0956513711113));
#74036=CARTESIAN_POINT('Ctrl Pts',(86.6448901103306,64.7215646893301,11.0469226697902));
#74037=CARTESIAN_POINT('Ctrl Pts',(86.6812590641617,64.717067586978,10.9981687764078));
#74038=CARTESIAN_POINT('Ctrl Pts',(86.7202041512511,64.7125704846259,10.9514142637556));
#74039=CARTESIAN_POINT('Ctrl Pts',(86.7614615221642,64.7080733822739,10.9069364003612));
#74040=CARTESIAN_POINT('Ctrl Pts',(86.8027923199855,64.7035682763017,10.8623793784571));
#74041=CARTESIAN_POINT('Ctrl Pts',(86.8464432283836,64.6990631703296,10.8201074552435));
#74042=CARTESIAN_POINT('Ctrl Pts',(86.8921154391265,64.6945580643574,10.7803592356187));
#74043=CARTESIAN_POINT('Ctrl Pts',(86.9157250454818,64.6922292132495,10.7598119530721));
#74044=CARTESIAN_POINT('Ctrl Pts',(86.9398742803986,64.6899003621415,10.7399383743142));
#74045=CARTESIAN_POINT('Ctrl Pts',(86.964518941691,64.6875715110336,10.7207668491297));
#74046=CARTESIAN_POINT('Ctrl Pts',(87.0132040064965,64.6829709094766,10.6828938617531));
#74047=CARTESIAN_POINT('Ctrl Pts',(87.0640472917073,64.6783703079196,10.6475897303211));
#74048=CARTESIAN_POINT('Ctrl Pts',(87.1167469574559,64.6737697063626,10.6151084356505));
#74049=CARTESIAN_POINT('Ctrl Pts',(87.1703047911227,64.6690941880371,10.5820982115335));
#74050=CARTESIAN_POINT('Ctrl Pts',(87.2257796473751,64.6644186697116,10.5520039826383));
#74051=CARTESIAN_POINT('Ctrl Pts',(87.2828196869196,64.6597431513861,10.5250495571751));
#74052=CARTESIAN_POINT('Ctrl Pts',(87.3387900792101,64.6551553110387,10.4986005964243));
#74053=CARTESIAN_POINT('Ctrl Pts',(87.3962669781763,64.6505674706913,10.4751749229019));
#74054=CARTESIAN_POINT('Ctrl Pts',(87.454891069006,64.6459796303438,10.4549389544562));
#74055=CARTESIAN_POINT('Ctrl Pts',(87.5134786793428,64.6413946449094,10.4347155784122));
#74056=CARTESIAN_POINT('Ctrl Pts',(87.5732115866053,64.6368096594749,10.4176781369421));
#74057=CARTESIAN_POINT('Ctrl Pts',(87.6337112909016,64.6322246740405,10.4039446261972));
#74058=CARTESIAN_POINT('Ctrl Pts',(87.6941954774681,64.6276408646211,10.3902146379969));
#74059=CARTESIAN_POINT('Ctrl Pts',(87.7554455752919,64.6230570552018,10.3797870106611));
#74060=CARTESIAN_POINT('Ctrl Pts',(87.8170707322931,64.6184732457824,10.3727291195067));
#74061=CARTESIAN_POINT('Ctrl Pts',(87.8808360388893,64.613730247513,10.3654261183414));
#74062=CARTESIAN_POINT('Ctrl Pts',(87.9450023692494,64.6089872492437,10.3617313487824));
#74063=CARTESIAN_POINT('Ctrl Pts',(88.0091310074875,64.6042442509744,10.3616610247762));
#74064=CARTESIAN_POINT('Ctrl Pts',(88.0711832546621,64.5996548240187,10.3615929777579));
#74065=CARTESIAN_POINT('Ctrl Pts',(88.1331996911742,64.5950653970631,10.3649181350441));
#74066=CARTESIAN_POINT('Ctrl Pts',(88.1947855492387,64.5904759701075,10.3715981269218));
#74067=CARTESIAN_POINT('Ctrl Pts',(88.259462584444,64.5856561861813,10.378613407433));
#74068=CARTESIAN_POINT('Ctrl Pts',(88.3236640465969,64.5808364022551,10.3893290966777));
#74069=CARTESIAN_POINT('Ctrl Pts',(88.3869450187697,64.5760166183289,10.4036401778008));
#74070=CARTESIAN_POINT('Ctrl Pts',(88.4502259909424,64.5711968344027,10.4179512589238));
#74071=CARTESIAN_POINT('Ctrl Pts',(88.5125858776316,64.5663770504765,10.435857483342));
#74072=CARTESIAN_POINT('Ctrl Pts',(88.5736014800555,64.5615572665503,10.4571947258169));
#74073=CARTESIAN_POINT('Ctrl Pts',(88.6318937333619,64.5569526071788,10.4775796092532));
#74074=CARTESIAN_POINT('Ctrl Pts',(88.6891919339384,64.5523479478074,10.5011770587036));
#74075=CARTESIAN_POINT('Ctrl Pts',(88.7451186757438,64.5477432884359,10.5278697696475));
#74076=CARTESIAN_POINT('Ctrl Pts',(88.8018998874603,64.5430682773372,10.5549703019236));
#74077=CARTESIAN_POINT('Ctrl Pts',(88.8572668522401,64.5383932662385,10.5852613856813));
#74078=CARTESIAN_POINT('Ctrl Pts',(88.9108417461413,64.5337182551398,10.6185679057374));
#74079=CARTESIAN_POINT('Ctrl Pts',(88.9634697272463,64.5291258728157,10.6512857476321));
#74080=CARTESIAN_POINT('Ctrl Pts',(89.014368024192,64.5245334904916,10.6869130163857));
#74081=CARTESIAN_POINT('Ctrl Pts',(89.0632019382488,64.5199411081675,10.7252368155616));
#74082=CARTESIAN_POINT('Ctrl Pts',(89.1120072809413,64.5153514127185,10.7635381925489));
#74083=CARTESIAN_POINT('Ctrl Pts',(89.1587502378458,64.5107617172695,10.8045326587561));
#74084=CARTESIAN_POINT('Ctrl Pts',(89.203126525106,64.5061720218205,10.8479650318079));
#74085=CARTESIAN_POINT('Ctrl Pts',(89.2474929939635,64.501583341857,10.8913877953012));
#74086=CARTESIAN_POINT('Ctrl Pts',(89.2894934706362,64.4969946618936,10.9372470400611));
#74087=CARTESIAN_POINT('Ctrl Pts',(89.328859613144,64.4924059819301,10.9852498551265));
#74088=CARTESIAN_POINT('Ctrl Pts',(89.3695117432992,64.4876674019416,11.0348207950649));
#74089=CARTESIAN_POINT('Ctrl Pts',(89.4073540249063,64.482928821953,11.0866773847202));
#74090=CARTESIAN_POINT('Ctrl Pts',(89.4421367360521,64.4781902419644,11.1404609795789));
#74091=CARTESIAN_POINT('Ctrl Pts',(89.4758628999393,64.4735955993956,11.1926108630955));
#74092=CARTESIAN_POINT('Ctrl Pts',(89.5067125275981,64.4690009568268,11.2465718563188));
#74093=CARTESIAN_POINT('Ctrl Pts',(89.5345040421865,64.4644063142581,11.3019906616792));
#74094=CARTESIAN_POINT('Ctrl Pts',(89.5636015034866,64.4595957655596,11.3600136434472));
#74095=CARTESIAN_POINT('Ctrl Pts',(89.5893460680003,64.4547852168611,11.4196342673676));
#74096=CARTESIAN_POINT('Ctrl Pts',(89.6115863532925,64.4499746681626,11.4804249311541));
#74097=CARTESIAN_POINT('Ctrl Pts',(89.6338266385846,64.4451641194641,11.5412155949405));
#74098=CARTESIAN_POINT('Ctrl Pts',(89.6525625340892,64.4403535707656,11.6031756741928));
#74099=CARTESIAN_POINT('Ctrl Pts',(89.6677033646476,64.4355430220671,11.6658640266545));
#74100=CARTESIAN_POINT('Ctrl Pts',(89.6821577798346,64.4309505614424,11.7257103785685));
#74101=CARTESIAN_POINT('Ctrl Pts',(89.6933954589065,64.4263581008177,11.7864662781755));
#74102=CARTESIAN_POINT('Ctrl Pts',(89.7013086450358,64.4217656401929,11.8477535335518));
#74103=CARTESIAN_POINT('Ctrl Pts',(89.7093666998291,64.4170891042509,11.9101627899345));
#74104=CARTESIAN_POINT('Ctrl Pts',(89.7139770955883,64.4124125683089,11.9731225581595));
#74105=CARTESIAN_POINT('Ctrl Pts',(89.7150797883853,64.4077360323668,12.036218958769));
#74106=CARTESIAN_POINT('Ctrl Pts',(89.7161596377748,64.4031563756426,12.0980082530039));
#74107=CARTESIAN_POINT('Ctrl Pts',(89.7138757163543,64.3985767189185,12.1599280362992));
#74108=CARTESIAN_POINT('Ctrl Pts',(89.7082237910141,64.3939970621943,12.2215835428821));
#74109=CARTESIAN_POINT('Ctrl Pts',(89.7025753799761,64.389420253048,12.2832007127805));
#74110=CARTESIAN_POINT('Ctrl Pts',(89.6935631635928,64.3848434439016,12.3445534247203));
#74111=CARTESIAN_POINT('Ctrl Pts',(89.681234938173,64.3802666347553,12.4052492990506));
#74112=CARTESIAN_POINT('Ctrl Pts',(89.6689098239339,64.3756909806236,12.4659298560236));
#74113=CARTESIAN_POINT('Ctrl Pts',(89.653270463239,64.3711153264919,12.5259534045835));
#74114=CARTESIAN_POINT('Ctrl Pts',(89.6344158767858,64.3665396723601,12.5849371123748));
#74115=CARTESIAN_POINT('Ctrl Pts',(89.6148391340697,64.3617887644621,12.6461799762655));
#74116=CARTESIAN_POINT('Ctrl Pts',(89.5917959979519,64.3570378565641,12.7063011518721));
#74117=CARTESIAN_POINT('Ctrl Pts',(89.5654535786364,64.3522869486661,12.7648911985886));
#74118=CARTESIAN_POINT('Ctrl Pts',(89.5400509202948,64.3477055285353,12.8213910561425));
#74119=CARTESIAN_POINT('Ctrl Pts',(89.5115807307275,64.3431241084046,12.876466755529));
#74120=CARTESIAN_POINT('Ctrl Pts',(89.480240170224,64.3385426882738,12.9297755251222));
#74121=CARTESIAN_POINT('Ctrl Pts',(89.4488774219902,64.3339580247002,12.983122034966));
#74122=CARTESIAN_POINT('Ctrl Pts',(89.4146405440095,64.3293733611267,13.0346987031291));
#74123=CARTESIAN_POINT('Ctrl Pts',(89.3777694578984,64.3247886975532,13.0841925577003));
#74124=CARTESIAN_POINT('Ctrl Pts',(89.3408368947595,64.320196389738,13.1337689358798));
#74125=CARTESIAN_POINT('Ctrl Pts',(89.3012616941458,64.3156040819229,13.1812551876722));
#74126=CARTESIAN_POINT('Ctrl Pts',(89.259322423621,64.3110117741078,13.226373199572));
#74127=CARTESIAN_POINT('Ctrl Pts',(89.2548079329476,64.3105174419332,13.2312298611538));
#74128=CARTESIAN_POINT('Ctrl Pts',(89.2502660819866,64.3100231097585,13.2360591193132));
#74129=CARTESIAN_POINT('Ctrl Pts',(89.2456972411236,64.3095287775839,13.2408606548701));
#74130=CARTESIAN_POINT('Ctrl Pts',(89.203200857864,64.3049308215201,13.2855214126807));
#74131=CARTESIAN_POINT('Ctrl Pts',(89.1581911054405,64.3003328654562,13.3279649817505));
#74132=CARTESIAN_POINT('Ctrl Pts',(89.1109284721037,64.2957349093924,13.3678956148077));
#74133=CARTESIAN_POINT('Ctrl Pts',(89.0628651730352,64.2910590603802,13.408502703815));
#74134=CARTESIAN_POINT('Ctrl Pts',(89.0124722475177,64.2863832113681,13.4465104722219));
#74135=CARTESIAN_POINT('Ctrl Pts',(88.9600647117717,64.2817073623559,13.4816450856305));
#74136=CARTESIAN_POINT('Ctrl Pts',(88.9086719748842,64.2771220546404,13.5160993662382));
#74137=CARTESIAN_POINT('Ctrl Pts',(88.8553423955163,64.2725367469249,13.5477904729261));
#74138=CARTESIAN_POINT('Ctrl Pts',(88.8004063281201,64.2679514392094,13.5765007397297));
#74139=CARTESIAN_POINT('Ctrl Pts',(88.7455038702107,64.2633689367518,13.6051934418006));
#74140=CARTESIAN_POINT('Ctrl Pts',(88.6889973231742,64.2587864342942,13.6309086848791));
#74141=CARTESIAN_POINT('Ctrl Pts',(88.6312431891249,64.2542039318366,13.6534738492158));
#74142=CARTESIAN_POINT('Ctrl Pts',(88.5735031945594,64.2496225512765,13.6760334891035));
#74143=CARTESIAN_POINT('Ctrl Pts',(88.5145166930798,64.2450411707164,13.6954443961278));
#74144=CARTESIAN_POINT('Ctrl Pts',(88.4546598940543,64.2404597901563,13.7115821869502));
#74145=CARTESIAN_POINT('Ctrl Pts',(88.3926596453967,64.2357143520684,13.7282978660386));
#74146=CARTESIAN_POINT('Ctrl Pts',(88.3297261296616,64.2309689139804,13.7415013476342));
#74147=CARTESIAN_POINT('Ctrl Pts',(88.2662917545099,64.2262234758924,13.751111555856));
#74148=CARTESIAN_POINT('Ctrl Pts',(88.2049731094462,64.2216363126534,13.7604012342918));
#74149=CARTESIAN_POINT('Ctrl Pts',(88.1431870238345,64.2170491494143,13.7663335972473));
#74150=CARTESIAN_POINT('Ctrl Pts',(88.081329211241,64.2124619861752,13.7688883221299));
#74151=CARTESIAN_POINT('Ctrl Pts',(88.0162698984721,64.2076374106628,13.7715752688259));
#74152=CARTESIAN_POINT('Ctrl Pts',(87.9511318747261,64.2028128351504,13.7705254476601));
#74153=CARTESIAN_POINT('Ctrl Pts',(87.8863722166979,64.1979882596379,13.7657772651819));
#74154=CARTESIAN_POINT('Ctrl Pts',(87.8216125586697,64.1931636841255,13.7610290827036));
#74155=CARTESIAN_POINT('Ctrl Pts',(87.7572318972208,64.188339108613,13.7525826992389));
#74156=CARTESIAN_POINT('Ctrl Pts',(87.6936744123666,64.1835145331006,13.7405385355474));
#74157=CARTESIAN_POINT('Ctrl Pts',(87.6331015097317,64.1789165137888,13.7290599511402));
#74158=CARTESIAN_POINT('Ctrl Pts',(87.5730283945625,64.174318494477,13.7142670174428));
#74159=CARTESIAN_POINT('Ctrl Pts',(87.5138448271403,64.1697204751652,13.6962182583013));
#74160=CARTESIAN_POINT('Ctrl Pts',(87.4536595737528,64.165044634059,13.677864022665));
#74161=CARTESIAN_POINT('Ctrl Pts',(87.3943947979762,64.1603687929529,13.6561427314989));
#74162=CARTESIAN_POINT('Ctrl Pts',(87.3364513882402,64.1556929518467,13.6311705996385));
#74163=CARTESIAN_POINT('Ctrl Pts',(87.2796285339039,64.1511075358471,13.6066813985779));
#74164=CARTESIAN_POINT('Ctrl Pts',(87.2240768824105,64.1465221198475,13.5790661837745));
#74165=CARTESIAN_POINT('Ctrl Pts',(87.1701584656107,64.1419367038479,13.5484845191927));
#74166=CARTESIAN_POINT('Ctrl Pts',(87.1162728404869,64.1373540765703,13.5179214535255));
#74167=CARTESIAN_POINT('Ctrl Pts',(87.0640189221741,64.1327714492927,13.4843957659505));
#74168=CARTESIAN_POINT('Ctrl Pts',(87.0137350678613,64.1281888220151,13.4481134145672));
#74169=CARTESIAN_POINT('Ctrl Pts',(86.9634633440896,64.1236073002564,13.4118398159845));
#74170=CARTESIAN_POINT('Ctrl Pts',(86.9151611532857,64.1190257784977,13.3728111714002));
#74171=CARTESIAN_POINT('Ctrl Pts',(86.8691370058838,64.1144442567389,13.3312761509915));
#74172=CARTESIAN_POINT('Ctrl Pts',(86.8214672991706,64.1096989260621,13.2882560766833));
#74173=CARTESIAN_POINT('Ctrl Pts',(86.7762420968786,64.1049535953853,13.2425473434725));
#74174=CARTESIAN_POINT('Ctrl Pts',(86.7337639413596,64.1002082647085,13.1944692667985));
#74175=CARTESIAN_POINT('Ctrl Pts',(86.6927000151676,64.0956209207835,13.1479918581664));
#74176=CARTESIAN_POINT('Ctrl Pts',(86.6542033522433,64.0910335768584,13.0993008622936));
#74177=CARTESIAN_POINT('Ctrl Pts',(86.618505603288,64.0864462329333,13.0487177574084));
#74178=CARTESIAN_POINT('Ctrl Pts',(86.5809637246491,64.0816219088806,12.9955215520355));
#74179=CARTESIAN_POINT('Ctrl Pts',(86.5465181371553,64.076797584828,12.9402329811251));
#74180=CARTESIAN_POINT('Ctrl Pts',(86.5153843596422,64.0719732607754,12.8832568090369));
#74181=CARTESIAN_POINT('Ctrl Pts',(86.4842505821292,64.0671489367227,12.8262806369487));
#74182=CARTESIAN_POINT('Ctrl Pts',(86.456428821725,64.0623246126701,12.7676174804095));
#74183=CARTESIAN_POINT('Ctrl Pts',(86.4320755186073,64.0575002886174,12.7076948789408));
#74184=CARTESIAN_POINT('Ctrl Pts',(86.4060606507051,64.0523468130358,12.6436839086822));
#74185=CARTESIAN_POINT('Ctrl Pts',(86.3839120926027,64.0471933374543,12.5780148787507));
#74186=CARTESIAN_POINT('Ctrl Pts',(86.3658179547188,64.0420398618727,12.5111414084137));
#74187=CARTESIAN_POINT('Ctrl Pts',(86.34779236838,64.0369059107756,12.4445212952546));
#74188=CARTESIAN_POINT('Ctrl Pts',(86.3337906946726,64.0317719596785,12.3767061001825));
#74189=CARTESIAN_POINT('Ctrl Pts',(86.3239521898502,64.0266380085813,12.3081663103502));
#74190=CARTESIAN_POINT('Ctrl Pts',(86.3141736527811,64.0215353499945,12.2400442849331));
#74191=CARTESIAN_POINT('Ctrl Pts',(86.3085078171002,64.0164326914076,12.1712067393078));
#74192=CARTESIAN_POINT('Ctrl Pts',(86.30704307437,64.0113300328208,12.1021335190311));
#74193=CARTESIAN_POINT('Ctrl Pts',(86.3067947769097,64.0104650500891,12.0904244968143));
#74194=CARTESIAN_POINT('Ctrl Pts',(86.3066670851384,64.0096000673575,12.0787087386656));
#74195=CARTESIAN_POINT('Ctrl Pts',(86.3066602867323,64.0087350846259,12.0669886246394));
#74196=CARTESIAN_POINT('',(86.306660578502,63.2149850845225,12.064595746523));
#74197=CARTESIAN_POINT('Ctrl Pts',(86.3066602867319,64.0087350845702,12.0669886238853));
#74198=CARTESIAN_POINT('Ctrl Pts',(86.3066239196403,64.0041079808479,12.0042935188232));
#74199=CARTESIAN_POINT('Ctrl Pts',(86.3100513046104,63.9994808771256,11.9415921390125));
#74200=CARTESIAN_POINT('Ctrl Pts',(86.3169180933848,63.9948537734033,11.8792881115757));
#74201=CARTESIAN_POINT('Ctrl Pts',(86.3237866480857,63.9902254797324,11.8169680614621));
#74202=CARTESIAN_POINT('Ctrl Pts',(86.3340963066402,63.9855971860615,11.7550460578555));
#74203=CARTESIAN_POINT('Ctrl Pts',(86.347771042048,63.9809688923906,11.6939190020573));
#74204=CARTESIAN_POINT('Ctrl Pts',(86.3614647011323,63.9763341938915,11.6327073560576));
#74205=CARTESIAN_POINT('Ctrl Pts',(86.3785326224402,63.9716994953924,11.5722933369329));
#74206=CARTESIAN_POINT('Ctrl Pts',(86.3988481836135,63.9670647968932,11.513061163851));
#74207=CARTESIAN_POINT('Ctrl Pts',(86.4191791147488,63.9624265919618,11.453784178015));
#74208=CARTESIAN_POINT('Ctrl Pts',(86.4427623903478,63.9577883870304,11.3956912762091));
#74209=CARTESIAN_POINT('Ctrl Pts',(86.4694233889334,63.9531501820989,11.3391462404222));
#74210=CARTESIAN_POINT('Ctrl Pts',(86.4961384510343,63.948502571756,11.2824865418854));
#74211=CARTESIAN_POINT('Ctrl Pts',(86.5259434617493,63.943854961413,11.2273814113902));
#74212=CARTESIAN_POINT('Ctrl Pts',(86.5586184485326,63.93920735107,11.174168925997));
#74213=CARTESIAN_POINT('Ctrl Pts',(86.576713310441,63.9366335820914,11.1447007403976));
#74214=CARTESIAN_POINT('Ctrl Pts',(86.5956875624115,63.9340598131128,11.1158124513202));
#74215=CARTESIAN_POINT('Ctrl Pts',(86.615498525731,63.9314860441341,11.0875571192384));
#74216=CARTESIAN_POINT('Ctrl Pts',(86.6508855750261,63.9268886861838,11.0370864372678));
#74217=CARTESIAN_POINT('Ctrl Pts',(86.6890868020166,63.9222913282335,10.9884344196781));
#74218=CARTESIAN_POINT('Ctrl Pts',(86.7298886226617,63.9176939702831,10.9419321753318));
#74219=CARTESIAN_POINT('Ctrl Pts',(86.7713877196069,63.9130180465068,10.8946352381906));
#74220=CARTESIAN_POINT('Ctrl Pts',(86.8155769034407,63.9083421227304,10.8495627296339));
#74221=CARTESIAN_POINT('Ctrl Pts',(86.8621852912376,63.9036661989541,10.807032327448));
#74222=CARTESIAN_POINT('Ctrl Pts',(86.907884525315,63.899081484801,10.7653315328748));
#74223=CARTESIAN_POINT('Ctrl Pts',(86.9559090376499,63.894496770648,10.7260749207465));
#74224=CARTESIAN_POINT('Ctrl Pts',(87.0059645427723,63.8899120564949,10.6895267654926));
#74225=CARTESIAN_POINT('Ctrl Pts',(87.05598945735,63.8853301442096,10.6530009460034));
#74226=CARTESIAN_POINT('Ctrl Pts',(87.1080424933373,63.8807482319242,10.6191806008449));
#74227=CARTESIAN_POINT('Ctrl Pts',(87.1617968156538,63.8761663196389,10.5882893424975));
#74228=CARTESIAN_POINT('Ctrl Pts',(87.2155380274884,63.8715855248651,10.5574056184147));
#74229=CARTESIAN_POINT('Ctrl Pts',(87.270979260806,63.8670047300914,10.5294498164671));
#74230=CARTESIAN_POINT('Ctrl Pts',(87.3277670277041,63.8624239353176,10.5046007745718));
#74231=CARTESIAN_POINT('Ctrl Pts',(87.3866029714709,63.8576779240121,10.4788554968216));
#74232=CARTESIAN_POINT('Ctrl Pts',(87.4468839301898,63.8529319127065,10.4564456591323));
#74233=CARTESIAN_POINT('Ctrl Pts',(87.5081941086608,63.848185901401,10.4375157135439));
#74234=CARTESIAN_POINT('Ctrl Pts',(87.5674449113936,63.8435993060485,10.4192216145904));
#74235=CARTESIAN_POINT('Ctrl Pts',(87.6276563540583,63.839012710696,10.4041773813569));
#74236=CARTESIAN_POINT('Ctrl Pts',(87.6884402080479,63.8344261153436,10.3924618270814));
#74237=CARTESIAN_POINT('Ctrl Pts',(87.7523930518672,63.8296003960615,10.3801354778347));
#74238=CARTESIAN_POINT('Ctrl Pts',(87.8169789902477,63.8247746767794,10.371494489716));
#74239=CARTESIAN_POINT('Ctrl Pts',(87.8817399184812,63.8199489574973,10.3665687225057));
#74240=CARTESIAN_POINT('Ctrl Pts',(87.9465008467147,63.8151232382152,10.3616429552955));
#74241=CARTESIAN_POINT('Ctrl Pts',(88.0114361157952,63.8102975189331,10.3604323437773));
#74242=CARTESIAN_POINT('Ctrl Pts',(88.0760911879079,63.8054717996509,10.3629034164626));
#74243=CARTESIAN_POINT('Ctrl Pts',(88.1376859515102,63.8008744953919,10.3652575262474));
#74244=CARTESIAN_POINT('Ctrl Pts',(88.1992792246782,63.7962771911329,10.3709622604175));
#74245=CARTESIAN_POINT('Ctrl Pts',(88.2604769952076,63.7916798868738,10.3800177745711));
#74246=CARTESIAN_POINT('Ctrl Pts',(88.3227214116909,63.7870039563861,10.3892281622955));
#74247=CARTESIAN_POINT('Ctrl Pts',(88.3845561365458,63.7823280258983,10.4019050968116));
#74248=CARTESIAN_POINT('Ctrl Pts',(88.445567347191,63.7776520954106,10.4179933081582));
#74249=CARTESIAN_POINT('Ctrl Pts',(88.5053877157701,63.7730674316698,10.4337675031357));
#74250=CARTESIAN_POINT('Ctrl Pts',(88.5644159129872,63.768482767929,10.4528208698359));
#74251=CARTESIAN_POINT('Ctrl Pts',(88.6222703039524,63.7638981041882,10.4750495133079));
#74252=CARTESIAN_POINT('Ctrl Pts',(88.6800893551115,63.7593162409457,10.4972645786238));
#74253=CARTESIAN_POINT('Ctrl Pts',(88.7367355475692,63.7547343777033,10.5226508925969));
#74254=CARTESIAN_POINT('Ctrl Pts',(88.7918437532103,63.7501525144609,10.5510551598581));
#74255=CARTESIAN_POINT('Ctrl Pts',(88.8469385355215,63.7455717672748,10.5794525083703));
#74256=CARTESIAN_POINT('Ctrl Pts',(88.900495622447,63.7409910200887,10.6108661177419));
#74257=CARTESIAN_POINT('Ctrl Pts',(88.952173046271,63.7364102729026,10.6450960157094));
#74258=CARTESIAN_POINT('Ctrl Pts',(89.0057154345313,63.7316642130914,10.6805612218181));
#74259=CARTESIAN_POINT('Ctrl Pts',(89.0572393760856,63.7269181532801,10.719049608478));
#74260=CARTESIAN_POINT('Ctrl Pts',(89.1063979774428,63.7221720934689,10.7602901905039));
#74261=CARTESIAN_POINT('Ctrl Pts',(89.1539044331854,63.7175855414892,10.8001447394684));
#74262=CARTESIAN_POINT('Ctrl Pts',(89.1992016919601,63.7129989895095,10.8425689986601));
#74263=CARTESIAN_POINT('Ctrl Pts',(89.2420129780526,63.7084124375298,10.8872795566946));
#74264=CARTESIAN_POINT('Ctrl Pts',(89.2870575546779,63.7035866238028,10.9343224825483));
#74265=CARTESIAN_POINT('Ctrl Pts',(89.329349261722,63.6987608100758,10.983896292323));
#74266=CARTESIAN_POINT('Ctrl Pts',(89.3686145299541,63.6939349963488,11.0356322871627));
#74267=CARTESIAN_POINT('Ctrl Pts',(89.4078797981862,63.6891091826218,11.0873682820025));
#74268=CARTESIAN_POINT('Ctrl Pts',(89.4441183303605,63.6842833688948,11.1412658811746));
#74269=CARTESIAN_POINT('Ctrl Pts',(89.4771117056078,63.6794575551678,11.1969250306909));
#74270=CARTESIAN_POINT('Ctrl Pts',(89.5085417152874,63.6748604088917,11.2499468144563));
#74271=CARTESIAN_POINT('Ctrl Pts',(89.5371562642813,63.6702632626157,11.3047846688));
#74272=CARTESIAN_POINT('Ctrl Pts',(89.5627414986066,63.6656661163397,11.3611076982246));
#74273=CARTESIAN_POINT('Ctrl Pts',(89.5887653132273,63.660990166104,11.4183962130762));
#74274=CARTESIAN_POINT('Ctrl Pts',(89.6116546258482,63.6563142158684,11.4772208925681));
#74275=CARTESIAN_POINT('Ctrl Pts',(89.6312313783171,63.6516382656328,11.5372040882185));
#74276=CARTESIAN_POINT('Ctrl Pts',(89.6504252492963,63.6470537674801,11.5960141344746));
#74277=CARTESIAN_POINT('Ctrl Pts',(89.6664348019616,63.6424692693275,11.6559372812805));
#74278=CARTESIAN_POINT('Ctrl Pts',(89.6791403089382,63.6378847711749,11.7165965866001));
#74279=CARTESIAN_POINT('Ctrl Pts',(89.6918380480151,63.6333030758952,11.777218806001));
#74280=CARTESIAN_POINT('Ctrl Pts',(89.7012356426772,63.6287213806155,11.8385757942671));
#74281=CARTESIAN_POINT('Ctrl Pts',(89.7072638202796,63.6241396853358,11.9002776792029));
#74282=CARTESIAN_POINT('Ctrl Pts',(89.7132905267104,63.6195591082149,11.9619645058468));
#74283=CARTESIAN_POINT('Ctrl Pts',(89.7159493989979,63.614978531094,12.0239955556393));
#74284=CARTESIAN_POINT('Ctrl Pts',(89.7152229405887,63.6103979539731,12.085975093775));
#74285=CARTESIAN_POINT('Ctrl Pts',(89.7144702119392,63.6056517336991,12.1501959403432));
#74286=CARTESIAN_POINT('Ctrl Pts',(89.7100825619892,63.600905513425,12.2143608961065));
#74287=CARTESIAN_POINT('Ctrl Pts',(89.7020994909172,63.596159293151,12.2780314774261));
#74288=CARTESIAN_POINT('Ctrl Pts',(89.6943852710916,63.5915729145249,12.339557781814));
#74289=CARTESIAN_POINT('Ctrl Pts',(89.6833141320636,63.5869865358989,12.4006219767003));
#74290=CARTESIAN_POINT('Ctrl Pts',(89.6689740403695,63.5824001572728,12.4608378364098));
#74291=CARTESIAN_POINT('Ctrl Pts',(89.6538842905872,63.5775740161748,12.5242016052985));
#74292=CARTESIAN_POINT('Ctrl Pts',(89.6351745986117,63.5727478750768,12.5866252872646));
#74293=CARTESIAN_POINT('Ctrl Pts',(89.6130063747922,63.5679217339787,12.6476789584687));
#74294=CARTESIAN_POINT('Ctrl Pts',(89.5908381509727,63.5630955928807,12.7087326296728));
#74295=CARTESIAN_POINT('Ctrl Pts',(89.5652117221723,63.5582694517826,12.7684157250627));
#74296=CARTESIAN_POINT('Ctrl Pts',(89.5363447766494,63.5534433106846,12.8263276582818));
#74297=CARTESIAN_POINT('Ctrl Pts',(89.5088469416784,63.5488460653212,12.8814929261572));
#74298=CARTESIAN_POINT('Ctrl Pts',(89.4782961644025,63.5442488199578,12.9352777815762));
#74299=CARTESIAN_POINT('Ctrl Pts',(89.4448544642557,63.5396515745944,12.9873230763061));
#74300=CARTESIAN_POINT('Ctrl Pts',(89.4108403320712,63.5349756367447,13.0402592466189));
#74301=CARTESIAN_POINT('Ctrl Pts',(89.3738355276833,63.530299698895,13.0913952257273));
#74302=CARTESIAN_POINT('Ctrl Pts',(89.3340607475308,63.5256237610453,13.1403766071277));
#74303=CARTESIAN_POINT('Ctrl Pts',(89.2950629069714,63.5210391605012,13.1884012120384));
#74304=CARTESIAN_POINT('Ctrl Pts',(89.2534026684274,63.5164545599571,13.2343542219115));
#74305=CARTESIAN_POINT('Ctrl Pts',(89.2093317869495,63.511869959413,13.2779305937166));
#74306=CARTESIAN_POINT('Ctrl Pts',(89.1652878398618,63.5072881607965,13.3214803333565));
#74307=CARTESIAN_POINT('Ctrl Pts',(89.1188365323839,63.50270636218,13.3626559578748));
#74308=CARTESIAN_POINT('Ctrl Pts',(89.0702678479934,63.4981245635635,13.4011878002017));
#74309=CARTESIAN_POINT('Ctrl Pts',(89.0217110082514,63.4935438823294,13.4397102456068));
#74310=CARTESIAN_POINT('Ctrl Pts',(88.971038215284,63.4889632010953,13.4755898725143));
#74311=CARTESIAN_POINT('Ctrl Pts',(88.9185724602104,63.4843825198612,13.5085973329615));
#74312=CARTESIAN_POINT('Ctrl Pts',(88.8642118058735,63.4796363987229,13.5427969198233));
#74313=CARTESIAN_POINT('Ctrl Pts',(88.8079266560086,63.4748902775846,13.5739125378752));
#74314=CARTESIAN_POINT('Ctrl Pts',(88.7501067800997,63.4701441564462,13.6017395622991));
#74315=CARTESIAN_POINT('Ctrl Pts',(88.6942316986764,63.465557672977,13.6286306137068));
#74316=CARTESIAN_POINT('Ctrl Pts',(88.6369240162277,63.4609711895078,13.6524506638998));
#74317=CARTESIAN_POINT('Ctrl Pts',(88.5785559360207,63.4563847060386,13.6730641228923));
#74318=CARTESIAN_POINT('Ctrl Pts',(88.5171405066834,63.4515587660657,13.6947537935079));
#74319=CARTESIAN_POINT('Ctrl Pts',(88.4545515346259,63.4467328260928,13.7128926772634));
#74320=CARTESIAN_POINT('Ctrl Pts',(88.3912376859154,63.4419068861199,13.7273832001708));
#74321=CARTESIAN_POINT('Ctrl Pts',(88.3279238372049,63.4370809461471,13.7418737230782));
#74322=CARTESIAN_POINT('Ctrl Pts',(88.2638857636009,63.4322550061742,13.7527158532581));
#74323=CARTESIAN_POINT('Ctrl Pts',(88.1995780088928,63.4274290662013,13.759875193207));
#74324=CARTESIAN_POINT('Ctrl Pts',(88.1383178995474,63.4228318350933,13.7666952408063));
#74325=CARTESIAN_POINT('Ctrl Pts',(88.0765615899772,63.4182346039852,13.7702017341098));
#74326=CARTESIAN_POINT('Ctrl Pts',(88.0146986851029,63.4136373728772,13.7703359866319));
#74327=CARTESIAN_POINT('Ctrl Pts',(87.9517766344529,63.4089614332456,13.7704725376718));
#74328=CARTESIAN_POINT('Ctrl Pts',(87.88874482066,63.4042854936139,13.7671201368571));
#74329=CARTESIAN_POINT('Ctrl Pts',(87.8260206957689,63.3996095539823,13.7602719653604));
#74330=CARTESIAN_POINT('Ctrl Pts',(87.7645220040835,63.3950249675852,13.7535575857144));
#74331=CARTESIAN_POINT('Ctrl Pts',(87.7033196171185,63.3904403811881,13.7434828577989));
#74332=CARTESIAN_POINT('Ctrl Pts',(87.6428063576431,63.385855794791,13.7300938306862));
#74333=CARTESIAN_POINT('Ctrl Pts',(87.5823300805425,63.3812740102409,13.7167129862103));
#74334=CARTESIAN_POINT('Ctrl Pts',(87.522542591832,63.3766922256908,13.7000219685882));
#74335=CARTESIAN_POINT('Ctrl Pts',(87.463827729285,63.3721104411407,13.6801181312905));
#74336=CARTESIAN_POINT('Ctrl Pts',(87.4051271844849,63.3675297738687,13.6602191475867));
#74337=CARTESIAN_POINT('Ctrl Pts',(87.3474992284899,63.3629491065967,13.6371090628348));
#74338=CARTESIAN_POINT('Ctrl Pts',(87.2913117294407,63.3583684393247,13.6109348299587));
#74339=CARTESIAN_POINT('Ctrl Pts',(87.2330945683247,63.3536223045241,13.5838151047845));
#74340=CARTESIAN_POINT('Ctrl Pts',(87.1764244778286,63.3488761697236,13.55340580834));
#74341=CARTESIAN_POINT('Ctrl Pts',(87.1216847825832,63.344130034923,13.5199234091488));
#74342=CARTESIAN_POINT('Ctrl Pts',(87.0687865871181,63.3395435649901,13.4875673923841));
#74343=CARTESIAN_POINT('Ctrl Pts',(87.0176913535797,63.3349570950571,13.4523421268085));
#74344=CARTESIAN_POINT('Ctrl Pts',(86.9687148743522,63.3303706251242,13.4144867639148));
#74345=CARTESIAN_POINT('Ctrl Pts',(86.9171809305,63.3255446578898,13.3746546613088));
#74346=CARTESIAN_POINT('Ctrl Pts',(86.8679935764349,63.3207186906555,13.3319106662234));
#74347=CARTESIAN_POINT('Ctrl Pts',(86.8214781474381,63.3158927234211,13.2865787962592));
#74348=CARTESIAN_POINT('Ctrl Pts',(86.7749627184413,63.3110667561868,13.2412469262951));
#74349=CARTESIAN_POINT('Ctrl Pts',(86.7311195948234,63.3062407889525,13.1933277117473));
#74350=CARTESIAN_POINT('Ctrl Pts',(86.6902242220587,63.3014148217181,13.1431843760488));
#74351=CARTESIAN_POINT('Ctrl Pts',(86.6514214335936,63.2968357954598,13.0956068356938));
#74352=CARTESIAN_POINT('Ctrl Pts',(86.6151082745464,63.2922567692015,13.0458263197573));
#74353=CARTESIAN_POINT('Ctrl Pts',(86.5815453095547,63.2876777429431,12.9941347550674));
#74354=CARTESIAN_POINT('Ctrl Pts',(86.5480322635142,63.2831055271733,12.9425200724017));
#74355=CARTESIAN_POINT('Ctrl Pts',(86.5172615811686,63.2785333114035,12.8890004005237));
#74356=CARTESIAN_POINT('Ctrl Pts',(86.4894535277513,63.2739610956337,12.8339004938059));
#74357=CARTESIAN_POINT('Ctrl Pts',(86.4616764260128,63.2693939689563,12.7788619158907));
#74358=CARTESIAN_POINT('Ctrl Pts',(86.4368556441183,63.2648268422789,12.7222470465303));
#74359=CARTESIAN_POINT('Ctrl Pts',(86.4151669271033,63.2602597156015,12.6644075860558));
#74360=CARTESIAN_POINT('Ctrl Pts',(86.3934918302003,63.255695456995,12.6066044476898));
#74361=CARTESIAN_POINT('Ctrl Pts',(86.3749450801124,63.2511311983884,12.5475787214813));
#74362=CARTESIAN_POINT('Ctrl Pts',(86.3596546020395,63.2465669397819,12.4877027534112));
#74363=CARTESIAN_POINT('Ctrl Pts',(86.3443695284116,63.2420042944202,12.4278479486022));
#74364=CARTESIAN_POINT('Ctrl Pts',(86.3323385650718,63.2374416490585,12.3671439962651));
#74365=CARTESIAN_POINT('Ctrl Pts',(86.3236393684921,63.2328790036969,12.3059769464703));
#74366=CARTESIAN_POINT('Ctrl Pts',(86.3149375352517,63.2283149754319,12.2447913574053));
#74367=CARTESIAN_POINT('Ctrl Pts',(86.3095695536903,63.2237509471669,12.1831428992014));
#74368=CARTESIAN_POINT('Ctrl Pts',(86.3075614321109,63.2191869189019,12.1214245525729));
#74369=CARTESIAN_POINT('Ctrl Pts',(86.3069451786826,63.217786307458,12.1024843932294));
#74370=CARTESIAN_POINT('Ctrl Pts',(86.3066449717231,63.2163856960141,12.0835376691406));
#74371=CARTESIAN_POINT('Ctrl Pts',(86.3066605785015,63.2149850845702,12.0645957471688));
#74372=CARTESIAN_POINT('',(86.306660007507,62.4212350846317,12.0658400339999));
#74373=CARTESIAN_POINT('Ctrl Pts',(86.306660578502,63.2149850845225,12.064595746523));
#74374=CARTESIAN_POINT('Ctrl Pts',(86.306721132394,63.2095507512284,11.9911016181765));
#74375=CARTESIAN_POINT('Ctrl Pts',(86.3115393780642,63.2041164179344,11.9178111520133));
#74376=CARTESIAN_POINT('Ctrl Pts',(86.3210134498976,63.1986820846404,11.8452732547402));
#74377=CARTESIAN_POINT('Ctrl Pts',(86.3306070180728,63.1931792081729,11.7718204379349));
#74378=CARTESIAN_POINT('Ctrl Pts',(86.3449745067232,63.1876763317055,11.6991393584463));
#74379=CARTESIAN_POINT('Ctrl Pts',(86.36396116775,63.182173455238,11.6277786852962));
#74380=CARTESIAN_POINT('Ctrl Pts',(86.3717506901681,63.179915829237,11.5985020493209));
#74381=CARTESIAN_POINT('Ctrl Pts',(86.380317132937,63.1776582032359,11.5694474071227));
#74382=CARTESIAN_POINT('Ctrl Pts',(86.389647512673,63.1754005772349,11.5406515942363));
#74383=CARTESIAN_POINT('Ctrl Pts',(86.4086470601855,63.1708033503603,11.4820143864718));
#74384=CARTESIAN_POINT('Ctrl Pts',(86.4308706862237,63.1662061234857,11.424288837461));
#74385=CARTESIAN_POINT('Ctrl Pts',(86.4562115126177,63.1616088966111,11.3678541734685));
#74386=CARTESIAN_POINT('Ctrl Pts',(86.481986222258,63.1569329564503,11.3104532404665));
#74387=CARTESIAN_POINT('Ctrl Pts',(86.5109858086307,63.1522570162895,11.2543883470906));
#74388=CARTESIAN_POINT('Ctrl Pts',(86.5430446607671,63.1475810761287,11.2000427506986));
#74389=CARTESIAN_POINT('Ctrl Pts',(86.5744771476656,63.142996494397,11.1467589575261));
#74390=CARTESIAN_POINT('Ctrl Pts',(86.6088501606325,63.1384119126653,11.0951283417784));
#74391=CARTESIAN_POINT('Ctrl Pts',(86.6459600448921,63.1338273309337,11.0454899527397));
#74392=CARTESIAN_POINT('Ctrl Pts',(86.6830472484086,63.1292455511973,10.9958819015901));
#74393=CARTESIAN_POINT('Ctrl Pts',(86.7228677022946,63.1246637714609,10.9482640696739));
#74394=CARTESIAN_POINT('Ctrl Pts',(86.765174693131,63.1200819917245,10.9029462005716));
#74395=CARTESIAN_POINT('Ctrl Pts',(86.807471366005,63.115501329407,10.8576393837342));
#74396=CARTESIAN_POINT('Ctrl Pts',(86.8522530247635,63.1109206670895,10.8146317881271));
#74397=CARTESIAN_POINT('Ctrl Pts',(86.899234326083,63.106340004772,10.77419818784));
#74398=CARTESIAN_POINT('Ctrl Pts',(86.9479128329776,63.101593865437,10.7323039185229));
#74399=CARTESIAN_POINT('Ctrl Pts',(86.9989525509673,63.096847726102,10.6931736046698));
#74400=CARTESIAN_POINT('Ctrl Pts',(87.0519984186674,63.0921015867669,10.6570674953705));
#74401=CARTESIAN_POINT('Ctrl Pts',(87.1032596610378,63.0875151220841,10.6221761060862));
#74402=CARTESIAN_POINT('Ctrl Pts',(87.1563937126347,63.0829286574012,10.5901088635486));
#74403=CARTESIAN_POINT('Ctrl Pts',(87.2110526384385,63.0783421927184,10.5610551324614));
#74404=CARTESIAN_POINT('Ctrl Pts',(87.2685659342977,63.0735162160573,10.5304841725082));
#74405=CARTESIAN_POINT('Ctrl Pts',(87.3277671532957,63.0686902393961,10.5032503734019));
#74406=CARTESIAN_POINT('Ctrl Pts',(87.3882270847903,63.063864262735,10.4795168668778));
#74407=CARTESIAN_POINT('Ctrl Pts',(87.4486870162849,63.0590382860739,10.4557833603537));
#74408=CARTESIAN_POINT('Ctrl Pts',(87.5104050204361,63.0542123094127,10.4355502747426));
#74409=CARTESIAN_POINT('Ctrl Pts',(87.5729366906525,63.0493863327516,10.4189191359853));
#74410=CARTESIAN_POINT('Ctrl Pts',(87.6325043444477,63.0447891085614,10.4030763172617));
#74411=CARTESIAN_POINT('Ctrl Pts',(87.6930548305815,63.0401918843712,10.3904365935124));
#74412=CARTESIAN_POINT('Ctrl Pts',(87.7542115829353,63.0355946601809,10.3811158661613));
#74413=CARTESIAN_POINT('Ctrl Pts',(87.816415496237,63.0309187196846,10.371635543977));
#74414=CARTESIAN_POINT('Ctrl Pts',(87.879246144788,63.0262427791882,10.3655891755679));
#74415=CARTESIAN_POINT('Ctrl Pts',(87.9422917184275,63.0215668386919,10.3630455062911));
#74416=CARTESIAN_POINT('Ctrl Pts',(88.0041054679006,63.016982259669,10.3605515368283));
#74417=CARTESIAN_POINT('Ctrl Pts',(88.0661252863284,63.0123976806461,10.3614246431067));
#74418=CARTESIAN_POINT('Ctrl Pts',(88.1279558695297,63.0078131016232,10.3656776305116));
#74419=CARTESIAN_POINT('Ctrl Pts',(88.1897486631999,63.0032313245971,10.3699280185816));
#74420=CARTESIAN_POINT('Ctrl Pts',(88.2513519441803,62.9986495475709,10.3775541569119));
#74421=CARTESIAN_POINT('Ctrl Pts',(88.3123716736544,62.9940677705448,10.3885167810321));
#74422=CARTESIAN_POINT('Ctrl Pts',(88.3733765214763,62.9894871109344,10.3994767315588));
#74423=CARTESIAN_POINT('Ctrl Pts',(88.4337975995137,62.9849064513241,10.4137714625632));
#74424=CARTESIAN_POINT('Ctrl Pts',(88.4932492947337,62.9803257917138,10.4313102883639));
#74425=CARTESIAN_POINT('Ctrl Pts',(88.5548487605118,62.97557964976,10.4494827272776));
#74426=CARTESIAN_POINT('Ctrl Pts',(88.6154068862498,62.9708335078062,10.4711380400035));
#74427=CARTESIAN_POINT('Ctrl Pts',(88.6745124453264,62.9660873658525,10.4961190903457));
#74428=CARTESIAN_POINT('Ctrl Pts',(88.7316294477733,62.9615009038373,10.5202596743417));
#74429=CARTESIAN_POINT('Ctrl Pts',(88.7873896358226,62.9569144418222,10.5475054553707));
#74430=CARTESIAN_POINT('Ctrl Pts',(88.8414452010442,62.9523279798071,10.5776668371421));
#74431=CARTESIAN_POINT('Ctrl Pts',(88.8983237230385,62.947501997884,10.6094033440018));
#74432=CARTESIAN_POINT('Ctrl Pts',(88.9533141489289,62.9426760159609,10.6443679899557));
#74433=CARTESIAN_POINT('Ctrl Pts',(89.0060466236306,62.9378500340378,10.6822886672426));
#74434=CARTESIAN_POINT('Ctrl Pts',(89.0587790983324,62.9330240521147,10.7202093445295));
#74435=CARTESIAN_POINT('Ctrl Pts',(89.10925316698,62.9281980701916,10.7610855852075));
#74436=CARTESIAN_POINT('Ctrl Pts',(89.1571424888919,62.9233720882684,10.8045990999065));
#74437=CARTESIAN_POINT('Ctrl Pts',(89.2027617782286,62.9187748658211,10.8460500024847));
#74438=CARTESIAN_POINT('Ctrl Pts',(89.2462231695869,62.9141776433737,10.8900639566383));
#74439=CARTESIAN_POINT('Ctrl Pts',(89.2872250427154,62.9095804209263,10.9363874664532));
#74440=CARTESIAN_POINT('Ctrl Pts',(89.328928991157,62.9049044802121,10.9835041739972));
#74441=CARTESIAN_POINT('Ctrl Pts',(89.3680879435471,62.9002285394979,11.0330099884105));
#74442=CARTESIAN_POINT('Ctrl Pts',(89.4044207797161,62.8955525987837,11.0845962266961));
#74443=CARTESIAN_POINT('Ctrl Pts',(89.4400437060474,62.8909680216035,11.1351745178484));
#74444=CARTESIAN_POINT('Ctrl Pts',(89.472949655108,62.8863834444233,11.1877522288493));
#74445=CARTESIAN_POINT('Ctrl Pts',(89.5029134562567,62.8817988672431,11.2420042022922));
#74446=CARTESIAN_POINT('Ctrl Pts',(89.5328589439531,62.8772170920918,11.2962230176948));
#74447=CARTESIAN_POINT('Ctrl Pts',(89.5598656037087,62.8726353169405,11.3521136218362));
#74448=CARTESIAN_POINT('Ctrl Pts',(89.5837526961807,62.8680535417892,11.4093236777099));
#74449=CARTESIAN_POINT('Ctrl Pts',(89.6076339628515,62.8634728840828,11.4665197806754));
#74450=CARTESIAN_POINT('Ctrl Pts',(89.6283969765519,62.8588922263765,11.5250342270168));
#74451=CARTESIAN_POINT('Ctrl Pts',(89.6459087681079,62.8543115686701,11.584493867574));
#74452=CARTESIAN_POINT('Ctrl Pts',(89.6640532105012,62.8495654249297,11.6461016145237));
#74453=CARTESIAN_POINT('Ctrl Pts',(89.6787067925887,62.8448192811893,11.7087236179717));
#74454=CARTESIAN_POINT('Ctrl Pts',(89.6897784786873,62.8400731374489,11.7719291665323));
#74455=CARTESIAN_POINT('Ctrl Pts',(89.7004776586677,62.8354866773885,11.8330081687542));
#74456=CARTESIAN_POINT('Ctrl Pts',(89.7078321649599,62.8309002173282,11.8946315377005));
#74457=CARTESIAN_POINT('Ctrl Pts',(89.7118126304884,62.8263137572678,11.9564042356148));
#74458=CARTESIAN_POINT('Ctrl Pts',(89.7160009737839,62.8214877716874,12.0214029809383));
#74459=CARTESIAN_POINT('Ctrl Pts',(89.716453181955,62.816661786107,12.0865664362988));
#74460=CARTESIAN_POINT('Ctrl Pts',(89.7131972496079,62.8118358005265,12.1514362863616));
#74461=CARTESIAN_POINT('Ctrl Pts',(89.7099413172608,62.8070098149461,12.2163061364244));
#74462=CARTESIAN_POINT('Ctrl Pts',(89.7029773908056,62.8021838293657,12.2808817452318));
#74463=CARTESIAN_POINT('Ctrl Pts',(89.6923958654503,62.7973578437852,12.3447163060295));
#74464=CARTESIAN_POINT('Ctrl Pts',(89.6823159258857,62.7927606197219,12.4055249790108));
#74465=CARTESIAN_POINT('Ctrl Pts',(89.6689122687689,62.7881633956585,12.4659109509055));
#74466=CARTESIAN_POINT('Ctrl Pts',(89.6522342632398,62.7835661715951,12.5254833280629));
#74467=CARTESIAN_POINT('Ctrl Pts',(89.6352706868203,62.7788902310829,12.5860757394659));
#74468=CARTESIAN_POINT('Ctrl Pts',(89.6149195688735,62.7742142905707,12.6458258934939));
#74469=CARTESIAN_POINT('Ctrl Pts',(89.5912877614663,62.7695383500585,12.7043301861575));
#74470=CARTESIAN_POINT('Ctrl Pts',(89.5681176881313,62.7649537712021,12.7616913827882));
#74471=CARTESIAN_POINT('Ctrl Pts',(89.541794172757,62.7603691923457,12.8178544705603));
#74472=CARTESIAN_POINT('Ctrl Pts',(89.5124682549575,62.7557846134893,12.8724539137204));
#74473=CARTESIAN_POINT('Ctrl Pts',(89.4831602606247,62.751202836644,12.9270199866956));
#74474=CARTESIAN_POINT('Ctrl Pts',(89.4508537428031,62.7466210597986,12.9800238624931));
#74475=CARTESIAN_POINT('Ctrl Pts',(89.4157466747345,62.7420392829533,13.0311225908777));
#74476=CARTESIAN_POINT('Ctrl Pts',(89.3806481687782,62.7374586235379,13.0822088570124));
#74477=CARTESIAN_POINT('Ctrl Pts',(89.3427507565923,62.7328779641225,13.1313904787341));
#74478=CARTESIAN_POINT('Ctrl Pts',(89.3022958066175,62.7282973047071,13.17835335007));
#74479=CARTESIAN_POINT('Ctrl Pts',(89.260379365226,62.72355116259,13.2270128205465));
#74480=CARTESIAN_POINT('Ctrl Pts',(89.2157173897576,62.7188050204729,13.2732896781071));
#74481=CARTESIAN_POINT('Ctrl Pts',(89.1686223518987,62.7140588783558,13.3168738249657));
#74482=CARTESIAN_POINT('Ctrl Pts',(89.1231117906529,62.7094724165687,13.3589916164601));
#74483=CARTESIAN_POINT('Ctrl Pts',(89.0753297472791,62.7048859547816,13.398594738683));
#74484=CARTESIAN_POINT('Ctrl Pts',(89.0255921728988,62.7002994929946,13.4354442516191));
#74485=CARTESIAN_POINT('Ctrl Pts',(88.9732571347242,62.6954735107125,13.4742181703365));
#74486=CARTESIAN_POINT('Ctrl Pts',(88.9187572485301,62.6906475284304,13.509942625556));
#74487=CARTESIAN_POINT('Ctrl Pts',(88.8624927379216,62.6858215461483,13.54239254701));
#74488=CARTESIAN_POINT('Ctrl Pts',(88.8062282273131,62.6809955638662,13.5748424684641));
#74489=CARTESIAN_POINT('Ctrl Pts',(88.7481997059805,62.6761695815841,13.6040176342137));
#74490=CARTESIAN_POINT('Ctrl Pts',(88.6888315748493,62.671343599302,13.6297516400431));
#74491=CARTESIAN_POINT('Ctrl Pts',(88.6322775804682,62.6667463756794,13.6542658161396));
#74492=CARTESIAN_POINT('Ctrl Pts',(88.5742759260267,62.6621491520569,13.6757583949161));
#74493=CARTESIAN_POINT('Ctrl Pts',(88.5151817872298,62.6575519284343,13.6940588321758));
#74494=CARTESIAN_POINT('Ctrl Pts',(88.4550757964022,62.652875987867,13.7126726225867));
#74495=CARTESIAN_POINT('Ctrl Pts',(88.3938400052592,62.6482000472997,13.7279836282808));
#74496=CARTESIAN_POINT('Ctrl Pts',(88.331871446533,62.6435241067324,13.7398627035691));
#74497=CARTESIAN_POINT('Ctrl Pts',(88.271113677649,62.6389395283245,13.751509676256));
#74498=CARTESIAN_POINT('Ctrl Pts',(88.2096520422967,62.6343549499166,13.7598575234163));
#74499=CARTESIAN_POINT('Ctrl Pts',(88.1478755584302,62.6297703715087,13.764834870464));
#74500=CARTESIAN_POINT('Ctrl Pts',(88.0861368312507,62.6251885951134,13.7698091754458));
#74501=CARTESIAN_POINT('Ctrl Pts',(88.0240841434678,62.6206068187182,13.7714170241801));
#74502=CARTESIAN_POINT('Ctrl Pts',(87.9621129952099,62.616025042323,13.7696387223712));
#74503=CARTESIAN_POINT('Ctrl Pts',(87.9001569608432,62.6114443833586,13.7678608542651));
#74504=CARTESIAN_POINT('Ctrl Pts',(87.8382829351339,62.6068637243942,13.7626984896173));
#74505=CARTESIAN_POINT('Ctrl Pts',(87.7768857230408,62.6022830654298,13.7541840364498));
#74506=CARTESIAN_POINT('Ctrl Pts',(87.7132704390637,62.5975369228789,13.745361985127));
#74507=CARTESIAN_POINT('Ctrl Pts',(87.6501676643083,62.592790780328,13.732941025464));
#74508=CARTESIAN_POINT('Ctrl Pts',(87.5880074029217,62.588044637777,13.7170154749175));
#74509=CARTESIAN_POINT('Ctrl Pts',(87.5279384874551,62.5834581764378,13.7016257302767));
#74510=CARTESIAN_POINT('Ctrl Pts',(87.468750149575,62.5788717150986,13.6829637124893));
#74511=CARTESIAN_POINT('Ctrl Pts',(87.4108144992807,62.5742852537594,13.6611652579988));
#74512=CARTESIAN_POINT('Ctrl Pts',(87.3498532370308,62.5694592706027,13.6382284083373));
#74513=CARTESIAN_POINT('Ctrl Pts',(87.2902796832104,62.5646332874459,13.6118187974817));
#74514=CARTESIAN_POINT('Ctrl Pts',(87.232500005162,62.5598073042891,13.5821505840903));
#74515=CARTESIAN_POINT('Ctrl Pts',(87.1747203271136,62.5549813211323,13.5524823706988));
#74516=CARTESIAN_POINT('Ctrl Pts',(87.1187350441588,62.5501553379755,13.5195559499669));
#74517=CARTESIAN_POINT('Ctrl Pts',(87.0649141507492,62.5453293548187,13.4836376128783));
#74518=CARTESIAN_POINT('Ctrl Pts',(87.0137790463661,62.5407441995595,13.449511685196));
#74519=CARTESIAN_POINT('Ctrl Pts',(86.9643850283897,62.5361590443002,13.4125435669695));
#74520=CARTESIAN_POINT('Ctrl Pts',(86.9170670094507,62.531573889041,13.3729374307089));
#74521=CARTESIAN_POINT('Ctrl Pts',(86.8696221089916,62.5269764388573,13.3332250920566));
#74522=CARTESIAN_POINT('Ctrl Pts',(86.8242648202487,62.5223789886736,13.290860805712));
#74523=CARTESIAN_POINT('Ctrl Pts',(86.7813047057607,62.5177815384898,13.2460950465644));
#74524=CARTESIAN_POINT('Ctrl Pts',(86.7385766298091,62.5132089203072,13.2015710787005));
#74525=CARTESIAN_POINT('Ctrl Pts',(86.6982202733338,62.5086363021247,13.1546718683068));
#74526=CARTESIAN_POINT('Ctrl Pts',(86.6605063021084,62.5040636839421,13.1056834169858));
#74527=CARTESIAN_POINT('Ctrl Pts',(86.6228152326411,62.4994938424757,13.0567247138355));
#74528=CARTESIAN_POINT('Ctrl Pts',(86.5877636789865,62.4949240010093,13.0056796899132));
#74529=CARTESIAN_POINT('Ctrl Pts',(86.5555825005124,62.4903541595429,12.9528679370601));
#74530=CARTESIAN_POINT('Ctrl Pts',(86.5234088769549,62.4857853909015,12.9000685823978));
#74531=CARTESIAN_POINT('Ctrl Pts',(86.4941045572299,62.48121662226,12.8455037592586));
#74532=CARTESIAN_POINT('Ctrl Pts',(86.4678563091501,62.4766478536186,12.78952082554));
#74533=CARTESIAN_POINT('Ctrl Pts',(86.4413267665586,62.4720301228697,12.7329379397046));
#74534=CARTESIAN_POINT('Ctrl Pts',(86.4179194492552,62.4674123921208,12.674906833083));
#74535=CARTESIAN_POINT('Ctrl Pts',(86.3977778179899,62.4627946613718,12.6158081729755));
#74536=CARTESIAN_POINT('Ctrl Pts',(86.3778244481651,62.458220092005,12.5572619010403));
#74537=CARTESIAN_POINT('Ctrl Pts',(86.3610760526445,62.4536455226381,12.4976684658435));
#74538=CARTESIAN_POINT('Ctrl Pts',(86.347621530971,62.4490709532713,12.4374120412304));
#74539=CARTESIAN_POINT('Ctrl Pts',(86.3339765927674,62.4444316418314,12.3763028312437));
#74540=CARTESIAN_POINT('Ctrl Pts',(86.3237195974269,62.4397923303914,12.3145122529744));
#74541=CARTESIAN_POINT('Ctrl Pts',(86.3168890009944,62.4351530189515,12.2524477370426));
#74542=CARTESIAN_POINT('Ctrl Pts',(86.3100584045619,62.4305137075115,12.1903832211108));
#74543=CARTESIAN_POINT('Ctrl Pts',(86.306654169042,62.4258743960716,12.1280453121899));
#74544=CARTESIAN_POINT('Ctrl Pts',(86.306660007507,62.4212350846317,12.0658400339999));
#74545=CARTESIAN_POINT('',(86.3066606648187,61.6274850846366,12.0675053748877));
#74546=CARTESIAN_POINT('Ctrl Pts',(86.3066600075071,62.4212350845702,12.0658400331759));
#74547=CARTESIAN_POINT('Ctrl Pts',(86.3066608129255,62.4205950931586,12.0572588365243));
#74548=CARTESIAN_POINT('Ctrl Pts',(86.3067264261332,62.4199551017471,12.0486779912057));
#74549=CARTESIAN_POINT('Ctrl Pts',(86.3068568343893,62.4193151103355,12.0400981332293));
#74550=CARTESIAN_POINT('Ctrl Pts',(86.3077935905844,62.4147178866782,11.9784667966938));
#74551=CARTESIAN_POINT('Ctrl Pts',(86.3120799811377,62.4101206630209,11.9167598298027));
#74552=CARTESIAN_POINT('Ctrl Pts',(86.3197252405793,62.4055234393636,11.8553711231895));
#74553=CARTESIAN_POINT('Ctrl Pts',(86.3275014075449,62.4008474988007,11.792931275847));
#74554=CARTESIAN_POINT('Ctrl Pts',(86.3387526387959,62.3961715582377,11.7308212219863));
#74555=CARTESIAN_POINT('Ctrl Pts',(86.3534332112112,62.3914956176747,11.6694559591868));
#74556=CARTESIAN_POINT('Ctrl Pts',(86.3678269433106,62.3869110392351,11.6092896980933));
#74557=CARTESIAN_POINT('Ctrl Pts',(86.3855170874842,62.3823264607956,11.5498399039925));
#74558=CARTESIAN_POINT('Ctrl Pts',(86.4064085691986,62.377741882356,11.4914904911155));
#74559=CARTESIAN_POINT('Ctrl Pts',(86.4272872824058,62.3731601059303,11.4331767403761));
#74560=CARTESIAN_POINT('Ctrl Pts',(86.4513632822594,62.3685783295047,11.3759625155834));
#74561=CARTESIAN_POINT('Ctrl Pts',(86.4784917266961,62.363996553079,11.3202163665947));
#74562=CARTESIAN_POINT('Ctrl Pts',(86.5056135548793,62.3594158940855,11.264483813323));
#74563=CARTESIAN_POINT('Ctrl Pts',(86.5357861271527,62.3548352350919,11.2102190826047));
#74564=CARTESIAN_POINT('Ctrl Pts',(86.56881740355,62.3502545760984,11.1577686450597));
#74565=CARTESIAN_POINT('Ctrl Pts',(86.6030419868765,62.3455084335778,11.1034233527774));
#74566=CARTESIAN_POINT('Ctrl Pts',(86.6403355237341,62.3407622910574,11.0510264780217));
#74567=CARTESIAN_POINT('Ctrl Pts',(86.6804350640614,62.3360161485369,11.0009310882151));
#74568=CARTESIAN_POINT('Ctrl Pts',(86.7191854790905,62.3314296871721,10.9525211281456));
#74569=CARTESIAN_POINT('Ctrl Pts',(86.7605556654545,62.3268432258073,10.9062605835551));
#74570=CARTESIAN_POINT('Ctrl Pts',(86.8042686639268,62.3222567644425,10.8624326698771));
#74571=CARTESIAN_POINT('Ctrl Pts',(86.8502645145462,62.3174307813442,10.8163159027611));
#74572=CARTESIAN_POINT('Ctrl Pts',(86.8988541147888,62.3126047982458,10.7728932528154));
#74573=CARTESIAN_POINT('Ctrl Pts',(86.9496751073592,62.3077788151474,10.732446736024));
#74574=CARTESIAN_POINT('Ctrl Pts',(87.0004960999296,62.3029528320491,10.6920002192326));
#74575=CARTESIAN_POINT('Ctrl Pts',(87.0535479109055,62.2981268489507,10.6545301462196));
#74576=CARTESIAN_POINT('Ctrl Pts',(87.1084355606251,62.2933008658524,10.6202641083601));
#74577=CARTESIAN_POINT('Ctrl Pts',(87.1607214457935,62.2887036422621,10.5876223368532));
#74578=CARTESIAN_POINT('Ctrl Pts',(87.2148877071279,62.2841064186718,10.5577536421674));
#74579=CARTESIAN_POINT('Ctrl Pts',(87.2706084375798,62.2795091950815,10.5308794282217));
#74580=CARTESIAN_POINT('Ctrl Pts',(87.3272832586035,62.2748332545102,10.5035450545842));
#74581=CARTESIAN_POINT('Ctrl Pts',(87.3855658837477,62.2701573139388,10.4793090355932));
#74582=CARTESIAN_POINT('Ctrl Pts',(87.4450828645907,62.2654813733675,10.4583580524724));
#74583=CARTESIAN_POINT('Ctrl Pts',(87.5034369559052,62.2608967949965,10.4378164261191));
#74584=CARTESIAN_POINT('Ctrl Pts',(87.562977097953,62.2563122166254,10.4204327960473));
#74585=CARTESIAN_POINT('Ctrl Pts',(87.6233291879626,62.2517276382544,10.4063355227353));
#74586=CARTESIAN_POINT('Ctrl Pts',(87.6836443918281,62.2471458618977,10.3922468654307));
#74587=CARTESIAN_POINT('Ctrl Pts',(87.7447700649916,62.2425640855409,10.3814406977421));
#74588=CARTESIAN_POINT('Ctrl Pts',(87.8063180187702,62.2379823091842,10.3739952357751));
#74589=CARTESIAN_POINT('Ctrl Pts',(87.8678509618479,62.2334016502598,10.366551589654));
#74590=CARTESIAN_POINT('Ctrl Pts',(87.9298054759566,62.2288209913354,10.3624670832712));
#74591=CARTESIAN_POINT('Ctrl Pts',(87.9917863215632,62.224240332411,10.361768305024));
#74592=CARTESIAN_POINT('Ctrl Pts',(88.0560063247892,62.2194941898242,10.3610442822899));
#74593=CARTESIAN_POINT('Ctrl Pts',(88.1202540178258,62.2147480472374,10.3639553717578));
#74594=CARTESIAN_POINT('Ctrl Pts',(88.1840901574413,62.2100019046506,10.3704721668469));
#74595=CARTESIAN_POINT('Ctrl Pts',(88.2457785661354,62.2054154433548,10.3767697080399));
#74596=CARTESIAN_POINT('Ctrl Pts',(88.3070821661325,62.2008289820591,10.3864340147995));
#74597=CARTESIAN_POINT('Ctrl Pts',(88.3676127998188,62.1962425207633,10.3993860235179));
#74598=CARTESIAN_POINT('Ctrl Pts',(88.4313045666032,62.1914165375309,10.413014433935));
#74599=CARTESIAN_POINT('Ctrl Pts',(88.494139795063,62.1865905542986,10.4302831943551));
#74600=CARTESIAN_POINT('Ctrl Pts',(88.5556850154075,62.1817645710662,10.4510408458446));
#74601=CARTESIAN_POINT('Ctrl Pts',(88.6172302357521,62.1769385878338,10.471798497334));
#74602=CARTESIAN_POINT('Ctrl Pts',(88.6774848757244,62.1721126046015,10.4960447262106));
#74603=CARTESIAN_POINT('Ctrl Pts',(88.7360434944745,62.1672866213691,10.5235711469503));
#74604=CARTESIAN_POINT('Ctrl Pts',(88.7918263370121,62.1626893977923,10.5497927694292));
#74605=CARTESIAN_POINT('Ctrl Pts',(88.8462993727308,62.1580921742156,10.5790982491545));
#74606=CARTESIAN_POINT('Ctrl Pts',(88.8990998239316,62.1534949506388,10.611333873931));
#74607=CARTESIAN_POINT('Ctrl Pts',(88.9528043627521,62.1488190100658,10.6441214604542));
#74608=CARTESIAN_POINT('Ctrl Pts',(89.0047779792158,62.1441430694927,10.6799403409917));
#74609=CARTESIAN_POINT('Ctrl Pts',(89.0546612805093,62.1394671289197,10.7185780292849));
#74610=CARTESIAN_POINT('Ctrl Pts',(89.1035699224995,62.1348825505633,10.7564607839356));
#74611=CARTESIAN_POINT('Ctrl Pts',(89.1504687774279,62.1302979722069,10.7970528581824));
#74612=CARTESIAN_POINT('Ctrl Pts',(89.1950470940587,62.1257133938505,10.8401095829352));
#74613=CARTESIAN_POINT('Ctrl Pts',(89.2395981651965,62.1211316175088,10.8831399921656));
#74614=CARTESIAN_POINT('Ctrl Pts',(89.281831144881,62.1165498411671,10.9286317121107));
#74615=CARTESIAN_POINT('Ctrl Pts',(89.3214697690442,62.1119680648254,10.9763010415619));
#74616=CARTESIAN_POINT('Ctrl Pts',(89.3610987258882,62.1073874059164,11.0239587451144));
#74617=CARTESIAN_POINT('Ctrl Pts',(89.3981342579493,62.1028067470074,11.0737926126485));
#74618=CARTESIAN_POINT('Ctrl Pts',(89.4323396503179,62.0982260880984,11.1254850165818));
#74619=CARTESIAN_POINT('Ctrl Pts',(89.4677807676618,62.0934799454973,11.179044891991));
#74620=CARTESIAN_POINT('Ctrl Pts',(89.5001829691893,62.0887338028963,11.234599710581));
#74621=CARTESIAN_POINT('Ctrl Pts',(89.529332715001,62.0839876602952,11.291764504716));
#74622=CARTESIAN_POINT('Ctrl Pts',(89.5575017338686,62.0794011990156,11.3470060212271));
#74623=CARTESIAN_POINT('Ctrl Pts',(89.5826335419652,62.0748147377359,11.4037503812814));
#74624=CARTESIAN_POINT('Ctrl Pts',(89.6045840260914,62.0702282764563,11.4616286014491));
#74625=CARTESIAN_POINT('Ctrl Pts',(89.6276808457352,62.0654022931945,11.5225294364757));
#74626=CARTESIAN_POINT('Ctrl Pts',(89.6472547448984,62.0605763099328,11.5846851968848));
#74627=CARTESIAN_POINT('Ctrl Pts',(89.6631978539558,62.0557503266711,11.6476495643794));
#74628=CARTESIAN_POINT('Ctrl Pts',(89.6791409630131,62.0509243434093,11.710613931874));
#74629=CARTESIAN_POINT('Ctrl Pts',(89.6914532351042,62.0460983601476,11.7743862555481));
#74630=CARTESIAN_POINT('Ctrl Pts',(89.700089828703,62.0412723768858,11.8385128878986));
#74631=CARTESIAN_POINT('Ctrl Pts',(89.7083170333511,62.036675153285,11.8995998108521));
#74632=CARTESIAN_POINT('Ctrl Pts',(89.7132429865986,62.0320779296842,11.9612590177146));
#74633=CARTESIAN_POINT('Ctrl Pts',(89.7148000551434,62.0274807060833,12.0231023579518));
#74634=CARTESIAN_POINT('Ctrl Pts',(89.7163837849359,62.0228047655133,12.0860046243433));
#74635=CARTESIAN_POINT('Ctrl Pts',(89.7144820103083,62.0181288249433,12.1490968763259));
#74636=CARTESIAN_POINT('Ctrl Pts',(89.7090783112516,62.0134528843732,12.2119619281077));
#74637=CARTESIAN_POINT('Ctrl Pts',(89.7037801938987,62.0088683059918,12.2735986732782));
#74638=CARTESIAN_POINT('Ctrl Pts',(89.6951158137425,62.0042837276103,12.3350164853722));
#74639=CARTESIAN_POINT('Ctrl Pts',(89.683122171383,61.9996991492289,12.3958215874824));
#74640=CARTESIAN_POINT('Ctrl Pts',(89.6711358593285,61.9951173728618,12.4565895265744));
#74641=CARTESIAN_POINT('Ctrl Pts',(89.6558244180651,61.9905355964947,12.5167449998295));
#74642=CARTESIAN_POINT('Ctrl Pts',(89.6372763456987,61.9859538201276,12.575902032768));
#74643=CARTESIAN_POINT('Ctrl Pts',(89.6187327969528,61.981373161193,12.6350446381171));
#74644=CARTESIAN_POINT('Ctrl Pts',(89.5969543363508,61.9767925022584,12.693188801032));
#74645=CARTESIAN_POINT('Ctrl Pts',(89.572079415678,61.9722118433237,12.7499633714948));
#74646=CARTESIAN_POINT('Ctrl Pts',(89.5463058486468,61.967465700747,12.8087890142671));
#74647=CARTESIAN_POINT('Ctrl Pts',(89.5172079834779,61.9627195581702,12.8661436542454));
#74648=CARTESIAN_POINT('Ctrl Pts',(89.4849934158513,61.9579734155935,12.9216390860795));
#74649=CARTESIAN_POINT('Ctrl Pts',(89.4538626890542,61.9533869542878,12.9752674056317));
#74650=CARTESIAN_POINT('Ctrl Pts',(89.4198220121885,61.9488004929822,13.0271592405708));
#74651=CARTESIAN_POINT('Ctrl Pts',(89.3831032092268,61.9442140316766,13.0769933821888));
#74652=CARTESIAN_POINT('Ctrl Pts',(89.3444668150961,61.9393880484642,13.1294300462794));
#74653=CARTESIAN_POINT('Ctrl Pts',(89.302865303941,61.9345620652519,13.1795877003108));
#74654=CARTESIAN_POINT('Ctrl Pts',(89.258615128848,61.9297360820396,13.2271336382474));
#74655=CARTESIAN_POINT('Ctrl Pts',(89.214364953755,61.9249100988273,13.274679576184));
#74656=CARTESIAN_POINT('Ctrl Pts',(89.1674666361469,61.920084115615,13.3196134056069));
#74657=CARTESIAN_POINT('Ctrl Pts',(89.1182769728918,61.9152581324026,13.3616513963654));
#74658=CARTESIAN_POINT('Ctrl Pts',(89.0714189813886,61.9106609088115,13.4016967165287));
#74659=CARTESIAN_POINT('Ctrl Pts',(89.0222896073878,61.9060636852203,13.4392789915989));
#74660=CARTESIAN_POINT('Ctrl Pts',(88.9711782601494,61.9014664616292,13.4741308690376));
#74661=CARTESIAN_POINT('Ctrl Pts',(88.9191917475371,61.8967905210579,13.5095795054739));
#74662=CARTESIAN_POINT('Ctrl Pts',(88.8651550907164,61.8921145804867,13.5422029438071));
#74663=CARTESIAN_POINT('Ctrl Pts',(88.8094098701109,61.8874386399155,13.5717611081807));
#74664=CARTESIAN_POINT('Ctrl Pts',(88.7547538434122,61.882854061544,13.6007417419214));
#74665=CARTESIAN_POINT('Ctrl Pts',(88.6984558902489,61.8782694831724,13.6267755579987));
#74666=CARTESIAN_POINT('Ctrl Pts',(88.6408669000153,61.8736849048009,13.6496800572922));
#74667=CARTESIAN_POINT('Ctrl Pts',(88.5833131071693,61.8691031284439,13.6725705577548));
#74668=CARTESIAN_POINT('Ctrl Pts',(88.524470313871,61.8645213520868,13.6923353460748));
#74669=CARTESIAN_POINT('Ctrl Pts',(88.4647107867141,61.8599395757297,13.7088394193041));
#74670=CARTESIAN_POINT('Ctrl Pts',(88.4049658340872,61.8553589168051,13.7253394674159));
#74671=CARTESIAN_POINT('Ctrl Pts',(88.3443050818981,61.8507782578806,13.7385802436641));
#74672=CARTESIAN_POINT('Ctrl Pts',(88.2831154372097,61.846197598956,13.7484767530139));
#74673=CARTESIAN_POINT('Ctrl Pts',(88.2197152183149,61.8414514563696,13.7587307896613));
#74674=CARTESIAN_POINT('Ctrl Pts',(88.1557477248056,61.8367053137832,13.7653941429532));
#74675=CARTESIAN_POINT('Ctrl Pts',(88.0916516958592,61.8319591711968,13.7684306563132));
#74676=CARTESIAN_POINT('Ctrl Pts',(88.0297121416607,61.8273727099013,13.7713650078936));
#74677=CARTESIAN_POINT('Ctrl Pts',(87.9676530916298,61.8227862486057,13.7709127817225));
#74678=CARTESIAN_POINT('Ctrl Pts',(87.9058701410369,61.8181997873101,13.7670945148211));
#74679=CARTESIAN_POINT('Ctrl Pts',(87.8408606567402,61.8133738040784,13.7630768439299));
#74680=CARTESIAN_POINT('Ctrl Pts',(87.7761575412377,61.8085478208466,13.7553319831836));
#74681=CARTESIAN_POINT('Ctrl Pts',(87.7122119516828,61.8037218376148,13.7439453321795));
#74682=CARTESIAN_POINT('Ctrl Pts',(87.648266362128,61.798895854383,13.7325586811753));
#74683=CARTESIAN_POINT('Ctrl Pts',(87.5850789110193,61.7940698711512,13.717530465124));
#74684=CARTESIAN_POINT('Ctrl Pts',(87.5230814922492,61.7892438879194,13.6990065417488));
#74685=CARTESIAN_POINT('Ctrl Pts',(87.4640228543667,61.7846466643291,13.6813606831874));
#74686=CARTESIAN_POINT('Ctrl Pts',(87.4058014777533,61.7800494407387,13.660470635492));
#74687=CARTESIAN_POINT('Ctrl Pts',(87.3487989461613,61.7754522171483,13.6364345258224));
#74688=CARTESIAN_POINT('Ctrl Pts',(87.2908203760746,61.7707762765769,13.6119868525318));
#74689=CARTESIAN_POINT('Ctrl Pts',(87.2341033190426,61.7661003360056,13.5842844257315));
#74690=CARTESIAN_POINT('Ctrl Pts',(87.1790347406746,61.7614243954343,13.5534839975192));
#74691=CARTESIAN_POINT('Ctrl Pts',(87.1250421354572,61.7568398170636,13.5232853722726));
#74692=CARTESIAN_POINT('Ctrl Pts',(87.072634635261,61.752255238693,13.4901089795872));
#74693=CARTESIAN_POINT('Ctrl Pts',(87.0221558834339,61.7476706603223,13.4541506217744));
#74694=CARTESIAN_POINT('Ctrl Pts',(86.971707983341,61.7430888839662,13.4182142410838));
#74695=CARTESIAN_POINT('Ctrl Pts',(86.9231869079409,61.73850710761,13.3794995614247));
#74696=CARTESIAN_POINT('Ctrl Pts',(86.8769079930086,61.7339253312539,13.3382461064111));
#74697=CARTESIAN_POINT('Ctrl Pts',(86.8306403648701,61.7293446723302,13.2970027125505));
#74698=CARTESIAN_POINT('Ctrl Pts',(86.7866141914748,61.7247640134066,13.2532221110623));
#74699=CARTESIAN_POINT('Ctrl Pts',(86.7451107368634,61.720183354483,13.2071832495596));
#74700=CARTESIAN_POINT('Ctrl Pts',(86.7021079032683,61.7154372118957,13.159481160212));
#74701=CARTESIAN_POINT('Ctrl Pts',(86.6618139897296,61.7106910693085,13.1093549092388));
#74702=CARTESIAN_POINT('Ctrl Pts',(86.6244973437402,61.7059449267213,13.0571534794292));
#74703=CARTESIAN_POINT('Ctrl Pts',(86.5884361952756,61.7013584654267,13.0067083373078));
#74704=CARTESIAN_POINT('Ctrl Pts',(86.555155368084,61.6967720041322,12.9543259286243));
#74705=CARTESIAN_POINT('Ctrl Pts',(86.5248521789646,61.6921855428377,12.9003497405954));
#74706=CARTESIAN_POINT('Ctrl Pts',(86.4929664454496,61.6873595596041,12.8435547167826));
#74707=CARTESIAN_POINT('Ctrl Pts',(86.4643781770976,61.6825335763705,12.7849954567107));
#74708=CARTESIAN_POINT('Ctrl Pts',(86.4392603349813,61.677707593137,12.7250973076921));
#74709=CARTESIAN_POINT('Ctrl Pts',(86.414142492865,61.6728816099034,12.6651991586735));
#74710=CARTESIAN_POINT('Ctrl Pts',(86.3924952199985,61.6680556266698,12.6039627574354));
#74711=CARTESIAN_POINT('Ctrl Pts',(86.3744302369339,61.6632296434362,12.5418300602294));
#74712=CARTESIAN_POINT('Ctrl Pts',(86.3521299505428,61.6572722169696,12.4651304620624));
#74713=CARTESIAN_POINT('Ctrl Pts',(86.335208780096,61.651314790503,12.3868010792025));
#74714=CARTESIAN_POINT('Ctrl Pts',(86.3238591749853,61.6453573640364,12.3075174365728));
#74715=CARTESIAN_POINT('Ctrl Pts',(86.313151704821,61.6397369952637,12.2327194828383));
#74716=CARTESIAN_POINT('Ctrl Pts',(86.3074028970101,61.6341166264909,12.1570722506466));
#74717=CARTESIAN_POINT('Ctrl Pts',(86.3067274670126,61.6284962577181,12.0811647256718));
#74718=CARTESIAN_POINT('Ctrl Pts',(86.3066869609735,61.6281592000243,12.0766124949644));
#74719=CARTESIAN_POINT('Ctrl Pts',(86.3066646871496,61.6278221423304,12.072059334826));
#74720=CARTESIAN_POINT('Ctrl Pts',(86.3066606648186,61.6274850846366,12.0675053748877));
#74721=CARTESIAN_POINT('',(86.3066601613137,60.8337350845235,12.065258469835));
#74722=CARTESIAN_POINT('Ctrl Pts',(86.3066606648178,61.6274850845702,12.0675053739911));
#74723=CARTESIAN_POINT('Ctrl Pts',(86.306606406938,61.6229384555704,12.0060762278913));
#74724=CARTESIAN_POINT('Ctrl Pts',(86.3098775506704,61.6183918265706,11.9445793182848));
#74725=CARTESIAN_POINT('Ctrl Pts',(86.3164694016912,61.6138451975707,11.8834051287813));
#74726=CARTESIAN_POINT('Ctrl Pts',(86.3230581031606,61.6093007409262,11.8222601679815));
#74727=CARTESIAN_POINT('Ctrl Pts',(86.3329643112659,61.6047562842816,11.7614381359344));
#74728=CARTESIAN_POINT('Ctrl Pts',(86.3461313706499,61.600211827637,11.7013257856581));
#74729=CARTESIAN_POINT('Ctrl Pts',(86.3592971677434,61.5956678066573,11.6412191981911));
#74730=CARTESIAN_POINT('Ctrl Pts',(86.3757230830511,61.5911237856775,11.5818226629785));
#74731=CARTESIAN_POINT('Ctrl Pts',(86.3953015242927,61.5865797646978,11.5235119621622));
#74732=CARTESIAN_POINT('Ctrl Pts',(86.414899289768,61.5820312586969,11.4651437077544));
#74733=CARTESIAN_POINT('Ctrl Pts',(86.4376556276918,61.577482752696,11.407863919384));
#74734=CARTESIAN_POINT('Ctrl Pts',(86.4634137187882,61.572934246695,11.3520311366698));
#74735=CARTESIAN_POINT('Ctrl Pts',(86.4891853727869,61.5683833456819,11.2961689552485));
#74736=CARTESIAN_POINT('Ctrl Pts',(86.5179616824663,61.5638324446688,11.2417557537004));
#74737=CARTESIAN_POINT('Ctrl Pts',(86.5495399535247,61.5592815436557,11.1891252266392));
#74738=CARTESIAN_POINT('Ctrl Pts',(86.581175969965,61.5547223206696,11.1363984571373));
#74739=CARTESIAN_POINT('Ctrl Pts',(86.6156238843628,61.5501630976836,11.0854612979128));
#74740=CARTESIAN_POINT('Ctrl Pts',(86.6526384547238,61.5456038746976,11.0366172976415));
#74741=CARTESIAN_POINT('Ctrl Pts',(86.6753393861925,61.542807716116,11.0066614102165));
#74742=CARTESIAN_POINT('Ctrl Pts',(86.6990049287886,61.5400115575345,10.9774921751297));
#74743=CARTESIAN_POINT('Ctrl Pts',(86.7235716774766,61.5372153989529,10.9491727304706));
#74744=CARTESIAN_POINT('Ctrl Pts',(86.7639623897164,61.5326181753611,10.9026121312417));
#74745=CARTESIAN_POINT('Ctrl Pts',(86.8069651078682,61.5280209517692,10.8581499110785));
#74746=CARTESIAN_POINT('Ctrl Pts',(86.8523333400228,61.5234237281773,10.8160934408296));
#74747=CARTESIAN_POINT('Ctrl Pts',(86.8984783997819,61.5187477876061,10.773316849353));
#74748=CARTESIAN_POINT('Ctrl Pts',(86.9470704683404,61.514071847035,10.7330296320008));
#74749=CARTESIAN_POINT('Ctrl Pts',(86.9978074100754,61.5093959064639,10.6955199339933));
#74750=CARTESIAN_POINT('Ctrl Pts',(87.0475530135985,61.5048113280916,10.6587431299221));
#74751=CARTESIAN_POINT('Ctrl Pts',(87.0993599987467,61.5002267497194,10.6246365997431));
#74752=CARTESIAN_POINT('Ctrl Pts',(87.1529084727936,61.4956421713472,10.5934329330939));
#74753=CARTESIAN_POINT('Ctrl Pts',(87.2064242189458,61.4910603949895,10.5622483375822));
#74754=CARTESIAN_POINT('Ctrl Pts',(87.2616789045999,61.4864786186317,10.5339633434187));
#74755=CARTESIAN_POINT('Ctrl Pts',(87.3183244427234,61.4818968422739,10.5087667458112));
#74756=CARTESIAN_POINT('Ctrl Pts',(87.3749561657757,61.4773161833487,10.4835762933088));
#74757=CARTESIAN_POINT('Ctrl Pts',(87.4329776030128,61.4727355244234,10.4614729489047));
#74758=CARTESIAN_POINT('Ctrl Pts',(87.4920187620624,61.4681548654982,10.4425982289437));
#74759=CARTESIAN_POINT('Ctrl Pts',(87.5531928778059,61.4634087229125,10.4230416294103));
#74760=CARTESIAN_POINT('Ctrl Pts',(87.6154612699018,61.4586625803268,10.4069516372537));
#74761=CARTESIAN_POINT('Ctrl Pts',(87.6783954351681,61.4539164377411,10.3944291701956));
#74762=CARTESIAN_POINT('Ctrl Pts',(87.7392122159518,61.4493299764449,10.3823280144765));
#74763=CARTESIAN_POINT('Ctrl Pts',(87.800650146486,61.4447435151487,10.3735581289527));
#74764=CARTESIAN_POINT('Ctrl Pts',(87.8623149687829,61.4401570538525,10.3681579587335));
#74765=CARTESIAN_POINT('Ctrl Pts',(87.9272001556612,61.435331070622,10.3624757716972));
#74766=CARTESIAN_POINT('Ctrl Pts',(87.9923359390259,61.4305050873916,10.3605249392997));
#74767=CARTESIAN_POINT('Ctrl Pts',(88.0572634817533,61.4256791041611,10.3622880155801));
#74768=CARTESIAN_POINT('Ctrl Pts',(88.1221910244806,61.4208531209306,10.3640510918604));
#74769=CARTESIAN_POINT('Ctrl Pts',(88.1869096874165,61.4160271377002,10.3695279450747));
#74770=CARTESIAN_POINT('Ctrl Pts',(88.250970703728,61.4112011544697,10.3786384806591));
#74771=CARTESIAN_POINT('Ctrl Pts',(88.311995121229,61.4066039308778,10.3873171616913));
#74772=CARTESIAN_POINT('Ctrl Pts',(88.372673394828,61.4020067072859,10.3993284023983));
#74773=CARTESIAN_POINT('Ctrl Pts',(88.4326135988613,61.397409483694,10.414631837277));
#74774=CARTESIAN_POINT('Ctrl Pts',(88.4935801423151,61.3927335431229,10.4301973086091));
#74775=CARTESIAN_POINT('Ctrl Pts',(88.5537825644107,61.3880576025517,10.449168797285));
#74776=CARTESIAN_POINT('Ctrl Pts',(88.61281491026,61.3833816619806,10.4714487623821));
#74777=CARTESIAN_POINT('Ctrl Pts',(88.6706938357778,61.3787970836084,10.4932934040246));
#74778=CARTESIAN_POINT('Ctrl Pts',(88.7274474985102,61.3742125052362,10.5183182092679));
#74779=CARTESIAN_POINT('Ctrl Pts',(88.7827069855596,61.3696279268639,10.5463805857918));
#74780=CARTESIAN_POINT('Ctrl Pts',(88.8379326989729,61.3650461505062,10.5744258110798));
#74781=CARTESIAN_POINT('Ctrl Pts',(88.8916655945412,61.3604643741484,10.6055046964431));
#74782=CARTESIAN_POINT('Ctrl Pts',(88.9435582594377,61.3558825977906,10.6394272088833));
#74783=CARTESIAN_POINT('Ctrl Pts',(88.9954382684238,61.3513019388654,10.6733414480872));
#74784=CARTESIAN_POINT('Ctrl Pts',(89.0454785117945,61.3467212799401,10.7100976592132));
#74785=CARTESIAN_POINT('Ctrl Pts',(89.0933594152672,61.3421406210148,10.7494617621268));
#74786=CARTESIAN_POINT('Ctrl Pts',(89.142970093277,61.3373944784292,10.7902479564787));
#74787=CARTESIAN_POINT('Ctrl Pts',(89.1902619351784,61.3326483358435,10.8338337591143));
#74788=CARTESIAN_POINT('Ctrl Pts',(89.2349177382608,61.3279021932578,10.8799139130862));
#74789=CARTESIAN_POINT('Ctrl Pts',(89.2780711220437,61.3233157319616,10.9244437262764));
#74790=CARTESIAN_POINT('Ctrl Pts',(89.3187627460656,61.3187292706654,10.9713022573559));
#74791=CARTESIAN_POINT('Ctrl Pts',(89.3567464667318,61.3141428093692,11.0201791344217));
#74792=CARTESIAN_POINT('Ctrl Pts',(89.3967138374619,61.3093168261387,11.0716085423776));
#74793=CARTESIAN_POINT('Ctrl Pts',(89.433682341388,61.3044908429083,11.1252723638878));
#74794=CARTESIAN_POINT('Ctrl Pts',(89.4674177625429,61.2996648596779,11.1807756575028));
#74795=CARTESIAN_POINT('Ctrl Pts',(89.5011531836978,61.2948388764474,11.2362789511179));
#74796=CARTESIAN_POINT('Ctrl Pts',(89.5316552860858,61.290012893217,11.2936211084133));
#74797=CARTESIAN_POINT('Ctrl Pts',(89.5587479482707,61.2851869099865,11.3523816676796));
#74798=CARTESIAN_POINT('Ctrl Pts',(89.5845563731709,61.2805896863943,11.4083568786268));
#74799=CARTESIAN_POINT('Ctrl Pts',(89.6073772961101,61.2759924628021,11.4658488629993));
#74800=CARTESIAN_POINT('Ctrl Pts',(89.6270320490069,61.2713952392099,11.5245064615504));
#74801=CARTESIAN_POINT('Ctrl Pts',(89.647023344762,61.2667192986387,11.5841684378208));
#74802=CARTESIAN_POINT('Ctrl Pts',(89.6637387147587,61.2620433580676,11.645035879155));
#74803=CARTESIAN_POINT('Ctrl Pts',(89.6770399157617,61.2573674174965,11.7067148281815));
#74804=CARTESIAN_POINT('Ctrl Pts',(89.6900812274551,61.252782839124,11.7671886454702));
#74805=CARTESIAN_POINT('Ctrl Pts',(89.6998404752371,61.2481982607514,11.8284420224734));
#74806=CARTESIAN_POINT('Ctrl Pts',(89.7062373560354,61.2436136823788,11.8900876857573));
#74807=CARTESIAN_POINT('Ctrl Pts',(89.7126303271715,61.2390319060207,11.9516956722856));
#74808=CARTESIAN_POINT('Ctrl Pts',(89.7156649536999,61.2344501296626,12.0136949644102));
#74809=CARTESIAN_POINT('Ctrl Pts',(89.7153124500783,61.2298683533045,12.0756906195969));
#74810=CARTESIAN_POINT('Ctrl Pts',(89.7149600324274,61.2252876943789,12.1376711548923));
#74811=CARTESIAN_POINT('Ctrl Pts',(89.711222127403,61.2207070354533,12.1996475461998));
#74812=CARTESIAN_POINT('Ctrl Pts',(89.7041220539864,61.2161263765277,12.2612243476233));
#74813=CARTESIAN_POINT('Ctrl Pts',(89.6967654790156,61.2113802339423,12.3250257098842));
#74814=CARTESIAN_POINT('Ctrl Pts',(89.685799160019,61.206634091357,12.3883974729087));
#74815=CARTESIAN_POINT('Ctrl Pts',(89.671307499463,61.2018879487716,12.4509075769934));
#74816=CARTESIAN_POINT('Ctrl Pts',(89.657303402648,61.197301487475,12.5113145639037));
#74817=CARTESIAN_POINT('Ctrl Pts',(89.6400076451835,61.1927150261785,12.5709164680236));
#74818=CARTESIAN_POINT('Ctrl Pts',(89.6195474690945,61.1881285648819,12.6293381535717));
#74819=CARTESIAN_POINT('Ctrl Pts',(89.5980187871109,61.1833025816521,12.6908108351185));
#74820=CARTESIAN_POINT('Ctrl Pts',(89.5729863453518,61.1784765984224,12.7509760483229));
#74821=CARTESIAN_POINT('Ctrl Pts',(89.5446549040389,61.1736506151926,12.8094228076386));
#74822=CARTESIAN_POINT('Ctrl Pts',(89.5163234627261,61.1688246319628,12.8678695669544));
#74823=CARTESIAN_POINT('Ctrl Pts',(89.4846934050063,61.1639986487331,12.9245973441079));
#74824=CARTESIAN_POINT('Ctrl Pts',(89.4500224416137,61.1591726655033,12.9792301178411));
#74825=CARTESIAN_POINT('Ctrl Pts',(89.4169949395942,61.1545754419113,13.0312732071655));
#74826=CARTESIAN_POINT('Ctrl Pts',(89.3810727467405,61.1499782183192,13.0816291288742));
#74827=CARTESIAN_POINT('Ctrl Pts',(89.3424539700237,61.1453809947272,13.1299573117885));
#74828=CARTESIAN_POINT('Ctrl Pts',(89.3031739347497,61.1407050541561,13.1791130047178));
#74829=CARTESIAN_POINT('Ctrl Pts',(89.2611043046755,61.1360291135849,13.2261703658227));
#74830=CARTESIAN_POINT('Ctrl Pts',(89.2165010687694,61.1313531730138,13.2707995720434));
#74831=CARTESIAN_POINT('Ctrl Pts',(89.1727693259121,61.1267685946414,13.3145567777869));
#74832=CARTESIAN_POINT('Ctrl Pts',(89.1266024710288,61.122184016269,13.3559794843794));
#74833=CARTESIAN_POINT('Ctrl Pts',(89.0782823044433,61.1175994378967,13.3947901708781));
#74834=CARTESIAN_POINT('Ctrl Pts',(89.0299916703019,61.1130176615387,13.4335771369612));
#74835=CARTESIAN_POINT('Ctrl Pts',(88.9795507300838,61.1084358851808,13.4697549303118));
#74836=CARTESIAN_POINT('Ctrl Pts',(88.9272756701305,61.1038541088229,13.5030851512443));
#74837=CARTESIAN_POINT('Ctrl Pts',(88.8750133593484,61.0992734498975,13.5364072433924));
#74838=CARTESIAN_POINT('Ctrl Pts',(88.8209182458546,61.0946927909721,13.5668828682304));
#74839=CARTESIAN_POINT('Ctrl Pts',(88.7653352003049,61.0901121320467,13.5943171271634));
#74840=CARTESIAN_POINT('Ctrl Pts',(88.7077441279694,61.0853659894611,13.6227424927592));
#74841=CARTESIAN_POINT('Ctrl Pts',(88.6485560503527,61.0806198468755,13.6479022218827));
#74842=CARTESIAN_POINT('Ctrl Pts',(88.588179729752,61.07587370429,13.6696328741839));
#74843=CARTESIAN_POINT('Ctrl Pts',(88.5298347363895,61.0712872429936,13.6906324109504));
#74844=CARTESIAN_POINT('Ctrl Pts',(88.4703807174589,61.0667007816973,13.7084298780083));
#74845=CARTESIAN_POINT('Ctrl Pts',(88.4102018483891,61.0621143204009,13.7229287008929));
#74846=CARTESIAN_POINT('Ctrl Pts',(88.3468802167051,61.0572883371708,13.7381847058119));
#74847=CARTESIAN_POINT('Ctrl Pts',(88.2827565818875,61.0524623539406,13.7497879587534));
#74848=CARTESIAN_POINT('Ctrl Pts',(88.2182872832856,61.0476363707105,13.7576875650628));
#74849=CARTESIAN_POINT('Ctrl Pts',(88.1538179846837,61.0428103874803,13.7655871713722));
#74850=CARTESIAN_POINT('Ctrl Pts',(88.0890036739298,61.0379844042502,13.7697831664042));
#74851=CARTESIAN_POINT('Ctrl Pts',(88.024300036427,61.03315842102,13.7702881049374));
#74852=CARTESIAN_POINT('Ctrl Pts',(87.9626634590428,61.028561197428,13.7707691085436));
#74853=CARTESIAN_POINT('Ctrl Pts',(87.9008742301636,61.0239639738359,13.7679031034688));
#74854=CARTESIAN_POINT('Ctrl Pts',(87.8393259238227,61.0193667502438,13.7616717981876));
#74855=CARTESIAN_POINT('Ctrl Pts',(87.776723742976,61.0146908096727,13.7553337960016));
#74856=CARTESIAN_POINT('Ctrl Pts',(87.7143713423495,61.0100148691016,13.7455140635796));
#74857=CARTESIAN_POINT('Ctrl Pts',(87.6526846613781,61.0053389285305,13.7322487670538));
#74858=CARTESIAN_POINT('Ctrl Pts',(87.59220326322,61.0007543501581,13.7192426583083));
#74859=CARTESIAN_POINT('Ctrl Pts',(87.5323623254715,60.9961697717857,13.7029245309443));
#74860=CARTESIAN_POINT('Ctrl Pts',(87.4735478474987,60.9915851934133,13.6833806043637));
#74861=CARTESIAN_POINT('Ctrl Pts',(87.4147693159106,60.9870034170553,13.6638486226905));
#74862=CARTESIAN_POINT('Ctrl Pts',(87.3570164822173,60.9824216406974,13.6410949112955));
#74863=CARTESIAN_POINT('Ctrl Pts',(87.3006611301225,60.9778398643395,13.6152557973237));
#74864=CARTESIAN_POINT('Ctrl Pts',(87.2443195223264,60.973259205414,13.589422985158));
#74865=CARTESIAN_POINT('Ctrl Pts',(87.1893751820561,60.9686785464886,13.5605064762839));
#74866=CARTESIAN_POINT('Ctrl Pts',(87.1361789051645,60.9640978875632,13.5286902910838));
#74867=CARTESIAN_POINT('Ctrl Pts',(87.0810608273384,60.9593517449776,13.4957246950974));
#74868=CARTESIAN_POINT('Ctrl Pts',(87.0278200661602,60.9546056023921,13.4596461439811));
#74869=CARTESIAN_POINT('Ctrl Pts',(86.9768156434923,60.9498594598066,13.420709397751));
#74870=CARTESIAN_POINT('Ctrl Pts',(86.9275272358445,60.9452729985102,13.3830826563766));
#74871=CARTESIAN_POINT('Ctrl Pts',(86.8803274206532,60.9406865372138,13.3427874004942));
#74872=CARTESIAN_POINT('Ctrl Pts',(86.8355057084484,60.9361000759175,13.3000940021447));
#74873=CARTESIAN_POINT('Ctrl Pts',(86.7883432410324,60.9312740926873,13.2551709969874));
#74874=CARTESIAN_POINT('Ctrl Pts',(86.7438145223771,60.9264481094572,13.2075929638639));
#74875=CARTESIAN_POINT('Ctrl Pts',(86.702209828058,60.9216221262271,13.1577156779253));
#74876=CARTESIAN_POINT('Ctrl Pts',(86.6606051337388,60.916796142997,13.1078383919867));
#74877=CARTESIAN_POINT('Ctrl Pts',(86.6219247874981,60.9119701597669,13.0556624198593));
#74878=CARTESIAN_POINT('Ctrl Pts',(86.5864054049996,60.9071441765368,13.0015774021938));
#74879=CARTESIAN_POINT('Ctrl Pts',(86.5519012991686,60.9024561379394,12.949038336418));
#74880=CARTESIAN_POINT('Ctrl Pts',(86.5202420108511,60.8977680993419,12.8944887870569));
#74881=CARTESIAN_POINT('Ctrl Pts',(86.4916626353851,60.8930800607445,12.8382621368972));
#74882=CARTESIAN_POINT('Ctrl Pts',(86.4631330034052,60.8884001818559,12.7821333513531));
#74883=CARTESIAN_POINT('Ctrl Pts',(86.4376728583687,60.8837203029673,12.7243336868688));
#74884=CARTESIAN_POINT('Ctrl Pts',(86.4154735085036,60.8790404240787,12.6652245409971));
#74885=CARTESIAN_POINT('Ctrl Pts',(86.3933119945547,60.8743685214374,12.6062161390075));
#74886=CARTESIAN_POINT('Ctrl Pts',(86.374400394826,60.8696966187961,12.5459031421756));
#74887=CARTESIAN_POINT('Ctrl Pts',(86.3588827577064,60.8650247161548,12.4846686677029));
#74888=CARTESIAN_POINT('Ctrl Pts',(86.3433806101681,60.8603574769695,12.4234953169933));
#74889=CARTESIAN_POINT('Ctrl Pts',(86.3312658171752,60.8556902377841,12.3614027807631));
#74890=CARTESIAN_POINT('Ctrl Pts',(86.3226328405803,60.8510229985987,12.298789970989));
#74891=CARTESIAN_POINT('Ctrl Pts',(86.3140063629978,60.8463592729692,12.2362242969188));
#74892=CARTESIAN_POINT('Ctrl Pts',(86.3088565581616,60.8416955473396,12.1731396048206));
#74893=CARTESIAN_POINT('Ctrl Pts',(86.3072266081747,60.8370318217101,12.1099438836244));
#74894=CARTESIAN_POINT('Ctrl Pts',(86.3068425435101,60.8359329093301,12.0950530933207));
#74895=CARTESIAN_POINT('Ctrl Pts',(86.306653679578,60.8348339969502,12.0801561643758));
#74896=CARTESIAN_POINT('Ctrl Pts',(86.3066601613135,60.8337350845702,12.0652584704679));
#74897=CARTESIAN_POINT('',(86.3066603586072,60.0399850846269,12.0648943883226));
#74898=CARTESIAN_POINT('Ctrl Pts',(86.3066601613138,60.8337350845235,12.065258469835));
#74899=CARTESIAN_POINT('Ctrl Pts',(86.3066897126874,60.8287249537047,11.9973373173053));
#74900=CARTESIAN_POINT('Ctrl Pts',(86.3107836349031,60.8237148228858,11.9295475736294));
#74901=CARTESIAN_POINT('Ctrl Pts',(86.3188700121392,60.818704692067,11.8623558501151));
#74902=CARTESIAN_POINT('Ctrl Pts',(86.3269823930434,60.8136784499816,11.7949480556427));
#74903=CARTESIAN_POINT('Ctrl Pts',(86.3391128067182,60.8086522078963,11.7281424584012));
#74904=CARTESIAN_POINT('Ctrl Pts',(86.3551385560175,60.8036259658109,11.6623941106326));
#74905=CARTESIAN_POINT('Ctrl Pts',(86.3712365037121,60.7985770797539,11.5963495567324));
#74906=CARTESIAN_POINT('Ctrl Pts',(86.3912648081972,60.7935281936968,11.5313721138635));
#74907=CARTESIAN_POINT('Ctrl Pts',(86.4150508733927,60.7884793076398,11.4679019972601));
#74908=CARTESIAN_POINT('Ctrl Pts',(86.426592213064,60.7860295157778,11.4371053871997));
#74909=CARTESIAN_POINT('Ctrl Pts',(86.4390175462652,60.7835797239157,11.4066633072305));
#74910=CARTESIAN_POINT('Ctrl Pts',(86.4523032711897,60.7811299320537,11.3766239464587));
#74911=CARTESIAN_POINT('Ctrl Pts',(86.4772349598801,60.7765327084616,11.3202527664535));
#74912=CARTESIAN_POINT('Ctrl Pts',(86.5052798154291,60.7719354848695,11.2651201185229));
#74913=CARTESIAN_POINT('Ctrl Pts',(86.5362925101349,60.7673382612775,11.2115922197594));
#74914=CARTESIAN_POINT('Ctrl Pts',(86.5678362265738,60.7626623207063,11.157147777695));
#74915=CARTESIAN_POINT('Ctrl Pts',(86.6024502461152,60.7579863801352,11.1043640807809));
#74916=CARTESIAN_POINT('Ctrl Pts',(86.6399304046922,60.7533104395641,11.0536053139104));
#74917=CARTESIAN_POINT('Ctrl Pts',(86.6766782464991,60.7487258611917,11.0038383116859));
#74918=CARTESIAN_POINT('Ctrl Pts',(86.7161809160319,60.7441412828193,10.956018250926));
#74919=CARTESIAN_POINT('Ctrl Pts',(86.7582009561544,60.7395567044469,10.9104614280174));
#74920=CARTESIAN_POINT('Ctrl Pts',(86.8001953143602,60.7349749280889,10.8649324486456));
#74921=CARTESIAN_POINT('Ctrl Pts',(86.8447036479709,60.730393151731,10.8216643377432));
#74922=CARTESIAN_POINT('Ctrl Pts',(86.8914486848574,60.725811375373,10.7809398113853));
#74923=CARTESIAN_POINT('Ctrl Pts',(86.9381823212695,60.7212307164476,10.7402252171818));
#74924=CARTESIAN_POINT('Ctrl Pts',(86.9871511944086,60.7166500575221,10.7020533102775));
#74925=CARTESIAN_POINT('Ctrl Pts',(87.0380432051213,60.7120693985967,10.6666680483533));
#74926=CARTESIAN_POINT('Ctrl Pts',(87.0907737714519,60.7073232560111,10.6300044370145));
#74927=CARTESIAN_POINT('Ctrl Pts',(87.1455686478471,60.7025771134256,10.5963330541753));
#74928=CARTESIAN_POINT('Ctrl Pts',(87.2020478798997,60.6978309708401,10.565876237444));
#74929=CARTESIAN_POINT('Ctrl Pts',(87.2566269000601,60.6932445095437,10.5364441231253));
#74930=CARTESIAN_POINT('Ctrl Pts',(87.3127782216355,60.6886580482473,10.5100138509726));
#74931=CARTESIAN_POINT('Ctrl Pts',(87.370136273385,60.6840715869509,10.4867379826295));
#74932=CARTESIAN_POINT('Ctrl Pts',(87.4304897742575,60.6792456037208,10.4622465625498));
#74933=CARTESIAN_POINT('Ctrl Pts',(87.4921788951917,60.6744196204907,10.4412482678737));
#74934=CARTESIAN_POINT('Ctrl Pts',(87.554759916953,60.6695936372607,10.423861204946));
#74935=CARTESIAN_POINT('Ctrl Pts',(87.6173409387144,60.6647676540306,10.4064741420184));
#74936=CARTESIAN_POINT('Ctrl Pts',(87.680813211647,60.6599416708005,10.3926983726578));
#74937=CARTESIAN_POINT('Ctrl Pts',(87.744724239612,60.6551156875704,10.3825891603563));
#74938=CARTESIAN_POINT('Ctrl Pts',(87.805605778471,60.6505184639783,10.3729591415448));
#74939=CARTESIAN_POINT('Ctrl Pts',(87.8671353781665,60.6459212403862,10.3666163383851));
#74940=CARTESIAN_POINT('Ctrl Pts',(87.9289265464004,60.6413240167941,10.3636372936961));
#74941=CARTESIAN_POINT('Ctrl Pts',(87.9917757475964,60.636648076223,10.3606072396547));
#74942=CARTESIAN_POINT('Ctrl Pts',(88.0548950502372,60.6319721356519,10.3610573983662));
#74943=CARTESIAN_POINT('Ctrl Pts',(88.1178677565465,60.6272961950808,10.3650137807111));
#74944=CARTESIAN_POINT('Ctrl Pts',(88.1796100526699,60.6227116167083,10.368892860151));
#74945=CARTESIAN_POINT('Ctrl Pts',(88.2412108972013,60.6181270383359,10.3761423473277));
#74946=CARTESIAN_POINT('Ctrl Pts',(88.302275766393,60.6135424599635,10.386734308243));
#74947=CARTESIAN_POINT('Ctrl Pts',(88.3633033138001,60.6089606836056,10.3973197955362));
#74948=CARTESIAN_POINT('Ctrl Pts',(88.4237950348914,60.6043789072476,10.4112436190516));
#74949=CARTESIAN_POINT('Ctrl Pts',(88.4833630218469,60.5997971308896,10.4284261814527));
#74950=CARTESIAN_POINT('Ctrl Pts',(88.5429164809861,60.5952164719642,10.4456045532621));
#74951=CARTESIAN_POINT('Ctrl Pts',(88.60154616433,60.5906358130387,10.466039945214));
#74952=CARTESIAN_POINT('Ctrl Pts',(88.6588778356715,60.5860551541133,10.4896024785462));
#74953=CARTESIAN_POINT('Ctrl Pts',(88.7182807057128,60.5813090115278,10.5140162462357));
#74954=CARTESIAN_POINT('Ctrl Pts',(88.7762894204689,60.5765628689422,10.5417872655508));
#74955=CARTESIAN_POINT('Ctrl Pts',(88.8325111026076,60.5718167263567,10.5727169243936));
#74956=CARTESIAN_POINT('Ctrl Pts',(88.8868412379758,60.5672302650603,10.6026059723178));
#74957=CARTESIAN_POINT('Ctrl Pts',(88.9395022765314,60.5626438037639,10.6354441394256));
#74958=CARTESIAN_POINT('Ctrl Pts',(88.9901677626185,60.5580573424675,10.6710070508248));
#74959=CARTESIAN_POINT('Ctrl Pts',(89.0434791873529,60.5532313592375,10.70842718869));
#74960=CARTESIAN_POINT('Ctrl Pts',(89.0945804021524,60.5484053760074,10.7488640761435));
#74961=CARTESIAN_POINT('Ctrl Pts',(89.1431315106124,60.5435793927773,10.7920089959978));
#74962=CARTESIAN_POINT('Ctrl Pts',(89.1916826190724,60.5387534095473,10.835153915852));
#74963=CARTESIAN_POINT('Ctrl Pts',(89.2376832168851,60.5339274263172,10.8810063558477));
#74964=CARTESIAN_POINT('Ctrl Pts',(89.280841442675,60.5291014430871,10.9292161392485));
#74965=CARTESIAN_POINT('Ctrl Pts',(89.3219538967252,60.5245042194951,10.9751406986705));
#74966=CARTESIAN_POINT('Ctrl Pts',(89.3606561987092,60.519906995903,11.0233926894249));
#74967=CARTESIAN_POINT('Ctrl Pts',(89.3966744104397,60.5153097723109,11.0736889278797));
#74968=CARTESIAN_POINT('Ctrl Pts',(89.433309351977,60.5106338317398,11.1248463748159));
#74969=CARTESIAN_POINT('Ctrl Pts',(89.4671669957909,60.5059578911687,11.1781184027865));
#74970=CARTESIAN_POINT('Ctrl Pts',(89.4979994732315,60.5012819505975,11.2331690434372));
#74971=CARTESIAN_POINT('Ctrl Pts',(89.5282295215163,60.4966973722251,11.2871440614417));
#74972=CARTESIAN_POINT('Ctrl Pts',(89.5555512957382,60.4921127938527,11.3428283479567));
#74973=CARTESIAN_POINT('Ctrl Pts',(89.5797742746477,60.4875282154803,11.399875303863));
#74974=CARTESIAN_POINT('Ctrl Pts',(89.6039824488944,60.4829464391223,11.4568873936634));
#74975=CARTESIAN_POINT('Ctrl Pts',(89.6250953846744,60.4783646627644,11.5152600338695));
#74976=CARTESIAN_POINT('Ctrl Pts',(89.6429695526732,60.4737828864064,11.5746241614126));
#74977=CARTESIAN_POINT('Ctrl Pts',(89.6608393614073,60.469202227481,11.6339738108579));
#74978=CARTESIAN_POINT('Ctrl Pts',(89.6754718237169,60.4646215685555,11.6943139803969));
#74979=CARTESIAN_POINT('Ctrl Pts',(89.6867730682438,60.4600409096301,11.7552598201892));
#74980=CARTESIAN_POINT('Ctrl Pts',(89.6984825883786,60.4552947670445,11.8184074263208));
#74981=CARTESIAN_POINT('Ctrl Pts',(89.7066154222443,60.450548624459,11.8822047422107));
#74982=CARTESIAN_POINT('Ctrl Pts',(89.7111253318904,60.4458024818735,11.9462139763385));
#74983=CARTESIAN_POINT('Ctrl Pts',(89.7154835081713,60.4412160205771,12.0080696559035));
#74984=CARTESIAN_POINT('Ctrl Pts',(89.7164587509438,60.4366295592807,12.0701226904972));
#74985=CARTESIAN_POINT('Ctrl Pts',(89.7140624931613,60.4320430979843,12.1319771171478));
#74986=CARTESIAN_POINT('Ctrl Pts',(89.7115410939549,60.4272171147543,12.1970618102108));
#74987=CARTESIAN_POINT('Ctrl Pts',(89.7052864444172,60.4223911315242,12.2619259403604));
#74988=CARTESIAN_POINT('Ctrl Pts',(89.6953735450039,60.4175651482941,12.3261165056106));
#74989=CARTESIAN_POINT('Ctrl Pts',(89.6854606455906,60.4127391650641,12.3903070708608));
#74990=CARTESIAN_POINT('Ctrl Pts',(89.6718897073655,60.407913181834,12.4538234536952));
#74991=CARTESIAN_POINT('Ctrl Pts',(89.6547966159694,60.4030871986039,12.5162305197647));
#74992=CARTESIAN_POINT('Ctrl Pts',(89.638513765557,60.3984899750119,12.5756793870255));
#74993=CARTESIAN_POINT('Ctrl Pts',(89.6189683273089,60.3938927514198,12.634365830386));
#74994=CARTESIAN_POINT('Ctrl Pts',(89.5962496260556,60.3892955278277,12.6919061101239));
#74995=CARTESIAN_POINT('Ctrl Pts',(89.5731419188089,60.3846195872566,12.7504316360445));
#74996=CARTESIAN_POINT('Ctrl Pts',(89.5467513044177,60.3799436466855,12.8077708414871));
#74997=CARTESIAN_POINT('Ctrl Pts',(89.5172255933602,60.3752677061143,12.8635332579315));
#74998=CARTESIAN_POINT('Ctrl Pts',(89.4882767788307,60.3706831277419,12.9182061444953));
#74999=CARTESIAN_POINT('Ctrl Pts',(89.4563145273844,60.3660985493695,12.9713628335739));
#75000=CARTESIAN_POINT('Ctrl Pts',(89.4215266857891,60.3615139709971,13.0226552692985));
#75001=CARTESIAN_POINT('Ctrl Pts',(89.3867601059168,60.3569321946391,13.0739163559798));
#75002=CARTESIAN_POINT('Ctrl Pts',(89.3491716453288,60.3523504182812,13.1233150281532));
#75003=CARTESIAN_POINT('Ctrl Pts',(89.3089935115999,60.3477686419232,13.1705305244512));
#75004=CARTESIAN_POINT('Ctrl Pts',(89.2688251767677,60.3431879829978,13.2177345055362));
#75005=CARTESIAN_POINT('Ctrl Pts',(89.2260687523383,60.3386073240723,13.262755980226));
#75006=CARTESIAN_POINT('Ctrl Pts',(89.1809966431017,60.3340266651469,13.3053073431279));
#75007=CARTESIAN_POINT('Ctrl Pts',(89.1342962315347,60.3292805225614,13.3493959423505));
#75008=CARTESIAN_POINT('Ctrl Pts',(89.0851099948366,60.3245343799758,13.3908320934861));
#75009=CARTESIAN_POINT('Ctrl Pts',(89.0337806515249,60.3197882373903,13.4293394934741));
#75010=CARTESIAN_POINT('Ctrl Pts',(88.9841782550046,60.3152017760939,13.4665513337187));
#75011=CARTESIAN_POINT('Ctrl Pts',(88.9325751573961,60.3106153147975,13.5010281450264));
#75012=CARTESIAN_POINT('Ctrl Pts',(88.8793102167946,60.3060288535011,13.5325647626375));
#75013=CARTESIAN_POINT('Ctrl Pts',(88.8232635844387,60.3012028702711,13.5657483387955));
#75014=CARTESIAN_POINT('Ctrl Pts',(88.765377341294,60.296376887041,13.5956758992624));
#75015=CARTESIAN_POINT('Ctrl Pts',(88.7060727440737,60.2915509038109,13.622164745792));
#75016=CARTESIAN_POINT('Ctrl Pts',(88.6467681468534,60.2867249205809,13.6486535923216));
#75017=CARTESIAN_POINT('Ctrl Pts',(88.586045828827,60.2818989373508,13.671703567293));
#75018=CARTESIAN_POINT('Ctrl Pts',(88.5243450597767,60.2770729541207,13.691192814777));
#75019=CARTESIAN_POINT('Ctrl Pts',(88.4655690098809,60.2724757305286,13.7097582394902));
#75020=CARTESIAN_POINT('Ctrl Pts',(88.4056638648384,60.2678785069365,13.7251691573103));
#75021=CARTESIAN_POINT('Ctrl Pts',(88.3450004621917,60.2632812833445,13.7372924719677));
#75022=CARTESIAN_POINT('Ctrl Pts',(88.2832983369987,60.2586053427733,13.749623370765));
#75023=CARTESIAN_POINT('Ctrl Pts',(88.2208122199804,60.2539294022022,13.7585527710084));
#75024=CARTESIAN_POINT('Ctrl Pts',(88.1579503242277,60.2492534616311,13.7639930617672));
#75025=CARTESIAN_POINT('Ctrl Pts',(88.0963166735571,60.2446688832587,13.7693270558531));
#75026=CARTESIAN_POINT('Ctrl Pts',(88.034322328037,60.2400843048863,13.7713070141474));
#75027=CARTESIAN_POINT('Ctrl Pts',(87.9723615846257,60.2354997265138,13.769901965624));
#75028=CARTESIAN_POINT('Ctrl Pts',(87.9104387105417,60.2309179501559,13.7684977758418));
#75029=CARTESIAN_POINT('Ctrl Pts',(87.8485499057051,60.2263361737979,13.7637126930032));
#75030=CARTESIAN_POINT('Ctrl Pts',(87.787090597633,60.2217543974399,13.7555678190388));
#75031=CARTESIAN_POINT('Ctrl Pts',(87.7256462786444,60.2171737385145,13.7474249314977));
#75032=CARTESIAN_POINT('Ctrl Pts',(87.664631752888,60.212593079589,13.7359239463246));
#75033=CARTESIAN_POINT('Ctrl Pts',(87.6044363957642,60.2080124206636,13.7211377197414));
#75034=CARTESIAN_POINT('Ctrl Pts',(87.5420663846926,60.2032662780781,13.7058173169767));
#75035=CARTESIAN_POINT('Ctrl Pts',(87.4805764429374,60.1985201354926,13.6869698353306));
#75036=CARTESIAN_POINT('Ctrl Pts',(87.4203845886494,60.193773992907,13.6647333334472));
#75037=CARTESIAN_POINT('Ctrl Pts',(87.3622178553335,60.1891875316106,13.6432449661219));
#75038=CARTESIAN_POINT('Ctrl Pts',(87.305263699935,60.1846010703142,13.6185922911435));
#75039=CARTESIAN_POINT('Ctrl Pts',(87.2498782819239,60.1800146090178,13.5909487092597));
#75040=CARTESIAN_POINT('Ctrl Pts',(87.1916004330032,60.1751886257878,13.5618614775207));
#75041=CARTESIAN_POINT('Ctrl Pts',(87.135060229181,60.1703626425577,13.5294626909284));
#75042=CARTESIAN_POINT('Ctrl Pts',(87.0806396482421,60.1655366593276,13.4940071608633));
#75043=CARTESIAN_POINT('Ctrl Pts',(87.0262190673033,60.1607106760976,13.4585516307983));
#75044=CARTESIAN_POINT('Ctrl Pts',(86.9739185851529,60.1558846928675,13.42003980379));
#75045=CARTESIAN_POINT('Ctrl Pts',(86.9240788349235,60.1510587096374,13.3787746251771));
#75046=CARTESIAN_POINT('Ctrl Pts',(86.8762830329794,60.1464306419287,13.3392017482045));
#75047=CARTESIAN_POINT('Ctrl Pts',(86.8305379272261,60.1418025742199,13.2969210980014));
#75048=CARTESIAN_POINT('Ctrl Pts',(86.787171265087,60.1371745065111,13.2521779222365));
#75049=CARTESIAN_POINT('Ctrl Pts',(86.7447554783474,60.1326479157322,13.2084158038791));
#75050=CARTESIAN_POINT('Ctrl Pts',(86.7046152985981,60.1281213249533,13.162298431376));
#75051=CARTESIAN_POINT('Ctrl Pts',(86.6670253249706,60.1235947341743,13.1140968030099));
#75052=CARTESIAN_POINT('Ctrl Pts',(86.6294715645995,60.1190725042017,13.0659416109076));
#75053=CARTESIAN_POINT('Ctrl Pts',(86.5944634655044,60.114550274229,13.015706550762));
#75054=CARTESIAN_POINT('Ctrl Pts',(86.5622372035043,60.1100280442564,12.9636977192184));
#75055=CARTESIAN_POINT('Ctrl Pts',(86.5300293850305,60.1055084024172,12.9117186530337));
#75056=CARTESIAN_POINT('Ctrl Pts',(86.5006005239128,60.100988760578,12.8579682721358));
#75057=CARTESIAN_POINT('Ctrl Pts',(86.4741437523452,60.0964691187388,12.80278199601));
#75058=CARTESIAN_POINT('Ctrl Pts',(86.4465902196966,60.0917621158962,12.7453079819525));
#75059=CARTESIAN_POINT('Ctrl Pts',(86.4222609259181,60.0870551130535,12.6862769207695));
#75060=CARTESIAN_POINT('Ctrl Pts',(86.40132014105,60.0823481102108,12.6260942664325));
#75061=CARTESIAN_POINT('Ctrl Pts',(86.3812012386156,60.0778258474807,12.5682736566287));
#75062=CARTESIAN_POINT('Ctrl Pts',(86.3642098974303,60.0733035847505,12.5093907181173));
#75063=CARTESIAN_POINT('Ctrl Pts',(86.3504409737101,60.0687813220203,12.4498209944845));
#75064=CARTESIAN_POINT('Ctrl Pts',(86.3366653153358,60.0642568473616,12.3902221341168));
#75065=CARTESIAN_POINT('Ctrl Pts',(86.3261152994707,60.059732372703,12.3299363366975));
#75066=CARTESIAN_POINT('Ctrl Pts',(86.318834348335,60.0552078980443,12.2693475913923));
#75067=CARTESIAN_POINT('Ctrl Pts',(86.3115430861579,60.0506770159747,12.2086730423168));
#75068=CARTESIAN_POINT('Ctrl Pts',(86.3075301486019,60.0461461339052,12.1476952119335));
#75069=CARTESIAN_POINT('Ctrl Pts',(86.3067869250066,60.0416152518357,12.086799774553));
#75070=CARTESIAN_POINT('Ctrl Pts',(86.306697790138,60.0410718627661,12.0794965796007));
#75071=CARTESIAN_POINT('Ctrl Pts',(86.306655622955,60.0405284736965,12.0721945642732));
#75072=CARTESIAN_POINT('Ctrl Pts',(86.3066603586072,60.0399850846269,12.0648943883225));
#75073=CARTESIAN_POINT('',(86.3066606119916,59.2462350845034,12.0674443279418));
#75074=CARTESIAN_POINT('Ctrl Pts',(86.3066603586077,60.0399850845702,12.0648943875605));
#75075=CARTESIAN_POINT('Ctrl Pts',(86.3067037612879,60.0350048780982,11.9979876616978));
#75076=CARTESIAN_POINT('Ctrl Pts',(86.3106868359654,60.0300246716262,11.9312088054057));
#75077=CARTESIAN_POINT('Ctrl Pts',(86.3185655492583,60.0250444651542,11.8649018509712));
#75078=CARTESIAN_POINT('Ctrl Pts',(86.3258383815855,60.0204472415621,11.8036939679327));
#75079=CARTESIAN_POINT('Ctrl Pts',(86.3364508532806,60.01585001797,11.7427554888319));
#75080=CARTESIAN_POINT('Ctrl Pts',(86.3503716237528,60.011252794378,11.6824791640566));
#75081=CARTESIAN_POINT('Ctrl Pts',(86.3645307557003,60.0065768538068,11.6211707445617));
#75082=CARTESIAN_POINT('Ctrl Pts',(86.3821125786744,60.0019009132357,11.5605479063764));
#75083=CARTESIAN_POINT('Ctrl Pts',(86.40302891446,59.9972249726646,11.5010187404283));
#75084=CARTESIAN_POINT('Ctrl Pts',(86.4235365704521,59.9926403942921,11.4426527020705));
#75085=CARTESIAN_POINT('Ctrl Pts',(86.4472494296751,59.9880558159197,11.3853384855202));
#75086=CARTESIAN_POINT('Ctrl Pts',(86.4740334224729,59.9834712375473,11.3294481856891));
#75087=CARTESIAN_POINT('Ctrl Pts',(86.5008010453608,59.9788894611894,11.2735920450358));
#75088=CARTESIAN_POINT('Ctrl Pts',(86.5306358604229,59.9743076848315,11.21915855358));
#75089=CARTESIAN_POINT('Ctrl Pts',(86.563355875376,59.9697259084735,11.1664994029787));
#75090=CARTESIAN_POINT('Ctrl Pts',(86.5960679103656,59.9651452495481,11.1138530952231));
#75091=CARTESIAN_POINT('Ctrl Pts',(86.6316634798331,59.9605645906227,11.062980701457));
#75092=CARTESIAN_POINT('Ctrl Pts',(86.6699159157286,59.9559839316972,11.0142070952351));
#75093=CARTESIAN_POINT('Ctrl Pts',(86.709550282303,59.9512377891117,10.9636714641595));
#75094=CARTESIAN_POINT('Ctrl Pts',(86.7520368494761,59.9464916465262,10.9153896651943));
#75095=CARTESIAN_POINT('Ctrl Pts',(86.7970777366679,59.9417455039407,10.8696858380063));
#75096=CARTESIAN_POINT('Ctrl Pts',(86.8406032486259,59.9371590426443,10.8255196902942));
#75097=CARTESIAN_POINT('Ctrl Pts',(86.8865134825776,59.9325725813479,10.7837610909495));
#75098=CARTESIAN_POINT('Ctrl Pts',(86.9345038099913,59.9279861200516,10.7446632569641));
#75099=CARTESIAN_POINT('Ctrl Pts',(86.9850003693947,59.9231601368215,10.7035235898105));
#75100=CARTESIAN_POINT('Ctrl Pts',(87.0377997247886,59.9183341535914,10.6653306049712));
#75101=CARTESIAN_POINT('Ctrl Pts',(87.092512426132,59.9135081703613,10.630327540053));
#75102=CARTESIAN_POINT('Ctrl Pts',(87.1472251274755,59.9086821871312,10.5953244751349));
#75103=CARTESIAN_POINT('Ctrl Pts',(87.2038505719327,59.9038562039012,10.5635115800648));
#75104=CARTESIAN_POINT('Ctrl Pts',(87.2619724597879,59.8990302206711,10.5350746002487));
#75105=CARTESIAN_POINT('Ctrl Pts',(87.3173392734142,59.894432997079,10.5079855806095));
#75106=CARTESIAN_POINT('Ctrl Pts',(87.374291171351,59.8898357734869,10.4838483870692));
#75107=CARTESIAN_POINT('Ctrl Pts',(87.4324811965851,59.8852385498949,10.4628497170585));
#75108=CARTESIAN_POINT('Ctrl Pts',(87.4916675934129,59.8805626093237,10.4414914926702));
#75109=CARTESIAN_POINT('Ctrl Pts',(87.5521344822472,59.8758866687526,10.4233806019292));
#75110=CARTESIAN_POINT('Ctrl Pts',(87.6134911895053,59.8712107281815,10.4086643124644));
#75111=CARTESIAN_POINT('Ctrl Pts',(87.673649061236,59.8666261498091,10.3942355614193));
#75112=CARTESIAN_POINT('Ctrl Pts',(87.7346617734659,59.8620415714367,10.3830700763129));
#75113=CARTESIAN_POINT('Ctrl Pts',(87.7961440021667,59.8574569930643,10.3752570462087));
#75114=CARTESIAN_POINT('Ctrl Pts',(87.8575886540001,59.8528752167063,10.3674487912923));
#75115=CARTESIAN_POINT('Ctrl Pts',(87.9195017493652,59.8482934403483,10.3629889926218));
#75116=CARTESIAN_POINT('Ctrl Pts',(87.9814891122661,59.8437116639904,10.3619155117468));
#75117=CARTESIAN_POINT('Ctrl Pts',(88.0434613572981,59.8391310050649,10.3608422926791));
#75118=CARTESIAN_POINT('Ctrl Pts',(88.1055073251662,59.8345503461395,10.3631537607271));
#75119=CARTESIAN_POINT('Ctrl Pts',(88.1672311382493,59.829969687214,10.3688356982775));
#75120=CARTESIAN_POINT('Ctrl Pts',(88.2311848232063,59.8252235446285,10.3747229049468));
#75121=CARTESIAN_POINT('Ctrl Pts',(88.2947920461684,59.820477402043,10.3842287814717));
#75122=CARTESIAN_POINT('Ctrl Pts',(88.3576189204811,59.8157312594575,10.3972788850247));
#75123=CARTESIAN_POINT('Ctrl Pts',(88.4183320200597,59.8111447981611,10.4098899252076));
#75124=CARTESIAN_POINT('Ctrl Pts',(88.4783159575446,59.8065583368647,10.4258102720808));
#75125=CARTESIAN_POINT('Ctrl Pts',(88.537192769841,59.8019718755683,10.4449213453484));
#75126=CARTESIAN_POINT('Ctrl Pts',(88.5991443465405,59.7971458923382,10.465030469385));
#75127=CARTESIAN_POINT('Ctrl Pts',(88.6598693867404,59.7923199091081,10.4886724979279));
#75128=CARTESIAN_POINT('Ctrl Pts',(88.7189523041574,59.787493925878,10.5156521775298));
#75129=CARTESIAN_POINT('Ctrl Pts',(88.7780352215745,59.782667942648,10.5426318571317));
#75130=CARTESIAN_POINT('Ctrl Pts',(88.8354754792623,59.7778419594179,10.5729488168974));
#75131=CARTESIAN_POINT('Ctrl Pts',(88.8908912281221,59.7730159761878,10.6063540627009));
#75132=CARTESIAN_POINT('Ctrl Pts',(88.943680178246,59.7684187525957,10.63817584425));
#75133=CARTESIAN_POINT('Ctrl Pts',(88.9948489845408,59.7638215290036,10.6729303555109));
#75134=CARTESIAN_POINT('Ctrl Pts',(89.0440526094874,59.7592243054116,10.7104273750067));
#75135=CARTESIAN_POINT('Ctrl Pts',(89.0940987343988,59.7545483648404,10.7485664455229));
#75136=CARTESIAN_POINT('Ctrl Pts',(89.1421112428444,59.7498724242693,10.7895426342364));
#75137=CARTESIAN_POINT('Ctrl Pts',(89.1877545113035,59.7451964836982,10.8331076057794));
#75138=CARTESIAN_POINT('Ctrl Pts',(89.2325059657415,59.7406119053258,10.8758213706986));
#75139=CARTESIAN_POINT('Ctrl Pts',(89.2749795458075,59.7360273269534,10.9210232966276));
#75140=CARTESIAN_POINT('Ctrl Pts',(89.3148913226047,59.731442748581,10.9684380407302));
#75141=CARTESIAN_POINT('Ctrl Pts',(89.354778706019,59.726860972223,11.0158238057671));
#75142=CARTESIAN_POINT('Ctrl Pts',(89.3921070636436,59.722279195865,11.0654193186582));
#75143=CARTESIAN_POINT('Ctrl Pts',(89.4266307866161,59.7176974195071,11.1169139598621));
#75144=CARTESIAN_POINT('Ctrl Pts',(89.4611460897254,59.7131167605816,11.1683960422282));
#75145=CARTESIAN_POINT('Ctrl Pts',(89.4928578327069,59.7085361016562,11.2217759108146));
#75146=CARTESIAN_POINT('Ctrl Pts',(89.5215632365467,59.7039554427307,11.2767132688348));
#75147=CARTESIAN_POINT('Ctrl Pts',(89.5513056692001,59.6992093001452,11.3336353271409));
#75148=CARTESIAN_POINT('Ctrl Pts',(89.5778200601397,59.6944631575597,11.3922290774437));
#75149=CARTESIAN_POINT('Ctrl Pts',(89.6009336107763,59.6897170149742,11.4520896246815));
#75150=CARTESIAN_POINT('Ctrl Pts',(89.6232695190444,59.6851305536778,11.5099361975859));
#75151=CARTESIAN_POINT('Ctrl Pts',(89.6424297120832,59.6805440923814,11.5689651498336));
#75152=CARTESIAN_POINT('Ctrl Pts',(89.6583088049945,59.675957631085,11.6287946288214));
#75153=CARTESIAN_POINT('Ctrl Pts',(89.6750171627342,59.671131647855,11.6917486239822));
#75154=CARTESIAN_POINT('Ctrl Pts',(89.688092180723,59.6663056646249,11.7555884228971));
#75155=CARTESIAN_POINT('Ctrl Pts',(89.6974724820299,59.6614796813948,11.8198589775027));
#75156=CARTESIAN_POINT('Ctrl Pts',(89.7068527833367,59.6566536981648,11.8841295321083));
#75157=CARTESIAN_POINT('Ctrl Pts',(89.7125383883193,59.6518277149347,11.9488301901317));
#75158=CARTESIAN_POINT('Ctrl Pts',(89.7145313677356,59.6470017317046,12.0135050979548));
#75159=CARTESIAN_POINT('Ctrl Pts',(89.7164298766103,59.6424045081125,12.0751143074951));
#75160=CARTESIAN_POINT('Ctrl Pts',(89.7149857731566,59.6378072845205,12.1369531088728));
#75161=CARTESIAN_POINT('Ctrl Pts',(89.7101717185409,59.6332100609284,12.1986284528696));
#75162=CARTESIAN_POINT('Ctrl Pts',(89.705275234209,59.6285341203573,12.2613598466025));
#75163=CARTESIAN_POINT('Ctrl Pts',(89.6968921957595,59.6238581797861,12.3239216054898));
#75164=CARTESIAN_POINT('Ctrl Pts',(89.6850491932099,59.619182239215,12.38589706831));
#75165=CARTESIAN_POINT('Ctrl Pts',(89.6734375885439,59.6145976608426,12.4466616058708));
#75166=CARTESIAN_POINT('Ctrl Pts',(89.6585001108952,59.6100130824702,12.5068620284009));
#75167=CARTESIAN_POINT('Ctrl Pts',(89.6403140789271,59.6054285040978,12.5661104556095));
#75168=CARTESIAN_POINT('Ctrl Pts',(89.622139161945,59.6008467277398,12.6253226712111));
#75169=CARTESIAN_POINT('Ctrl Pts',(89.6007197765852,59.5962649513818,12.6835835595728));
#75170=CARTESIAN_POINT('Ctrl Pts',(89.5761836629574,59.5916831750239,12.7405182998342));
#75171=CARTESIAN_POINT('Ctrl Pts',(89.5516535333517,59.5871025160984,12.7974391544923));
#75172=CARTESIAN_POINT('Ctrl Pts',(89.524008385819,59.582521857173,12.8530340358315));
#75173=CARTESIAN_POINT('Ctrl Pts',(89.4934241238076,59.5779411982475,12.9069480083532));
#75174=CARTESIAN_POINT('Ctrl Pts',(89.4617349562139,59.573195055662,12.9628097097161));
#75175=CARTESIAN_POINT('Ctrl Pts',(89.4268904789498,59.5684489130765,13.0168661885659));
#75176=CARTESIAN_POINT('Ctrl Pts',(89.3891371271877,59.563702770491,13.0687526585689));
#75177=CARTESIAN_POINT('Ctrl Pts',(89.3526539656419,59.5591163091946,13.1188934375673));
#75178=CARTESIAN_POINT('Ctrl Pts',(89.3134549581655,59.5545298478982,13.167007552062));
#75179=CARTESIAN_POINT('Ctrl Pts',(89.2718037465764,59.5499433866018,13.2127993495895));
#75180=CARTESIAN_POINT('Ctrl Pts',(89.2279773550185,59.5451174033717,13.2609825637628));
#75181=CARTESIAN_POINT('Ctrl Pts',(89.181436061987,59.5402914201416,13.306593791151));
#75182=CARTESIAN_POINT('Ctrl Pts',(89.1325288722219,59.5354654369115,13.3493346501878));
#75183=CARTESIAN_POINT('Ctrl Pts',(89.0836216824568,59.5306394536815,13.3920755092247));
#75184=CARTESIAN_POINT('Ctrl Pts',(89.0323491549886,59.5258134704514,13.4319456632212));
#75185=CARTESIAN_POINT('Ctrl Pts',(88.9790953852693,59.5209874872213,13.4686995974264));
#75186=CARTESIAN_POINT('Ctrl Pts',(88.928365932876,59.5163902636292,13.5037113339731));
#75187=CARTESIAN_POINT('Ctrl Pts',(88.8756305667272,59.5117930400372,13.5360394014651));
#75188=CARTESIAN_POINT('Ctrl Pts',(88.8212046672429,59.5071958164451,13.5654476425597));
#75189=CARTESIAN_POINT('Ctrl Pts',(88.7658468482415,59.502519875874,13.5953594327751));
#75190=CARTESIAN_POINT('Ctrl Pts',(88.7087404404245,59.4978439353028,13.6222500853325));
#75191=CARTESIAN_POINT('Ctrl Pts',(88.6502499120977,59.4931679947317,13.6459159425371));
#75192=CARTESIAN_POINT('Ctrl Pts',(88.5929022176438,59.4885834163593,13.6691193976398));
#75193=CARTESIAN_POINT('Ctrl Pts',(88.5342244987779,59.4839988379869,13.6892227411431));
#75194=CARTESIAN_POINT('Ctrl Pts',(88.4745845594918,59.4794142596145,13.7060805443029));
#75195=CARTESIAN_POINT('Ctrl Pts',(88.4149810710979,59.4748324832565,13.722928044267));
#75196=CARTESIAN_POINT('Ctrl Pts',(88.3544170172239,59.4702507068986,13.7365337989402));
#75197=CARTESIAN_POINT('Ctrl Pts',(88.2932765788874,59.4656689305406,13.7468018231224));
#75198=CARTESIAN_POINT('Ctrl Pts',(88.2321510518664,59.4610882716152,13.7570673430741));
#75199=CARTESIAN_POINT('Ctrl Pts',(88.1704499212321,59.4565076126897,13.7639966642296));
#75200=CARTESIAN_POINT('Ctrl Pts',(88.1085667856242,59.4519269537643,13.7675450502243));
#75201=CARTESIAN_POINT('Ctrl Pts',(88.0444480223602,59.4471808111788,13.7712216273617));
#75202=CARTESIAN_POINT('Ctrl Pts',(87.9801344286854,59.4424346685933,13.7712682115861));
#75203=CARTESIAN_POINT('Ctrl Pts',(87.9160661354544,59.4376885260077,13.7676939786467));
#75204=CARTESIAN_POINT('Ctrl Pts',(87.8541533837963,59.4331020647113,13.7642399987577));
#75205=CARTESIAN_POINT('Ctrl Pts',(87.7924702044208,59.428515603415,13.7574051188854));
#75206=CARTESIAN_POINT('Ctrl Pts',(87.7314079802175,59.4239291421186,13.7472504685721));
#75207=CARTESIAN_POINT('Ctrl Pts',(87.667156861337,59.4191031588885,13.7365655049472));
#75208=CARTESIAN_POINT('Ctrl Pts',(87.6035939638048,59.4142771756584,13.7222046526664));
#75209=CARTESIAN_POINT('Ctrl Pts',(87.5411592640312,59.4094511924283,13.7042992762082));
#75210=CARTESIAN_POINT('Ctrl Pts',(87.4787245642576,59.4046252091983,13.6863938997501));
#75211=CARTESIAN_POINT('Ctrl Pts',(87.4174186483194,59.3997992259682,13.6649442861482));
#75212=CARTESIAN_POINT('Ctrl Pts',(87.3576561112549,59.3949732427381,13.6401399552262));
#75213=CARTESIAN_POINT('Ctrl Pts',(87.3007264179224,59.390376019146,13.6165113908768));
#75214=CARTESIAN_POINT('Ctrl Pts',(87.2449633266387,59.385778795554,13.5897419971388));
#75215=CARTESIAN_POINT('Ctrl Pts',(87.1907363001367,59.3811815719619,13.559968640329));
#75216=CARTESIAN_POINT('Ctrl Pts',(87.1355807593645,59.3765056313907,13.5296854826238));
#75217=CARTESIAN_POINT('Ctrl Pts',(87.0820149078883,59.3718296908196,13.4962946371064));
#75218=CARTESIAN_POINT('Ctrl Pts',(87.0304075300075,59.3671537502485,13.4599918376354));
#75219=CARTESIAN_POINT('Ctrl Pts',(86.9798084976009,59.3625691718761,13.4243983507675));
#75220=CARTESIAN_POINT('Ctrl Pts',(86.9310925309854,59.3579845935037,13.3860059855364));
#75221=CARTESIAN_POINT('Ctrl Pts',(86.8845813043578,59.3534000151312,13.3450448614915));
#75222=CARTESIAN_POINT('Ctrl Pts',(86.8380985045819,59.3488182387733,13.3041087721722));
#75223=CARTESIAN_POINT('Ctrl Pts',(86.7938181541273,59.3442364624153,13.2606073728211));
#75224=CARTESIAN_POINT('Ctrl Pts',(86.7520292715015,59.3396546860573,13.2148113597906));
#75225=CARTESIAN_POINT('Ctrl Pts',(86.7102505806119,59.3350740271319,13.1690265157805));
#75226=CARTESIAN_POINT('Ctrl Pts',(86.6709624942735,59.3304933682064,13.1209485448884));
#75227=CARTESIAN_POINT('Ctrl Pts',(86.6344160838686,59.325912709281,13.0708838527156));
#75228=CARTESIAN_POINT('Ctrl Pts',(86.5965493756957,59.3211665666955,13.0190104931359));
#75229=CARTESIAN_POINT('Ctrl Pts',(86.5616266256454,59.3164204241099,12.9650045487374));
#75230=CARTESIAN_POINT('Ctrl Pts',(86.5298788514076,59.3116742815244,12.909240759684));
#75231=CARTESIAN_POINT('Ctrl Pts',(86.4991992131193,59.307087820228,12.8553531118466));
#75232=CARTESIAN_POINT('Ctrl Pts',(86.4714844602057,59.3025013589316,12.799824536575));
#75233=CARTESIAN_POINT('Ctrl Pts',(86.4468955220396,59.2979148976352,12.743016999509));
#75234=CARTESIAN_POINT('Ctrl Pts',(86.4210224587854,59.2930889144052,12.6832427632287));
#75235=CARTESIAN_POINT('Ctrl Pts',(86.398610877821,59.2882629311751,12.6220529188133));
#75236=CARTESIAN_POINT('Ctrl Pts',(86.3797890597276,59.283436947945,12.5598883516905));
#75237=CARTESIAN_POINT('Ctrl Pts',(86.3609672416341,59.2786109647149,12.4977237845676));
#75238=CARTESIAN_POINT('Ctrl Pts',(86.3457352631559,59.2737849814849,12.4345851427995));
#75239=CARTESIAN_POINT('Ctrl Pts',(86.3341587805129,59.2689589982548,12.370923531773));
#75240=CARTESIAN_POINT('Ctrl Pts',(86.317476416287,59.2620044843083,12.2791835607388));
#75241=CARTESIAN_POINT('Ctrl Pts',(86.3083194512944,59.2550499703619,12.1860357551626));
#75242=CARTESIAN_POINT('Ctrl Pts',(86.3068657192959,59.2480954564154,12.092479972224));
#75243=CARTESIAN_POINT('Ctrl Pts',(86.3067360921165,59.247475332467,12.0841377383939));
#75244=CARTESIAN_POINT('Ctrl Pts',(86.3066676863994,59.2468552085185,12.0757922827587));
#75245=CARTESIAN_POINT('Ctrl Pts',(86.3066606119924,59.2462350845701,12.0674443288396));
#75246=CARTESIAN_POINT('',(86.3066600110215,58.4524850846251,12.0661938267317));
#75247=CARTESIAN_POINT('Ctrl Pts',(86.3066606119916,59.2462350845034,12.0674443279418));
#75248=CARTESIAN_POINT('Ctrl Pts',(86.3066090340479,59.2417138945661,12.0065811967051));
#75249=CARTESIAN_POINT('Ctrl Pts',(86.3098218829355,59.2371927046287,11.9456054229486));
#75250=CARTESIAN_POINT('Ctrl Pts',(86.316308791185,59.2326715146914,11.8849018432859));
#75251=CARTESIAN_POINT('Ctrl Pts',(86.3227894495779,59.2281546807257,11.8242567489068));
#75252=CARTESIAN_POINT('Ctrl Pts',(86.3325378663834,59.2236378467601,11.7638838491837));
#75253=CARTESIAN_POINT('Ctrl Pts',(86.3455116517119,59.2191210127945,11.7041666166359));
#75254=CARTESIAN_POINT('Ctrl Pts',(86.3584780340612,59.2146067561822,11.6444834593736));
#75255=CARTESIAN_POINT('Ctrl Pts',(86.3746660274517,59.2100924995698,11.5854557406869));
#75256=CARTESIAN_POINT('Ctrl Pts',(86.3939818959597,59.2055782429575,11.5274581847191));
#75257=CARTESIAN_POINT('Ctrl Pts',(86.4132943289906,59.2010647892408,11.469470944067));
#75258=CARTESIAN_POINT('Ctrl Pts',(86.4357333662765,59.1965513355241,11.4125140007435));
#75259=CARTESIAN_POINT('Ctrl Pts',(86.4611556745391,59.1920378818073,11.3569461216265));
#75260=CARTESIAN_POINT('Ctrl Pts',(86.4866007770444,59.1875203812213,11.3013284190351));
#75261=CARTESIAN_POINT('Ctrl Pts',(86.5150342723639,59.1830028806352,11.2471027464347));
#75262=CARTESIAN_POINT('Ctrl Pts',(86.5462656085468,59.1784853800492,11.1946057160537));
#75263=CARTESIAN_POINT('Ctrl Pts',(86.5775117273783,59.1739657412061,11.1420838373874));
#75264=CARTESIAN_POINT('Ctrl Pts',(86.6115580285535,59.169446102363,11.091292665473));
#75265=CARTESIAN_POINT('Ctrl Pts',(86.6481708840654,59.1649264635199,11.0425393821154));
#75266=CARTESIAN_POINT('Ctrl Pts',(86.6848489330696,59.1603987769287,10.9936992878067));
#75267=CARTESIAN_POINT('Ctrl Pts',(86.7241023185719,59.1558710903375,10.9469047261865));
#75268=CARTESIAN_POINT('Ctrl Pts',(86.7656582713082,59.1513434037462,10.902428423182));
#75269=CARTESIAN_POINT('Ctrl Pts',(86.7913530637336,59.1485438537547,10.8749279257008));
#75270=CARTESIAN_POINT('Ctrl Pts',(86.8179274394261,59.1457443037632,10.8483130006402));
#75271=CARTESIAN_POINT('Ctrl Pts',(86.8453106821457,59.1429447537717,10.8226403376978));
#75272=CARTESIAN_POINT('Ctrl Pts',(86.8902775124721,59.1383475301797,10.7804825008638));
#75273=CARTESIAN_POINT('Ctrl Pts',(86.9376265916061,59.1337503065876,10.7406806479449));
#75274=CARTESIAN_POINT('Ctrl Pts',(86.9870811113661,59.1291530829955,10.7035151578463));
#75275=CARTESIAN_POINT('Ctrl Pts',(87.0373824270928,59.1244771424244,10.6657132934129));
#75276=CARTESIAN_POINT('Ctrl Pts',(87.0898616419325,59.1198012018533,10.6306393569566));
#75277=CARTESIAN_POINT('Ctrl Pts',(87.1441885773489,59.1151252612821,10.5985488787828));
#75278=CARTESIAN_POINT('Ctrl Pts',(87.1974540304404,59.1105406829097,10.5670854095709));
#75279=CARTESIAN_POINT('Ctrl Pts',(87.2524951897762,59.1059561045373,10.5384901321586));
#75280=CARTESIAN_POINT('Ctrl Pts',(87.3089699298852,59.1013715261649,10.512961489127));
#75281=CARTESIAN_POINT('Ctrl Pts',(87.3654101536167,59.0967897498069,10.4874484487574));
#75282=CARTESIAN_POINT('Ctrl Pts',(87.4232817578894,59.092207973449,10.4649985356));
#75283=CARTESIAN_POINT('Ctrl Pts',(87.4822190784173,59.087626197091,10.4457637293993));
#75284=CARTESIAN_POINT('Ctrl Pts',(87.5411420249399,59.0830455381655,10.4265336143044));
#75285=CARTESIAN_POINT('Ctrl Pts',(87.6011296880393,59.0784648792401,10.4105172074319));
#75286=CARTESIAN_POINT('Ctrl Pts',(87.661799478708,59.0738842203146,10.3978172067998));
#75287=CARTESIAN_POINT('Ctrl Pts',(87.7246610629982,59.0691380777291,10.384658398249));
#75288=CARTESIAN_POINT('Ctrl Pts',(87.7882544484531,59.0643919351436,10.3750603865884));
#75289=CARTESIAN_POINT('Ctrl Pts',(87.8521430228283,59.0596457925581,10.3690794666798));
#75290=CARTESIAN_POINT('Ctrl Pts',(87.9138821021699,59.0550593312617,10.3632997714465));
#75291=CARTESIAN_POINT('Ctrl Pts',(87.9758962913229,59.0504728699653,10.3608975756909));
#75292=CARTESIAN_POINT('Ctrl Pts',(88.0377894691039,59.0458864086689,10.3618705565758));
#75293=CARTESIAN_POINT('Ctrl Pts',(88.1029149370244,59.0410604254388,10.362894350113));
#75294=CARTESIAN_POINT('Ctrl Pts',(88.1679057646038,59.0362344422087,10.3676554793341));
#75295=CARTESIAN_POINT('Ctrl Pts',(88.2323073446897,59.0314084589786,10.3760893826044));
#75296=CARTESIAN_POINT('Ctrl Pts',(88.2967089247756,59.0265824757486,10.3845232858747));
#75297=CARTESIAN_POINT('Ctrl Pts',(88.3605206351605,59.0217564925185,10.3966297663892));
#75298=CARTESIAN_POINT('Ctrl Pts',(88.4233043312516,59.0169305092884,10.4122829824812));
#75299=CARTESIAN_POINT('Ctrl Pts',(88.483111975644,59.0123332856963,10.4271942100756));
#75300=CARTESIAN_POINT('Ctrl Pts',(88.5422324368774,59.0077360621043,10.4453846980889));
#75301=CARTESIAN_POINT('Ctrl Pts',(88.6002800222825,59.0031388385122,10.466773971279));
#75302=CARTESIAN_POINT('Ctrl Pts',(88.6593215403238,58.998462897941,10.4885294870361));
#75303=CARTESIAN_POINT('Ctrl Pts',(88.7172525581037,58.9937869573699,10.5135943267067));
#75304=CARTESIAN_POINT('Ctrl Pts',(88.7736793107733,58.9891110167988,10.5418296996338));
#75305=CARTESIAN_POINT('Ctrl Pts',(88.8290035532396,58.9845264384264,10.5695133876725));
#75306=CARTESIAN_POINT('Ctrl Pts',(88.8828813079232,58.979941860054,10.6002445878048));
#75307=CARTESIAN_POINT('Ctrl Pts',(88.9349602905783,58.9753572816816,10.6338435081897));
#75308=CARTESIAN_POINT('Ctrl Pts',(88.9870074434662,58.9707755053236,10.6674218934996));
#75309=CARTESIAN_POINT('Ctrl Pts',(89.037257577369,58.9661937289657,10.7038642483169));
#75310=CARTESIAN_POINT('Ctrl Pts',(89.0853846750293,58.9616119526077,10.7429458039588));
#75311=CARTESIAN_POINT('Ctrl Pts',(89.1335000351496,58.9570312936823,10.7820178281445));
#75312=CARTESIAN_POINT('Ctrl Pts',(89.1794929919092,58.9524506347568,10.8237274546321));
#75313=CARTESIAN_POINT('Ctrl Pts',(89.2230697507249,58.9478699758314,10.8678089655744));
#75314=CARTESIAN_POINT('Ctrl Pts',(89.2682207899355,58.9431238332458,10.913482991893));
#75315=CARTESIAN_POINT('Ctrl Pts',(89.3107772563399,58.9383776906603,10.9617031916916));
#75316=CARTESIAN_POINT('Ctrl Pts',(89.3504550374916,58.9336315480748,11.0121332920438));
#75317=CARTESIAN_POINT('Ctrl Pts',(89.3887978820859,58.9290450867784,11.0608667001265));
#75318=CARTESIAN_POINT('Ctrl Pts',(89.4244524370856,58.9244586254821,11.1116631853249));
#75319=CARTESIAN_POINT('Ctrl Pts',(89.4572057983156,58.9198721641857,11.1641886979427));
#75320=CARTESIAN_POINT('Ctrl Pts',(89.4916696609342,58.9150461809556,11.2194572866571));
#75321=CARTESIAN_POINT('Ctrl Pts',(89.5229206799675,58.9102201977255,11.2766398874224));
#75322=CARTESIAN_POINT('Ctrl Pts',(89.5507665166544,58.9053942144955,11.3353195569949));
#75323=CARTESIAN_POINT('Ctrl Pts',(89.5786123533412,58.9005682312654,11.3939992265674));
#75324=CARTESIAN_POINT('Ctrl Pts',(89.6030528355372,58.8957422480353,11.4541753354705));
#75325=CARTESIAN_POINT('Ctrl Pts',(89.6239560364055,58.8909162648052,11.5154115327915));
#75326=CARTESIAN_POINT('Ctrl Pts',(89.6438683907591,58.8863190412132,11.5737450324314));
#75327=CARTESIAN_POINT('Ctrl Pts',(89.6606530417143,58.8817218176211,11.6332798817462));
#75328=CARTESIAN_POINT('Ctrl Pts',(89.6741683989992,58.877124594029,11.693648402487));
#75329=CARTESIAN_POINT('Ctrl Pts',(89.6879151759822,58.8724486534579,11.7550505965932));
#75330=CARTESIAN_POINT('Ctrl Pts',(89.6982793859158,58.8677727128868,11.8173148091167));
#75331=CARTESIAN_POINT('Ctrl Pts',(89.7051640522025,58.8630967723156,11.880034949991));
#75332=CARTESIAN_POINT('Ctrl Pts',(89.711914200473,58.8585121939432,11.9415296155013));
#75333=CARTESIAN_POINT('Ctrl Pts',(89.715319496131,58.8539276155708,12.0034620227918));
#75334=CARTESIAN_POINT('Ctrl Pts',(89.7153399075691,58.8493430371984,12.0654386915373));
#75335=CARTESIAN_POINT('Ctrl Pts',(89.7153603065322,58.8447612608404,12.1273774812223));
#75336=CARTESIAN_POINT('Ctrl Pts',(89.7119999232045,58.8401794844825,12.1893599707316));
#75337=CARTESIAN_POINT('Ctrl Pts',(89.7052707591578,58.8355977081245,12.2509903518097));
#75338=CARTESIAN_POINT('Ctrl Pts',(89.6985432362622,58.8310170491991,12.3126057020819));
#75339=CARTESIAN_POINT('Ctrl Pts',(89.6884486188747,58.8264363902736,12.3738686085835));
#75340=CARTESIAN_POINT('Ctrl Pts',(89.6750507883657,58.8218557313482,12.4343881232336));
#75341=CARTESIAN_POINT('Ctrl Pts',(89.661168939713,58.8171095887627,12.4970940025428));
#75342=CARTESIAN_POINT('Ctrl Pts',(89.6437407037342,58.8123634461771,12.5590011676541));
#75343=CARTESIAN_POINT('Ctrl Pts',(89.6228944881943,58.8076173035916,12.6196885356668));
#75344=CARTESIAN_POINT('Ctrl Pts',(89.6027496318131,58.8030308422952,12.6783341114277));
#75345=CARTESIAN_POINT('Ctrl Pts',(89.5794134157189,58.7984443809988,12.7358402086623));
#75346=CARTESIAN_POINT('Ctrl Pts',(89.5530510031723,58.7938579197024,12.7918467739235));
#75347=CARTESIAN_POINT('Ctrl Pts',(89.5253118481611,58.7890319364724,12.8507782086959));
#75348=CARTESIAN_POINT('Ctrl Pts',(89.4942220487179,58.7842059532423,12.9080486233223));
#75349=CARTESIAN_POINT('Ctrl Pts',(89.4600275633828,58.7793799700122,12.9632702804379));
#75350=CARTESIAN_POINT('Ctrl Pts',(89.4258330780476,58.7745539867822,13.0184919375534));
#75351=CARTESIAN_POINT('Ctrl Pts',(89.3885343422863,58.7697280035521,13.0716643511086));
#75352=CARTESIAN_POINT('Ctrl Pts',(89.3484263867851,58.764902020322,13.1224400103796));
#75353=CARTESIAN_POINT('Ctrl Pts',(89.3102196151348,58.76030479673,13.1708088188845));
#75354=CARTESIAN_POINT('Ctrl Pts',(89.2693071017345,58.7557075731379,13.2172015881259));
#75355=CARTESIAN_POINT('Ctrl Pts',(89.2259209424767,58.7511103495458,13.261299936891));
#75356=CARTESIAN_POINT('Ctrl Pts',(89.1817918940987,58.7464344089747,13.3061533693988));
#75357=CARTESIAN_POINT('Ctrl Pts',(89.1351039456151,58.7417584684036,13.3486325934397));
#75358=CARTESIAN_POINT('Ctrl Pts',(89.0861456619014,58.7370825278324,13.3884358741711));
#75359=CARTESIAN_POINT('Ctrl Pts',(89.0381439635799,58.73249794946,13.4274614471476));
#75360=CARTESIAN_POINT('Ctrl Pts',(88.9879602652018,58.7279133710876,13.4639143692309));
#75361=CARTESIAN_POINT('Ctrl Pts',(88.9359034248243,58.7233287927152,13.4975475857785));
#75362=CARTESIAN_POINT('Ctrl Pts',(88.883878400681,58.7187470163572,13.5311602462899));
#75363=CARTESIAN_POINT('Ctrl Pts',(88.8299829312574,58.7141652399993,13.5619563427552));
#75364=CARTESIAN_POINT('Ctrl Pts',(88.7745560530864,58.7095834636413,13.5897312720408));
#75365=CARTESIAN_POINT('Ctrl Pts',(88.719142692772,58.7050028047159,13.6174994274015));
#75366=CARTESIAN_POINT('Ctrl Pts',(88.6621991200432,58.7004221457904,13.64224765033));
#75367=CARTESIAN_POINT('Ctrl Pts',(88.6040884278359,58.695841486865,13.6638175591622));
#75368=CARTESIAN_POINT('Ctrl Pts',(88.5438783935489,58.6910953442794,13.6861667155915));
#75369=CARTESIAN_POINT('Ctrl Pts',(88.48241581987,58.6863492016939,13.7051032553549));
#75370=CARTESIAN_POINT('Ctrl Pts',(88.4201241156717,58.6816030591084,13.7205066616898));
#75371=CARTESIAN_POINT('Ctrl Pts',(88.3599281807109,58.677016597812,13.7353918291104));
#75372=CARTESIAN_POINT('Ctrl Pts',(88.298958556223,58.6724301365156,13.746977815929));
#75373=CARTESIAN_POINT('Ctrl Pts',(88.23760731508,58.6678436752192,13.7552080867532));
#75374=CARTESIAN_POINT('Ctrl Pts',(88.1730520857285,58.6630176919892,13.7638681726907));
#75375=CARTESIAN_POINT('Ctrl Pts',(88.1080749291716,58.6581917087591,13.7688123760322));
#75376=CARTESIAN_POINT('Ctrl Pts',(88.0431349993862,58.653365725529,13.770037023487));
#75377=CARTESIAN_POINT('Ctrl Pts',(87.9781950696008,58.648539742299,13.7712616709419));
#75378=CARTESIAN_POINT('Ctrl Pts',(87.9132930111233,58.6437137590689,13.7687668647215));
#75379=CARTESIAN_POINT('Ctrl Pts',(87.8488807993496,58.6388877758388,13.7626119769648));
#75380=CARTESIAN_POINT('Ctrl Pts',(87.7875218336287,58.6342905522468,13.7567488411327));
#75381=CARTESIAN_POINT('Ctrl Pts',(87.7263553893494,58.6296933286547,13.7475407531209));
#75382=CARTESIAN_POINT('Ctrl Pts',(87.6657748338337,58.6250961050626,13.7350100120267));
#75383=CARTESIAN_POINT('Ctrl Pts',(87.6041569743401,58.6204201644915,13.7222647105431));
#75384=CARTESIAN_POINT('Ctrl Pts',(87.5431457933917,58.6157442239204,13.7060818551707));
#75385=CARTESIAN_POINT('Ctrl Pts',(87.4831513020492,58.6110682833492,13.6865402147653));
#75386=CARTESIAN_POINT('Ctrl Pts',(87.42432903019,58.6064837049768,13.6673803942755));
#75387=CARTESIAN_POINT('Ctrl Pts',(87.3664845826797,58.6018991266044,13.6449920266809));
#75388=CARTESIAN_POINT('Ctrl Pts',(87.3099930395823,58.597314548232,13.6195005880417));
#75389=CARTESIAN_POINT('Ctrl Pts',(87.2535360231321,58.592732771874,13.5940247293258));
#75390=CARTESIAN_POINT('Ctrl Pts',(87.1984307345598,58.5881509955161,13.5654497690762));
#75391=CARTESIAN_POINT('Ctrl Pts',(87.1450329582858,58.5835692191581,13.5339495625752));
#75392=CARTESIAN_POINT('Ctrl Pts',(87.0916482049982,58.5789885602326,13.5024570385433));
#75393=CARTESIAN_POINT('Ctrl Pts',(87.0399705755609,58.5744079013072,13.4680409430503));
#75394=CARTESIAN_POINT('Ctrl Pts',(86.9903300709222,58.5698272423817,13.43092041214));
#75395=CARTESIAN_POINT('Ctrl Pts',(86.9388962233326,58.5650810997962,13.3924588424363));
#75396=CARTESIAN_POINT('Ctrl Pts',(86.8896500114354,58.5603349572107,13.3510939888136));
#75397=CARTESIAN_POINT('Ctrl Pts',(86.8429223403631,58.5555888146252,13.3071161978869));
#75398=CARTESIAN_POINT('Ctrl Pts',(86.7977667954163,58.5510023533288,13.2646180149199));
#75399=CARTESIAN_POINT('Ctrl Pts',(86.7549633136975,58.5464158920324,13.2196803675238));
#75400=CARTESIAN_POINT('Ctrl Pts',(86.7147720516274,58.541829430736,13.1726019796918));
#75401=CARTESIAN_POINT('Ctrl Pts',(86.67248185354,58.5370034475059,13.1230649847206));
#75402=CARTESIAN_POINT('Ctrl Pts',(86.6330845942958,58.5321774642759,13.0711580296476));
#75403=CARTESIAN_POINT('Ctrl Pts',(86.5968324044532,58.5273514810458,13.0172648670615));
#75404=CARTESIAN_POINT('Ctrl Pts',(86.5605802146106,58.5225254978157,12.9633717044754));
#75405=CARTESIAN_POINT('Ctrl Pts',(86.5274733578954,58.5176995145857,12.9074929313042));
#75406=CARTESIAN_POINT('Ctrl Pts',(86.4977071054124,58.5128735313556,12.8500404650213));
#75407=CARTESIAN_POINT('Ctrl Pts',(86.4666678734959,58.5078411607947,12.7901309945178));
#75408=CARTESIAN_POINT('Ctrl Pts',(86.4391419040733,58.5028087902338,12.7282820959685));
#75409=CARTESIAN_POINT('Ctrl Pts',(86.4153585462241,58.497776419673,12.6649183471827));
#75410=CARTESIAN_POINT('Ctrl Pts',(86.3923709072428,58.492912416936,12.6036745568471));
#75411=CARTESIAN_POINT('Ctrl Pts',(86.3728796178103,58.4880484141989,12.5410160954335));
#75412=CARTESIAN_POINT('Ctrl Pts',(86.3570458087894,58.4831844114619,12.4773518797536));
#75413=CARTESIAN_POINT('Ctrl Pts',(86.3412447005935,58.4783304541222,12.4138191468002));
#75414=CARTESIAN_POINT('Ctrl Pts',(86.3290861550402,58.4734764967825,12.3492851894886));
#75415=CARTESIAN_POINT('Ctrl Pts',(86.3206822455971,58.4686225394428,12.2841759032306));
#75416=CARTESIAN_POINT('Ctrl Pts',(86.3122999148258,58.4637810455825,12.2192337977265));
#75417=CARTESIAN_POINT('Ctrl Pts',(86.3076530849219,58.4589395517222,12.153719713652));
#75418=CARTESIAN_POINT('Ctrl Pts',(86.3068028996812,58.4540980578619,12.0880698632754));
#75419=CARTESIAN_POINT('Ctrl Pts',(86.3067084848801,58.4535604001163,12.0807793137938));
#75420=CARTESIAN_POINT('Ctrl Pts',(86.3066608404519,58.4530227423707,12.0734871001454));
#75421=CARTESIAN_POINT('Ctrl Pts',(86.3066600110215,58.4524850846251,12.0661938267317));
#75422=CARTESIAN_POINT('',(86.3066607017018,57.6587350846356,12.0644534307351));
#75423=CARTESIAN_POINT('Ctrl Pts',(86.3066600110214,58.4524850845702,12.0661938259872));
#75424=CARTESIAN_POINT('Ctrl Pts',(86.3066526701297,58.4477265146277,12.0016443018099));
#75425=CARTESIAN_POINT('Ctrl Pts',(86.3103167313048,58.4429679446852,11.9371518094558));
#75426=CARTESIAN_POINT('Ctrl Pts',(86.3176069473779,58.4382093747427,11.8731404528388));
#75427=CARTESIAN_POINT('Ctrl Pts',(86.3249149448926,58.4334391982535,11.8089729672149));
#75428=CARTESIAN_POINT('Ctrl Pts',(86.335866710533,58.4286690217644,11.7452894092002));
#75429=CARTESIAN_POINT('Ctrl Pts',(86.3503654536597,58.4238988452752,11.6825058812692));
#75430=CARTESIAN_POINT('Ctrl Pts',(86.3648829022572,58.41912251457,11.6196413535275));
#75431=CARTESIAN_POINT('Ctrl Pts',(86.3829563199365,58.4143461838648,11.5576796008999));
#75432=CARTESIAN_POINT('Ctrl Pts',(86.4044392596024,58.4095698531597,11.4970207182917));
#75433=CARTESIAN_POINT('Ctrl Pts',(86.4259782863255,58.4047810525441,11.4362034691719));
#75434=CARTESIAN_POINT('Ctrl Pts',(86.4509444481393,58.3999922519284,11.3766963024248));
#75435=CARTESIAN_POINT('Ctrl Pts',(86.4791434823621,58.3952034513128,11.3188785607612));
#75436=CARTESIAN_POINT('Ctrl Pts',(86.4955217920549,58.392422063166,11.2852973795325));
#75437=CARTESIAN_POINT('Ctrl Pts',(86.5129898292057,58.3896406750192,11.2522856335913));
#75438=CARTESIAN_POINT('Ctrl Pts',(86.5315028123033,58.3868592868723,11.21991317987));
#75439=CARTESIAN_POINT('Ctrl Pts',(86.5621020376408,58.3822620632802,11.1664062976502));
#75440=CARTESIAN_POINT('Ctrl Pts',(86.5956704799675,58.3776648396882,11.114451678314));
#75441=CARTESIAN_POINT('Ctrl Pts',(86.6320259039401,58.3730676160961,11.0643986431739));
#75442=CARTESIAN_POINT('Ctrl Pts',(86.6690038317109,58.368391675525,11.0134885638551));
#75443=CARTESIAN_POINT('Ctrl Pts',(86.7088649000607,58.3637157349538,10.964546309731));
#75444=CARTESIAN_POINT('Ctrl Pts',(86.7513685586074,58.3590397943827,10.9179131272177));
#75445=CARTESIAN_POINT('Ctrl Pts',(86.7930417472969,58.3544552160103,10.8721911004435));
#75446=CARTESIAN_POINT('Ctrl Pts',(86.8372548295851,58.3498706376379,10.8286891181222));
#75447=CARTESIAN_POINT('Ctrl Pts',(86.8837390657971,58.3452860592655,10.7876973668884));
#75448=CARTESIAN_POINT('Ctrl Pts',(86.9301948916535,58.3407042829075,10.746730669099));
#75449=CARTESIAN_POINT('Ctrl Pts',(86.9789187380448,58.3361225065496,10.7082714962698));
#75450=CARTESIAN_POINT('Ctrl Pts',(87.0296057165671,58.3315407301916,10.6725725364967));
#75451=CARTESIAN_POINT('Ctrl Pts',(87.0802803332294,58.3269600712662,10.6368822832111));
#75452=CARTESIAN_POINT('Ctrl Pts',(87.1329167155715,58.3223794123407,10.6039511996096));
#75453=CARTESIAN_POINT('Ctrl Pts',(87.1871793207144,58.3177987534153,10.5739898378424));
#75454=CARTESIAN_POINT('Ctrl Pts',(87.243402249612,58.3130526108298,10.5429460737646));
#75455=CARTESIAN_POINT('Ctrl Pts',(87.3013706727908,58.3083064682442,10.5150910488029));
#75456=CARTESIAN_POINT('Ctrl Pts',(87.3606837766397,58.3035603256587,10.4906068283649));
#75457=CARTESIAN_POINT('Ctrl Pts',(87.4180013245791,58.2989738643623,10.4669463657075));
#75458=CARTESIAN_POINT('Ctrl Pts',(87.4765739800833,58.2943874030659,10.4464335836454));
#75459=CARTESIAN_POINT('Ctrl Pts',(87.5360224153988,58.2898009417696,10.4291826217545));
#75460=CARTESIAN_POINT('Ctrl Pts',(87.5985754673809,58.2849749585395,10.4110307509748));
#75461=CARTESIAN_POINT('Ctrl Pts',(87.6620976550911,58.2801489753094,10.396490885452));
#75462=CARTESIAN_POINT('Ctrl Pts',(87.7261354625014,58.2753229920793,10.3856348519218));
#75463=CARTESIAN_POINT('Ctrl Pts',(87.7901732699117,58.2704970088493,10.3747788183917));
#75464=CARTESIAN_POINT('Ctrl Pts',(87.8547260444536,58.2656710256192,10.367606611504));
#75465=CARTESIAN_POINT('Ctrl Pts',(87.9193380054694,58.2608450423891,10.3641266456171));
#75466=CARTESIAN_POINT('Ctrl Pts',(87.980887251986,58.2562478187971,10.3608116359055));
#75467=CARTESIAN_POINT('Ctrl Pts',(88.0427429092134,58.251650595205,10.3608330737158));
#75468=CARTESIAN_POINT('Ctrl Pts',(88.1045126606968,58.2470533716129,10.3642273307256));
#75469=CARTESIAN_POINT('Ctrl Pts',(88.1673400784293,58.2423774310418,10.3676797066527));
#75470=CARTESIAN_POINT('Ctrl Pts',(88.2300780964387,58.2377014904707,10.3746216159706));
#75471=CARTESIAN_POINT('Ctrl Pts',(88.2923095521568,58.2330255498995,10.3850360588444));
#75472=CARTESIAN_POINT('Ctrl Pts',(88.3533250808252,58.2284409715271,10.3952470161553));
#75473=CARTESIAN_POINT('Ctrl Pts',(88.4138531382947,58.2238563931547,10.4087959412156));
#75474=CARTESIAN_POINT('Ctrl Pts',(88.4735041685626,58.2192718147823,10.4256144570064));
#75475=CARTESIAN_POINT('Ctrl Pts',(88.5331187411596,58.2146900384243,10.4424226936134));
#75476=CARTESIAN_POINT('Ctrl Pts',(88.5918568604838,58.2101082620664,10.4624964207244));
#75477=CARTESIAN_POINT('Ctrl Pts',(88.6493408668227,58.2055264857084,10.4857165528476));
#75478=CARTESIAN_POINT('Ctrl Pts',(88.7068108535999,58.200945826783,10.5089310218985));
#75479=CARTESIAN_POINT('Ctrl Pts',(88.7630268627893,58.1963651678575,10.5352901820531));
#75480=CARTESIAN_POINT('Ctrl Pts',(88.8176300070296,58.1917845089321,10.5646263398609));
#75481=CARTESIAN_POINT('Ctrl Pts',(88.8742057775462,58.1870383663465,10.5950223134824));
#75482=CARTESIAN_POINT('Ctrl Pts',(88.9290493747618,58.182292223761,10.6286142819556));
#75483=CARTESIAN_POINT('Ctrl Pts',(88.9817904408662,58.1775460811755,10.665164265332));
#75484=CARTESIAN_POINT('Ctrl Pts',(89.0327570635624,58.1729596198791,10.7004845451423));
#75485=CARTESIAN_POINT('Ctrl Pts',(89.081760021942,58.1683731585827,10.738566565451));
#75486=CARTESIAN_POINT('Ctrl Pts',(89.1284976780263,58.1637866972863,10.7791535541465));
#75487=CARTESIAN_POINT('Ctrl Pts',(89.1776761469809,58.1589607140563,10.8218601451642));
#75488=CARTESIAN_POINT('Ctrl Pts',(89.2243457518699,58.1541347308262,10.867340074808));
#75489=CARTESIAN_POINT('Ctrl Pts',(89.2682001629992,58.1493087475961,10.9152512933943));
#75490=CARTESIAN_POINT('Ctrl Pts',(89.3120545741286,58.1444827643661,10.9631625119805));
#75491=CARTESIAN_POINT('Ctrl Pts',(89.3530934420407,58.139656781136,11.0135044683705));
#75492=CARTESIAN_POINT('Ctrl Pts',(89.3910624827904,58.1348307979059,11.0658988155219));
#75493=CARTESIAN_POINT('Ctrl Pts',(89.4272317278088,58.1302335743138,11.1158095834077));
#75494=CARTESIAN_POINT('Ctrl Pts',(89.4607641494191,58.1256363507218,11.1677874584275));
#75495=CARTESIAN_POINT('Ctrl Pts',(89.4914163990448,58.1210391271297,11.2215225751749));
#75496=CARTESIAN_POINT('Ctrl Pts',(89.5225934986028,58.1163631865586,11.2761777833587));
#75497=CARTESIAN_POINT('Ctrl Pts',(89.5507904769835,58.1116872459874,11.3326506035374));
#75498=CARTESIAN_POINT('Ctrl Pts',(89.5757953476468,58.1070113054163,11.3905813479162));
#75499=CARTESIAN_POINT('Ctrl Pts',(89.6003116535118,58.1024267270439,11.4473801959205));
#75500=CARTESIAN_POINT('Ctrl Pts',(89.6217592582274,58.0978421486715,11.5055800186288));
#75501=CARTESIAN_POINT('Ctrl Pts',(89.6399843120806,58.0932575702991,11.5648164541856));
#75502=CARTESIAN_POINT('Ctrl Pts',(89.6581982270984,58.0886757939411,11.6240166854645));
#75503=CARTESIAN_POINT('Ctrl Pts',(89.673193347239,58.0840940175832,11.6842517878039));
#75504=CARTESIAN_POINT('Ctrl Pts',(89.6848648765849,58.0795122412252,11.7451398894603));
#75505=CARTESIAN_POINT('Ctrl Pts',(89.6965335594045,58.0749315822998,11.8060131413426));
#75506=CARTESIAN_POINT('Ctrl Pts',(89.7048801647596,58.0703509233743,11.8675385766705));
#75507=CARTESIAN_POINT('Ctrl Pts',(89.7098509154069,58.0657702644489,11.9293237298535));
#75508=CARTESIAN_POINT('Ctrl Pts',(89.7150012424042,58.0610241218634,11.9933409709199));
#75509=CARTESIAN_POINT('Ctrl Pts',(89.7165270178085,58.0562779792778,12.0576364801789));
#75510=CARTESIAN_POINT('Ctrl Pts',(89.7144272919947,58.0515318366923,12.1217700321634));
#75511=CARTESIAN_POINT('Ctrl Pts',(89.7123982102711,58.0469453753959,12.1837458469809));
#75512=CARTESIAN_POINT('Ctrl Pts',(89.7069838427897,58.0423589140995,12.2455699104637));
#75513=CARTESIAN_POINT('Ctrl Pts',(89.6982363011712,58.0377724528032,12.3068495372842));
#75514=CARTESIAN_POINT('Ctrl Pts',(89.6890319306496,58.0329464695731,12.371329412349));
#75515=CARTESIAN_POINT('Ctrl Pts',(89.6761368148682,58.028120486343,12.4352057930377));
#75516=CARTESIAN_POINT('Ctrl Pts',(89.6596721641605,58.0232945031129,12.4980357979638));
#75517=CARTESIAN_POINT('Ctrl Pts',(89.6432075134529,58.0184685198829,12.5608658028898));
#75518=CARTESIAN_POINT('Ctrl Pts',(89.6231736012971,58.0136425366528,12.6226488395295));
#75519=CARTESIAN_POINT('Ctrl Pts',(89.5997503617558,58.0088165534227,12.6829660635892));
#75520=CARTESIAN_POINT('Ctrl Pts',(89.5774374227569,58.0042193298306,12.7404241508301));
#75521=CARTESIAN_POINT('Ctrl Pts',(89.5519576535371,57.9996221062385,12.7967881832545));
#75522=CARTESIAN_POINT('Ctrl Pts',(89.5234393866178,57.9950248826465,12.8516856479581));
#75523=CARTESIAN_POINT('Ctrl Pts',(89.4944328093575,57.9903489420753,12.9075231066585));
#75524=CARTESIAN_POINT('Ctrl Pts',(89.4622828037395,57.9856730015042,12.9618427729636));
#75525=CARTESIAN_POINT('Ctrl Pts',(89.427176569858,57.9809970609331,13.0142714582782));
#75526=CARTESIAN_POINT('Ctrl Pts',(89.3927562691416,57.9764124825607,13.0656757507691));
#75527=CARTESIAN_POINT('Ctrl Pts',(89.3554945202088,57.9718279041882,13.1152618494036));
#75528=CARTESIAN_POINT('Ctrl Pts',(89.3156139832743,57.9672433258158,13.1627028723611));
#75529=CARTESIAN_POINT('Ctrl Pts',(89.2757578206295,57.9626615494579,13.2101149001916));
#75530=CARTESIAN_POINT('Ctrl Pts',(89.2332863705377,57.9580797730999,13.2553840630841));
#75531=CARTESIAN_POINT('Ctrl Pts',(89.1884636103591,57.9534979967419,13.2982151930081));
#75532=CARTESIAN_POINT('Ctrl Pts',(89.1436517818379,57.9489173378165,13.3410358770061));
#75533=CARTESIAN_POINT('Ctrl Pts',(89.0964901494892,57.944336678891,13.3814193568888));
#75534=CARTESIAN_POINT('Ctrl Pts',(89.0472792632542,57.9397560199656,13.4191075804049));
#75535=CARTESIAN_POINT('Ctrl Pts',(88.996290554723,57.9350098773801,13.4581573515216));
#75536=CARTESIAN_POINT('Ctrl Pts',(88.9431021148915,57.9302637347945,13.4943129924332));
#75537=CARTESIAN_POINT('Ctrl Pts',(88.8880832714187,57.925517592209,13.527334927591));
#75538=CARTESIAN_POINT('Ctrl Pts',(88.8349155058883,57.9209311309126,13.5592458583742));
#75539=CARTESIAN_POINT('Ctrl Pts',(88.7800390550594,57.9163446696162,13.5882304291864));
#75540=CARTESIAN_POINT('Ctrl Pts',(88.7238120874676,57.9117582083198,13.6141194280675));
#75541=CARTESIAN_POINT('Ctrl Pts',(88.6646487401417,57.9069322250898,13.6413604460047));
#75542=CARTESIAN_POINT('Ctrl Pts',(88.603990545554,57.9021062418597,13.6651734561096));
#75543=CARTESIAN_POINT('Ctrl Pts',(88.5422753220686,57.8972802586296,13.6854200714333));
#75544=CARTESIAN_POINT('Ctrl Pts',(88.4805600985832,57.8924542753996,13.7056666867569));
#75545=CARTESIAN_POINT('Ctrl Pts',(88.4177884923259,57.8876282921695,13.72234681567));
#75546=CARTESIAN_POINT('Ctrl Pts',(88.3544099792681,57.8828023089394,13.735384443961));
#75547=CARTESIAN_POINT('Ctrl Pts',(88.2940357132232,57.8782050853474,13.7478040669699));
#75548=CARTESIAN_POINT('Ctrl Pts',(88.2328629009972,57.8736078617553,13.7569697548862));
#75549=CARTESIAN_POINT('Ctrl Pts',(88.1712741059682,57.8690106381632,13.7627872720398));
#75550=CARTESIAN_POINT('Ctrl Pts',(88.1086307431569,57.8643346975921,13.7687044009191));
#75551=CARTESIAN_POINT('Ctrl Pts',(88.0455575182171,57.8596587570209,13.7711574203679));
#75552=CARTESIAN_POINT('Ctrl Pts',(87.9824694918876,57.8549828164498,13.7701011841164));
#75553=CARTESIAN_POINT('Ctrl Pts',(87.920614128957,57.8503982380774,13.7690655854381));
#75554=CARTESIAN_POINT('Ctrl Pts',(87.8587450711802,57.845813659705,13.7646566398585));
#75555=CARTESIAN_POINT('Ctrl Pts',(87.7972577095201,57.8412290813326,13.7568841086427));
#75556=CARTESIAN_POINT('Ctrl Pts',(87.7358079278645,57.8366473049746,13.7491163278626));
#75557=CARTESIAN_POINT('Ctrl Pts',(87.6747398837335,57.8320655286167,13.7379891014385));
#75558=CARTESIAN_POINT('Ctrl Pts',(87.614444735032,57.8274837522587,13.7235641035647));
#75559=CARTESIAN_POINT('Ctrl Pts',(87.5541642914916,57.8229030933333,13.7091426237503));
#75560=CARTESIAN_POINT('Ctrl Pts',(87.4946568640368,57.8183224344078,13.6914250874954));
#75561=CARTESIAN_POINT('Ctrl Pts',(87.4363022657435,57.8137417754824,13.6705240259468));
#75562=CARTESIAN_POINT('Ctrl Pts',(87.3758395138713,57.8089956328969,13.6488678799833));
#75563=CARTESIAN_POINT('Ctrl Pts',(87.3166150505194,57.8042494903113,13.6237939205407));
#75564=CARTESIAN_POINT('Ctrl Pts',(87.2590304710439,57.7995033477258,13.5954824821231));
#75565=CARTESIAN_POINT('Ctrl Pts',(87.2033832922507,57.7949168864294,13.5681235660754));
#75566=CARTESIAN_POINT('Ctrl Pts',(87.1492678216305,57.790330425133,13.5377418933054));
#75567=CARTESIAN_POINT('Ctrl Pts',(87.097020487904,57.7857439638366,13.5045465884249));
#75568=CARTESIAN_POINT('Ctrl Pts',(87.0420446056094,57.7809179806066,13.4696177022275));
#75569=CARTESIAN_POINT('Ctrl Pts',(86.989137861963,57.7760919973765,13.4315736159901));
#75570=CARTESIAN_POINT('Ctrl Pts',(86.9386539909095,57.7712660141464,13.3907070892796));
#75571=CARTESIAN_POINT('Ctrl Pts',(86.888170119856,57.7664400309164,13.3498405625691));
#75572=CARTESIAN_POINT('Ctrl Pts',(86.8401095488331,57.7616140476863,13.3061520885097));
#75573=CARTESIAN_POINT('Ctrl Pts',(86.7947799342,57.7567880644562,13.2599780513667));
#75574=CARTESIAN_POINT('Ctrl Pts',(86.7521948455824,57.7522542751182,13.216599666629));
#75575=CARTESIAN_POINT('Ctrl Pts',(86.7118345839947,57.7477204857802,13.1708391521557));
#75576=CARTESIAN_POINT('Ctrl Pts',(86.6739822128349,57.7431866964423,13.1229570816283));
#75577=CARTESIAN_POINT('Ctrl Pts',(86.6361827559377,57.7386592449402,13.0751419459949));
#75578=CARTESIAN_POINT('Ctrl Pts',(86.6008845694283,57.7341317934382,13.0252115336295));
#75579=CARTESIAN_POINT('Ctrl Pts',(86.5683338286842,57.7296043419362,12.9734630316111));
#75580=CARTESIAN_POINT('Ctrl Pts',(86.5358158593164,57.7250814485736,12.921766628857));
#75581=CARTESIAN_POINT('Ctrl Pts',(86.5060401334303,57.7205585552111,12.8682562039503));
#75582=CARTESIAN_POINT('Ctrl Pts',(86.4792110692454,57.7160356618486,12.8132599997442));
#75583=CARTESIAN_POINT('Ctrl Pts',(86.4523985287984,57.7115155540884,12.7582976671208));
#75584=CARTESIAN_POINT('Ctrl Pts',(86.4285292807412,57.7069954463283,12.7018518396974));
#75585=CARTESIAN_POINT('Ctrl Pts',(86.4077619763422,57.7024753385681,12.6442756047923));
#75586=CARTESIAN_POINT('Ctrl Pts',(86.3869919659206,57.6979546418286,12.5866918675851));
#75587=CARTESIAN_POINT('Ctrl Pts',(86.3693248955293,57.6934339450891,12.5279779177786));
#75588=CARTESIAN_POINT('Ctrl Pts',(86.3548706951831,57.6889132483495,12.4685053556498));
#75589=CARTESIAN_POINT('Ctrl Pts',(86.3404150396387,57.6843920964821,12.4090268060319));
#75590=CARTESIAN_POINT('Ctrl Pts',(86.3291730065193,57.6798709446147,12.3487900050384));
#75591=CARTESIAN_POINT('Ctrl Pts',(86.3212035647576,57.6753497927472,12.2881775034565));
#75592=CARTESIAN_POINT('Ctrl Pts',(86.3132266214071,57.670824385146,12.2275079476818));
#75593=CARTESIAN_POINT('Ctrl Pts',(86.3085284608619,57.6662989775448,12.1664625077594));
#75594=CARTESIAN_POINT('Ctrl Pts',(86.307116119423,57.6617735699435,12.1054278722451));
#75595=CARTESIAN_POINT('Ctrl Pts',(86.3068000242341,57.6607607415076,12.0917677514613));
#75596=CARTESIAN_POINT('Ctrl Pts',(86.3066483109801,57.6597479130716,12.0781081660735));
#75597=CARTESIAN_POINT('Ctrl Pts',(86.3066607017018,57.6587350846356,12.0644534307351));
#75598=CARTESIAN_POINT('',(86.3066601734134,56.8649850845176,12.0667688372946));
#75599=CARTESIAN_POINT('Ctrl Pts',(86.3066607017026,57.6587350845702,12.0644534298534));
#75600=CARTESIAN_POINT('Ctrl Pts',(86.3067373367494,57.6524708723721,11.980000667048));
#75601=CARTESIAN_POINT('Ctrl Pts',(86.3130947576162,57.6462066601741,11.8958234833704));
#75602=CARTESIAN_POINT('Ctrl Pts',(86.3255895191783,57.639942447976,11.8126892289375));
#75603=CARTESIAN_POINT('Ctrl Pts',(86.3316855142865,57.6368862386417,11.772129350637));
#75604=CARTESIAN_POINT('Ctrl Pts',(86.3392416907942,57.6338300293073,11.7318172679732));
#75605=CARTESIAN_POINT('Ctrl Pts',(86.3482375021317,57.630773819973,11.6918399924058));
#75606=CARTESIAN_POINT('Ctrl Pts',(86.3617692179229,57.6261765963809,11.6317052129194));
#75607=CARTESIAN_POINT('Ctrl Pts',(86.3785951317794,57.6215793727888,11.5721820122873));
#75608=CARTESIAN_POINT('Ctrl Pts',(86.3986436606239,57.6169821491968,11.5136578320698));
#75609=CARTESIAN_POINT('Ctrl Pts',(86.4190354748435,57.6123062086256,11.4541315586159));
#75610=CARTESIAN_POINT('Ctrl Pts',(86.4427612789035,57.6076302680545,11.3956393776817));
#75611=CARTESIAN_POINT('Ctrl Pts',(86.4696913753969,57.6029543274834,11.3385781421183));
#75612=CARTESIAN_POINT('Ctrl Pts',(86.4960952905178,57.598369749111,11.2826318137832));
#75613=CARTESIAN_POINT('Ctrl Pts',(86.5255791805818,57.5937851707386,11.2280614982444));
#75614=CARTESIAN_POINT('Ctrl Pts',(86.5579714037962,57.5892005923661,11.1752235217441));
#75615=CARTESIAN_POINT('Ctrl Pts',(86.5903438294479,57.5846188160082,11.1224178388948));
#75616=CARTESIAN_POINT('Ctrl Pts',(86.6256207981772,57.5800370396502,11.0713428287709));
#75617=CARTESIAN_POINT('Ctrl Pts',(86.6635850991102,57.5754552632923,11.0223295920358));
#75618=CARTESIAN_POINT('Ctrl Pts',(86.7015401410702,57.5708746043668,10.9733283089578));
#75619=CARTESIAN_POINT('Ctrl Pts',(86.7421809025778,57.5662939454414,10.9263882033198));
#75620=CARTESIAN_POINT('Ctrl Pts',(86.7852484933105,57.5617132865159,10.8818091034599));
#75621=CARTESIAN_POINT('Ctrl Pts',(86.8298719699235,57.5569671439304,10.835619512025));
#75622=CARTESIAN_POINT('Ctrl Pts',(86.8771006212783,57.5522210013449,10.7919652454218));
#75623=CARTESIAN_POINT('Ctrl Pts',(86.926604797949,57.5474748587594,10.7511380751696));
#75624=CARTESIAN_POINT('Ctrl Pts',(86.97444343453,57.542888397463,10.7116845120224));
#75625=CARTESIAN_POINT('Ctrl Pts',(87.0244064327555,57.5383019361666,10.6748710768518));
#75626=CARTESIAN_POINT('Ctrl Pts',(87.0761647280618,57.5337154748702,10.6409183006086));
#75627=CARTESIAN_POINT('Ctrl Pts',(87.1306260325454,57.5288894916401,10.6051923850988));
#75628=CARTESIAN_POINT('Ctrl Pts',(87.1870747377085,57.52406350841,10.5726344412704));
#75629=CARTESIAN_POINT('Ctrl Pts',(87.2450984343659,57.51923752518,10.5434463466402));
#75630=CARTESIAN_POINT('Ctrl Pts',(87.3031221310233,57.5144115419499,10.51425825201));
#75631=CARTESIAN_POINT('Ctrl Pts',(87.3627201938244,57.5095855587198,10.4884401931547));
#75632=CARTESIAN_POINT('Ctrl Pts',(87.4234594215836,57.5047595754897,10.4661340980213));
#75633=CARTESIAN_POINT('Ctrl Pts',(87.481319508846,57.5001623518977,10.4448853489259));
#75634=CARTESIAN_POINT('Ctrl Pts',(87.5404525647213,57.4955651283056,10.4267358449806));
#75635=CARTESIAN_POINT('Ctrl Pts',(87.6004942647793,57.4909679047135,10.4118355955496));
#75636=CARTESIAN_POINT('Ctrl Pts',(87.6615640421432,57.4862919641424,10.3966802132979));
#75637=CARTESIAN_POINT('Ctrl Pts',(87.7235734084541,57.4816160235713,10.3848866769984));
#75638=CARTESIAN_POINT('Ctrl Pts',(87.786118611517,57.4769400830001,10.376561277609));
#75639=CARTESIAN_POINT('Ctrl Pts',(87.8474417572882,57.4723555046277,10.3683985464106));
#75640=CARTESIAN_POINT('Ctrl Pts',(87.9092794601771,57.4677709262553,10.3635697150064));
#75641=CARTESIAN_POINT('Ctrl Pts',(87.9712392646679,57.4631863478829,10.3621238544055));
#75642=CARTESIAN_POINT('Ctrl Pts',(88.0331612004054,57.458604571525,10.3606788774895));
#75643=CARTESIAN_POINT('Ctrl Pts',(88.0952045819187,57.454022795167,10.3626127834504));
#75644=CARTESIAN_POINT('Ctrl Pts',(88.1569734296218,57.449441018809,10.3679226774247));
#75645=CARTESIAN_POINT('Ctrl Pts',(88.2187272127489,57.4448603598836,10.3732312763886));
#75646=CARTESIAN_POINT('Ctrl Pts',(88.2802060880323,57.4402797009581,10.3819141852975));
#75647=CARTESIAN_POINT('Ctrl Pts',(88.3410177415467,57.4356990420327,10.3939165314302));
#75648=CARTESIAN_POINT('Ctrl Pts',(88.4040263137057,57.4309528994472,10.4063524815923));
#75649=CARTESIAN_POINT('Ctrl Pts',(88.4663179493559,57.4262067568617,10.4223522512616));
#75650=CARTESIAN_POINT('Ctrl Pts',(88.5274687236262,57.4214606142762,10.4417971514876));
#75651=CARTESIAN_POINT('Ctrl Pts',(88.5865621146025,57.4168741529798,10.4605878390179));
#75652=CARTESIAN_POINT('Ctrl Pts',(88.6445897293,57.4122876916834,10.4825952498893));
#75653=CARTESIAN_POINT('Ctrl Pts',(88.7011878107857,57.407701230387,10.50766254571));
#75654=CARTESIAN_POINT('Ctrl Pts',(88.7607416529426,57.4028752471569,10.534038948221));
#75655=CARTESIAN_POINT('Ctrl Pts',(88.8187119786913,57.3980492639268,10.5638033120392));
#75656=CARTESIAN_POINT('Ctrl Pts',(88.8747054962242,57.3932232806968,10.5967186615927));
#75657=CARTESIAN_POINT('Ctrl Pts',(88.9306990137571,57.3883972974667,10.6296340111461));
#75658=CARTESIAN_POINT('Ctrl Pts',(88.9847152271377,57.3835713142366,10.6656999222634));
#75659=CARTESIAN_POINT('Ctrl Pts',(89.0363999319057,57.3787453310065,10.7046294350003));
#75660=CARTESIAN_POINT('Ctrl Pts',(89.0856346956381,57.3741481074145,10.7417136240349));
#75661=CARTESIAN_POINT('Ctrl Pts',(89.1329561745072,57.3695508838224,10.7815482876868));
#75662=CARTESIAN_POINT('Ctrl Pts',(89.1780407333497,57.3649536602303,10.823908714183));
#75663=CARTESIAN_POINT('Ctrl Pts',(89.2238972625354,57.3602777196592,10.8669944664629));
#75664=CARTESIAN_POINT('Ctrl Pts',(89.2674390656458,57.3556017790881,10.9126930483951));
#75665=CARTESIAN_POINT('Ctrl Pts',(89.3083578507059,57.3509258385169,10.9607229112971));
#75666=CARTESIAN_POINT('Ctrl Pts',(89.3484771324116,57.3463412601445,11.0078143290216));
#75667=CARTESIAN_POINT('Ctrl Pts',(89.3860746294626,57.3417566817721,11.0571463401991));
#75668=CARTESIAN_POINT('Ctrl Pts',(89.4208962488789,57.3371721033997,11.1084158506966));
#75669=CARTESIAN_POINT('Ctrl Pts',(89.4556965859279,57.3325903270417,11.1596540261622));
#75670=CARTESIAN_POINT('Ctrl Pts',(89.4877241239766,57.3280085506838,11.2128269326882));
#75671=CARTESIAN_POINT('Ctrl Pts',(89.5167665162233,57.3234267743258,11.2676003292707));
#75672=CARTESIAN_POINT('Ctrl Pts',(89.5458018254284,57.3188461154004,11.3223603673719));
#75673=CARTESIAN_POINT('Ctrl Pts',(89.5718531957369,57.3142654564749,11.3787196711139));
#75674=CARTESIAN_POINT('Ctrl Pts',(89.594753936296,57.3096847975495,11.4363188863663));
#75675=CARTESIAN_POINT('Ctrl Pts',(89.6184820028855,57.3049386549639,11.4959989657719));
#75676=CARTESIAN_POINT('Ctrl Pts',(89.6388271637822,57.3001925123784,11.5570097429308));
#75677=CARTESIAN_POINT('Ctrl Pts',(89.6556591957603,57.2954463697929,11.6189306928439));
#75678=CARTESIAN_POINT('Ctrl Pts',(89.6719249235205,57.2908599084965,11.6787683473381));
#75679=CARTESIAN_POINT('Ctrl Pts',(89.6849101381656,57.2862734472001,11.7394553673784));
#75680=CARTESIAN_POINT('Ctrl Pts',(89.6945493016383,57.2816869859037,11.8006010841146));
#75681=CARTESIAN_POINT('Ctrl Pts',(89.7046918577976,57.2768610026737,11.8649400558162));
#75682=CARTESIAN_POINT('Ctrl Pts',(89.7111292185952,57.2720350194436,11.9297863078811));
#75683=CARTESIAN_POINT('Ctrl Pts',(89.7138471512364,57.2672090362135,11.9946808922782));
#75684=CARTESIAN_POINT('Ctrl Pts',(89.7165650838775,57.2623830529835,12.0595754766754));
#75685=CARTESIAN_POINT('Ctrl Pts',(89.7155636757222,57.2575570697534,12.124517746688));
#75686=CARTESIAN_POINT('Ctrl Pts',(89.7108918878337,57.2527310865233,12.1890544809313));
#75687=CARTESIAN_POINT('Ctrl Pts',(89.7064415504673,57.2481338629312,12.2505320665497));
#75688=CARTESIAN_POINT('Ctrl Pts',(89.6986427178016,57.2435366393392,12.3118941150787));
#75689=CARTESIAN_POINT('Ctrl Pts',(89.6875086356423,57.2389394157471,12.3727468503782));
#75690=CARTESIAN_POINT('Ctrl Pts',(89.6761839076955,57.234263475176,12.4346415501142));
#75691=CARTESIAN_POINT('Ctrl Pts',(89.6614085816817,57.2295875346049,12.496008795041));
#75692=CARTESIAN_POINT('Ctrl Pts',(89.6432519754239,57.2249115940337,12.5564368708864));
#75693=CARTESIAN_POINT('Ctrl Pts',(89.6254501271968,57.2203270156613,12.6156842555341));
#75694=CARTESIAN_POINT('Ctrl Pts',(89.6043980960972,57.2157424372889,12.6740283306222));
#75695=CARTESIAN_POINT('Ctrl Pts',(89.5802126982047,57.2111578589165,12.7310912293762));
#75696=CARTESIAN_POINT('Ctrl Pts',(89.5560420820062,57.2065760825585,12.7881192522803));
#75697=CARTESIAN_POINT('Ctrl Pts',(89.5287420945357,57.2019943062006,12.8438671837755));
#75698=CARTESIAN_POINT('Ctrl Pts',(89.4984783620945,57.1974125298426,12.8979753349112));
#75699=CARTESIAN_POINT('Ctrl Pts',(89.4682220105632,57.1928318709172,12.9520702898098));
#75700=CARTESIAN_POINT('Ctrl Pts',(89.4350035973426,57.1882512119917,13.0045258141742));
#75701=CARTESIAN_POINT('Ctrl Pts',(89.3990346105331,57.1836705530663,13.0550069542538));
#75702=CARTESIAN_POINT('Ctrl Pts',(89.3617661863101,57.1789244104807,13.1073118065897));
#75703=CARTESIAN_POINT('Ctrl Pts',(89.3215449308692,57.1741782678952,13.1574963770492));
#75704=CARTESIAN_POINT('Ctrl Pts',(89.2786535032484,57.1694321253097,13.2052231701041));
#75705=CARTESIAN_POINT('Ctrl Pts',(89.237205133507,57.1648456640133,13.251344222138));
#75706=CARTESIAN_POINT('Ctrl Pts',(89.1932638475326,57.1602592027169,13.295169940474));
#75707=CARTESIAN_POINT('Ctrl Pts',(89.147122306736,57.1556727414205,13.3364333669016));
#75708=CARTESIAN_POINT('Ctrl Pts',(89.0985710844093,57.1508467581905,13.3798517217258));
#75709=CARTESIAN_POINT('Ctrl Pts',(89.0475839917287,57.1460207749604,13.420432411726));
#75710=CARTESIAN_POINT('Ctrl Pts',(88.9945388808011,57.1411947917303,13.4579145467853));
#75711=CARTESIAN_POINT('Ctrl Pts',(88.9414937698736,57.1363688085003,13.4953966818446));
#75712=CARTESIAN_POINT('Ctrl Pts',(88.8863912314035,57.1315428252702,13.5297799845778));
#75713=CARTESIAN_POINT('Ctrl Pts',(88.8296385826915,57.1267168420401,13.5608597614923));
#75714=CARTESIAN_POINT('Ctrl Pts',(88.7755761039937,57.1221196184481,13.5904663052485));
#75715=CARTESIAN_POINT('Ctrl Pts',(88.7197944707422,57.117522394856,13.6171970400385));
#75716=CARTESIAN_POINT('Ctrl Pts',(88.6626316871176,57.1129251712639,13.640849510253));
#75717=CARTESIAN_POINT('Ctrl Pts',(88.6044901210713,57.1082492306928,13.6649069751268));
#75718=CARTESIAN_POINT('Ctrl Pts',(88.5449200808534,57.1035732901217,13.6857794286762));
#75719=CARTESIAN_POINT('Ctrl Pts',(88.4843050542421,57.0988973495505,13.7033017929596));
#75720=CARTESIAN_POINT('Ctrl Pts',(88.4248743716193,57.0943127711781,13.7204817915301));
#75721=CARTESIAN_POINT('Ctrl Pts',(88.3644396833116,57.0897281928057,13.7344412886722));
#75722=CARTESIAN_POINT('Ctrl Pts',(88.3033818040932,57.0851436144333,13.7450734695764));
#75723=CARTESIAN_POINT('Ctrl Pts',(88.2423612423872,57.0805618380753,13.7556991522768));
#75724=CARTESIAN_POINT('Ctrl Pts',(88.1807187454674,57.0759800617174,13.7630014639232));
#75725=CARTESIAN_POINT('Ctrl Pts',(88.1188463311372,57.0713982853594,13.7669244558358));
#75726=CARTESIAN_POINT('Ctrl Pts',(88.0569890066415,57.066817626434,13.7708464909843));
#75727=CARTESIAN_POINT('Ctrl Pts',(87.9949023838495,57.0622369675085,13.7713908103042));
#75728=CARTESIAN_POINT('Ctrl Pts',(87.9329825753824,57.057656308583,13.7685534109261));
#75729=CARTESIAN_POINT('Ctrl Pts',(87.8688258143933,57.0529101659975,13.7656135059386));
#75730=CARTESIAN_POINT('Ctrl Pts',(87.8048487350968,57.048164023412,13.7590428266637));
#75731=CARTESIAN_POINT('Ctrl Pts',(87.7414881885438,57.0434178808265,13.7488957837863));
#75732=CARTESIAN_POINT('Ctrl Pts',(87.6802593718263,57.0388314195301,13.7390901324406));
#75733=CARTESIAN_POINT('Ctrl Pts',(87.6196067588616,57.0342449582337,13.7259451432318));
#75734=CARTESIAN_POINT('Ctrl Pts',(87.5599133660812,57.0296584969373,13.7095618894036));
#75735=CARTESIAN_POINT('Ctrl Pts',(87.4971025640516,57.0248325137073,13.6923230416036));
#75736=CARTESIAN_POINT('Ctrl Pts',(87.4353545312499,57.0200065304772,13.6714986216592));
#75737=CARTESIAN_POINT('Ctrl Pts',(87.3750933935017,57.0151805472471,13.6472645646481));
#75738=CARTESIAN_POINT('Ctrl Pts',(87.3148322557535,57.010354564017,13.6230305076371));
#75739=CARTESIAN_POINT('Ctrl Pts',(87.2560585664935,57.005528580787,13.5953871593694));
#75740=CARTESIAN_POINT('Ctrl Pts',(87.1991652214584,57.0007025975569,13.5645656902353));
#75741=CARTESIAN_POINT('Ctrl Pts',(87.1449687156773,56.9961053739648,13.5352052100406));
#75742=CARTESIAN_POINT('Ctrl Pts',(87.0922557705887,56.9915081503727,13.5028405964833));
#75743=CARTESIAN_POINT('Ctrl Pts',(87.0413798064858,56.9869109267807,13.4676460023592));
#75744=CARTESIAN_POINT('Ctrl Pts',(86.9896327074207,56.9822349862095,13.4318487810031));
#75745=CARTESIAN_POINT('Ctrl Pts',(86.9397866011751,56.9775590456384,13.3931239220507));
#75746=CARTESIAN_POINT('Ctrl Pts',(86.8921881765191,56.9728831050673,13.3517040636318));
#75747=CARTESIAN_POINT('Ctrl Pts',(86.8455197672612,56.9682985266949,13.3110934989321));
#75748=CARTESIAN_POINT('Ctrl Pts',(86.8010123979926,56.9637139483225,13.2678926518096));
#75749=CARTESIAN_POINT('Ctrl Pts',(86.7589623595588,56.95912936995,13.2223635165978));
#75750=CARTESIAN_POINT('Ctrl Pts',(86.716938021376,56.9545475935921,13.1768622080004));
#75751=CARTESIAN_POINT('Ctrl Pts',(86.6773683806839,56.9499658172341,13.1290358061143));
#75752=CARTESIAN_POINT('Ctrl Pts',(86.6405130711245,56.9453840408761,13.0791833069003));
#75753=CARTESIAN_POINT('Ctrl Pts',(86.6036667500704,56.9408033819507,13.0293429660282));
#75754=CARTESIAN_POINT('Ctrl Pts',(86.569533748481,56.9362227230252,12.9774779179155));
#75755=CARTESIAN_POINT('Ctrl Pts',(86.5383322802473,56.9316420640998,12.9239187740098));
#75756=CARTESIAN_POINT('Ctrl Pts',(86.5060036088653,56.9268959215143,12.8684247200164));
#75757=CARTESIAN_POINT('Ctrl Pts',(86.4768226869568,56.9221497789288,12.8111122929345));
#75758=CARTESIAN_POINT('Ctrl Pts',(86.4509807504232,56.9174036363432,12.7523780128688));
#75759=CARTESIAN_POINT('Ctrl Pts',(86.426008251262,56.9128171750468,12.6956198145131));
#75760=CARTESIAN_POINT('Ctrl Pts',(86.4041537327394,56.9082307137504,12.6375344444024));
#75761=CARTESIAN_POINT('Ctrl Pts',(86.3855400287221,56.9036442524541,12.5784985047522));
#75762=CARTESIAN_POINT('Ctrl Pts',(86.3659542483934,56.898818269224,12.5163794904813));
#75763=CARTESIAN_POINT('Ctrl Pts',(86.3499572278478,56.8939922859939,12.4532085212426));
#75764=CARTESIAN_POINT('Ctrl Pts',(86.3376312056248,56.8891663027639,12.3894373410898));
#75765=CARTESIAN_POINT('Ctrl Pts',(86.3253051834018,56.8843403195338,12.325666160937));
#75766=CARTESIAN_POINT('Ctrl Pts',(86.3166501691614,56.8795143363037,12.2612954223893));
#75767=CARTESIAN_POINT('Ctrl Pts',(86.3116850579265,56.8746883530737,12.1967805920066));
#75768=CARTESIAN_POINT('Ctrl Pts',(86.3083573900941,56.8714539302392,12.1535420993296));
#75769=CARTESIAN_POINT('Ctrl Pts',(86.3066797541958,56.8682195074047,12.1101749998648));
#75770=CARTESIAN_POINT('Ctrl Pts',(86.3066601734137,56.8649850845702,12.0667688380001));
#75771=CARTESIAN_POINT('',(86.3066603287391,56.0712350846273,12.0670585679921));
#75772=CARTESIAN_POINT('Ctrl Pts',(86.3066601734134,56.8649850845176,12.0667688372946));
#75773=CARTESIAN_POINT('Ctrl Pts',(86.3066326469133,56.8604381556952,12.0057487608988));
#75774=CARTESIAN_POINT('Ctrl Pts',(86.3098864040988,56.8558912268728,11.9445956778901));
#75775=CARTESIAN_POINT('Ctrl Pts',(86.3164380357149,56.8513442980503,11.88369644875));
#75776=CARTESIAN_POINT('Ctrl Pts',(86.3229791074586,56.8468046979349,11.8228953765471));
#75777=CARTESIAN_POINT('Ctrl Pts',(86.3328074517629,56.8422650978195,11.7623478602083));
#75778=CARTESIAN_POINT('Ctrl Pts',(86.3458876518779,56.8377254977041,11.7024402336185));
#75779=CARTESIAN_POINT('Ctrl Pts',(86.3589562899846,56.8331899102868,11.6425855613012));
#75780=CARTESIAN_POINT('Ctrl Pts',(86.375270979909,56.8286543228695,11.5833701651223));
#75781=CARTESIAN_POINT('Ctrl Pts',(86.3947447908381,56.8241187354522,11.5251729163059));
#75782=CARTESIAN_POINT('Ctrl Pts',(86.4142089121486,56.8195854048152,11.4670046247979));
#75783=CARTESIAN_POINT('Ctrl Pts',(86.4368288739004,56.8150520741782,11.4098539698692));
#75784=CARTESIAN_POINT('Ctrl Pts',(86.4624677567148,56.8105187435412,11.354085168643));
#75785=CARTESIAN_POINT('Ctrl Pts',(86.4881037872398,56.8059859172308,11.2983225716169));
#75786=CARTESIAN_POINT('Ctrl Pts',(86.516757853045,56.8014530909204,11.2439419956563));
#75787=CARTESIAN_POINT('Ctrl Pts',(86.5482455976834,56.79692026461,11.1912861072879));
#75788=CARTESIAN_POINT('Ctrl Pts',(86.57976336295,56.7923831166724,11.1385800164404));
#75789=CARTESIAN_POINT('Ctrl Pts',(86.6141199317628,56.7878459687348,11.0876023433603));
#75790=CARTESIAN_POINT('Ctrl Pts',(86.6510865547072,56.7833088207972,11.0386683802627));
#75791=CARTESIAN_POINT('Ctrl Pts',(86.6880724563637,56.7787693066611,10.9897088972851));
#75792=CARTESIAN_POINT('Ctrl Pts',(86.7276707835967,56.774229792525,10.9427956426883));
#75793=CARTESIAN_POINT('Ctrl Pts',(86.7696133021856,56.7696902783889,10.898209821034));
#75794=CARTESIAN_POINT('Ctrl Pts',(86.8116301298614,56.7651427216468,10.8535450071825));
#75795=CARTESIAN_POINT('Ctrl Pts',(86.8559990591959,56.7605951649048,10.8112162136019));
#75796=CARTESIAN_POINT('Ctrl Pts',(86.9024168423656,56.7560476081627,10.7714660227675));
#75797=CARTESIAN_POINT('Ctrl Pts',(86.927504416768,56.7535897749719,10.7499821042783));
#75798=CARTESIAN_POINT('Ctrl Pts',(86.953189941594,56.7511319417812,10.7292507026567));
#75799=CARTESIAN_POINT('Ctrl Pts',(86.9794221332777,56.7486741085904,10.7093047724383));
#75800=CARTESIAN_POINT('Ctrl Pts',(87.0284878106936,56.7440768849983,10.6719971547732));
#75801=CARTESIAN_POINT('Ctrl Pts',(87.0796806949913,56.7394796614063,10.6372781198228));
#75802=CARTESIAN_POINT('Ctrl Pts',(87.1326965997162,56.7348824378142,10.6053980786505));
#75803=CARTESIAN_POINT('Ctrl Pts',(87.1866202810107,56.7302064972431,10.572972164413));
#75804=CARTESIAN_POINT('Ctrl Pts',(87.2424296358469,56.7255305566719,10.5434837781992));
#75805=CARTESIAN_POINT('Ctrl Pts',(87.2997699472393,56.7208546161008,10.5171531232397));
#75806=CARTESIAN_POINT('Ctrl Pts',(87.3559898986006,56.7162700377284,10.4913369372933));
#75807=CARTESIAN_POINT('Ctrl Pts',(87.4136810337534,56.711685459356,10.4685564185088));
#75808=CARTESIAN_POINT('Ctrl Pts',(87.472482625749,56.7071008809836,10.4489737561716));
#75809=CARTESIAN_POINT('Ctrl Pts',(87.5312482792357,56.7025191046256,10.4294030624166));
#75810=CARTESIAN_POINT('Ctrl Pts',(87.5911225618507,56.6979373282677,10.4130265101782));
#75811=CARTESIAN_POINT('Ctrl Pts',(87.651726113159,56.6933555519097,10.399957650648));
#75812=CARTESIAN_POINT('Ctrl Pts',(87.7123148840911,56.6887748929843,10.3868919784338));
#75813=CARTESIAN_POINT('Ctrl Pts',(87.7736320732545,56.6841942340588,10.3771325047629));
#75814=CARTESIAN_POINT('Ctrl Pts',(87.8352865557474,56.6796135751334,10.3707420193054));
#75815=CARTESIAN_POINT('Ctrl Pts',(87.8991684054352,56.6748674325478,10.3641206672978));
#75816=CARTESIAN_POINT('Ctrl Pts',(87.9634118138756,56.6701212899623,10.3611165079455));
#75817=CARTESIAN_POINT('Ctrl Pts',(88.0275766938965,56.6653751473768,10.3617406157455));
#75818=CARTESIAN_POINT('Ctrl Pts',(88.0895827827364,56.6607886860804,10.3623437257908));
#75819=CARTESIAN_POINT('Ctrl Pts',(88.1515150214752,56.656202224784,10.3663347163375));
#75820=CARTESIAN_POINT('Ctrl Pts',(88.2129796301034,56.6516157634876,10.3736705212568));
#75821=CARTESIAN_POINT('Ctrl Pts',(88.2776541474084,56.6467897802576,10.3813894289792));
#75822=CARTESIAN_POINT('Ctrl Pts',(88.3418102165966,56.6419637970275,10.3928119859271));
#75823=CARTESIAN_POINT('Ctrl Pts',(88.405002285617,56.6371378137974,10.4078272000396));
#75824=CARTESIAN_POINT('Ctrl Pts',(88.4681943546375,56.6323118305674,10.4228424141521));
#75825=CARTESIAN_POINT('Ctrl Pts',(88.5304218248333,56.6274858473373,10.4414500256515));
#75826=CARTESIAN_POINT('Ctrl Pts',(88.5912618242507,56.6226598641072,10.4634797814326));
#75827=CARTESIAN_POINT('Ctrl Pts',(88.6492179064269,56.6180626405152,10.484465290121));
#75828=CARTESIAN_POINT('Ctrl Pts',(88.7061530598434,56.6134654169231,10.5086419544082));
#75829=CARTESIAN_POINT('Ctrl Pts',(88.7616919185075,56.608868193331,10.535890043465));
#75830=CARTESIAN_POINT('Ctrl Pts',(88.8181817535786,56.6041922527599,10.5636046939609));
#75831=CARTESIAN_POINT('Ctrl Pts',(88.8732264961636,56.5995163121888,10.5944968502872));
#75832=CARTESIAN_POINT('Ctrl Pts',(88.926448750812,56.5948403716176,10.6283879451546));
#75833=CARTESIAN_POINT('Ctrl Pts',(88.9786311072557,56.5902557932452,10.6616168491971));
#75834=CARTESIAN_POINT('Ctrl Pts',(89.0290611037177,56.5856712148728,10.6977282680028));
#75835=CARTESIAN_POINT('Ctrl Pts',(89.0774068236945,56.5810866365004,10.736507118493));
#75836=CARTESIAN_POINT('Ctrl Pts',(89.1257229956094,56.5765048601425,10.7752622680252));
#75837=CARTESIAN_POINT('Ctrl Pts',(89.1719570206811,56.5719230837845,10.8166812987665));
#75838=CARTESIAN_POINT('Ctrl Pts',(89.215807737519,56.5673413074265,10.8605070920099));
#75839=CARTESIAN_POINT('Ctrl Pts',(89.2596477597674,56.5627606485011,10.9043221967425));
#75840=CARTESIAN_POINT('Ctrl Pts',(89.301105267772,56.5581799895756,10.9505425390528));
#75841=CARTESIAN_POINT('Ctrl Pts',(89.3399153649386,56.5535993306502,10.9988735836697));
#75842=CARTESIAN_POINT('Ctrl Pts',(89.3801275391931,56.5488531880647,11.0489506648913));
#75843=CARTESIAN_POINT('Ctrl Pts',(89.4174969423386,56.5441070454791,11.1012934600975));
#75844=CARTESIAN_POINT('Ctrl Pts',(89.4517755677182,56.5393609028936,11.1555382495314));
#75845=CARTESIAN_POINT('Ctrl Pts',(89.4849009080898,56.5347744415972,11.2079580036344));
#75846=CARTESIAN_POINT('Ctrl Pts',(89.5151399621241,56.5301879803008,11.2621532968973));
#75847=CARTESIAN_POINT('Ctrl Pts',(89.5423153247976,56.5256015190044,11.3177699473826));
#75848=CARTESIAN_POINT('Ctrl Pts',(89.5709098851914,56.5207755357744,11.3762911045904));
#75849=CARTESIAN_POINT('Ctrl Pts',(89.596111725844,56.5159495525443,11.436385557318));
#75850=CARTESIAN_POINT('Ctrl Pts',(89.6177724266541,56.5111235693142,11.4976187858981));
#75851=CARTESIAN_POINT('Ctrl Pts',(89.6394331274642,56.5062975860842,11.5588520144781));
#75852=CARTESIAN_POINT('Ctrl Pts',(89.6575525819659,56.5014716028541,11.6212233750633));
#75853=CARTESIAN_POINT('Ctrl Pts',(89.6720444581726,56.496645619624,11.6842852588988));
#75854=CARTESIAN_POINT('Ctrl Pts',(89.6858493953253,56.492048396032,11.7443579044736));
#75855=CARTESIAN_POINT('Ctrl Pts',(89.6964196246031,56.4874511724399,11.8053037250327));
#75856=CARTESIAN_POINT('Ctrl Pts',(89.7036521363606,56.4828539488478,11.8667424258054));
#75857=CARTESIAN_POINT('Ctrl Pts',(89.7110084884024,56.4781780082767,11.9292331243382));
#75858=CARTESIAN_POINT('Ctrl Pts',(89.7149115341484,56.4735020677056,11.9922332453114));
#75859=CARTESIAN_POINT('Ctrl Pts',(89.7153065929332,56.4688261271344,12.0553288761405));
#75860=CARTESIAN_POINT('Ctrl Pts',(89.7156939327493,56.464241548762,12.117191694988));
#75861=CARTESIAN_POINT('Ctrl Pts',(89.7127091330007,56.4596569703896,12.1791457915578));
#75862=CARTESIAN_POINT('Ctrl Pts',(89.7063528584347,56.4550723920172,12.2407956549726));
#75863=CARTESIAN_POINT('Ctrl Pts',(89.7000004687129,56.4504906156592,12.3024078390647));
#75864=CARTESIAN_POINT('Ctrl Pts',(89.6902807421184,56.4459088393013,12.3637156533857));
#75865=CARTESIAN_POINT('Ctrl Pts',(89.6772463399544,56.4413270629433,12.4243266250066));
#75866=CARTESIAN_POINT('Ctrl Pts',(89.6642151167026,56.4367464040179,12.4849228144415));
#75867=CARTESIAN_POINT('Ctrl Pts',(89.6478709296617,56.4321657450924,12.5448220011071));
#75868=CARTESIAN_POINT('Ctrl Pts',(89.6283175445639,56.427585086167,12.6036418841998));
#75869=CARTESIAN_POINT('Ctrl Pts',(89.6080577620272,56.4228389435814,12.6645867300321));
#75870=CARTESIAN_POINT('Ctrl Pts',(89.5843525896718,56.4180928009959,12.7243722241343));
#75871=CARTESIAN_POINT('Ctrl Pts',(89.5573730776615,56.4133466584104,12.7825927297172));
#75872=CARTESIAN_POINT('Ctrl Pts',(89.5313012761087,56.408760197114,12.8388544392428));
#75873=CARTESIAN_POINT('Ctrl Pts',(89.5021722883785,56.4041737358176,12.8936543687552));
#75874=CARTESIAN_POINT('Ctrl Pts',(89.4701874459501,56.3995872745212,12.9466513686935));
#75875=CARTESIAN_POINT('Ctrl Pts',(89.4365322370208,56.3947612912912,13.0024160675359));
#75876=CARTESIAN_POINT('Ctrl Pts',(89.3997150622263,56.3899353080611,13.0561838242406));
#75877=CARTESIAN_POINT('Ctrl Pts',(89.3600204678588,56.385109324831,13.1075942650083));
#75878=CARTESIAN_POINT('Ctrl Pts',(89.3203258734913,56.380283341601,13.1590047057759));
#75879=CARTESIAN_POINT('Ctrl Pts',(89.2777543427136,56.3754573583709,13.2080573919401));
#75880=CARTESIAN_POINT('Ctrl Pts',(89.2326350947542,56.3706313751408,13.2544370117364));
#75881=CARTESIAN_POINT('Ctrl Pts',(89.1896545742493,56.3660341515487,13.2986181603551));
#75882=CARTESIAN_POINT('Ctrl Pts',(89.1441859794039,56.3614369279567,13.3405553714379));
#75883=CARTESIAN_POINT('Ctrl Pts',(89.096492931602,56.3568397043646,13.3799558329876));
#75884=CARTESIAN_POINT('Ctrl Pts',(89.0479832490271,56.3521637637934,13.4200309376656));
#75885=CARTESIAN_POINT('Ctrl Pts',(88.9971725208118,56.3474878232223,13.4574811567165));
#75886=CARTESIAN_POINT('Ctrl Pts',(88.9443788249558,56.3428118826512,13.4920360460816));
#75887=CARTESIAN_POINT('Ctrl Pts',(88.8926166537863,56.3382273042788,13.5259157748838));
#75888=CARTESIAN_POINT('Ctrl Pts',(88.8389487539412,56.3336427259064,13.5570120067701));
#75889=CARTESIAN_POINT('Ctrl Pts',(88.7837077630397,56.3290581475339,13.5851107755981));
#75890=CARTESIAN_POINT('Ctrl Pts',(88.7285005344698,56.324476371176,13.6131923709479));
#75891=CARTESIAN_POINT('Ctrl Pts',(88.6717225740338,56.319894594818,13.6382799055139));
#75892=CARTESIAN_POINT('Ctrl Pts',(88.6137321699741,56.3153128184601,13.6602047443407));
#75893=CARTESIAN_POINT('Ctrl Pts',(88.5557559089797,56.3107321595346,13.6821242359996));
#75894=CARTESIAN_POINT('Ctrl Pts',(88.4965682673067,56.3061515006092,13.7008823832009));
#75895=CARTESIAN_POINT('Ctrl Pts',(88.4365467063585,56.3015708416837,13.7163590022499));
#75896=CARTESIAN_POINT('Ctrl Pts',(88.3743567701286,56.2968246990982,13.732394739017));
#75897=CARTESIAN_POINT('Ctrl Pts',(88.3112720546555,56.2920785565127,13.744907099911));
#75898=CARTESIAN_POINT('Ctrl Pts',(88.2477261213912,56.2873324139272,13.753819770903));
#75899=CARTESIAN_POINT('Ctrl Pts',(88.1863181551937,56.2827459526308,13.7624325801087));
#75900=CARTESIAN_POINT('Ctrl Pts',(88.1244800473313,56.2781594913344,13.7676841148125));
#75901=CARTESIAN_POINT('Ctrl Pts',(88.0626076067181,56.273573030038,13.7695584787523));
#75902=CARTESIAN_POINT('Ctrl Pts',(87.9975039589366,56.2687470468079,13.7715307288937));
#75903=CARTESIAN_POINT('Ctrl Pts',(87.932362938148,56.2639210635778,13.7697634056245));
#75904=CARTESIAN_POINT('Ctrl Pts',(87.8676416395676,56.2590950803478,13.764300096006));
#75905=CARTESIAN_POINT('Ctrl Pts',(87.8029203409871,56.2542690971177,13.7588367863876));
#75906=CARTESIAN_POINT('Ctrl Pts',(87.7386193952144,56.2494431138876,13.749677658403));
#75907=CARTESIAN_POINT('Ctrl Pts',(87.6751822704408,56.2446171306575,13.736928271385));
#75908=CARTESIAN_POINT('Ctrl Pts',(87.614752170973,56.2400199070655,13.7247832265331));
#75909=CARTESIAN_POINT('Ctrl Pts',(87.5548577224907,56.2354226834734,13.709330788809));
#75910=CARTESIAN_POINT('Ctrl Pts',(87.4958879104644,56.2308254598813,13.6906336112534));
#75911=CARTESIAN_POINT('Ctrl Pts',(87.4359083747724,56.2261495193102,13.6716162871345));
#75912=CARTESIAN_POINT('Ctrl Pts',(87.3768859767579,56.2214735787391,13.6492420711404));
#75913=CARTESIAN_POINT('Ctrl Pts',(87.3192204473137,56.2167976381679,13.62363149881));
#75914=CARTESIAN_POINT('Ctrl Pts',(87.2626816322662,56.2122130597955,13.5985213259528));
#75915=CARTESIAN_POINT('Ctrl Pts',(87.2074476270305,56.2076284814231,13.570300344805));
#75916=CARTESIAN_POINT('Ctrl Pts',(87.153878611326,56.2030439030507,13.5391319563018));
#75917=CARTESIAN_POINT('Ctrl Pts',(87.1003423360712,56.1984621266927,13.5079826173749));
#75918=CARTESIAN_POINT('Ctrl Pts',(87.0484694716465,56.1938803503348,13.4738896984878));
#75919=CARTESIAN_POINT('Ctrl Pts',(86.9985960269477,56.1892985739768,13.437062737787));
#75920=CARTESIAN_POINT('Ctrl Pts',(86.948734745699,56.1847179150514,13.4002447586775));
#75921=CARTESIAN_POINT('Ctrl Pts',(86.9008723254761,56.1801372561259,13.3606943636905));
#75922=CARTESIAN_POINT('Ctrl Pts',(86.8553144697435,56.1755565972005,13.3186634786549));
#75923=CARTESIAN_POINT('Ctrl Pts',(86.8081107633081,56.170810454615,13.2751141603971));
#75924=CARTESIAN_POINT('Ctrl Pts',(86.7633817923823,56.1660643120295,13.2289020444386));
#75925=CARTESIAN_POINT('Ctrl Pts',(86.7214268331923,56.161318169444,13.1803499822989));
#75926=CARTESIAN_POINT('Ctrl Pts',(86.6808834249297,56.1567317081476,13.1334314268927));
#75927=CARTESIAN_POINT('Ctrl Pts',(86.6429305862306,56.1521452468512,13.0843283492353));
#75928=CARTESIAN_POINT('Ctrl Pts',(86.6077963581465,56.1475587855548,13.0333646546619));
#75929=CARTESIAN_POINT('Ctrl Pts',(86.5708272910209,56.1427328023247,12.9797394478937));
#75930=CARTESIAN_POINT('Ctrl Pts',(86.536979647615,56.1379068190946,12.9240545032787));
#75931=CARTESIAN_POINT('Ctrl Pts',(86.506464737395,56.1330808358645,12.8667174777524));
#75932=CARTESIAN_POINT('Ctrl Pts',(86.4759498271751,56.1282548526345,12.8093804522262));
#75933=CARTESIAN_POINT('Ctrl Pts',(86.4487678510513,56.1234288694044,12.7503919666829));
#75934=CARTESIAN_POINT('Ctrl Pts',(86.425070662992,56.1186028861743,12.6901818433898));
#75935=CARTESIAN_POINT('Ctrl Pts',(86.3995423106974,56.1134039824159,12.625319074217));
#75936=CARTESIAN_POINT('Ctrl Pts',(86.3779687741055,56.1082050786575,12.5588164507142));
#75937=CARTESIAN_POINT('Ctrl Pts',(86.360535813958,56.1030061748991,12.4911385729297));
#75938=CARTESIAN_POINT('Ctrl Pts',(86.3427800146496,56.0977109931871,12.4222073756234));
#75939=CARTESIAN_POINT('Ctrl Pts',(86.3293199176743,56.0924158114752,12.3520571510168));
#75940=CARTESIAN_POINT('Ctrl Pts',(86.320301082368,56.0871206297632,12.2812022432926));
#75941=CARTESIAN_POINT('Ctrl Pts',(86.3112822470618,56.0818254480512,12.2103473355684));
#75942=CARTESIAN_POINT('Ctrl Pts',(86.3067048800023,56.0765302663393,12.13878800421));
#75943=CARTESIAN_POINT('Ctrl Pts',(86.3066603287391,56.0712350846273,12.0670585679921));
#75944=CARTESIAN_POINT('',(86.3066605389047,55.2774850845187,12.0646446574837));
#75945=CARTESIAN_POINT('Ctrl Pts',(86.3066603287386,56.0712350845702,12.0670585672184));
#75946=CARTESIAN_POINT('Ctrl Pts',(86.3066214924812,56.0666191618022,12.0045304887141));
#75947=CARTESIAN_POINT('Ctrl Pts',(86.310027997416,56.0620032390342,11.9419890370945));
#75948=CARTESIAN_POINT('Ctrl Pts',(86.3168577898452,56.0573873162662,11.8798360739244));
#75949=CARTESIAN_POINT('Ctrl Pts',(86.3236886814535,56.0527706506168,11.8176731079272));
#75950=CARTESIAN_POINT('Ctrl Pts',(86.3339438978837,56.0481539849675,11.7558992492126));
#75951=CARTESIAN_POINT('Ctrl Pts',(86.3475496637027,56.0435373193181,11.694909964736));
#75952=CARTESIAN_POINT('Ctrl Pts',(86.3611730542256,56.0389146733097,11.6338416756595));
#75953=CARTESIAN_POINT('Ctrl Pts',(86.3781555491344,56.0342920273012,11.573560476663));
#75954=CARTESIAN_POINT('Ctrl Pts',(86.3983727018363,56.0296693812928,11.5144494285949));
#75955=CARTESIAN_POINT('Ctrl Pts',(86.4186037073804,56.025043567836,11.4552978774931));
#75956=CARTESIAN_POINT('Ctrl Pts',(86.4420735959647,56.0204177543793,11.3973185353219));
#75957=CARTESIAN_POINT('Ctrl Pts',(86.4686098104151,56.0157919409226,11.3408742600954));
#75958=CARTESIAN_POINT('Ctrl Pts',(86.4951999452586,56.0111567280212,11.2843152926427));
#75959=CARTESIAN_POINT('Ctrl Pts',(86.524868612324,56.0065215151197,11.2292980601706));
#75960=CARTESIAN_POINT('Ctrl Pts',(86.557397738338,56.0018863022183,11.1761599579187));
#75961=CARTESIAN_POINT('Ctrl Pts',(86.5791475318828,55.9987870820426,11.1406304834152));
#75962=CARTESIAN_POINT('Ctrl Pts',(86.6021752031633,55.9956878618668,11.1059405079902));
#75963=CARTESIAN_POINT('Ctrl Pts',(86.6264055081682,55.9925886416911,11.0721826481747));
#75964=CARTESIAN_POINT('Ctrl Pts',(86.6623474946987,55.987991418099,11.0221079775279));
#75965=CARTESIAN_POINT('Ctrl Pts',(86.7010832335385,55.9833941945069,10.9738828250952));
#75966=CARTESIAN_POINT('Ctrl Pts',(86.7423955159203,55.9787969709148,10.9278359087667));
#75967=CARTESIAN_POINT('Ctrl Pts',(86.7844151770062,55.9741210303437,10.8810005439159));
#75968=CARTESIAN_POINT('Ctrl Pts',(86.8291002149384,55.9694450897726,10.8364191981116));
#75969=CARTESIAN_POINT('Ctrl Pts',(86.8761762461845,55.9647691492015,10.7944065573556));
#75970=CARTESIAN_POINT('Ctrl Pts',(86.9223324689652,55.9601845708291,10.7532147925657));
#75971=CARTESIAN_POINT('Ctrl Pts',(86.9707866931789,55.9555999924566,10.7144926120077));
#75972=CARTESIAN_POINT('Ctrl Pts',(87.0212417489732,55.9510154140842,10.6785010125682));
#75973=CARTESIAN_POINT('Ctrl Pts',(87.0716659675162,55.9464336377263,10.6425314105673));
#75974=CARTESIAN_POINT('Ctrl Pts',(87.1240881793043,55.9418518613683,10.6092893755345));
#75975=CARTESIAN_POINT('Ctrl Pts',(87.1781791156971,55.9372700850103,10.5789948855942));
#75976=CARTESIAN_POINT('Ctrl Pts',(87.2322568600514,55.9326894260849,10.5487077840652));
#75977=CARTESIAN_POINT('Ctrl Pts',(87.28800207716,55.9281087671594,10.521367049204));
#75978=CARTESIAN_POINT('Ctrl Pts',(87.3450593418189,55.923528108234,10.4971475928624));
#75979=CARTESIAN_POINT('Ctrl Pts',(87.4041778917956,55.9187819656485,10.472053169765));
#75980=CARTESIAN_POINT('Ctrl Pts',(87.4647045938634,55.9140358230629,10.4503101516155));
#75981=CARTESIAN_POINT('Ctrl Pts',(87.526222029381,55.9092896804774,10.4320583992068));
#75982=CARTESIAN_POINT('Ctrl Pts',(87.5856697454938,55.904703219181,10.4144207167088));
#75983=CARTESIAN_POINT('Ctrl Pts',(87.6460420538035,55.9001167578846,10.4000431442394));
#75984=CARTESIAN_POINT('Ctrl Pts',(87.70694989617,55.8955302965882,10.3890001878471));
#75985=CARTESIAN_POINT('Ctrl Pts',(87.7710385708246,55.8907043133582,10.3773805275216));
#75986=CARTESIAN_POINT('Ctrl Pts',(87.8357196106168,55.8858783301281,10.3694534150399));
#75987=CARTESIAN_POINT('Ctrl Pts',(87.9005345162743,55.881052346898,10.3652436351713));
#75988=CARTESIAN_POINT('Ctrl Pts',(87.9653494219317,55.876226363668,10.3610338553027));
#75989=CARTESIAN_POINT('Ctrl Pts',(88.0302975448992,55.8714003804379,10.3605413355845));
#75990=CARTESIAN_POINT('Ctrl Pts',(88.0949246575862,55.8665743972078,10.3637275519327));
#75991=CARTESIAN_POINT('Ctrl Pts',(88.1564883375595,55.8619771736158,10.3667627363225));
#75992=CARTESIAN_POINT('Ctrl Pts',(88.2180135259219,55.8573799500237,10.373148187565));
#75993=CARTESIAN_POINT('Ctrl Pts',(88.2791062460481,55.8527827264316,10.3828797201537));
#75994=CARTESIAN_POINT('Ctrl Pts',(88.3412450398043,55.8481067858605,10.3927778830642));
#75995=CARTESIAN_POINT('Ctrl Pts',(88.4029358815445,55.8434308452894,10.4061378626346));
#75996=CARTESIAN_POINT('Ctrl Pts',(88.4637655716076,55.8387549047182,10.4228998287485));
#75997=CARTESIAN_POINT('Ctrl Pts',(88.523406723419,55.8341703263458,10.4393342864058));
#75998=CARTESIAN_POINT('Ctrl Pts',(88.5822195583685,55.8295857479734,10.4590388431506));
#75999=CARTESIAN_POINT('Ctrl Pts',(88.639823622886,55.825001169601,10.4819054046868));
#76000=CARTESIAN_POINT('Ctrl Pts',(88.6973924808026,55.8204193932431,10.5047579905788));
#76001=CARTESIAN_POINT('Ctrl Pts',(88.753753561029,55.8158376168851,10.530768561845));
#76002=CARTESIAN_POINT('Ctrl Pts',(88.8085434603824,55.8112558405271,10.5597798087924));
#76003=CARTESIAN_POINT('Ctrl Pts',(88.8633199972296,55.8066751816017,10.588783980294));
#76004=CARTESIAN_POINT('Ctrl Pts',(88.9165256642212,55.8020945226762,10.6207871365946));
#76005=CARTESIAN_POINT('Ctrl Pts',(88.9678207320166,55.7975138637508,10.6555855494277));
#76006=CARTESIAN_POINT('Ctrl Pts',(89.0209689165142,55.7927677211653,10.6916411108095));
#76007=CARTESIAN_POINT('Ctrl Pts',(89.0720652947151,55.7880215785798,10.7306974884732));
#76008=CARTESIAN_POINT('Ctrl Pts',(89.1207659592515,55.7832754359943,10.7724798605021));
#76009=CARTESIAN_POINT('Ctrl Pts',(89.1678281174105,55.7786889746979,10.8128564882012));
#76010=CARTESIAN_POINT('Ctrl Pts',(89.2126528857788,55.7741025134015,10.8557781650263));
#76011=CARTESIAN_POINT('Ctrl Pts',(89.2549666455938,55.7695160521051,10.9009584469857));
#76012=CARTESIAN_POINT('Ctrl Pts',(89.2994901860911,55.764690068875,10.9484982099916));
#76013=CARTESIAN_POINT('Ctrl Pts',(89.3412328370882,55.7598640856449,10.9985384648737));
#76014=CARTESIAN_POINT('Ctrl Pts',(89.3799250869373,55.7550381024149,11.0507074599143));
#76015=CARTESIAN_POINT('Ctrl Pts',(89.4186173367865,55.7502121191848,11.102876454955));
#76016=CARTESIAN_POINT('Ctrl Pts',(89.4542588945896,55.7453861359547,11.1571736059858));
#76017=CARTESIAN_POINT('Ctrl Pts',(89.4866357527621,55.7405601527246,11.2131964113759));
#76018=CARTESIAN_POINT('Ctrl Pts',(89.5174778939656,55.7359629291326,11.2665636425399));
#76019=CARTESIAN_POINT('Ctrl Pts',(89.5454845272557,55.7313657055405,11.3217157166837));
#76020=CARTESIAN_POINT('Ctrl Pts',(89.570445476531,55.7267684819484,11.3783193754897));
#76021=CARTESIAN_POINT('Ctrl Pts',(89.5958338251882,55.7220925413773,11.435892242979));
#76022=CARTESIAN_POINT('Ctrl Pts',(89.61807085976,55.7174166008062,11.4949664615704));
#76023=CARTESIAN_POINT('Ctrl Pts',(89.6369827258091,55.712740660235,11.5551624416996));
#76024=CARTESIAN_POINT('Ctrl Pts',(89.6555250769686,55.7081560818626,11.6141822654994));
#76025=CARTESIAN_POINT('Ctrl Pts',(89.6708708706124,55.7035715034902,11.6742799004675));
#76026=CARTESIAN_POINT('Ctrl Pts',(89.6829045615013,55.6989869251178,11.7350770892925));
#76027=CARTESIAN_POINT('Ctrl Pts',(89.6949308976079,55.6944051487598,11.7958371199345));
#76028=CARTESIAN_POINT('Ctrl Pts',(89.703649046219,55.6898233724019,11.8572953583299));
#76029=CARTESIAN_POINT('Ctrl Pts',(89.7089940571011,55.6852415960439,11.9190611771885));
#76030=CARTESIAN_POINT('Ctrl Pts',(89.7143377644083,55.6806609371185,11.9808119322097));
#76031=CARTESIAN_POINT('Ctrl Pts',(89.716309923228,55.676080278193,12.0428696118538));
#76032=CARTESIAN_POINT('Ctrl Pts',(89.7148974212158,55.6714996192676,12.1048383003497));
#76033=CARTESIAN_POINT('Ctrl Pts',(89.7134338903,55.6667534766821,12.1690457072371));
#76034=CARTESIAN_POINT('Ctrl Pts',(89.7083364128982,55.6620073340966,12.2331569872555));
#76035=CARTESIAN_POINT('Ctrl Pts',(89.6996493377902,55.657261191511,12.2967341534767));
#76036=CARTESIAN_POINT('Ctrl Pts',(89.6912545344222,55.6526747302146,12.3581723018159));
#76037=CARTESIAN_POINT('Ctrl Pts',(89.6795080239475,55.6480882689183,12.4191112031222));
#76038=CARTESIAN_POINT('Ctrl Pts',(89.6645020435493,55.6435018076219,12.4791656176138));
#76039=CARTESIAN_POINT('Ctrl Pts',(89.6487123954803,55.6386758243918,12.5423562952405));
#76040=CARTESIAN_POINT('Ctrl Pts',(89.6293136802233,55.6338498411617,12.6045669524247));
#76041=CARTESIAN_POINT('Ctrl Pts',(89.6064720314822,55.6290238579316,12.6653695290536));
#76042=CARTESIAN_POINT('Ctrl Pts',(89.5836303827412,55.6241978747016,12.7261721056825));
#76043=CARTESIAN_POINT('Ctrl Pts',(89.5573461335055,55.6193718914715,12.7855660405143));
#76044=CARTESIAN_POINT('Ctrl Pts',(89.5278413564675,55.6145459082414,12.8431532248596));
#76045=CARTESIAN_POINT('Ctrl Pts',(89.4997351549721,55.6099486846493,12.8980106808127));
#76046=CARTESIAN_POINT('Ctrl Pts',(89.4685914931177,55.6053514610573,12.9514540631619));
#76047=CARTESIAN_POINT('Ctrl Pts',(89.4345763490148,55.6007542374652,13.0031260396156));
#76048=CARTESIAN_POINT('Ctrl Pts',(89.3999787730742,55.5960782968941,13.0556827809292));
#76049=CARTESIAN_POINT('Ctrl Pts',(89.3624106114259,55.5914023563229,13.1064063675443));
#76050=CARTESIAN_POINT('Ctrl Pts',(89.3220964668672,55.5867264157518,13.1549448517571));
#76051=CARTESIAN_POINT('Ctrl Pts',(89.2825700117221,55.5821418373794,13.20253495295));
#76052=CARTESIAN_POINT('Ctrl Pts',(89.2404042557537,55.577557259007,13.2480241619443));
#76053=CARTESIAN_POINT('Ctrl Pts',(89.1958543093425,55.5729726806346,13.2911102404407));
#76054=CARTESIAN_POINT('Ctrl Pts',(89.1513315910827,55.5683909042766,13.3341699854762));
#76055=CARTESIAN_POINT('Ctrl Pts',(89.104427936902,55.5638091279187,13.3748291591812));
#76056=CARTESIAN_POINT('Ctrl Pts',(89.0554362921307,55.5592273515607,13.4128213197304));
#76057=CARTESIAN_POINT('Ctrl Pts',(89.0064565957507,55.5546466926353,13.4508042145119));
#76058=CARTESIAN_POINT('Ctrl Pts',(88.9553903217678,55.5500660337098,13.4861210755661));
#76059=CARTESIAN_POINT('Ctrl Pts',(88.902562975284,55.5454853747844,13.5185461427103));
#76060=CARTESIAN_POINT('Ctrl Pts',(88.8478271560696,55.5407392321988,13.5521426174787));
#76061=CARTESIAN_POINT('Ctrl Pts',(88.7912010469939,55.5359930896133,13.5826339977754));
#76062=CARTESIAN_POINT('Ctrl Pts',(88.7330766648711,55.5312469470278,13.6098199783811));
#76063=CARTESIAN_POINT('Ctrl Pts',(88.6769078447862,55.5266604857314,13.6360913020099));
#76064=CARTESIAN_POINT('Ctrl Pts',(88.6193404909143,55.522074024435,13.6592759945665));
#76065=CARTESIAN_POINT('Ctrl Pts',(88.5607482806862,55.5174875631386,13.6792425928801));
#76066=CARTESIAN_POINT('Ctrl Pts',(88.4990961690254,55.5126615799086,13.7002519206376));
#76067=CARTESIAN_POINT('Ctrl Pts',(88.4363098397077,55.5078355966785,13.7176976327675));
#76068=CARTESIAN_POINT('Ctrl Pts',(88.3728390258118,55.5030096134484,13.7314871224358));
#76069=CARTESIAN_POINT('Ctrl Pts',(88.3093682119159,55.4981836302183,13.7452766121042));
#76070=CARTESIAN_POINT('Ctrl Pts',(88.245213565566,55.4933576469883,13.7554098546456));
#76071=CARTESIAN_POINT('Ctrl Pts',(88.180829998254,55.4885316637582,13.7618574843698));
#76072=CARTESIAN_POINT('Ctrl Pts',(88.1194983191995,55.4839344401661,13.7679994857129));
#76073=CARTESIAN_POINT('Ctrl Pts',(88.0577071185754,55.479337216574,13.770822660529));
#76074=CARTESIAN_POINT('Ctrl Pts',(87.9958466251266,55.474739992982,13.7702726339497));
#76075=CARTESIAN_POINT('Ctrl Pts',(87.9329269116793,55.4700640524108,13.7697131894185));
#76076=CARTESIAN_POINT('Ctrl Pts',(87.8699360282904,55.4653881118397,13.7656637921032));
#76077=CARTESIAN_POINT('Ctrl Pts',(87.8072914779564,55.4607121712686,13.7581222395698));
#76078=CARTESIAN_POINT('Ctrl Pts',(87.745870926039,55.4561275928962,13.7507280398119));
#76079=CARTESIAN_POINT('Ctrl Pts',(87.6847838246336,55.4515430145238,13.7399769862261));
#76080=CARTESIAN_POINT('Ctrl Pts',(87.6244224620891,55.4469584361513,13.7259194687643));
#76081=CARTESIAN_POINT('Ctrl Pts',(87.564097991358,55.4423766597934,13.7118705430123));
#76082=CARTESIAN_POINT('Ctrl Pts',(87.5044988747256,55.4377948834354,13.6945192756662));
#76083=CARTESIAN_POINT('Ctrl Pts',(87.4460078487948,55.4332131070774,13.6739672585835));
#76084=CARTESIAN_POINT('Ctrl Pts',(87.3875310880244,55.428632448152,13.6534202538564));
#76085=CARTESIAN_POINT('Ctrl Pts',(87.3301623615197,55.4240517892265,13.6296742177143));
#76086=CARTESIAN_POINT('Ctrl Pts',(87.2742678887547,55.4194711303011,13.6028801618409));
#76087=CARTESIAN_POINT('Ctrl Pts',(87.2163541383964,55.4147249877156,13.5751181276687));
#76088=CARTESIAN_POINT('Ctrl Pts',(87.1600237527588,55.4099788451301,13.5440838215642));
#76089=CARTESIAN_POINT('Ctrl Pts',(87.1056576419326,55.4052327025445,13.5099979398493));
#76090=CARTESIAN_POINT('Ctrl Pts',(87.0531206482273,55.4006462412482,13.4770588583906));
#76091=CARTESIAN_POINT('Ctrl Pts',(87.0024182356365,55.3960597799518,13.4412706542136));
#76092=CARTESIAN_POINT('Ctrl Pts',(86.9538635313293,55.3914733186554,13.4028759561778));
#76093=CARTESIAN_POINT('Ctrl Pts',(86.9027731211883,55.3866473354253,13.362476145328));
#76094=CARTESIAN_POINT('Ctrl Pts',(86.8540613817271,55.3818213521952,13.3191905535037));
#76095=CARTESIAN_POINT('Ctrl Pts',(86.8080500485729,55.3769953689651,13.2733467811534));
#76096=CARTESIAN_POINT('Ctrl Pts',(86.7620387154187,55.3721693857351,13.2275030088032));
#76097=CARTESIAN_POINT('Ctrl Pts',(86.7187281630047,55.367343402505,13.1791015904119));
#76098=CARTESIAN_POINT('Ctrl Pts',(86.6783898054996,55.3625174192749,13.1285087788407));
#76099=CARTESIAN_POINT('Ctrl Pts',(86.6400443941757,55.357929867291,13.0804155422857));
#76100=CARTESIAN_POINT('Ctrl Pts',(86.6042233165221,55.3533423153071,13.0301403208289));
#76101=CARTESIAN_POINT('Ctrl Pts',(86.5711844148976,55.3487547633232,12.9779791206471));
#76102=CARTESIAN_POINT('Ctrl Pts',(86.5381952169409,55.3441741128448,12.9258963916868));
#76103=CARTESIAN_POINT('Ctrl Pts',(86.5079801689771,55.3395934623664,12.87193373564));
#76104=CARTESIAN_POINT('Ctrl Pts',(86.4807564203913,55.3350128118879,12.816419497792));
#76105=CARTESIAN_POINT('Ctrl Pts',(86.4522648267378,55.3302188346114,12.7583198903199));
#76106=CARTESIAN_POINT('Ctrl Pts',(86.4270503576331,55.325424857335,12.6985210776844));
#76107=CARTESIAN_POINT('Ctrl Pts',(86.4053099444063,55.3206308800585,12.6374317815517));
#76108=CARTESIAN_POINT('Ctrl Pts',(86.3845752197675,55.316058667115,12.5791684118324));
#76109=CARTESIAN_POINT('Ctrl Pts',(86.3670004043682,55.3114864541715,12.5197318589521));
#76110=CARTESIAN_POINT('Ctrl Pts',(86.3527074033412,55.3069142412281,12.4594977756818));
#76111=CARTESIAN_POINT('Ctrl Pts',(86.3384195452644,55.3023436734719,12.3992853660188));
#76112=CARTESIAN_POINT('Ctrl Pts',(86.3274112711726,55.2977731057157,12.3382764932761));
#76113=CARTESIAN_POINT('Ctrl Pts',(86.3197539981865,55.2932025379595,12.2768596617421));
#76114=CARTESIAN_POINT('Ctrl Pts',(86.3120950388772,55.2886309636499,12.2154293046841));
#76115=CARTESIAN_POINT('Ctrl Pts',(86.3077886127174,55.2840593893402,12.1535913168771));
#76116=CARTESIAN_POINT('Ctrl Pts',(86.3068543848883,55.2794878150306,12.0917402038738));
#76117=CARTESIAN_POINT('Ctrl Pts',(86.306717961678,55.2788202382105,12.0827082235222));
#76118=CARTESIAN_POINT('Ctrl Pts',(86.3066533569379,55.2781526613903,12.0736759654379));
#76119=CARTESIAN_POINT('Ctrl Pts',(86.3066605389041,55.2774850845702,12.0646446581799));
#76120=CARTESIAN_POINT('',(86.3066600222213,54.4837350846202,12.065724781343));
#76121=CARTESIAN_POINT('Ctrl Pts',(86.3066605389047,55.2774850845187,12.0646446574837));
#76122=CARTESIAN_POINT('Ctrl Pts',(86.3067183698751,55.272109593413,11.9919223723883));
#76123=CARTESIAN_POINT('Ctrl Pts',(86.3114346070278,55.2667341023073,11.9193961867115));
#76124=CARTESIAN_POINT('Ctrl Pts',(86.3207108495257,55.2613586112016,11.8476026021471));
#76125=CARTESIAN_POINT('Ctrl Pts',(86.3300933787503,55.2559215279853,11.7749864102502));
#76126=CARTESIAN_POINT('Ctrl Pts',(86.344140905695,55.2504844447691,11.7031198126283));
#76127=CARTESIAN_POINT('Ctrl Pts',(86.362702441516,55.2450473615528,11.6325372054077));
#76128=CARTESIAN_POINT('Ctrl Pts',(86.3724253770384,55.2421992992991,11.5955645030609));
#76129=CARTESIAN_POINT('Ctrl Pts',(86.3833861065539,55.2393512370455,11.5589437609058));
#76130=CARTESIAN_POINT('Ctrl Pts',(86.3955577594668,55.2365031747918,11.5227494103998));
#76131=CARTESIAN_POINT('Ctrl Pts',(86.4152047351794,55.2319059511997,11.4643259957317));
#76132=CARTESIAN_POINT('Ctrl Pts',(86.4380655035453,55.2273087276076,11.4068498436307));
#76133=CARTESIAN_POINT('Ctrl Pts',(86.464028998772,55.2227115040156,11.3506989745851));
#76134=CARTESIAN_POINT('Ctrl Pts',(86.4904370596955,55.2180355634444,11.2935866498493));
#76135=CARTESIAN_POINT('Ctrl Pts',(86.5200550228199,55.2133596228733,11.2378459531449));
#76136=CARTESIAN_POINT('Ctrl Pts',(86.5527130481342,55.2086836823022,11.1838582871114));
#76137=CARTESIAN_POINT('Ctrl Pts',(86.5847329753049,55.2040991039298,11.1309254744913));
#76138=CARTESIAN_POINT('Ctrl Pts',(86.6196749587524,55.1995145255574,11.0796782608688));
#76139=CARTESIAN_POINT('Ctrl Pts',(86.6573316063267,55.194929947185,11.0304534218251));
#76140=CARTESIAN_POINT('Ctrl Pts',(86.6949652388138,55.190348170827,10.9812586681456));
#76141=CARTESIAN_POINT('Ctrl Pts',(86.73530993691,55.185766394469,10.9340842416265));
#76142=CARTESIAN_POINT('Ctrl Pts',(86.7781155765936,55.1811846181111,10.8892371376858));
#76143=CARTESIAN_POINT('Ctrl Pts',(86.8209107765679,55.1766039591856,10.8444009713395));
#76144=CARTESIAN_POINT('Ctrl Pts',(86.8661653753469,55.1720233002602,10.8018913688645));
#76145=CARTESIAN_POINT('Ctrl Pts',(86.9135910081573,55.1674426413347,10.7619799310506));
#76146=CARTESIAN_POINT('Ctrl Pts',(86.9627299681169,55.1626964987492,10.7206266284493));
#76147=CARTESIAN_POINT('Ctrl Pts',(87.0141994260388,55.1579503561637,10.6820632338545));
#76148=CARTESIAN_POINT('Ctrl Pts',(87.0676414624996,55.1532042135781,10.6465460538203));
#76149=CARTESIAN_POINT('Ctrl Pts',(87.1192854718,55.1486177522818,10.6122238292667));
#76150=CARTESIAN_POINT('Ctrl Pts',(87.1727709347492,55.1440312909854,10.5807462903879));
#76151=CARTESIAN_POINT('Ctrl Pts',(87.2277478433918,55.139444829689,10.5522989414126));
#76152=CARTESIAN_POINT('Ctrl Pts',(87.2855958490775,55.1346188464589,10.5223659668984));
#76153=CARTESIAN_POINT('Ctrl Pts',(87.3450947661675,55.1297928632288,10.4957886290704));
#76154=CARTESIAN_POINT('Ctrl Pts',(87.4058136035802,55.1249668799987,10.4727253026586));
#76155=CARTESIAN_POINT('Ctrl Pts',(87.4665324409929,55.1201408967687,10.4496619762467));
#76156=CARTESIAN_POINT('Ctrl Pts',(87.5284705574999,55.1153149135386,10.4301127824971));
#76157=CARTESIAN_POINT('Ctrl Pts',(87.5911824483766,55.1104889303085,10.4141743254965));
#76158=CARTESIAN_POINT('Ctrl Pts',(87.6509216912412,55.1058917067164,10.3989913778875));
#76159=CARTESIAN_POINT('Ctrl Pts',(87.7116082759286,55.1012944831244,10.3870221995701));
#76160=CARTESIAN_POINT('Ctrl Pts',(87.7728643774751,55.0966972595323,10.378378519666));
#76161=CARTESIAN_POINT('Ctrl Pts',(87.835169350186,55.0920213189612,10.3695868364386));
#76162=CARTESIAN_POINT('Ctrl Pts',(87.8980630361323,55.08734537839,10.3642358293543));
#76163=CARTESIAN_POINT('Ctrl Pts',(87.9611328898701,55.0826694378189,10.3623896845442));
#76164=CARTESIAN_POINT('Ctrl Pts',(88.0229704352794,55.0780848594465,10.3605796111612));
#76165=CARTESIAN_POINT('Ctrl Pts',(88.0849767929952,55.0735002810741,10.3621386859302));
#76166=CARTESIAN_POINT('Ctrl Pts',(88.1467565414764,55.0689157027017,10.3670753409741));
#76167=CARTESIAN_POINT('Ctrl Pts',(88.2084985312513,55.0643339263437,10.3720089788203));
#76168=CARTESIAN_POINT('Ctrl Pts',(88.2700136800395,55.0597521499858,10.3803160632334));
#76169=CARTESIAN_POINT('Ctrl Pts',(88.3309084075311,55.0551703736278,10.3919529736621));
#76170=CARTESIAN_POINT('Ctrl Pts',(88.3917882836326,55.0505897147024,10.4035870460076));
#76171=CARTESIAN_POINT('Ctrl Pts',(88.4520475390398,55.0460090557769,10.4185492367228));
#76172=CARTESIAN_POINT('Ctrl Pts',(88.5113015874829,55.0414283968515,10.4367446003889));
#76173=CARTESIAN_POINT('Ctrl Pts',(88.572696283586,55.0366822542659,10.4555973007885));
#76174=CARTESIAN_POINT('Ctrl Pts',(88.6330111781199,55.0319361116804,10.4779211445169));
#76175=CARTESIAN_POINT('Ctrl Pts',(88.6918368074698,55.0271899690949,10.5035544562468));
#76176=CARTESIAN_POINT('Ctrl Pts',(88.7486832817145,55.0226035077985,10.5283253496679));
#76177=CARTESIAN_POINT('Ctrl Pts',(88.8041386774804,55.0180170465021,10.556186241276));
#76178=CARTESIAN_POINT('Ctrl Pts',(88.8578573048559,55.0134305852057,10.5869436992419));
#76179=CARTESIAN_POINT('Ctrl Pts',(88.9143813171833,55.0086046019757,10.6193074251627));
#76180=CARTESIAN_POINT('Ctrl Pts',(88.9689816403924,55.0037786187456,10.6548782098936));
#76181=CARTESIAN_POINT('Ctrl Pts',(89.02129145149,54.9989526355155,10.6933798709598));
#76182=CARTESIAN_POINT('Ctrl Pts',(89.0736012625875,54.9941266522855,10.731881532026));
#76183=CARTESIAN_POINT('Ctrl Pts',(89.1236201119107,54.9893006690554,10.7733135964818));
#76184=CARTESIAN_POINT('Ctrl Pts',(89.1710251991094,54.9844746858253,10.8173541843136));
#76185=CARTESIAN_POINT('Ctrl Pts',(89.2161832062687,54.9798774622332,10.8593071749762));
#76186=CARTESIAN_POINT('Ctrl Pts',(89.2591550948405,54.9752802386412,10.9037991920487));
#76187=CARTESIAN_POINT('Ctrl Pts',(89.2996420670314,54.9706830150491,10.9505734185178));
#76188=CARTESIAN_POINT('Ctrl Pts',(89.3408222863697,54.966007074478,10.9981485470381));
#76189=CARTESIAN_POINT('Ctrl Pts',(89.3794312381686,54.9613311339068,11.0480844844952));
#76190=CARTESIAN_POINT('Ctrl Pts',(89.415191234162,54.9566551933357,11.1000694572058));
#76191=CARTESIAN_POINT('Ctrl Pts',(89.4502525232727,54.9520706149633,11.1510387066979));
#76192=CARTESIAN_POINT('Ctrl Pts',(89.4825748832792,54.9474860365909,11.2039772007729));
#76193=CARTESIAN_POINT('Ctrl Pts',(89.5119367540217,54.9429014582185,11.2585573109956));
#76194=CARTESIAN_POINT('Ctrl Pts',(89.5412806793003,54.9383196818605,11.3131040628055));
#76195=CARTESIAN_POINT('Ctrl Pts',(89.5676674624285,54.9337379055025,11.3692899939451));
#76196=CARTESIAN_POINT('Ctrl Pts',(89.5909202724816,54.9291561291446,11.4267607895306));
#76197=CARTESIAN_POINT('Ctrl Pts',(89.6141674114928,54.9245754702191,11.4842175687761));
#76198=CARTESIAN_POINT('Ctrl Pts',(89.6342819039056,54.9199948112937,11.5429581187242));
#76199=CARTESIAN_POINT('Ctrl Pts',(89.651134916259,54.9154141523682,11.60260784203));
#76200=CARTESIAN_POINT('Ctrl Pts',(89.668596770749,54.9106680097827,11.6644125073856));
#76201=CARTESIAN_POINT('Ctrl Pts',(89.6825567612058,54.9059218671972,11.7271927524304));
#76202=CARTESIAN_POINT('Ctrl Pts',(89.6929286219364,54.9011757246117,11.7905168856154));
#76203=CARTESIAN_POINT('Ctrl Pts',(89.7029515272654,54.8965892633153,11.8517105140722));
#76204=CARTESIAN_POINT('Ctrl Pts',(89.7096239404532,54.8920028020189,11.913411479243));
#76205=CARTESIAN_POINT('Ctrl Pts',(89.7129208658942,54.8874163407225,11.9752244425295));
#76206=CARTESIAN_POINT('Ctrl Pts',(89.7163899689478,54.8825903574924,12.0402655068587));
#76207=CARTESIAN_POINT('Ctrl Pts',(89.7161213474005,54.8777643742623,12.1054299439649));
#76208=CARTESIAN_POINT('Ctrl Pts',(89.7121480636584,54.8729383910322,12.170259777053));
#76209=CARTESIAN_POINT('Ctrl Pts',(89.7081747799164,54.8681124078022,12.2350896101411));
#76210=CARTESIAN_POINT('Ctrl Pts',(89.7004969874147,54.8632864245721,12.2995842049145));
#76211=CARTESIAN_POINT('Ctrl Pts',(89.6892100178568,54.858460441342,12.3632977826439));
#76212=CARTESIAN_POINT('Ctrl Pts',(89.6784580694433,54.8538632177499,12.4239912307372));
#76213=CARTESIAN_POINT('Ctrl Pts',(89.6643872831714,54.8492659941579,12.4842252391071));
#76214=CARTESIAN_POINT('Ctrl Pts',(89.6470513488977,54.8446687705658,12.543609484171));
#76215=CARTESIAN_POINT('Ctrl Pts',(89.6294185762502,54.8399928299947,12.6040105491222));
#76216=CARTESIAN_POINT('Ctrl Pts',(89.6084077857015,54.8353168894235,12.6635319376246));
#76217=CARTESIAN_POINT('Ctrl Pts',(89.5841302871514,54.8306409488524,12.7217712522267));
#76218=CARTESIAN_POINT('Ctrl Pts',(89.5603271414321,54.82605637048,12.778872641367));
#76219=CARTESIAN_POINT('Ctrl Pts',(89.5333839998898,54.8214717921076,12.8347411140072));
#76220=CARTESIAN_POINT('Ctrl Pts',(89.5034559361524,54.8168872137352,12.8890128275083));
#76221=CARTESIAN_POINT('Ctrl Pts',(89.4735461639264,54.8123054373772,12.9432513710835));
#76222=CARTESIAN_POINT('Ctrl Pts',(89.440655332198,54.8077236610193,12.9958946457735));
#76223=CARTESIAN_POINT('Ctrl Pts',(89.4049851955275,54.8031418846613,13.0466019122202));
#76224=CARTESIAN_POINT('Ctrl Pts',(89.3693237583149,54.7985612257359,13.0972968118591));
#76225=CARTESIAN_POINT('Ctrl Pts',(89.3308846545162,54.7939805668104,13.1460562244108));
#76226=CARTESIAN_POINT('Ctrl Pts',(89.2899127121818,54.789399907885,13.1925687330206));
#76227=CARTESIAN_POINT('Ctrl Pts',(89.2474605926311,54.7846537652995,13.2407615807016));
#76228=CARTESIAN_POINT('Ctrl Pts',(89.2022894612093,54.779907622714,13.2865415914872));
#76229=CARTESIAN_POINT('Ctrl Pts',(89.1547152007213,54.7751614801285,13.3296021427803));
#76230=CARTESIAN_POINT('Ctrl Pts',(89.108741549382,54.7705750188321,13.3712139461235));
#76231=CARTESIAN_POINT('Ctrl Pts',(89.0605243709355,54.7659885575357,13.410286108892));
#76232=CARTESIAN_POINT('Ctrl Pts',(89.0103822401222,54.7614020962393,13.4465832005817));
#76233=CARTESIAN_POINT('Ctrl Pts',(88.9576215022053,54.7565761130092,13.4847758603415));
#76234=CARTESIAN_POINT('Ctrl Pts',(88.9027297790061,54.7517501297791,13.5198952957746));
#76235=CARTESIAN_POINT('Ctrl Pts',(88.8461097595345,54.7469241465491,13.5517208772613));
#76236=CARTESIAN_POINT('Ctrl Pts',(88.7894897400629,54.742098163319,13.583546458748));
#76237=CARTESIAN_POINT('Ctrl Pts',(88.7311420404278,54.7372721800889,13.6120779711507));
#76238=CARTESIAN_POINT('Ctrl Pts',(88.6714928765752,54.7324461968588,13.6371537148202));
#76239=CARTESIAN_POINT('Ctrl Pts',(88.6146711823758,54.7278489732668,13.661040826501));
#76240=CARTESIAN_POINT('Ctrl Pts',(88.5564353396656,54.7232517496747,13.6818905126966));
#76241=CARTESIAN_POINT('Ctrl Pts',(88.4971423888616,54.7186545260826,13.6995361683636));
#76242=CARTESIAN_POINT('Ctrl Pts',(88.4368341813766,54.7139785855115,13.7174839656775));
#76243=CARTESIAN_POINT('Ctrl Pts',(88.3754327759686,54.7093026449404,13.7321166832191));
#76244=CARTESIAN_POINT('Ctrl Pts',(88.3133366096077,54.7046267043692,13.7433095749118));
#76245=CARTESIAN_POINT('Ctrl Pts',(88.2524537269068,54.7000421259968,13.7542837710974));
#76246=CARTESIAN_POINT('Ctrl Pts',(88.1909035136092,54.6954575476244,13.7619512579306));
#76247=CARTESIAN_POINT('Ctrl Pts',(88.1290757533627,54.690872969252,13.7662449682525));
#76248=CARTESIAN_POINT('Ctrl Pts',(88.0672857811664,54.686291192894,13.7705360543333));
#76249=CARTESIAN_POINT('Ctrl Pts',(88.0052191051471,54.6817094165361,13.7714574173445));
#76250=CARTESIAN_POINT('Ctrl Pts',(87.9432714190773,54.6771276401781,13.7689937389568));
#76251=CARTESIAN_POINT('Ctrl Pts',(87.8813388411998,54.6725469812527,13.7665306614266));
#76252=CARTESIAN_POINT('Ctrl Pts',(87.8195257040799,54.6679663223272,13.7606842015897));
#76253=CARTESIAN_POINT('Ctrl Pts',(87.7582264300416,54.6633856634017,13.7514911325577));
#76254=CARTESIAN_POINT('Ctrl Pts',(87.6947126212843,54.6586395208162,13.7419659491431));
#76255=CARTESIAN_POINT('Ctrl Pts',(87.6317510992091,54.6538933782307,13.7288477465443));
#76256=CARTESIAN_POINT('Ctrl Pts',(87.569770798394,54.6491472356452,13.7122355928755));
#76257=CARTESIAN_POINT('Ctrl Pts',(87.5098757898254,54.6445607743488,13.6961823457429));
#76258=CARTESIAN_POINT('Ctrl Pts',(87.4508975007422,54.6399743130524,13.6768667660837));
#76259=CARTESIAN_POINT('Ctrl Pts',(87.3932065158404,54.635387851756,13.6544287980674));
#76260=CARTESIAN_POINT('Ctrl Pts',(87.3325026948182,54.630561868526,13.6308190365617));
#76261=CARTESIAN_POINT('Ctrl Pts',(87.2732249108346,54.6257358852959,13.6037520761322));
#76262=CARTESIAN_POINT('Ctrl Pts',(87.2157769375249,54.6209099020658,13.5734465551083));
#76263=CARTESIAN_POINT('Ctrl Pts',(87.1583289642153,54.6160839188357,13.5431410340843));
#76264=CARTESIAN_POINT('Ctrl Pts',(87.102711316498,54.6112579356057,13.5095973533818));
#76265=CARTESIAN_POINT('Ctrl Pts',(87.0492910206734,54.6064319523756,13.4730858803508));
#76266=CARTESIAN_POINT('Ctrl Pts',(86.9986250991325,54.6018547989938,13.4384569551571));
#76267=CARTESIAN_POINT('Ctrl Pts',(86.9497234381032,54.5972776456119,13.4010137474302));
#76268=CARTESIAN_POINT('Ctrl Pts',(86.9029180125317,54.5927004922301,13.3609629896828));
#76269=CARTESIAN_POINT('Ctrl Pts',(86.8561945285598,54.5881313520062,13.3209823482332));
#76270=CARTESIAN_POINT('Ctrl Pts',(86.8115603826973,54.5835622117823,13.2784035495247));
#76271=CARTESIAN_POINT('Ctrl Pts',(86.7693177776882,54.5789930715585,13.2334759502425));
#76272=CARTESIAN_POINT('Ctrl Pts',(86.7271165208912,54.5744284037335,13.1885923273181));
#76273=CARTESIAN_POINT('Ctrl Pts',(86.6873025169719,54.5698637359085,13.1413648317498));
#76274=CARTESIAN_POINT('Ctrl Pts',(86.6501428681452,54.5652990680836,13.0920812357118));
#76275=CARTESIAN_POINT('Ctrl Pts',(86.6130056287687,54.5607371530213,13.0428273605761));
#76276=CARTESIAN_POINT('Ctrl Pts',(86.5785198800985,54.5561752379591,12.9915202526092));
#76277=CARTESIAN_POINT('Ctrl Pts',(86.546912586667,54.5516133228969,12.9384808775668));
#76278=CARTESIAN_POINT('Ctrl Pts',(86.5153124778442,54.547052444797,12.8854535588291));
#76279=CARTESIAN_POINT('Ctrl Pts',(86.4865897883838,54.5424915666972,12.8306951961169));
#76280=CARTESIAN_POINT('Ctrl Pts',(86.4609271044993,54.5379306885974,12.7745540587944));
#76281=CARTESIAN_POINT('Ctrl Pts',(86.4352419934899,54.5333658246563,12.7183638586263));
#76282=CARTESIAN_POINT('Ctrl Pts',(86.4126224475418,54.5288009607153,12.6607889370642));
#76283=CARTESIAN_POINT('Ctrl Pts',(86.3932035947369,54.5242360967743,12.6021992416235));
#76284=CARTESIAN_POINT('Ctrl Pts',(86.3737769978184,54.5196694123949,12.5435861809895));
#76285=CARTESIAN_POINT('Ctrl Pts',(86.3575537741795,54.5151027280155,12.4839580367219));
#76286=CARTESIAN_POINT('Ctrl Pts',(86.3446187416312,54.5105360436361,12.4236986683751));
#76287=CARTESIAN_POINT('Ctrl Pts',(86.331659116281,54.5059606768229,12.3633247315716));
#76288=CARTESIAN_POINT('Ctrl Pts',(86.3220002556448,54.5013853100096,12.3023176819412));
#76289=CARTESIAN_POINT('Ctrl Pts',(86.3156753947611,54.4968099431963,12.2410694675598));
#76290=CARTESIAN_POINT('Ctrl Pts',(86.3096506201407,54.4924516570043,12.1827272060709));
#76291=CARTESIAN_POINT('Ctrl Pts',(86.3066505849826,54.4880933708122,12.1241665433601));
#76292=CARTESIAN_POINT('Ctrl Pts',(86.3066600222213,54.4837350846202,12.065724781343));
#76293=CARTESIAN_POINT('',(86.3066606861718,53.6899850846232,12.0675293592027));
#76294=CARTESIAN_POINT('Ctrl Pts',(86.3066600222214,54.4837350845702,12.065724780673));
#76295=CARTESIAN_POINT('Ctrl Pts',(86.3066624166605,54.4826292923442,12.0508968315069));
#76296=CARTESIAN_POINT('Ctrl Pts',(86.3068583141327,54.4815235001183,12.0360706484629));
#76297=CARTESIAN_POINT('Ctrl Pts',(86.3072476018017,54.4804177078924,12.0212495672259));
#76298=CARTESIAN_POINT('Ctrl Pts',(86.3088660274098,54.4758204843003,11.9596323639894));
#76299=CARTESIAN_POINT('Ctrl Pts',(86.3138347189205,54.4712232607082,11.8979765865206));
#76300=CARTESIAN_POINT('Ctrl Pts',(86.3221585533405,54.4666260371161,11.8366762034915));
#76301=CARTESIAN_POINT('Ctrl Pts',(86.3306249144588,54.461950096545,11.7743261910786));
#76302=CARTESIAN_POINT('Ctrl Pts',(86.3425624793092,54.4572741559739,11.7123443908936));
#76303=CARTESIAN_POINT('Ctrl Pts',(86.3579209371358,54.4525982154028,11.6511452693774));
#76304=CARTESIAN_POINT('Ctrl Pts',(86.3729793093529,54.4480136370303,11.5911419043546));
#76305=CARTESIAN_POINT('Ctrl Pts',(86.3913259667826,54.4434290586579,11.5318914252639));
#76306=CARTESIAN_POINT('Ctrl Pts',(86.4128615941009,54.4388444802855,11.473776671187));
#76307=CARTESIAN_POINT('Ctrl Pts',(86.434384059219,54.4342627039276,11.4156974358355));
#76308=CARTESIAN_POINT('Ctrl Pts',(86.4590914530389,54.4296809275696,11.3587530254644));
#76309=CARTESIAN_POINT('Ctrl Pts',(86.4868348657027,54.4250991512116,11.3033103652255));
#76310=CARTESIAN_POINT('Ctrl Pts',(86.514571512128,54.4205184922862,11.2478812266922));
#76311=CARTESIAN_POINT('Ctrl Pts',(86.5453424798089,54.4159378333607,11.1939535662459));
#76312=CARTESIAN_POINT('Ctrl Pts',(86.578951908098,54.4113571744353,11.1418717090793));
#76313=CARTESIAN_POINT('Ctrl Pts',(86.6137755309597,54.4066110318498,11.0879083111809));
#76314=CARTESIAN_POINT('Ctrl Pts',(86.651646367545,54.4018648892642,11.035927158464));
#76315=CARTESIAN_POINT('Ctrl Pts',(86.6922975784569,54.3971187466787,10.9862783881868));
#76316=CARTESIAN_POINT('Ctrl Pts',(86.7315811023166,54.3925322853823,10.9383000227696));
#76317=CARTESIAN_POINT('Ctrl Pts',(86.7734604617028,54.3879458240859,10.8924999195148));
#76318=CARTESIAN_POINT('Ctrl Pts',(86.8176555815901,54.3833593627895,10.8491582129751));
#76319=CARTESIAN_POINT('Ctrl Pts',(86.864158733725,54.3785333795595,10.803553042582));
#76320=CARTESIAN_POINT('Ctrl Pts',(86.9132256763394,54.3737073963294,10.7606705150984));
#76321=CARTESIAN_POINT('Ctrl Pts',(86.9644909547854,54.3688814130993,10.7207886211141));
#76322=CARTESIAN_POINT('Ctrl Pts',(87.0157562332315,54.3640554298693,10.6809067271298));
#76323=CARTESIAN_POINT('Ctrl Pts',(87.0692192701858,54.3592294466392,10.6440257709017));
#76324=CARTESIAN_POINT('Ctrl Pts',(87.1244825926361,54.3544034634091,10.610368960883));
#76325=CARTESIAN_POINT('Ctrl Pts',(87.177126341616,54.349806239817,10.5783075396812));
#76326=CARTESIAN_POINT('Ctrl Pts',(87.2316196777066,54.345209016225,10.5490398251764));
#76327=CARTESIAN_POINT('Ctrl Pts',(87.2876342647683,54.3406117926329,10.5227836027657));
#76328=CARTESIAN_POINT('Ctrl Pts',(87.3446079740018,54.3359358520618,10.4960778023722));
#76329=CARTESIAN_POINT('Ctrl Pts',(87.4031551169578,54.3312599114906,10.4724879515797));
#76330=CARTESIAN_POINT('Ctrl Pts',(87.462900203113,54.3265839709195,10.4521965893417));
#76331=CARTESIAN_POINT('Ctrl Pts',(87.5214779428595,54.3219993925471,10.432301695673));
#76332=CARTESIAN_POINT('Ctrl Pts',(87.5812067290269,54.3174148141747,10.4155777244258));
#76333=CARTESIAN_POINT('Ctrl Pts',(87.6417110618891,54.3128302358023,10.402148890138));
#76334=CARTESIAN_POINT('Ctrl Pts',(87.7021784155568,54.3082484594443,10.3887282633199));
#76335=CARTESIAN_POINT('Ctrl Pts',(87.7634198801215,54.3036666830864,10.3785988901978));
#76336=CARTESIAN_POINT('Ctrl Pts',(87.8250464254723,54.2990849067284,10.3718346881959));
#76337=CARTESIAN_POINT('Ctrl Pts',(87.8866579409526,54.294504247803,10.3650721358901));
#76338=CARTESIAN_POINT('Ctrl Pts',(87.9486538450002,54.2899235888775,10.3616731809678));
#76339=CARTESIAN_POINT('Ctrl Pts',(88.0106386281579,54.2853429299521,10.3616600383109));
#76340=CARTESIAN_POINT('Ctrl Pts',(88.0748627111526,54.2805967873665,10.3616464208545));
#76341=CARTESIAN_POINT('Ctrl Pts',(88.1390742729589,54.275850644781,10.3652679994941));
#76342=CARTESIAN_POINT('Ctrl Pts',(88.2028344224945,54.2711045021955,10.372490510819));
#76343=CARTESIAN_POINT('Ctrl Pts',(88.2644493977779,54.2665180408991,10.3794700248258));
#76344=CARTESIAN_POINT('Ctrl Pts',(88.3256423468815,54.2619315796027,10.3898118419173));
#76345=CARTESIAN_POINT('Ctrl Pts',(88.3860260104896,54.2573451183063,10.40343260977));
#76346=CARTESIAN_POINT('Ctrl Pts',(88.4495631318367,54.2525191350763,10.4177647043827));
#76347=CARTESIAN_POINT('Ctrl Pts',(88.5122035000195,54.2476931518462,10.4357274518014));
#76348=CARTESIAN_POINT('Ctrl Pts',(88.5735153471093,54.2428671686161,10.4571646075914));
#76349=CARTESIAN_POINT('Ctrl Pts',(88.634827194199,54.2380411853861,10.4786017633815));
#76350=CARTESIAN_POINT('Ctrl Pts',(88.6948099514436,54.233215202156,10.50351300755));
#76351=CARTESIAN_POINT('Ctrl Pts',(88.7530605078257,54.2283892189259,10.5316854825931));
#76352=CARTESIAN_POINT('Ctrl Pts',(88.8085498908767,54.2237919953339,10.5585225354259));
#76353=CARTESIAN_POINT('Ctrl Pts',(88.8626954355473,54.2191947717418,10.5884287686047));
#76354=CARTESIAN_POINT('Ctrl Pts',(88.9151360865985,54.2145975481497,10.6212464665174));
#76355=CARTESIAN_POINT('Ctrl Pts',(88.9684746643107,54.2099216075786,10.6546260927303));
#76356=CARTESIAN_POINT('Ctrl Pts',(89.0200488953005,54.2052456670075,10.691017681134));
#76357=CARTESIAN_POINT('Ctrl Pts',(89.0695017591331,54.2005697264363,10.7302047830928));
#76358=CARTESIAN_POINT('Ctrl Pts',(89.1179883740787,54.1959851480639,10.7686262166814));
#76359=CARTESIAN_POINT('Ctrl Pts',(89.1644353561218,54.1914005696915,10.809734573136));
#76360=CARTESIAN_POINT('Ctrl Pts',(89.208534679412,54.1868159913191,10.853281760999));
#76361=CARTESIAN_POINT('Ctrl Pts',(89.2526070499638,54.1822342149611,10.8968023335792));
#76362=CARTESIAN_POINT('Ctrl Pts',(89.2943342453998,54.1776524386032,10.9427584250462));
#76363=CARTESIAN_POINT('Ctrl Pts',(89.3334431566761,54.1730706622452,10.9908632956872));
#76364=CARTESIAN_POINT('Ctrl Pts',(89.3725425298244,54.1684900033198,11.038956434209));
#76365=CARTESIAN_POINT('Ctrl Pts',(89.4090245654839,54.1639093443943,11.0891969167641));
#76366=CARTESIAN_POINT('Ctrl Pts',(89.4426560766216,54.1593286854689,11.141264516809));
#76367=CARTESIAN_POINT('Ctrl Pts',(89.4775025801101,54.1545825428834,11.1952131425243));
#76368=CARTESIAN_POINT('Ctrl Pts',(89.5092882869207,54.1498364002978,11.2511229747902));
#76369=CARTESIAN_POINT('Ctrl Pts',(89.5378039284902,54.1450902577123,11.308606707485));
#76370=CARTESIAN_POINT('Ctrl Pts',(89.5653601773901,54.1405037964159,11.3641564324304));
#76371=CARTESIAN_POINT('Ctrl Pts',(89.5898627778076,54.1359173351195,11.4211753132817));
#76372=CARTESIAN_POINT('Ctrl Pts',(89.6111717068205,54.1313308738231,11.4792927950918));
#76373=CARTESIAN_POINT('Ctrl Pts',(89.6335934667398,54.1265048905931,11.5404453862649));
#76374=CARTESIAN_POINT('Ctrl Pts',(89.6524786405656,54.121678907363,11.6028138577107));
#76375=CARTESIAN_POINT('Ctrl Pts',(89.6677243021645,54.1168529241329,11.6659507252631));
#76376=CARTESIAN_POINT('Ctrl Pts',(89.6829699637634,54.1120269409029,11.7290875928155));
#76377=CARTESIAN_POINT('Ctrl Pts',(89.6945760734779,54.1072009576728,11.7929922050902));
#76378=CARTESIAN_POINT('Ctrl Pts',(89.7025028104862,54.1023749744427,11.8572104463405));
#76379=CARTESIAN_POINT('Ctrl Pts',(89.7100538069661,54.0977777508506,11.9183846360638));
#76380=CARTESIAN_POINT('Ctrl Pts',(89.7142974237847,54.0931805272586,11.9800945583366));
#76381=CARTESIAN_POINT('Ctrl Pts',(89.7151703252516,54.0885833036665,12.041951338256));
#76382=CARTESIAN_POINT('Ctrl Pts',(89.7160581731673,54.0839073630954,12.1048672745882));
#76383=CARTESIAN_POINT('Ctrl Pts',(89.7134586284006,54.0792314225243,12.1679346304526));
#76384=CARTESIAN_POINT('Ctrl Pts',(89.7073598865906,54.0745554819531,12.2307360639514));
#76385=CARTESIAN_POINT('Ctrl Pts',(89.7013803067872,54.0699709035807,12.2923104337271));
#76386=CARTESIAN_POINT('Ctrl Pts',(89.692037091836,54.0653863252083,12.3536286483593));
#76387=CARTESIAN_POINT('Ctrl Pts',(89.6793715957827,54.0608017468359,12.4142973643104));
#76388=CARTESIAN_POINT('Ctrl Pts',(89.66671384066,54.0562199704779,12.4749290005989));
#76389=CARTESIAN_POINT('Ctrl Pts',(89.6507379344762,54.05163819412,12.5349114280546));
#76390=CARTESIAN_POINT('Ctrl Pts',(89.6315366393272,54.047056417762,12.5938596747223));
#76391=CARTESIAN_POINT('Ctrl Pts',(89.6123400271112,54.0424757588366,12.65279354472));
#76392=CARTESIAN_POINT('Ctrl Pts',(89.589919745095,54.0378950999111,12.7106932508293));
#76393=CARTESIAN_POINT('Ctrl Pts',(89.5644183420192,54.0333144409857,12.767189197206));
#76394=CARTESIAN_POINT('Ctrl Pts',(89.5379956598028,54.0285682984001,12.8257261503761));
#76395=CARTESIAN_POINT('Ctrl Pts',(89.5082651541107,54.0238221558146,12.8827554194644));
#76396=CARTESIAN_POINT('Ctrl Pts',(89.4754387020055,54.0190760132291,12.9378911191591));
#76397=CARTESIAN_POINT('Ctrl Pts',(89.4437166773578,54.0144895519327,12.9911718093498));
#76398=CARTESIAN_POINT('Ctrl Pts',(89.4091040885707,54.0099030906363,13.042683933148));
#76399=CARTESIAN_POINT('Ctrl Pts',(89.3718362984402,54.0053166293399,13.0921088657875));
#76400=CARTESIAN_POINT('Ctrl Pts',(89.3326222467849,54.0004906461099,13.1441149507953));
#76401=CARTESIAN_POINT('Ctrl Pts',(89.2904684684486,53.9956646628798,13.193809366909));
#76402=CARTESIAN_POINT('Ctrl Pts',(89.2456950773454,53.9908386796497,13.240862928847));
#76403=CARTESIAN_POINT('Ctrl Pts',(89.2009216862423,53.9860126964196,13.2879164907849));
#76404=CARTESIAN_POINT('Ctrl Pts',(89.1535292081039,53.9811867131896,13.3323288119198));
#76405=CARTESIAN_POINT('Ctrl Pts',(89.1038775564186,53.9763607299595,13.3738201261169));
#76406=CARTESIAN_POINT('Ctrl Pts',(89.0565794756688,53.9717635063674,13.4133446829584));
#76407=CARTESIAN_POINT('Ctrl Pts',(89.0070373960248,53.9671662827753,13.4503812207983));
#76408=CARTESIAN_POINT('Ctrl Pts',(88.9555436663255,53.9625690591833,13.4846656047161));
#76409=CARTESIAN_POINT('Ctrl Pts',(88.9031682238357,53.9578931186121,13.51953703059));
#76410=CARTESIAN_POINT('Ctrl Pts',(88.848774013114,53.953217178041,13.5515607538071));
#76411=CARTESIAN_POINT('Ctrl Pts',(88.7927052492535,53.9485412374699,13.5805004915448));
#76412=CARTESIAN_POINT('Ctrl Pts',(88.7377320009299,53.9439566590975,13.6088747819613));
#76413=CARTESIAN_POINT('Ctrl Pts',(88.6811495224217,53.9393720807251,13.634284273046));
#76414=CARTESIAN_POINT('Ctrl Pts',(88.6233107003458,53.9347875023526,13.6565503581597));
#76415=CARTESIAN_POINT('Ctrl Pts',(88.5655072283506,53.9302057259947,13.67880283463));
#76416=CARTESIAN_POINT('Ctrl Pts',(88.5064494094089,53.9256239496367,13.6979155320779));
#76417=CARTESIAN_POINT('Ctrl Pts',(88.4465109806567,53.9210421732788,13.7137575735913));
#76418=CARTESIAN_POINT('Ctrl Pts',(88.3865871700665,53.9164615143533,13.7295957514477));
#76419=CARTESIAN_POINT('Ctrl Pts',(88.3257836679409,53.9118808554279,13.7421647268433));
#76420=CARTESIAN_POINT('Ctrl Pts',(88.2644882978339,53.9073001965024,13.7513837896637));
#76421=CARTESIAN_POINT('Ctrl Pts',(88.2009785340436,53.9025540539169,13.7609359059341));
#76422=CARTESIAN_POINT('Ctrl Pts',(88.1369412482078,53.8978079113314,13.7668912836917));
#76423=CARTESIAN_POINT('Ctrl Pts',(88.0728155526031,53.8930617687459,13.7692186216268));
#76424=CARTESIAN_POINT('Ctrl Pts',(88.0108473298419,53.8884753074495,13.7714676575904));
#76425=CARTESIAN_POINT('Ctrl Pts',(87.9487970787355,53.8838888461531,13.7703290012007));
#76426=CARTESIAN_POINT('Ctrl Pts',(87.8870601431849,53.8793023848567,13.7658275640466));
#76427=CARTESIAN_POINT('Ctrl Pts',(87.8220990770406,53.8744764016266,13.7610910452333));
#76428=CARTESIAN_POINT('Ctrl Pts',(87.7574855887589,53.8696504183965,13.7526309534498));
#76429=CARTESIAN_POINT('Ctrl Pts',(87.6936698632552,53.8648244351664,13.7405376734829));
#76430=CARTESIAN_POINT('Ctrl Pts',(87.6298541377515,53.8599984519364,13.728444393516));
#76431=CARTESIAN_POINT('Ctrl Pts',(87.5668367849956,53.8551724687063,13.7127181573378));
#76432=CARTESIAN_POINT('Ctrl Pts',(87.5050480590712,53.8503464854762,13.693509591084));
#76433=CARTESIAN_POINT('Ctrl Pts',(87.4461882216034,53.8457492618841,13.6752115428435));
#76434=CARTESIAN_POINT('Ctrl Pts',(87.3882014793481,53.8411520382921,13.6536787651955));
#76435=CARTESIAN_POINT('Ctrl Pts',(87.3314683072925,53.8365548147,13.6290136001347));
#76436=CARTESIAN_POINT('Ctrl Pts',(87.2737637089344,53.8318788741288,13.6039261003229));
#76437=CARTESIAN_POINT('Ctrl Pts',(87.2173565484748,53.8272029335577,13.5755980001816));
#76438=CARTESIAN_POINT('Ctrl Pts',(87.1626320339562,53.8225269929866,13.5441903225873));
#76439=CARTESIAN_POINT('Ctrl Pts',(87.1089767699752,53.8179424146142,13.5133963128609));
#76440=CARTESIAN_POINT('Ctrl Pts',(87.0569394522188,53.8133578362418,13.4796422512973));
#76441=CARTESIAN_POINT('Ctrl Pts',(87.0068615371703,53.8087732578693,13.443127729394));
#76442=CARTESIAN_POINT('Ctrl Pts',(86.9568142288713,53.8041914815114,13.4066355245306));
#76443=CARTESIAN_POINT('Ctrl Pts',(86.9087243591689,53.7996097051534,13.3673865039837));
#76444=CARTESIAN_POINT('Ctrl Pts',(86.8629045950878,53.7950279287955,13.3256236647585));
#76445=CARTESIAN_POINT('Ctrl Pts',(86.8170960058197,53.79044726987,13.2838710109178));
#76446=CARTESIAN_POINT('Ctrl Pts',(86.7735567991505,53.7858666109446,13.2396060982234));
#76447=CARTESIAN_POINT('Ctrl Pts',(86.7325651363716,53.7812859520191,13.1931109683875));
#76448=CARTESIAN_POINT('Ctrl Pts',(86.6900925839436,53.7765398094336,13.1449361273167));
#76449=CARTESIAN_POINT('Ctrl Pts',(86.6503556003815,53.7717936668481,13.0943672372871));
#76450=CARTESIAN_POINT('Ctrl Pts',(86.613618656534,53.7670475242626,13.0417562280268));
#76451=CARTESIAN_POINT('Ctrl Pts',(86.5781177064321,53.7624610629662,12.9909152864855));
#76452=CARTESIAN_POINT('Ctrl Pts',(86.5454183363236,53.7578746016698,12.9381679510526));
#76453=CARTESIAN_POINT('Ctrl Pts',(86.5157140514985,53.7532881403734,12.8838598705243));
#76454=CARTESIAN_POINT('Ctrl Pts',(86.4844584993063,53.7484621571433,12.8267156216255));
#76455=CARTESIAN_POINT('Ctrl Pts',(86.4565197254006,53.7436361739133,12.7678437188743));
#76456=CARTESIAN_POINT('Ctrl Pts',(86.4320659753496,53.7388101906832,12.7076713967456));
#76457=CARTESIAN_POINT('Ctrl Pts',(86.4076122252987,53.7339842074531,12.6474990746169));
#76458=CARTESIAN_POINT('Ctrl Pts',(86.3866436350648,53.7291582242231,12.5860269713807));
#76459=CARTESIAN_POINT('Ctrl Pts',(86.3692670297251,53.724332240993,12.5236982520312));
#76460=CARTESIAN_POINT('Ctrl Pts',(86.3485464875666,53.7185775503028,12.4493750553121));
#76461=CARTESIAN_POINT('Ctrl Pts',(86.3328622147382,53.7128228596126,12.3735907719497));
#76462=CARTESIAN_POINT('Ctrl Pts',(86.3223801757244,53.7070681689225,12.2969500479836));
#76463=CARTESIAN_POINT('Ctrl Pts',(86.3120080250888,53.7013738074894,12.2211127864775));
#76464=CARTESIAN_POINT('Ctrl Pts',(86.3067296976861,53.6956794460563,12.1444367572088));
#76465=CARTESIAN_POINT('Ctrl Pts',(86.3066606861718,53.6899850846232,12.0675293592027));
#76466=CARTESIAN_POINT('',(86.3066601233575,52.8962350845279,12.0653515508395));
#76467=CARTESIAN_POINT('Ctrl Pts',(86.3066606861711,53.6899850845702,12.0675293584867));
#76468=CARTESIAN_POINT('Ctrl Pts',(86.3066056477354,53.6854436845471,12.0061937261784));
#76469=CARTESIAN_POINT('Ctrl Pts',(86.3098658996797,53.6809022845239,11.9447845824161));
#76470=CARTESIAN_POINT('Ctrl Pts',(86.3164385719836,53.6763608845008,11.8836914640537));
#76471=CARTESIAN_POINT('Ctrl Pts',(86.3230076991165,53.6718219340199,11.822631298124));
#76472=CARTESIAN_POINT('Ctrl Pts',(86.3328856501294,53.6672829835391,11.7618873353594));
#76473=CARTESIAN_POINT('Ctrl Pts',(86.3460175785588,53.6627440330583,11.7018456757199));
#76474=CARTESIAN_POINT('Ctrl Pts',(86.3591474682364,53.6582057872564,11.6418133376396));
#76475=CARTESIAN_POINT('Ctrl Pts',(86.3755302206782,53.6536675414546,11.58248359339));
#76476=CARTESIAN_POINT('Ctrl Pts',(86.395059996133,53.6491292956528,11.5242318397116));
#76477=CARTESIAN_POINT('Ctrl Pts',(86.4146081007246,53.6445867906044,11.4659254154424));
#76478=CARTESIAN_POINT('Ctrl Pts',(86.4373089614595,53.640044285556,11.4086994959161));
#76479=CARTESIAN_POINT('Ctrl Pts',(86.463007420663,53.6355017805077,11.352912480885));
#76480=CARTESIAN_POINT('Ctrl Pts',(86.4887181511995,53.6309571063568,11.2970988268621));
#76481=CARTESIAN_POINT('Ctrl Pts',(86.5174290864942,53.626412432206,11.2427259048733));
#76482=CARTESIAN_POINT('Ctrl Pts',(86.548939071428,53.6218677580551,11.1901274768877));
#76483=CARTESIAN_POINT('Ctrl Pts',(86.5805074415662,53.6173146630266,11.1374315886849));
#76484=CARTESIAN_POINT('Ctrl Pts',(86.6148849254102,53.612761567998,11.0865171903036));
#76485=CARTESIAN_POINT('Ctrl Pts',(86.6518276286619,53.6082084729694,11.0376881306766));
#76486=CARTESIAN_POINT('Ctrl Pts',(86.6785772670636,53.6049116474829,11.0023317659945));
#76487=CARTESIAN_POINT('Ctrl Pts',(86.7066709528863,53.6016148219963,10.9680680892726));
#76488=CARTESIAN_POINT('Ctrl Pts',(86.7360040762212,53.5983179965098,10.93500034043));
#76489=CARTESIAN_POINT('Ctrl Pts',(86.7769073412483,53.5937207729177,10.8888893661803));
#76490=CARTESIAN_POINT('Ctrl Pts',(86.8203992414488,53.5891235493257,10.8449055349744));
#76491=CARTESIAN_POINT('Ctrl Pts',(86.8662299000522,53.5845263257336,10.8033534723188));
#76492=CARTESIAN_POINT('Ctrl Pts',(86.9128453042571,53.5798503851625,10.7610899252683));
#76493=CARTESIAN_POINT('Ctrl Pts',(86.9618800316775,53.5751744445913,10.7213426673058));
#76494=CARTESIAN_POINT('Ctrl Pts',(87.0130287778948,53.5704985040202,10.6843964839905));
#76495=CARTESIAN_POINT('Ctrl Pts',(87.0631781397433,53.5659139256478,10.6481721842172));
#76496=CARTESIAN_POINT('Ctrl Pts',(87.1153592202268,53.5613293472754,10.6146407966693));
#76497=CARTESIAN_POINT('Ctrl Pts',(87.1692495734302,53.556744768903,10.5840313583043));
#76498=CARTESIAN_POINT('Ctrl Pts',(87.2231069897883,53.552162992545,10.5534406278948));
#76499=CARTESIAN_POINT('Ctrl Pts',(87.2786711657099,53.5475812161871,10.5257685564865));
#76500=CARTESIAN_POINT('Ctrl Pts',(87.3355919471247,53.5429994398291,10.5012000774185));
#76501=CARTESIAN_POINT('Ctrl Pts',(87.3924988463404,53.5384187809037,10.4766375902661));
#76502=CARTESIAN_POINT('Ctrl Pts',(87.4507612270868,53.5338381219783,10.4551773944843));
#76503=CARTESIAN_POINT('Ctrl Pts',(87.5100075542628,53.5292574630528,10.436956905139));
#76504=CARTESIAN_POINT('Ctrl Pts',(87.5713942501557,53.5245113204673,10.4180781713547));
#76505=CARTESIAN_POINT('Ctrl Pts',(87.6338368100407,53.5197651778818,10.4026779370554));
#76506=CARTESIAN_POINT('Ctrl Pts',(87.6969056406633,53.5150190352963,10.3908523739584));
#76507=CARTESIAN_POINT('Ctrl Pts',(87.7578525560681,53.5104325739999,10.3794246752589));
#76508=CARTESIAN_POINT('Ctrl Pts',(87.8193837348227,53.5058461127035,10.3713349137168));
#76509=CARTESIAN_POINT('Ctrl Pts',(87.881104517804,53.5012596514071,10.3666171710574));
#76510=CARTESIAN_POINT('Ctrl Pts',(87.9460485878324,53.496433668177,10.361653050467));
#76511=CARTESIAN_POINT('Ctrl Pts',(88.0112019651358,53.4916076849469,10.3604228281746));
#76512=CARTESIAN_POINT('Ctrl Pts',(88.0761060336377,53.4867817017169,10.3629039839211));
#76513=CARTESIAN_POINT('Ctrl Pts',(88.1410101021396,53.4819557184868,10.3653851396675));
#76514=CARTESIAN_POINT('Ctrl Pts',(88.2056642241824,53.4771297352567,10.3715775346472));
#76515=CARTESIAN_POINT('Ctrl Pts',(88.2696205463436,53.4723037520266,10.3813961152221));
#76516=CARTESIAN_POINT('Ctrl Pts',(88.3305452323787,53.4677065284345,10.3907492787346));
#76517=CARTESIAN_POINT('Ctrl Pts',(88.3910869330253,53.4631093048424,10.4034309692159));
#76518=CARTESIAN_POINT('Ctrl Pts',(88.4508541930947,53.4585120812503,10.4193964883989));
#76519=CARTESIAN_POINT('Ctrl Pts',(88.5116448313103,53.4538361406792,10.4356353807198));
#76520=CARTESIAN_POINT('Ctrl Pts',(88.5716337197105,53.4491602001081,10.4552716297821));
#76521=CARTESIAN_POINT('Ctrl Pts',(88.6304160071788,53.4444842595369,10.4782032102153));
#76522=CARTESIAN_POINT('Ctrl Pts',(88.6880497601553,53.4398996811645,10.5006867354227));
#76523=CARTESIAN_POINT('Ctrl Pts',(88.7445231422343,53.4353151027921,10.5263377827289));
#76524=CARTESIAN_POINT('Ctrl Pts',(88.7994688403535,53.4307305244196,10.5550096878565));
#76525=CARTESIAN_POINT('Ctrl Pts',(88.854380956619,53.4261487480617,10.583664069215));
#76526=CARTESIAN_POINT('Ctrl Pts',(88.907766789943,53.4215669717037,10.6153354124485));
#76527=CARTESIAN_POINT('Ctrl Pts',(88.9592810507774,53.4169851953457,10.6498298533239));
#76528=CARTESIAN_POINT('Ctrl Pts',(89.0107827479892,53.4124045364202,10.6843158814777));
#76529=CARTESIAN_POINT('Ctrl Pts',(89.0604133560476,53.4078238774947,10.7216233573642));
#76530=CARTESIAN_POINT('Ctrl Pts',(89.1078559094675,53.4032432185693,10.7615146802412));
#76531=CARTESIAN_POINT('Ctrl Pts',(89.1570124013203,53.3984970759838,10.8028471412208));
#76532=CARTESIAN_POINT('Ctrl Pts',(89.2038192314359,53.3937509333983,10.8469533897118));
#76533=CARTESIAN_POINT('Ctrl Pts',(89.2479625930688,53.3890047908128,10.8935246787465));
#76534=CARTESIAN_POINT('Ctrl Pts',(89.2906207762093,53.3844183295164,10.9385291030415));
#76535=CARTESIAN_POINT('Ctrl Pts',(89.3307915913948,53.3798318682199,10.9858348723314));
#76536=CARTESIAN_POINT('Ctrl Pts',(89.3682323432263,53.3752454069235,11.0351289110172));
#76537=CARTESIAN_POINT('Ctrl Pts',(89.4076283892803,53.3704194236935,11.0869972663054));
#76538=CARTESIAN_POINT('Ctrl Pts',(89.4440010363312,53.3655934404635,11.1410667268849));
#76539=CARTESIAN_POINT('Ctrl Pts',(89.477120451333,53.3607674572334,11.1969397847196));
#76540=CARTESIAN_POINT('Ctrl Pts',(89.5102398663347,53.3559414740034,11.2528128425543));
#76541=CARTESIAN_POINT('Ctrl Pts',(89.540105820036,53.3511154907734,11.3104888866465));
#76542=CARTESIAN_POINT('Ctrl Pts',(89.5665468526566,53.3462895075433,11.3695455328667));
#76543=CARTESIAN_POINT('Ctrl Pts',(89.5917345363198,53.3416922839513,11.4258027957559));
#76544=CARTESIAN_POINT('Ctrl Pts',(89.6139181232076,53.3370950603592,11.4835436934228));
#76545=CARTESIAN_POINT('Ctrl Pts',(89.6329228404703,53.3324978367672,11.5424151117911));
#76546=CARTESIAN_POINT('Ctrl Pts',(89.6522529702132,53.327821896196,11.6022945690582));
#76547=CARTESIAN_POINT('Ctrl Pts',(89.6682940405242,53.3231459556249,11.6633431814259));
#76548=CARTESIAN_POINT('Ctrl Pts',(89.6809121743324,53.3184700150538,11.7251654864652));
#76549=CARTESIAN_POINT('Ctrl Pts',(89.6932837651337,53.3138854366814,11.7857798587618));
#76550=CARTESIAN_POINT('Ctrl Pts',(89.702364869821,53.309300858309,11.8471374389696));
#76551=CARTESIAN_POINT('Ctrl Pts',(89.7080794740081,53.3047162799366,11.9088500890859));
#76552=CARTESIAN_POINT('Ctrl Pts',(89.7137905855287,53.3001345035787,11.9705250215053));
#76553=CARTESIAN_POINT('Ctrl Pts',(89.7161392295267,53.2955527272207,12.0325540877018));
#76554=CARTESIAN_POINT('Ctrl Pts',(89.715100990825,53.2909709508628,12.094542050896));
#76555=CARTESIAN_POINT('Ctrl Pts',(89.7140630053354,53.2863902919374,12.1565148960749));
#76556=CARTESIAN_POINT('Ctrl Pts',(89.7096397854306,53.2818096330119,12.2184461494038));
#76557=CARTESIAN_POINT('Ctrl Pts',(89.7018590228373,53.2772289740865,12.2799406471193));
#76558=CARTESIAN_POINT('Ctrl Pts',(89.6937971676995,53.272482831501,12.3436567323232));
#76559=CARTESIAN_POINT('Ctrl Pts',(89.68213054133,53.2677366889154,12.4069033158724));
#76560=CARTESIAN_POINT('Ctrl Pts',(89.6669483202019,53.2629905463299,12.469249298103));
#76561=CARTESIAN_POINT('Ctrl Pts',(89.6522768963367,53.2584040850335,12.5294976849418));
#76562=CARTESIAN_POINT('Ctrl Pts',(89.6343229185176,53.2538176237372,12.5889046279803));
#76563=CARTESIAN_POINT('Ctrl Pts',(89.6132177704993,53.2492311624408,12.6470964218582));
#76564=CARTESIAN_POINT('Ctrl Pts',(89.5910104337698,53.2444051792107,12.7083272059501));
#76565=CARTESIAN_POINT('Ctrl Pts',(89.5653140140062,53.2395791959806,12.7682118453188));
#76566=CARTESIAN_POINT('Ctrl Pts',(89.536337804965,53.2347532127505,12.8263416444892));
#76567=CARTESIAN_POINT('Ctrl Pts',(89.5073615959238,53.2299272295204,12.8844714436596));
#76568=CARTESIAN_POINT('Ctrl Pts',(89.4751059865718,53.2251012462903,12.9408458786286));
#76569=CARTESIAN_POINT('Ctrl Pts',(89.4398328311856,53.2202752630601,12.9950918017754));
#76570=CARTESIAN_POINT('Ctrl Pts',(89.4062316820777,53.2156780394681,13.0467663778713));
#76571=CARTESIAN_POINT('Ctrl Pts',(89.3697546816081,53.2110808158761,13.096721870335));
#76572=CARTESIAN_POINT('Ctrl Pts',(89.3306036918106,53.206483592284,13.1446199201572));
#76573=CARTESIAN_POINT('Ctrl Pts',(89.2907823305195,53.2018076517129,13.1933381149453));
#76574=CARTESIAN_POINT('Ctrl Pts',(89.248194755509,53.1971317111418,13.2399272495526));
#76575=CARTESIAN_POINT('Ctrl Pts',(89.20310058838,53.1924557705706,13.2840603526854));
#76576=CARTESIAN_POINT('Ctrl Pts',(89.1588875064995,53.1878711921983,13.3273311485927));
#76577=CARTESIAN_POINT('Ctrl Pts',(89.1122652843203,53.1832866138259,13.3682406525049));
#76578=CARTESIAN_POINT('Ctrl Pts',(89.0635187746866,53.1787020354535,13.4065144775541));
#76579=CARTESIAN_POINT('Ctrl Pts',(89.0148020580706,53.1741202590956,13.4447649103081));
#76580=CARTESIAN_POINT('Ctrl Pts',(88.9639640279461,53.1695384827377,13.4803825446326));
#76581=CARTESIAN_POINT('Ctrl Pts',(88.911323488337,53.1649567063797,13.5131324928799));
#76582=CARTESIAN_POINT('Ctrl Pts',(88.8586957870345,53.1603760474543,13.5458744538633));
#76583=CARTESIAN_POINT('Ctrl Pts',(88.8042668809664,53.1557953885289,13.5757498483781));
#76584=CARTESIAN_POINT('Ctrl Pts',(88.7483837755344,53.1512147296035,13.6025676044934));
#76585=CARTESIAN_POINT('Ctrl Pts',(88.6904818031715,53.1464685870179,13.6303541951172));
#76586=CARTESIAN_POINT('Ctrl Pts',(88.6310190456313,53.1417224444324,13.654857683996));
#76587=CARTESIAN_POINT('Ctrl Pts',(88.5704060480769,53.1369763018468,13.6759191622485));
#76588=CARTESIAN_POINT('Ctrl Pts',(88.5118323406232,53.1323898405505,13.6962720389496));
#76589=CARTESIAN_POINT('Ctrl Pts',(88.4521850947159,53.1278033792541,13.7134107745029));
#76590=CARTESIAN_POINT('Ctrl Pts',(88.3918495305261,53.1232169179578,13.727243049857));
#76591=CARTESIAN_POINT('Ctrl Pts',(88.328363020525,53.1183909347276,13.7417976976737));
#76592=CARTESIAN_POINT('Ctrl Pts',(88.2641149608831,53.1135649514975,13.7526909457334));
#76593=CARTESIAN_POINT('Ctrl Pts',(88.1995622259961,53.1087389682673,13.759876950232));
#76594=CARTESIAN_POINT('Ctrl Pts',(88.1350094911091,53.1039129850372,13.7670629547306));
#76595=CARTESIAN_POINT('Ctrl Pts',(88.0701527321782,53.0990870018071,13.7705417582285));
#76596=CARTESIAN_POINT('Ctrl Pts',(88.0054474678553,53.0942610185769,13.7703309552393));
#76597=CARTESIAN_POINT('Ctrl Pts',(87.9438093407625,53.0896637949847,13.7701301446626));
#76598=CARTESIAN_POINT('Ctrl Pts',(87.8820555940026,53.0850665713925,13.7665808416365));
#76599=CARTESIAN_POINT('Ctrl Pts',(87.8205799798599,53.0804693478002,13.7596691092211));
#76600=CARTESIAN_POINT('Ctrl Pts',(87.7580517359021,53.0757934072291,13.752639029137));
#76601=CARTESIAN_POINT('Ctrl Pts',(87.6958117695767,53.071117466658,13.7421301947354));
#76602=CARTESIAN_POINT('Ctrl Pts',(87.634275594825,53.0664415260869,13.7281833707944));
#76603=CARTESIAN_POINT('Ctrl Pts',(87.5739417621752,53.0618569477144,13.714509050851));
#76604=CARTESIAN_POINT('Ctrl Pts',(87.5142849862034,53.0572723693418,13.6975299992812));
#76605=CARTESIAN_POINT('Ctrl Pts',(87.4556902889564,53.0526877909692,13.6773366998926));
#76606=CARTESIAN_POINT('Ctrl Pts',(87.3971314037679,53.0481060146111,13.6571557422968));
#76607=CARTESIAN_POINT('Ctrl Pts',(87.3396337904558,53.043524238253,13.6337645977005));
#76608=CARTESIAN_POINT('Ctrl Pts',(87.283567702014,53.0389424618949,13.6073036973442));
#76609=CARTESIAN_POINT('Ctrl Pts',(87.2275152873234,53.0343618029693,13.5808492504391));
#76610=CARTESIAN_POINT('Ctrl Pts',(87.1728941645742,53.0297811440437,13.5513267511701));
#76611=CARTESIAN_POINT('Ctrl Pts',(87.1200530726413,53.025200485118,13.5189240889428));
#76612=CARTESIAN_POINT('Ctrl Pts',(87.065303011405,53.0204543425327,13.4853508285072));
#76613=CARTESIAN_POINT('Ctrl Pts',(87.0124645855012,53.0157081999473,13.4486855690757));
#76614=CARTESIAN_POINT('Ctrl Pts',(86.961893976834,53.010962057362,13.4091870263507));
#76615=CARTESIAN_POINT('Ctrl Pts',(86.9130247877561,53.0063755960654,13.3710173898049));
#76616=CARTESIAN_POINT('Ctrl Pts',(86.8662735807736,53.0017891347689,13.3302025046934));
#76617=CARTESIAN_POINT('Ctrl Pts',(86.8219268580204,52.9972026734723,13.2870159288981));
#76618=CARTESIAN_POINT('Ctrl Pts',(86.7752641857629,52.9923766902426,13.2415739907536));
#76619=CARTESIAN_POINT('Ctrl Pts',(86.731264469373,52.9875507070128,13.1935063199345));
#76620=CARTESIAN_POINT('Ctrl Pts',(86.6902140313079,52.982724723783,13.14317188067));
#76621=CARTESIAN_POINT('Ctrl Pts',(86.6491635932428,52.9778987405532,13.0928374414054));
#76622=CARTESIAN_POINT('Ctrl Pts',(86.6110627509574,52.9730727573235,13.0402368038683));
#76623=CARTESIAN_POINT('Ctrl Pts',(86.5761437956817,52.9682467740937,12.9857622021639));
#76624=CARTESIAN_POINT('Ctrl Pts',(86.5421066500874,52.9635426615986,12.9326632496102));
#76625=CARTESIAN_POINT('Ctrl Pts',(86.5109575200296,52.9588385491035,12.8775741112516));
#76626=CARTESIAN_POINT('Ctrl Pts',(86.482928763992,52.9541344366084,12.8208331824218));
#76627=CARTESIAN_POINT('Ctrl Pts',(86.4541800394326,52.9493094906052,12.7626347617718));
#76628=CARTESIAN_POINT('Ctrl Pts',(86.4287145702846,52.9444845446021,12.7026988858379));
#76629=CARTESIAN_POINT('Ctrl Pts',(86.4067358730977,52.9396595985989,12.6414228416863));
#76630=CARTESIAN_POINT('Ctrl Pts',(86.385384982539,52.9349724739168,12.5818971063152));
#76631=CARTESIAN_POINT('Ctrl Pts',(86.3673245239217,52.9302853492346,12.5211072211321));
#76632=CARTESIAN_POINT('Ctrl Pts',(86.35269385782,52.9255982245525,12.4594406872809));
#76633=CARTESIAN_POINT('Ctrl Pts',(86.3374178863764,52.9207043678888,12.3950542674426));
#76634=CARTESIAN_POINT('Ctrl Pts',(86.3258815299883,52.9158105112251,12.3297125519769));
#76635=CARTESIAN_POINT('Ctrl Pts',(86.3181857479463,52.9109166545614,12.2638755761682));
#76636=CARTESIAN_POINT('Ctrl Pts',(86.3104899659043,52.9060227978976,12.1980386003594));
#76637=CARTESIAN_POINT('Ctrl Pts',(86.3066348771815,52.9011289412339,12.1317069497035));
#76638=CARTESIAN_POINT('Ctrl Pts',(86.3066601233573,52.8962350845702,12.0653515514135));
#76639=CARTESIAN_POINT('',(86.306660409711,52.1024850846248,12.0648182329483));
#76640=CARTESIAN_POINT('Ctrl Pts',(86.3066601233575,52.8962350845279,12.0653515508395));
#76641=CARTESIAN_POINT('Ctrl Pts',(86.3066858000485,52.8912577788647,11.9978646744587));
#76642=CARTESIAN_POINT('Ctrl Pts',(86.3107241159865,52.8862804732015,11.9305012550205));
#76643=CARTESIAN_POINT('Ctrl Pts',(86.3187061355887,52.8813031675382,11.8637221908469));
#76644=CARTESIAN_POINT('Ctrl Pts',(86.3267111976187,52.8763114934303,11.7967503494251));
#76645=CARTESIAN_POINT('Ctrl Pts',(86.3386826266837,52.8713198193224,11.7303665837433));
#76646=CARTESIAN_POINT('Ctrl Pts',(86.3545006531629,52.8663281452145,11.6650202629455));
#76647=CARTESIAN_POINT('Ctrl Pts',(86.3703867161387,52.8613150009176,11.5993928745479));
#76648=CARTESIAN_POINT('Ctrl Pts',(86.3901523795347,52.8563018566207,11.5348122054962));
#76649=CARTESIAN_POINT('Ctrl Pts',(86.4136279471483,52.8512887123237,11.4717127290877));
#76650=CARTESIAN_POINT('Ctrl Pts',(86.4277640539517,52.8482699847526,11.4337165897641));
#76651=CARTESIAN_POINT('Ctrl Pts',(86.4432444489851,52.8452512571815,11.396257107537));
#76652=CARTESIAN_POINT('Ctrl Pts',(86.4600240713583,52.8422325296104,11.3594248062846));
#76653=CARTESIAN_POINT('Ctrl Pts',(86.4855777770241,52.8376353060185,11.3033328535416));
#76654=CARTESIAN_POINT('Ctrl Pts',(86.5142307592316,52.8330380824266,11.2485137929798));
#76655=CARTESIAN_POINT('Ctrl Pts',(86.5458336483086,52.8284408588347,11.1953322117642));
#76656=CARTESIAN_POINT('Ctrl Pts',(86.5779776648541,52.8237649182636,11.1412400171441));
#76657=CARTESIAN_POINT('Ctrl Pts',(86.6131734265545,52.8190889776924,11.088842427819));
#76658=CARTESIAN_POINT('Ctrl Pts',(86.6512127534507,52.8144130371213,11.0385013480681));
#76659=CARTESIAN_POINT('Ctrl Pts',(86.6885088381055,52.8098284587491,10.9891438718666));
#76660=CARTESIAN_POINT('Ctrl Pts',(86.7285380461163,52.8052438803768,10.9417636901763));
#76661=CARTESIAN_POINT('Ctrl Pts',(86.7710594362043,52.8006593020046,10.8966744534331));
#76662=CARTESIAN_POINT('Ctrl Pts',(86.8135548379592,52.7960775256469,10.851612774446));
#76663=CARTESIAN_POINT('Ctrl Pts',(86.8585390530228,52.7914957492891,10.8088396336136));
#76664=CARTESIAN_POINT('Ctrl Pts',(86.9057316990031,52.7869139729314,10.7686346627062));
#76665=CARTESIAN_POINT('Ctrl Pts',(86.9529128353433,52.7823333140061,10.7284394972406));
#76666=CARTESIAN_POINT('Ctrl Pts',(87.0023009460659,52.7777526550809,10.6908115882876));
#76667=CARTESIAN_POINT('Ctrl Pts',(87.0535812526061,52.7731719961556,10.6559914263599));
#76668=CARTESIAN_POINT('Ctrl Pts',(87.1067141425788,52.7684258535699,10.6199133301595));
#76669=CARTESIAN_POINT('Ctrl Pts',(87.1618781181891,52.7636797109842,10.5868501134878));
#76670=CARTESIAN_POINT('Ctrl Pts',(87.2186907889171,52.7589335683985,10.5570198975357));
#76671=CARTESIAN_POINT('Ctrl Pts',(87.2735920293924,52.7543471071023,10.5281933023689));
#76672=CARTESIAN_POINT('Ctrl Pts',(87.3300322706156,52.7497606458062,10.5023857575206));
#76673=CARTESIAN_POINT('Ctrl Pts',(87.3876442761706,52.74517418451,10.4797457715835));
#76674=CARTESIAN_POINT('Ctrl Pts',(87.4482649932609,52.7403482012795,10.4559234420326));
#76675=CARTESIAN_POINT('Ctrl Pts',(87.5101826099621,52.7355222180491,10.4356087979634));
#76676=CARTESIAN_POINT('Ctrl Pts',(87.5729521277682,52.7306962348186,10.4189150303542));
#76677=CARTESIAN_POINT('Ctrl Pts',(87.6357216455744,52.7258702515882,10.4022212627449));
#76678=CARTESIAN_POINT('Ctrl Pts',(87.6993424141855,52.7210442683577,10.3891484262244));
#76679=CARTESIAN_POINT('Ctrl Pts',(87.7633613538561,52.7162182851273,10.3797467756781));
#76680=CARTESIAN_POINT('Ctrl Pts',(87.8243456892375,52.711621061534,10.3707907790152));
#76681=CARTESIAN_POINT('Ctrl Pts',(87.8859416847116,52.7070238379407,10.3651289653363));
#76682=CARTESIAN_POINT('Ctrl Pts',(87.9477620249569,52.7024266143474,10.3628335976445));
#76683=CARTESIAN_POINT('Ctrl Pts',(88.0106408976501,52.6977506737764,10.3604989270119));
#76684=CARTESIAN_POINT('Ctrl Pts',(88.0737513593552,52.6930747332054,10.3616472439076));
#76685=CARTESIAN_POINT('Ctrl Pts',(88.1366764500734,52.6883987926345,10.3662999483741));
#76686=CARTESIAN_POINT('Ctrl Pts',(88.1983720609748,52.6838142142608,10.3708617446486));
#76687=CARTESIAN_POINT('Ctrl Pts',(88.2598889476235,52.6792296358872,10.3787921778162));
#76688=CARTESIAN_POINT('Ctrl Pts',(88.3208329193961,52.6746450575136,10.390058951616));
#76689=CARTESIAN_POINT('Ctrl Pts',(88.3817396432744,52.6700632811544,10.4013188393598));
#76690=CARTESIAN_POINT('Ctrl Pts',(88.4420736470582,52.6654815047953,10.4159109321208));
#76691=CARTESIAN_POINT('Ctrl Pts',(88.501447927114,52.6608997284361,10.4337513466418));
#76692=CARTESIAN_POINT('Ctrl Pts',(88.560807726596,52.6563190695094,10.45158741013));
#76693=CARTESIAN_POINT('Ctrl Pts',(88.6192077797048,52.6517384105828,10.4726700762792));
#76694=CARTESIAN_POINT('Ctrl Pts',(88.676275309765,52.6471577516561,10.4968653347093));
#76695=CARTESIAN_POINT('Ctrl Pts',(88.735404495967,52.6424116090718,10.5219346856941));
#76696=CARTESIAN_POINT('Ctrl Pts',(88.7931024763872,52.6376654664874,10.5503456616479));
#76697=CARTESIAN_POINT('Ctrl Pts',(88.8489785946509,52.6329193239031,10.5818953168638));
#76698=CARTESIAN_POINT('Ctrl Pts',(88.902974792473,52.6283328626055,10.6123835017483));
#76699=CARTESIAN_POINT('Ctrl Pts',(88.9552693743075,52.6237464013079,10.6458021629032));
#76700=CARTESIAN_POINT('Ctrl Pts',(89.0055383863637,52.6191599400103,10.6819233281176));
#76701=CARTESIAN_POINT('Ctrl Pts',(89.0584326316906,52.6143339567826,10.719930873844));
#76702=CARTESIAN_POINT('Ctrl Pts',(89.1090834329309,52.6095079735549,10.7609305366531));
#76703=CARTESIAN_POINT('Ctrl Pts',(89.1571543293087,52.6046819903272,10.8046098585264));
#76704=CARTESIAN_POINT('Ctrl Pts',(89.2052252256866,52.5998560070995,10.8482891803997));
#76705=CARTESIAN_POINT('Ctrl Pts',(89.2507158185852,52.5950300238717,10.8946476446369));
#76706=CARTESIAN_POINT('Ctrl Pts',(89.2933381379182,52.590204040644,10.9433318675404));
#76707=CARTESIAN_POINT('Ctrl Pts',(89.333940088373,52.5856068170538,10.9897083772467));
#76708=CARTESIAN_POINT('Ctrl Pts',(89.3721062896434,52.5810095934636,11.0383855163199));
#76709=CARTESIAN_POINT('Ctrl Pts',(89.4075659526996,52.5764123698734,11.0890770883226));
#76710=CARTESIAN_POINT('Ctrl Pts',(89.4436327817057,52.571736429302,11.1406366380165));
#76711=CARTESIAN_POINT('Ctrl Pts',(89.4768990927446,52.5670604887307,11.1942799186709));
#76712=CARTESIAN_POINT('Ctrl Pts',(89.5071207485995,52.5623845481593,11.2496682407195));
#76713=CARTESIAN_POINT('Ctrl Pts',(89.536751909997,52.5577999697888,11.3039743422129));
#76714=CARTESIAN_POINT('Ctrl Pts',(89.5634560684134,52.5532153914182,11.3599574381604));
#76715=CARTESIAN_POINT('Ctrl Pts',(89.5870465481152,52.5486308130476,11.4172688432222));
#76716=CARTESIAN_POINT('Ctrl Pts',(89.6106226097266,52.5440490366915,11.4745452205516));
#76717=CARTESIAN_POINT('Ctrl Pts',(89.6310885726903,52.5394672603354,11.5331478274829));
#76718=CARTESIAN_POINT('Ctrl Pts',(89.6483049988145,52.5348854839793,11.5927060358961));
#76719=CARTESIAN_POINT('Ctrl Pts',(89.6655172260881,52.5303048250556,11.6522497188782));
#76720=CARTESIAN_POINT('Ctrl Pts',(89.6794813484911,52.525724166132,11.7127480518802));
#76721=CARTESIAN_POINT('Ctrl Pts',(89.6901077573731,52.5211435072084,11.7738151702612));
#76722=CARTESIAN_POINT('Ctrl Pts',(89.7011180623501,52.5163973646211,11.8370884364144));
#76723=CARTESIAN_POINT('Ctrl Pts',(89.7085447131949,52.5116512220338,11.9009718095415));
#76724=CARTESIAN_POINT('Ctrl Pts',(89.7123463173579,52.5069050794465,11.9650270134499));
#76725=CARTESIAN_POINT('Ctrl Pts',(89.7160200186911,52.5023186181519,12.026927116121));
#76726=CARTESIAN_POINT('Ctrl Pts',(89.716308810466,52.4977321568572,12.0889871418802));
#76727=CARTESIAN_POINT('Ctrl Pts',(89.7132285048279,52.4931456955626,12.1508112784445));
#76728=CARTESIAN_POINT('Ctrl Pts',(89.7099873342589,52.488319712329,12.2158640996341));
#76729=CARTESIAN_POINT('Ctrl Pts',(89.703015581476,52.4834937290953,12.2806550765543));
#76730=CARTESIAN_POINT('Ctrl Pts',(89.6923932531676,52.4786677458617,12.3447320645396));
#76731=CARTESIAN_POINT('Ctrl Pts',(89.6817709248592,52.4738417626281,12.408809052525));
#76732=CARTESIAN_POINT('Ctrl Pts',(89.6674982389069,52.4690157793944,12.4721714364314));
#76733=CARTESIAN_POINT('Ctrl Pts',(89.6497158858192,52.4641897961608,12.5343856116107));
#76734=CARTESIAN_POINT('Ctrl Pts',(89.632776445882,52.4595925725695,12.5936507312766));
#76735=CARTESIAN_POINT('Ctrl Pts',(89.6125830511616,52.4549953489782,12.6521173850085));
#76736=CARTESIAN_POINT('Ctrl Pts',(89.5892292657091,52.4503981253869,12.7094028446156));
#76737=CARTESIAN_POINT('Ctrl Pts',(89.5654755998887,52.4457221848157,12.7676691872022));
#76738=CARTESIAN_POINT('Ctrl Pts',(89.5384523500933,52.4410462442445,12.8247129684509));
#76739=CARTESIAN_POINT('Ctrl Pts',(89.5083116368733,52.4363703036732,12.8801453787155));
#76740=CARTESIAN_POINT('Ctrl Pts',(89.4787598365825,52.4317857253017,12.9344947070085));
#76741=CARTESIAN_POINT('Ctrl Pts',(89.44621155495,52.4272011469301,12.987294597847));
#76742=CARTESIAN_POINT('Ctrl Pts',(89.4108584772245,52.4226165685585,13.0381990944979));
#76743=CARTESIAN_POINT('Ctrl Pts',(89.3755270066846,52.4180347922014,13.0890724792069));
#76744=CARTESIAN_POINT('Ctrl Pts',(89.337394428918,52.4134530158443,13.1380523494934));
#76745=CARTESIAN_POINT('Ctrl Pts',(89.2966964853522,52.4088712394872,13.1848205321466));
#76746=CARTESIAN_POINT('Ctrl Pts',(89.2560084674577,52.4042905805626,13.2315773086804));
#76747=CARTESIAN_POINT('Ctrl Pts',(89.2127566598054,52.399709921638,13.2761230845364));
#76748=CARTESIAN_POINT('Ctrl Pts',(89.1672166318282,52.3951292627134,13.3181732850863));
#76749=CARTESIAN_POINT('Ctrl Pts',(89.1200313971876,52.3903831201271,13.361742616678));
#76750=CARTESIAN_POINT('Ctrl Pts',(89.0703898291941,52.3856369775408,13.4026321658333));
#76751=CARTESIAN_POINT('Ctrl Pts',(89.0186376816877,52.3808908349544,13.4405694373305));
#76752=CARTESIAN_POINT('Ctrl Pts',(88.9686267059997,52.376304373659,13.477230330722));
#76753=CARTESIAN_POINT('Ctrl Pts',(88.9166454047811,52.3717179123635,13.5111342320162));
#76754=CARTESIAN_POINT('Ctrl Pts',(88.8630348847986,52.367131451068,13.5420797372385));
#76755=CARTESIAN_POINT('Ctrl Pts',(88.8066246256006,52.3623054678362,13.5746413309551));
#76756=CARTESIAN_POINT('Ctrl Pts',(88.7484108841394,52.3574794846045,13.6039267595688));
#76757=CARTESIAN_POINT('Ctrl Pts',(88.688816912249,52.3526535013727,13.6297579956852));
#76758=CARTESIAN_POINT('Ctrl Pts',(88.6292229403586,52.347827518141,13.6555892318015));
#76759=CARTESIAN_POINT('Ctrl Pts',(88.5682493730131,52.3430015349092,13.6779661248141));
#76760=CARTESIAN_POINT('Ctrl Pts',(88.5063368010146,52.3381755516775,13.6967716851726));
#76761=CARTESIAN_POINT('Ctrl Pts',(88.4473589878856,52.3335783280763,13.7146858306975));
#76762=CARTESIAN_POINT('Ctrl Pts',(88.3872870418415,52.328981104475,13.7294331729696));
#76763=CARTESIAN_POINT('Ctrl Pts',(88.3264932499655,52.3243838808738,13.7408847258323));
#76764=CARTESIAN_POINT('Ctrl Pts',(88.2646585030634,52.3197079403038,13.7525323604187));
#76765=CARTESIAN_POINT('Ctrl Pts',(88.2020774375247,52.3150319997338,13.7607700325316));
#76766=CARTESIAN_POINT('Ctrl Pts',(88.1391592105617,52.3103560591638,13.7655146519957));
#76767=CARTESIAN_POINT('Ctrl Pts',(88.0774703291852,52.3057714807822,13.7701665673696));
#76768=CARTESIAN_POINT('Ctrl Pts',(88.0154578752452,52.3011869024006,13.7714606623572));
#76769=CARTESIAN_POINT('Ctrl Pts',(87.9535164641609,52.296602324019,13.7693703292906));
#76770=CARTESIAN_POINT('Ctrl Pts',(87.8916129105884,52.2920205476518,13.7672812737991));
#76771=CARTESIAN_POINT('Ctrl Pts',(87.8297808214775,52.2874387712846,13.7618119089304));
#76772=CARTESIAN_POINT('Ctrl Pts',(87.7684153667387,52.2828569949175,13.752987709293));
#76773=CARTESIAN_POINT('Ctrl Pts',(87.7070648781943,52.2782763359829,13.744165661757));
#76774=CARTESIAN_POINT('Ctrl Pts',(87.6461813017391,52.2736956770482,13.731990476122));
#76775=CARTESIAN_POINT('Ctrl Pts',(87.586153183064,52.2691150181136,13.7165393111766));
#76776=CARTESIAN_POINT('Ctrl Pts',(87.5239564524399,52.264368875537,13.7005299481457));
#76777=CARTESIAN_POINT('Ctrl Pts',(87.4626787516,52.2596227329604,13.6810034567997));
#76778=CARTESIAN_POINT('Ctrl Pts',(87.4027365460003,52.2548765903838,13.6581025111871));
#76779=CARTESIAN_POINT('Ctrl Pts',(87.3448110618613,52.2502901290784,13.6359720548821));
#76780=CARTESIAN_POINT('Ctrl Pts',(87.288133083026,52.245703667773,13.6106908972693));
#76781=CARTESIAN_POINT('Ctrl Pts',(87.2330568291272,52.2411172064676,13.5824363680987));
#76782=CARTESIAN_POINT('Ctrl Pts',(87.1751042903378,52.2362912232554,13.5527062833194));
#76783=CARTESIAN_POINT('Ctrl Pts',(87.1189259206474,52.2314652400432,13.5196840670374));
#76784=CARTESIAN_POINT('Ctrl Pts',(87.0649008559051,52.226639256831,13.483628740236));
#76785=CARTESIAN_POINT('Ctrl Pts',(87.0108757911629,52.2218132736188,13.4475734134345));
#76786=CARTESIAN_POINT('Ctrl Pts',(86.9590045023056,52.2169872904066,13.4084854278801));
#76787=CARTESIAN_POINT('Ctrl Pts',(86.9096242506336,52.2121613071944,13.3666714782402));
#76788=CARTESIAN_POINT('Ctrl Pts',(86.8628648716396,52.2075914645873,13.3270768173739));
#76789=CARTESIAN_POINT('Ctrl Pts',(86.8181334255304,52.2030216219802,13.2848640209387));
#76790=CARTESIAN_POINT('Ctrl Pts',(86.7757433169464,52.1984517793732,13.2402724396713));
#76791=CARTESIAN_POINT('Ctrl Pts',(86.733775453883,52.1939274567148,13.1961250326716));
#76792=CARTESIAN_POINT('Ctrl Pts',(86.6941028933692,52.1894031340565,13.1496463735899));
#76793=CARTESIAN_POINT('Ctrl Pts',(86.6569975161341,52.1848788113982,13.1011097088159));
#76794=CARTESIAN_POINT('Ctrl Pts',(86.6199281062314,52.1803588742988,13.0526200920573));
#76795=CARTESIAN_POINT('Ctrl Pts',(86.5854212685,52.1758389371994,13.0020768350406));
#76796=CARTESIAN_POINT('Ctrl Pts',(86.553710141661,52.1713190000999,12.9497879295297));
#76797=CARTESIAN_POINT('Ctrl Pts',(86.5220173283185,52.1668016733099,12.8975292213904));
#76798=CARTESIAN_POINT('Ctrl Pts',(86.4931172975748,52.1622843465199,12.843527310607));
#76799=CARTESIAN_POINT('Ctrl Pts',(86.4671998749245,52.1577670197298,12.7881191102698));
#76800=CARTESIAN_POINT('Ctrl Pts',(86.4407689541676,52.1531601918044,12.7316131153585));
#76801=CARTESIAN_POINT('Ctrl Pts',(86.4174404093148,52.148553363879,12.673644980549));
#76802=CARTESIAN_POINT('Ctrl Pts',(86.3973653048879,52.1439465359536,12.6145963054291));
#76803=CARTESIAN_POINT('Ctrl Pts',(86.3776695877166,52.1394267696826,12.5566635555033));
#76804=CARTESIAN_POINT('Ctrl Pts',(86.3611054955156,52.1349070034116,12.4976912889509));
#76805=CARTESIAN_POINT('Ctrl Pts',(86.3477652985263,52.1303872371406,12.4380553230553));
#76806=CARTESIAN_POINT('Ctrl Pts',(86.3340396547405,52.1257368783879,12.376696257266));
#76807=CARTESIAN_POINT('Ctrl Pts',(86.323727234676,52.1210865196353,12.3146351214984));
#76808=CARTESIAN_POINT('Ctrl Pts',(86.3168715966915,52.1164361608827,12.2522895292375));
#76809=CARTESIAN_POINT('Ctrl Pts',(86.3100159587071,52.11178580213,12.1899439369766));
#76810=CARTESIAN_POINT('Ctrl Pts',(86.3066170756141,52.1071354433774,12.1273144895588));
#76811=CARTESIAN_POINT('Ctrl Pts',(86.3066604097109,52.1024850846248,12.0648182329483));
#76812=CARTESIAN_POINT('',(86.3066605745511,51.3087350845309,12.0673994500905));
#76813=CARTESIAN_POINT('Ctrl Pts',(86.3066604097115,52.1024850845701,12.0648182322137));
#76814=CARTESIAN_POINT('Ctrl Pts',(86.3067111580443,52.0970390772838,11.9916292403597));
#76815=CARTESIAN_POINT('Ctrl Pts',(86.3114763800807,52.0915930699975,11.9186024518142));
#76816=CARTESIAN_POINT('Ctrl Pts',(86.3208935106417,52.0861470627112,11.8461935164083));
#76817=CARTESIAN_POINT('Ctrl Pts',(86.3288429408399,52.0815498391194,11.7850698254908));
#76818=CARTESIAN_POINT('Ctrl Pts',(86.340128826112,52.0769526155277,11.7242524630003));
#76819=CARTESIAN_POINT('Ctrl Pts',(86.3547154834296,52.0723553919359,11.6641338086265));
#76820=CARTESIAN_POINT('Ctrl Pts',(86.3695519040185,52.0676794513647,11.6029857592751));
#76821=CARTESIAN_POINT('Ctrl Pts',(86.38780322277,52.0630035107936,11.5425611089259));
#76822=CARTESIAN_POINT('Ctrl Pts',(86.4093767528214,52.0583275702224,11.4832669481684));
#76823=CARTESIAN_POINT('Ctrl Pts',(86.4305287622981,52.0537429918508,11.4251313232952));
#76824=CARTESIAN_POINT('Ctrl Pts',(86.454874144327,52.0491584134791,11.3680829098034));
#76825=CARTESIAN_POINT('Ctrl Pts',(86.4822747215772,52.0445738351075,11.3124922968469));
#76826=CARTESIAN_POINT('Ctrl Pts',(86.5096585520707,52.0399920587504,11.2569356599069));
#76827=CARTESIAN_POINT('Ctrl Pts',(86.5400936506463,52.0354102823934,11.2028355124607));
#76828=CARTESIAN_POINT('Ctrl Pts',(86.5733941459654,52.0308285060364,11.1505415115662));
#76829=CARTESIAN_POINT('Ctrl Pts',(86.6066865197486,52.026247847112,11.0982602644643));
#76830=CARTESIAN_POINT('Ctrl Pts',(86.6428426296857,52.0216671881876,11.0477847186531));
#76831=CARTESIAN_POINT('Ctrl Pts',(86.6816322280494,52.0170865292632,10.9994372205542));
#76832=CARTESIAN_POINT('Ctrl Pts',(86.7218231629647,52.012340386677,10.9493430914222));
#76833=CARTESIAN_POINT('Ctrl Pts',(86.7648411935247,52.0075942440907,10.9015342057474));
#76834=CARTESIAN_POINT('Ctrl Pts',(86.8103848719461,52.0028481015044,10.8563313884009));
#76835=CARTESIAN_POINT('Ctrl Pts',(86.8543962589852,51.9982616402095,10.812649394358));
#76836=CARTESIAN_POINT('Ctrl Pts',(86.9007655913499,51.9936751789146,10.7714011796717));
#76837=CARTESIAN_POINT('Ctrl Pts',(86.9491854582199,51.9890887176196,10.7328365762352));
#76838=CARTESIAN_POINT('Ctrl Pts',(87.0001339892513,51.9842627343877,10.6922579868686));
#76839=CARTESIAN_POINT('Ctrl Pts',(87.0533525810631,51.9794367511557,10.6546513716129));
#76840=CARTESIAN_POINT('Ctrl Pts',(87.1084491168998,51.9746107679237,10.6202556453456));
#76841=CARTESIAN_POINT('Ctrl Pts',(87.1635456527366,51.9697847846918,10.5858599190783));
#76842=CARTESIAN_POINT('Ctrl Pts',(87.2205195270349,51.9649588014598,10.5546753250427));
#76843=CARTESIAN_POINT('Ctrl Pts',(87.2789524109492,51.9601328182278,10.5268829924386));
#76844=CARTESIAN_POINT('Ctrl Pts',(87.3346154797033,51.9555355945679,10.5004080622803));
#76845=CARTESIAN_POINT('Ctrl Pts',(87.3918308845876,51.950938370908,10.4769023109299));
#76846=CARTESIAN_POINT('Ctrl Pts',(87.4502496246742,51.9463411472481,10.4565485865762));
#76847=CARTESIAN_POINT('Ctrl Pts',(87.5096686515911,51.9416652066855,10.4358463514125));
#76848=CARTESIAN_POINT('Ctrl Pts',(87.5703321721983,51.9369892661229,10.418405415213));
#76849=CARTESIAN_POINT('Ctrl Pts',(87.6318479078409,51.9323133255602,10.4043687152044));
#76850=CARTESIAN_POINT('Ctrl Pts',(87.6921617017417,51.9277287471196,10.3906062750333));
#76851=CARTESIAN_POINT('Ctrl Pts',(87.7532941876698,51.9231441686789,10.3801163569567));
#76852=CARTESIAN_POINT('Ctrl Pts',(87.8148590786071,51.9185595902382,10.3729838823699));
#76853=CARTESIAN_POINT('Ctrl Pts',(87.8763863421556,51.9139778138121,10.3658557670274));
#76854=CARTESIAN_POINT('Ctrl Pts',(87.9383449820718,51.9093960373859,10.3620810847948));
#76855=CARTESIAN_POINT('Ctrl Pts',(88.0003404276645,51.9048142609597,10.3616933347787));
#76856=CARTESIAN_POINT('Ctrl Pts',(88.0623207534155,51.9002336019662,10.3613056793296));
#76857=CARTESIAN_POINT('Ctrl Pts',(88.1243373582144,51.8956529429727,10.3643033194917));
#76858=CARTESIAN_POINT('Ctrl Pts',(88.185994545916,51.8910722839792,10.3706676595724));
#76859=CARTESIAN_POINT('Ctrl Pts',(88.2498791967054,51.8863261414596,10.3772619214698));
#76860=CARTESIAN_POINT('Ctrl Pts',(88.3133773792603,51.8815799989401,10.3874707993819));
#76861=CARTESIAN_POINT('Ctrl Pts',(88.3760560569369,51.8768338564206,10.4012150556622));
#76862=CARTESIAN_POINT('Ctrl Pts',(88.4366259475975,51.8722473950572,10.4144968945741));
#76863=CARTESIAN_POINT('Ctrl Pts',(88.4964301152985,51.8676609336939,10.4310797722773));
#76864=CARTESIAN_POINT('Ctrl Pts',(88.5550919317186,51.8630744723306,10.4508409349421));
#76865=CARTESIAN_POINT('Ctrl Pts',(88.6168172820691,51.8582484892329,10.4716340975691));
#76866=CARTESIAN_POINT('Ctrl Pts',(88.677277092279,51.8534225061353,10.4959463811966));
#76867=CARTESIAN_POINT('Ctrl Pts',(88.7360579612984,51.8485965230376,10.5235779473964));
#76868=CARTESIAN_POINT('Ctrl Pts',(88.7948388303178,51.84377053994,10.5512095135962));
#76869=CARTESIAN_POINT('Ctrl Pts',(88.8519402253361,51.8389445568423,10.5821599855566));
#76870=CARTESIAN_POINT('Ctrl Pts',(88.9069830748624,51.8341185737447,10.6161761606457));
#76871=CARTESIAN_POINT('Ctrl Pts',(88.9594168014754,51.8295213502986,10.6485799122753));
#76872=CARTESIAN_POINT('Ctrl Pts',(89.0101980435192,51.8249241268526,10.6838982930395));
#76873=CARTESIAN_POINT('Ctrl Pts',(89.0589838887052,51.8203269034065,10.7219372765327));
#76874=CARTESIAN_POINT('Ctrl Pts',(89.108605082099,51.8156509628171,10.7606275923245));
#76875=CARTESIAN_POINT('Ctrl Pts',(89.1561614010464,51.8109750222277,10.8021323582303));
#76876=CARTESIAN_POINT('Ctrl Pts',(89.2013199894643,51.8062990816384,10.8461995416128));
#76877=CARTESIAN_POINT('Ctrl Pts',(89.2455962323468,51.801714503411,10.8894057042266));
#76878=CARTESIAN_POINT('Ctrl Pts',(89.2875672179041,51.7971299251836,10.9350746791043));
#76879=CARTESIAN_POINT('Ctrl Pts',(89.3269520802885,51.7925453469563,10.9829279996305));
#76880=CARTESIAN_POINT('Ctrl Pts',(89.3663128713366,51.7879635707426,11.0307520730475));
#76881=CARTESIAN_POINT('Ctrl Pts',(89.403090350482,51.783381794529,11.0807574527049));
#76882=CARTESIAN_POINT('Ctrl Pts',(89.4370423597757,51.7788000183153,11.1326308213117));
#76883=CARTESIAN_POINT('Ctrl Pts',(89.4709860886462,51.7742193595332,11.1844915387248));
#76884=CARTESIAN_POINT('Ctrl Pts',(89.5021054369677,51.7696387007511,11.2382189149636));
#76885=CARTESIAN_POINT('Ctrl Pts',(89.5302014022898,51.7650580419689,11.2934704310639));
#76886=CARTESIAN_POINT('Ctrl Pts',(89.5593123812506,51.7603118992433,11.3507180003967));
#76887=CARTESIAN_POINT('Ctrl Pts',(89.5851770245851,51.7555657565177,11.409601453028));
#76888=CARTESIAN_POINT('Ctrl Pts',(89.6076270229513,51.7508196137921,11.4697140072234));
#76889=CARTESIAN_POINT('Ctrl Pts',(89.6293217024915,51.746233152635,11.5278041049746));
#76890=CARTESIAN_POINT('Ctrl Pts',(89.6478277825351,51.7416466914778,11.5870413819114));
#76891=CARTESIAN_POINT('Ctrl Pts',(89.6630441084574,51.7370602303207,11.6470428431076));
#76892=CARTESIAN_POINT('Ctrl Pts',(89.6790550884844,51.7322342468108,11.7101778076001));
#76893=CARTESIAN_POINT('Ctrl Pts',(89.6914231524119,51.727408263301,11.7741583320411));
#76894=CARTESIAN_POINT('Ctrl Pts',(89.7000919605218,51.7225822797911,11.8385287171955));
#76895=CARTESIAN_POINT('Ctrl Pts',(89.7087607686316,51.7177562962812,11.90289910235));
#76896=CARTESIAN_POINT('Ctrl Pts',(89.7137303484956,51.7129303127714,11.9676586962098));
#76897=CARTESIAN_POINT('Ctrl Pts',(89.7150078131359,51.7081043292615,12.0323516958568));
#76898=CARTESIAN_POINT('Ctrl Pts',(89.7162247237674,51.7035071056239,12.0939781366755));
#76899=CARTESIAN_POINT('Ctrl Pts',(89.71409668693,51.6989098819864,12.1557971814345));
#76900=CARTESIAN_POINT('Ctrl Pts',(89.7086007131203,51.6943126583488,12.2174155025532));
#76901=CARTESIAN_POINT('Ctrl Pts',(89.703010633344,51.6896367177834,12.2800888963248));
#76902=CARTESIAN_POINT('Ctrl Pts',(89.6939360891808,51.6849607772179,12.3425540995861));
#76903=CARTESIAN_POINT('Ctrl Pts',(89.6814082778584,51.6802848366525,12.4043947707369));
#76904=CARTESIAN_POINT('Ctrl Pts',(89.6691252446246,51.6757002582384,12.465027150919));
#76905=CARTESIAN_POINT('Ctrl Pts',(89.6535227817232,51.6711156798242,12.5250586618879));
#76906=CARTESIAN_POINT('Ctrl Pts',(89.6346824935692,51.6665311014101,12.5841023023275));
#76907=CARTESIAN_POINT('Ctrl Pts',(89.6158537202772,51.661949325012,12.6431098563032));
#76908=CARTESIAN_POINT('Ctrl Pts',(89.5937912000363,51.6573675486138,12.7011302529871));
#76909=CARTESIAN_POINT('Ctrl Pts',(89.5686268111683,51.6527857722156,12.757790107424));
#76910=CARTESIAN_POINT('Ctrl Pts',(89.5434685595586,51.6482051132515,12.8144361432792));
#76911=CARTESIAN_POINT('Ctrl Pts',(89.5152101476267,51.6436244542874,12.8697218305777));
#76912=CARTESIAN_POINT('Ctrl Pts',(89.4840313941275,51.6390437953233,12.9232942012605));
#76913=CARTESIAN_POINT('Ctrl Pts',(89.4517262586315,51.6342976527779,12.9788019589325));
#76914=CARTESIAN_POINT('Ctrl Pts',(89.4162859747846,51.6295515102325,13.0324697025458));
#76915=CARTESIAN_POINT('Ctrl Pts',(89.3779609977017,51.6248053676871,13.0839353940022));
#76916=CARTESIAN_POINT('Ctrl Pts',(89.3409254422562,51.6202189063563,13.1336695521035));
#76917=CARTESIAN_POINT('Ctrl Pts',(89.3011966246599,51.6156324450255,13.1813471287117));
#76918=CARTESIAN_POINT('Ctrl Pts',(89.2590414409187,51.6110459836947,13.2266754056796));
#76919=CARTESIAN_POINT('Ctrl Pts',(89.2146847589663,51.606220000542,13.2743708914178));
#76920=CARTESIAN_POINT('Ctrl Pts',(89.1676417913895,51.6013940173892,13.319464517301));
#76921=CARTESIAN_POINT('Ctrl Pts',(89.1182648220577,51.5965680342365,13.3616617804943));
#76922=CARTESIAN_POINT('Ctrl Pts',(89.0688878527258,51.5917420510837,13.4038590436876));
#76923=CARTESIAN_POINT('Ctrl Pts',(89.0171774443592,51.586916067931,13.4431596137063));
#76924=CARTESIAN_POINT('Ctrl Pts',(88.963520384612,51.5820900847782,13.479322239441));
#76925=CARTESIAN_POINT('Ctrl Pts',(88.9124067525923,51.5774928607006,13.5137707007131));
#76926=CARTESIAN_POINT('Ctrl Pts',(88.8593170143169,51.572895636623,13.5455134682698));
#76927=CARTESIAN_POINT('Ctrl Pts',(88.804569143224,51.5682984125454,13.5743178877553));
#76928=CARTESIAN_POINT('Ctrl Pts',(88.7488838461878,51.563622472035,13.6036155138181));
#76929=CARTESIAN_POINT('Ctrl Pts',(88.6914834854479,51.5589465315246,13.6298728452724));
#76930=CARTESIAN_POINT('Ctrl Pts',(88.6327347597007,51.5542705910141,13.6528902684748));
#76931=CARTESIAN_POINT('Ctrl Pts',(88.5751339057874,51.5496860121518,13.6754579618924));
#76932=CARTESIAN_POINT('Ctrl Pts',(88.5162374001639,51.5451014332895,13.6949110208099));
#76933=CARTESIAN_POINT('Ctrl Pts',(88.4564146330363,51.5405168544272,13.7111080937972));
#76934=CARTESIAN_POINT('Ctrl Pts',(88.3966284285346,51.535935077579,13.7272952674177));
#76935=CARTESIAN_POINT('Ctrl Pts',(88.3359175753889,51.5313533007309,13.7402302682345));
#76936=CARTESIAN_POINT('Ctrl Pts',(88.2746672929125,51.5267715238828,13.74982136649));
#76937=CARTESIAN_POINT('Ctrl Pts',(88.2134319485466,51.5221908644677,13.7594101256071));
#76938=CARTESIAN_POINT('Ctrl Pts',(88.1516579387086,51.5176102050526,13.7656565224022));
#76939=CARTESIAN_POINT('Ctrl Pts',(88.0897393328737,51.5130295456375,13.7685201769902));
#76940=CARTESIAN_POINT('Ctrl Pts',(88.0255838312244,51.5082834035256,13.7714872850857));
#76941=CARTESIAN_POINT('Ctrl Pts',(87.9612736639141,51.5035372614137,13.7708224680467));
#76942=CARTESIAN_POINT('Ctrl Pts',(87.8972488331793,51.4987911193018,13.7665397694988));
#76943=CARTESIAN_POINT('Ctrl Pts',(87.8353780690605,51.4942046575228,13.7624011590782));
#76944=CARTESIAN_POINT('Ctrl Pts',(87.7737742606188,51.4896181957437,13.7548843942375));
#76945=CARTESIAN_POINT('Ctrl Pts',(87.7128280906952,51.4850317339646,13.7440549300013));
#76946=CARTESIAN_POINT('Ctrl Pts',(87.6486991062743,51.4802057516863,13.7326599146268));
#76947=CARTESIAN_POINT('Ctrl Pts',(87.5852989611591,51.475379769408,13.717596849635));
#76948=CARTESIAN_POINT('Ctrl Pts',(87.523066151467,51.4705537871298,13.6990019580686));
#76949=CARTESIAN_POINT('Ctrl Pts',(87.4608333417749,51.4657278048515,13.6804070665021));
#76950=CARTESIAN_POINT('Ctrl Pts',(87.3997684503712,51.4609018225733,13.6582806418593));
#76951=CARTESIAN_POINT('Ctrl Pts',(87.3402839503183,51.456075840295,13.6328167781522));
#76952=CARTESIAN_POINT('Ctrl Pts',(87.2836191186344,51.4514786179385,13.6085599457052));
#76953=CARTESIAN_POINT('Ctrl Pts',(87.2281555585013,51.4468813955821,13.5811753816928));
#76954=CARTESIAN_POINT('Ctrl Pts',(87.1742611959948,51.4422841732256,13.5508040306626));
#76955=CARTESIAN_POINT('Ctrl Pts',(87.1194439987869,51.4376082325,13.5199126301253));
#76956=CARTESIAN_POINT('Ctrl Pts',(87.06625076872,51.4329322917744,13.4859313155132));
#76957=CARTESIAN_POINT('Ctrl Pts',(87.0150481026579,51.4282563510489,13.4490598879949));
#76958=CARTESIAN_POINT('Ctrl Pts',(86.9648458896195,51.4236717739064,13.4129088942742));
#76959=CARTESIAN_POINT('Ctrl Pts',(86.9165575854691,51.419087196764,13.3739800239028));
#76960=CARTESIAN_POINT('Ctrl Pts',(86.8705022991761,51.4145026196216,13.332506940374));
#76961=CARTESIAN_POINT('Ctrl Pts',(86.8244751610249,51.4099208444882,13.2910592044291));
#76962=CARTESIAN_POINT('Ctrl Pts',(86.7806787120628,51.4053390693548,13.2470706785538));
#76963=CARTESIAN_POINT('Ctrl Pts',(86.7393989587362,51.4007572942213,13.2008152393482));
#76964=CARTESIAN_POINT('Ctrl Pts',(86.6981292729125,51.3961766365131,13.1545710811394));
#76965=CARTESIAN_POINT('Ctrl Pts',(86.659375403062,51.3915959788048,13.1060614867506));
#76966=CARTESIAN_POINT('Ctrl Pts',(86.6233850158349,51.3870153210966,13.0555956200997));
#76967=CARTESIAN_POINT('Ctrl Pts',(86.586094398825,51.3822691773228,13.0033065659844));
#76968=CARTESIAN_POINT('Ctrl Pts',(86.5517711506645,51.3775230335491,12.9489176203987));
#76969=CARTESIAN_POINT('Ctrl Pts',(86.5206421299862,51.3727768897754,12.8928060563928));
#76970=CARTESIAN_POINT('Ctrl Pts',(86.4905604429464,51.368190429664,12.8385823618802));
#76971=CARTESIAN_POINT('Ctrl Pts',(86.463461609385,51.3636039695526,12.7827506368254));
#76972=CARTESIAN_POINT('Ctrl Pts',(86.4395025448572,51.3590175094412,12.7256746046951));
#76973=CARTESIAN_POINT('Ctrl Pts',(86.4142922306473,51.3541915238363,12.6656178064765));
#76974=CARTESIAN_POINT('Ctrl Pts',(86.3925588490335,51.3493655382314,12.604183774149));
#76975=CARTESIAN_POINT('Ctrl Pts',(86.3744257960406,51.3445395526265,12.5418147859562));
#76976=CARTESIAN_POINT('Ctrl Pts',(86.3562927430476,51.3397135670216,12.4794457977634));
#76977=CARTESIAN_POINT('Ctrl Pts',(86.3417600882466,51.3348875814167,12.4161425025795));
#76978=CARTESIAN_POINT('Ctrl Pts',(86.3308884938938,51.3300615958118,12.3523567052638));
#76979=CARTESIAN_POINT('Ctrl Pts',(86.3148742743359,51.3229527587313,12.2583981073123));
#76980=CARTESIAN_POINT('Ctrl Pts',(86.3067391222564,51.3158439216507,12.163059810845));
#76981=CARTESIAN_POINT('Ctrl Pts',(86.3066605745515,51.3087350845701,12.0673994506177));
#76982=CARTESIAN_POINT('',(86.3066600260026,50.5149850846118,12.0662977153839));
#76983=CARTESIAN_POINT('Ctrl Pts',(86.3066605745511,51.3087350845309,12.0673994500905));
#76984=CARTESIAN_POINT('Ctrl Pts',(86.3066106156482,51.3042136305189,12.0065563171497));
#76985=CARTESIAN_POINT('Ctrl Pts',(86.3098229390638,51.2996921765069,11.9455970361689));
#76986=CARTESIAN_POINT('Ctrl Pts',(86.3163083194618,51.2951707224949,11.8849062576601));
#76987=CARTESIAN_POINT('Ctrl Pts',(86.3227871823644,51.2906538123267,11.8242764704651));
#76988=CARTESIAN_POINT('Ctrl Pts',(86.3325325346701,51.2861369021586,11.7639151711377));
#76989=CARTESIAN_POINT('Ctrl Pts',(86.3455031304503,51.2816199919904,11.7042058415065));
#76990=CARTESIAN_POINT('Ctrl Pts',(86.3584657883159,51.2771058461399,11.6445330535706));
#76991=CARTESIAN_POINT('Ctrl Pts',(86.3746496682963,51.2725917002894,11.5855119574642));
#76992=CARTESIAN_POINT('Ctrl Pts',(86.3939621494986,51.268077554439,11.5275174787927));
#76993=CARTESIAN_POINT('Ctrl Pts',(86.4132703985603,51.2635643978192,11.4695357090415));
#76994=CARTESIAN_POINT('Ctrl Pts',(86.4357057221016,51.2590512411994,11.4125806087351));
#76995=CARTESIAN_POINT('Ctrl Pts',(86.4611258432148,51.2545380845797,11.3570113303237));
#76996=CARTESIAN_POINT('Ctrl Pts',(86.4865680009035,51.250021015527,11.3013938791837));
#76997=CARTESIAN_POINT('Ctrl Pts',(86.5149999056639,51.2455039464744,11.2471651287774));
#76998=CARTESIAN_POINT('Ctrl Pts',(86.5462319704495,51.2409868774218,11.1946622611142));
#76999=CARTESIAN_POINT('Ctrl Pts',(86.5774776671001,51.2364678368033,11.1421364775147));
#77000=CARTESIAN_POINT('Ctrl Pts',(86.6115256631514,51.2319487961847,11.091338513034));
#77001=CARTESIAN_POINT('Ctrl Pts',(86.6481431777198,51.2274297555662,11.0425762766262));
#77002=CARTESIAN_POINT('Ctrl Pts',(86.6848270397391,51.2229025268761,10.9937256876876));
#77003=CARTESIAN_POINT('Ctrl Pts',(86.7240893763254,51.2183752981861,10.9469185934149));
#77004=CARTESIAN_POINT('Ctrl Pts',(86.7656580695585,51.2138480694961,10.9024286391097));
#77005=CARTESIAN_POINT('Ctrl Pts',(86.7956545696152,51.2105811634403,10.8703241197457));
#77006=CARTESIAN_POINT('Ctrl Pts',(86.8268512280379,51.2073142573844,10.8394254501484));
#77007=CARTESIAN_POINT('Ctrl Pts',(86.8591352487777,51.2040473513286,10.8098222934268));
#77008=CARTESIAN_POINT('Ctrl Pts',(86.9045656857548,51.1994501243947,10.7681643984389));
#77009=CARTESIAN_POINT('Ctrl Pts',(86.9523521679268,51.1948528974607,10.7288886987404));
#77010=CARTESIAN_POINT('Ctrl Pts',(87.0022148020363,51.1902556705268,10.6922724942809));
#77011=CARTESIAN_POINT('Ctrl Pts',(87.0529311787428,51.1855797303734,10.6550293511518));
#77012=CARTESIAN_POINT('Ctrl Pts',(87.1057951451597,51.18090379022,10.620538059968));
#77013=CARTESIAN_POINT('Ctrl Pts',(87.1604737166441,51.1762278500666,10.5890504826092));
#77014=CARTESIAN_POINT('Ctrl Pts',(87.2140839796211,51.1716432683103,10.5581781087179));
#77015=CARTESIAN_POINT('Ctrl Pts',(87.2694381156879,51.167058686554,10.5301933974363));
#77016=CARTESIAN_POINT('Ctrl Pts',(87.3261918247247,51.1624741047977,10.5052909948757));
#77017=CARTESIAN_POINT('Ctrl Pts',(87.3829108469857,51.1578923250496,10.4804038121848));
#77018=CARTESIAN_POINT('Ctrl Pts',(87.4410272809177,51.1533105453016,10.4585954069282));
#77019=CARTESIAN_POINT('Ctrl Pts',(87.5001738029954,51.1487287655535,10.4400137048382));
#77020=CARTESIAN_POINT('Ctrl Pts',(87.5593059000659,51.1441481032372,10.4214365345649));
#77021=CARTESIAN_POINT('Ctrl Pts',(87.6194671011378,51.139567440921,10.4060846577511));
#77022=CARTESIAN_POINT('Ctrl Pts',(87.6802737041403,51.1349867786048,10.3940565342013));
#77023=CARTESIAN_POINT('Ctrl Pts',(87.7432769532544,51.1302406392915,10.3815938931893));
#77024=CARTESIAN_POINT('Ctrl Pts',(87.8069725695866,51.1254944999782,10.3726999207212));
#77025=CARTESIAN_POINT('Ctrl Pts',(87.8709233462469,51.1207483606649,10.3674260785373));
#77026=CARTESIAN_POINT('Ctrl Pts',(87.9327226229017,51.1161618960153,10.362329664558));
#77027=CARTESIAN_POINT('Ctrl Pts',(87.9947596329381,51.1115754313658,10.3606135911176));
#77028=CARTESIAN_POINT('Ctrl Pts',(88.0566383046152,51.1069889667162,10.3622711539826));
#77029=CARTESIAN_POINT('Ctrl Pts',(88.1217483724266,51.1021629900711,10.3640152772421));
#77030=CARTESIAN_POINT('Ctrl Pts',(88.1866824684781,51.0973370134259,10.3694950077655));
#77031=CARTESIAN_POINT('Ctrl Pts',(88.2509867298057,51.0925110367808,10.37864075991));
#77032=CARTESIAN_POINT('Ctrl Pts',(88.3152909911333,51.0876850601356,10.3877865120545));
#77033=CARTESIAN_POINT('Ctrl Pts',(88.3789647977517,51.0828590834905,10.4005980821477));
#77034=CARTESIAN_POINT('Ctrl Pts',(88.4415714258755,51.0780331068453,10.4169447908516));
#77035=CARTESIAN_POINT('Ctrl Pts',(88.5012103445833,51.0734358934599,10.4325166250287));
#77036=CARTESIAN_POINT('Ctrl Pts',(88.5601258555124,51.0688386800745,10.4513599045846));
#77037=CARTESIAN_POINT('Ctrl Pts',(88.6179331809773,51.0642414666891,10.4733898940956));
#77038=CARTESIAN_POINT('Ctrl Pts',(88.6767304717578,51.0595655248421,10.4957971528427));
#77039=CARTESIAN_POINT('Ctrl Pts',(88.734380726769,51.0548895829952,10.5215012533864));
#77040=CARTESIAN_POINT('Ctrl Pts',(88.7904917387102,51.0502136411482,10.5503590580607));
#77041=CARTESIAN_POINT('Ctrl Pts',(88.8455062724811,51.0456290729547,10.5786529457466));
#77042=CARTESIAN_POINT('Ctrl Pts',(88.8990407051215,51.0410445047613,10.6099781477268));
#77043=CARTESIAN_POINT('Ctrl Pts',(88.9507447637455,51.0364599365678,10.6441509874065));
#77044=CARTESIAN_POINT('Ctrl Pts',(89.0024172221083,51.0318781703507,10.6783029414792));
#77045=CARTESIAN_POINT('Ctrl Pts',(89.0522611008404,51.0272964041336,10.7152988021777));
#77046=CARTESIAN_POINT('Ctrl Pts',(89.0999528899065,51.0227146379165,10.7549102093432));
#77047=CARTESIAN_POINT('Ctrl Pts',(89.1476330481359,51.0181339890778,10.7945119562756));
#77048=CARTESIAN_POINT('Ctrl Pts',(89.193161767169,51.0135533402391,10.8367276583122));
#77049=CARTESIAN_POINT('Ctrl Pts',(89.2362482106196,51.0089726914004,10.8812883650553));
#77050=CARTESIAN_POINT('Ctrl Pts',(89.2808914118443,51.0042265389805,10.9274590962302));
#77051=CARTESIAN_POINT('Ctrl Pts',(89.322912024005,50.9994803865607,10.9761471583441));
#77052=CARTESIAN_POINT('Ctrl Pts',(89.3620296693481,50.9947342341408,11.0270131530471));
#77053=CARTESIAN_POINT('Ctrl Pts',(89.3998310641828,50.9901477826815,11.0761675827823));
#77054=CARTESIAN_POINT('Ctrl Pts',(89.4349215240421,50.9855613312222,11.1273552188832));
#77055=CARTESIAN_POINT('Ctrl Pts',(89.4670918540817,50.9809748797629,11.1802396779733));
#77056=CARTESIAN_POINT('Ctrl Pts',(89.5009424480424,50.9761488768628,11.2358863048274));
#77057=CARTESIAN_POINT('Ctrl Pts',(89.5315591962283,50.9713228739626,11.293411303298));
#77058=CARTESIAN_POINT('Ctrl Pts',(89.5587543818358,50.9664968710625,11.3523956214344));
#77059=CARTESIAN_POINT('Ctrl Pts',(89.5859495674434,50.9616708681624,11.4113799395709));
#77060=CARTESIAN_POINT('Ctrl Pts',(89.6097230252991,50.9568448652623,11.4718229460076));
#77061=CARTESIAN_POINT('Ctrl Pts',(89.6299476630851,50.9520188623621,11.5332868503675));
#77062=CARTESIAN_POINT('Ctrl Pts',(89.64921357763,50.9474216299938,11.5918371364854));
#77063=CARTESIAN_POINT('Ctrl Pts',(89.6653386807364,50.9428243976255,11.6515541042634));
#77064=CARTESIAN_POINT('Ctrl Pts',(89.6781854577588,50.9382271652571,11.7120685305917));
#77065=CARTESIAN_POINT('Ctrl Pts',(89.6912521785553,50.933551225783,11.7736189966437));
#77066=CARTESIAN_POINT('Ctrl Pts',(89.7009270074487,50.9288752863089,11.8359940100405));
#77067=CARTESIAN_POINT('Ctrl Pts',(89.7071174661682,50.9241993468348,11.898786434285));
#77068=CARTESIAN_POINT('Ctrl Pts',(89.7131869835846,50.9196147599146,11.9603521000679));
#77069=CARTESIAN_POINT('Ctrl Pts',(89.7159070005629,50.9150301729943,12.0223184828421));
#77070=CARTESIAN_POINT('Ctrl Pts',(89.7152418402189,50.9104455860741,12.0842916824639));
#77071=CARTESIAN_POINT('Ctrl Pts',(89.7145770864241,50.9058638012758,12.1462270037628));
#77072=CARTESIAN_POINT('Ctrl Pts',(89.7105312633608,50.9012820164775,12.208168625688));
#77073=CARTESIAN_POINT('Ctrl Pts',(89.703120749887,50.8967002316792,12.2697208958398));
#77074=CARTESIAN_POINT('Ctrl Pts',(89.695712043927,50.8921195644336,12.331258152649));
#77075=CARTESIAN_POINT('Ctrl Pts',(89.6849403375673,50.887538897188,12.3924057410408));
#77076=CARTESIAN_POINT('Ctrl Pts',(89.6708738325338,50.8829582299424,12.4527734423014));
#77077=CARTESIAN_POINT('Ctrl Pts',(89.6562992042134,50.8782120956037,12.5153218014233));
#77078=CARTESIAN_POINT('Ctrl Pts',(89.6381872542293,50.8734659612651,12.5770322703839));
#77079=CARTESIAN_POINT('Ctrl Pts',(89.6166710385845,50.8687198269265,12.6374852154264));
#77080=CARTESIAN_POINT('Ctrl Pts',(89.5958786517995,50.8641333577011,12.6959044577488));
#77081=CARTESIAN_POINT('Ctrl Pts',(89.571907694026,50.8595468884757,12.7531489879837));
#77082=CARTESIAN_POINT('Ctrl Pts',(89.5449273008262,50.8549604192503,12.808860600234));
#77083=CARTESIAN_POINT('Ctrl Pts',(89.5165380371022,50.850134452355,12.8674813786989));
#77084=CARTESIAN_POINT('Ctrl Pts',(89.48481672904,50.8453084854598,12.924404189032));
#77085=CARTESIAN_POINT('Ctrl Pts',(89.4500136048722,50.8404825185646,12.9792440421884));
#77086=CARTESIAN_POINT('Ctrl Pts',(89.4152104807044,50.8356565516694,13.0340838953448));
#77087=CARTESIAN_POINT('Ctrl Pts',(89.3773259812303,50.8308305847741,13.0868403101328));
#77088=CARTESIAN_POINT('Ctrl Pts',(89.3366589580983,50.8260046178789,13.1371690634133));
#77089=CARTESIAN_POINT('Ctrl Pts',(89.2979193047422,50.8214073724887,13.18511253962));
#77090=CARTESIAN_POINT('Ctrl Pts',(89.2564959118719,50.8168101270984,13.2310501401612));
#77091=CARTESIAN_POINT('Ctrl Pts',(89.212624387168,50.8122128817082,13.2746660695838));
#77092=CARTESIAN_POINT('Ctrl Pts',(89.1680019001511,50.8075369438618,13.3190285862168));
#77093=CARTESIAN_POINT('Ctrl Pts',(89.1208469412602,50.8028610060155,13.3609887302104));
#77094=CARTESIAN_POINT('Ctrl Pts',(89.0714513947245,50.7981850681691,13.400247981084));
#77095=CARTESIAN_POINT('Ctrl Pts',(89.0230207146095,50.7936004676138,13.438740362563));
#77096=CARTESIAN_POINT('Ctrl Pts',(88.9724366103187,50.7890158670586,13.4746360859703));
#77097=CARTESIAN_POINT('Ctrl Pts',(88.9200106573475,50.7844312665033,13.5076915274873));
#77098=CARTESIAN_POINT('Ctrl Pts',(88.8676167451246,50.7798494678816,13.5407267667758));
#77099=CARTESIAN_POINT('Ctrl Pts',(88.8133836459609,50.7752676692598,13.5709248952249));
#77100=CARTESIAN_POINT('Ctrl Pts',(88.757652642223,50.770685870638,13.5980850718748));
#77101=CARTESIAN_POINT('Ctrl Pts',(88.7019352299095,50.7661051894045,13.6252386248239));
#77102=CARTESIAN_POINT('Ctrl Pts',(88.6447210955907,50.761524508171,13.6493554738316));
#77103=CARTESIAN_POINT('Ctrl Pts',(88.5863750651557,50.7569438269374,13.6702812627457));
#77104=CARTESIAN_POINT('Ctrl Pts',(88.5259217583888,50.752197705809,13.6919628257781));
#77105=CARTESIAN_POINT('Ctrl Pts',(88.4642537550222,50.7474515846805,13.7102181578227));
#77106=CARTESIAN_POINT('Ctrl Pts',(88.4017957626031,50.742705463552,13.7249314354522));
#77107=CARTESIAN_POINT('Ctrl Pts',(88.3414385696333,50.7381189800978,13.7391498261289));
#77108=CARTESIAN_POINT('Ctrl Pts',(88.2803442229204,50.7335324966437,13.750060649943));
#77109=CARTESIAN_POINT('Ctrl Pts',(88.218905399802,50.7289460131895,13.7576117108643));
#77110=CARTESIAN_POINT('Ctrl Pts',(88.1542589064933,50.7241200732239,13.765557006437));
#77111=CARTESIAN_POINT('Ctrl Pts',(88.0892316229153,50.7192941332582,13.7697820481331));
#77112=CARTESIAN_POINT('Ctrl Pts',(88.0242827004128,50.7144681932926,13.7702882401371));
#77113=CARTESIAN_POINT('Ctrl Pts',(87.9593337779103,50.7096422533269,13.7707944321412));
#77114=CARTESIAN_POINT('Ctrl Pts',(87.8944638597993,50.7048163133613,13.7675818837741));
#77115=CARTESIAN_POINT('Ctrl Pts',(87.8301242227846,50.6999903733956,13.7607149579846));
#77116=CARTESIAN_POINT('Ctrl Pts',(87.7688349409761,50.69539323222,13.7541735945359));
#77117=CARTESIAN_POINT('Ctrl Pts',(87.7077751321042,50.6907960910443,13.7442897274374));
#77118=CARTESIAN_POINT('Ctrl Pts',(87.6473378815273,50.6861989498687,13.7310899973239));
#77119=CARTESIAN_POINT('Ctrl Pts',(87.5858645432479,50.6815229989955,13.7176639816345));
#77120=CARTESIAN_POINT('Ctrl Pts',(87.5250358470893,50.6768470481223,13.7008073044624));
#77121=CARTESIAN_POINT('Ctrl Pts',(87.4652609216621,50.6721710972492,13.6806032620972));
#77122=CARTESIAN_POINT('Ctrl Pts',(87.4066551073436,50.6675866012138,13.6607943815863));
#77123=CARTESIAN_POINT('Ctrl Pts',(87.3490627197813,50.6630021051784,13.6377680671013));
#77124=CARTESIAN_POINT('Ctrl Pts',(87.2928574184861,50.6584176091431,13.6116539289947));
#77125=CARTESIAN_POINT('Ctrl Pts',(87.2366864663903,50.6538359148677,13.585555750232));
#77126=CARTESIAN_POINT('Ctrl Pts',(87.1819013804066,50.6492542205924,13.5563737037183));
#77127=CARTESIAN_POINT('Ctrl Pts',(87.1288559908015,50.6446725263171,13.5242855627878));
#77128=CARTESIAN_POINT('Ctrl Pts',(87.0758235340169,50.6400919490895,13.4922052451604));
#77129=CARTESIAN_POINT('Ctrl Pts',(87.0245303669891,50.6355113718619,13.4572205030133));
#77130=CARTESIAN_POINT('Ctrl Pts',(86.9753040373237,50.6309307946342,13.4195541025375));
#77131=CARTESIAN_POINT('Ctrl Pts',(86.9242975627487,50.6261845724907,13.3805255925661));
#77132=CARTESIAN_POINT('Ctrl Pts',(86.8755107748959,50.6214383503473,13.3386180591));
#77133=CARTESIAN_POINT('Ctrl Pts',(86.8292713698261,50.6166921282038,13.2941255148507));
#77134=CARTESIAN_POINT('Ctrl Pts',(86.784589189961,50.6121057467143,13.25113136599));
#77135=CARTESIAN_POINT('Ctrl Pts',(86.7422858376984,50.6075193652249,13.2057239984065));
#77136=CARTESIAN_POINT('Ctrl Pts',(86.7026181382662,50.6029329837355,13.1582049896819));
#77137=CARTESIAN_POINT('Ctrl Pts',(86.6608767416166,50.598106841265,13.1082018430421));
#77138=CARTESIAN_POINT('Ctrl Pts',(86.6220545207183,50.5932806987945,13.0558607267832));
#77139=CARTESIAN_POINT('Ctrl Pts',(86.5863993683685,50.5884545563239,13.0015682102098));
#77140=CARTESIAN_POINT('Ctrl Pts',(86.5507442160188,50.5836284138534,12.9472756936364));
#77141=CARTESIAN_POINT('Ctrl Pts',(86.5182563893731,50.5788022713829,12.8910323767418));
#77142=CARTESIAN_POINT('Ctrl Pts',(86.4891266012826,50.5739761289124,12.8332523664847));
#77143=CARTESIAN_POINT('Ctrl Pts',(86.459454928889,50.569060208554,12.7743975087041));
#77144=CARTESIAN_POINT('Ctrl Pts',(86.433157332778,50.5641442881956,12.7137323715273));
#77145=CARTESIAN_POINT('Ctrl Pts',(86.4104420441128,50.5592283678373,12.6516526832911));
#77146=CARTESIAN_POINT('Ctrl Pts',(86.3878424418835,50.5543374837139,12.589889159995));
#77147=CARTESIAN_POINT('Ctrl Pts',(86.3687889427545,50.5494465995905,12.5267258171671));
#77148=CARTESIAN_POINT('Ctrl Pts',(86.3534411451279,50.5445557154672,12.4625772033731));
#77149=CARTESIAN_POINT('Ctrl Pts',(86.3379755003825,50.5396272769913,12.3979360283986));
#77150=CARTESIAN_POINT('Ctrl Pts',(86.3262729414904,50.5346988385154,12.3322947441721));
#77151=CARTESIAN_POINT('Ctrl Pts',(86.3184469541847,50.5297704000395,12.2660975329719));
#77152=CARTESIAN_POINT('Ctrl Pts',(86.310620966879,50.5248419615636,12.1999003217717));
#77153=CARTESIAN_POINT('Ctrl Pts',(86.3066717033888,50.5199135230877,12.1331475901878));
#77154=CARTESIAN_POINT('Ctrl Pts',(86.3066600260026,50.5149850846118,12.0662977153839));
#77155=CARTESIAN_POINT('',(86.3066605689282,49.7212350845238,12.0646074147082));
#77156=CARTESIAN_POINT('Ctrl Pts',(86.3066600260025,50.5149850845702,12.06629771482));
#77157=CARTESIAN_POINT('Ctrl Pts',(86.3066487968142,50.5102457989619,12.0020135300569));
#77158=CARTESIAN_POINT('Ctrl Pts',(86.3102788918965,50.5055065133535,11.9377784889388));
#77159=CARTESIAN_POINT('Ctrl Pts',(86.3175077249544,50.5007672277452,11.8740136724633));
#77160=CARTESIAN_POINT('Ctrl Pts',(86.3247527769692,50.4960173088482,11.8101057901849));
#77161=CARTESIAN_POINT('Ctrl Pts',(86.3356126403743,50.4912673899512,11.7466706948135));
#77162=CARTESIAN_POINT('Ctrl Pts',(86.3499931349081,50.4865174710542,11.6841217082398));
#77163=CARTESIAN_POINT('Ctrl Pts',(86.3643903902438,50.4817620160159,11.6214998193629));
#77164=CARTESIAN_POINT('Ctrl Pts',(86.3823163239311,50.4770065609776,11.5597665355359));
#77165=CARTESIAN_POINT('Ctrl Pts',(86.4036270091007,50.4722511059393,11.4993193988433));
#77166=CARTESIAN_POINT('Ctrl Pts',(86.4249924565275,50.467483430766,11.4387169306058));
#77167=CARTESIAN_POINT('Ctrl Pts',(86.449759860851,50.4627157555925,11.3794076368747));
#77168=CARTESIAN_POINT('Ctrl Pts',(86.4777373601943,50.4579480804192,11.3217685084759));
#77169=CARTESIAN_POINT('Ctrl Pts',(86.4972709051324,50.4546193484225,11.2815255800086));
#77170=CARTESIAN_POINT('Ctrl Pts',(86.5183682753801,50.4512906164259,11.2420963079173));
#77171=CARTESIAN_POINT('Ctrl Pts',(86.5409516333099,50.4479618844293,11.2036006521386));
#77172=CARTESIAN_POINT('Ctrl Pts',(86.5721417994069,50.4433645298556,11.1504338068234));
#77173=CARTESIAN_POINT('Ctrl Pts',(86.606283984092,50.4387671752819,11.0988521303865));
#77174=CARTESIAN_POINT('Ctrl Pts',(86.6431920725684,50.4341698207082,11.0492029163814));
#77175=CARTESIAN_POINT('Ctrl Pts',(86.680730926981,50.4294938965098,10.9987051882904));
#77176=CARTESIAN_POINT('Ctrl Pts',(86.7211309265507,50.4248179723114,10.950207100825));
#77177=CARTESIAN_POINT('Ctrl Pts',(86.7641477588114,50.420142048113,10.9040471936248));
#77178=CARTESIAN_POINT('Ctrl Pts',(86.8063254783426,50.4155573353616,10.8587877099031));
#77179=CARTESIAN_POINT('Ctrl Pts',(86.851018492454,50.4109726226102,10.8157763956407));
#77180=CARTESIAN_POINT('Ctrl Pts',(86.8979548455414,50.4063879098588,10.7753004533447));
#77181=CARTESIAN_POINT('Ctrl Pts',(86.9448625218334,50.4018059982384,10.7348492407143));
#77182=CARTESIAN_POINT('Ctrl Pts',(86.9940104346816,50.3972240866179,10.6969306602472));
#77183=CARTESIAN_POINT('Ctrl Pts',(87.0450908979768,50.3926421749974,10.6617940171653));
#77184=CARTESIAN_POINT('Ctrl Pts',(87.0961589111338,50.3880613801529,10.6266659381416));
#77185=CARTESIAN_POINT('Ctrl Pts',(87.1491581204776,50.3834805853084,10.594318738798));
#77186=CARTESIAN_POINT('Ctrl Pts',(87.2037506543892,50.3788997904638,10.5649592511824));
#77187=CARTESIAN_POINT('Ctrl Pts',(87.2603122030945,50.3741537779207,10.5345408410126));
#77188=CARTESIAN_POINT('Ctrl Pts',(87.318583726246,50.3694077653775,10.5073301125322));
#77189=CARTESIAN_POINT('Ctrl Pts',(87.3781624688156,50.3646617528344,10.4835046620213));
#77190=CARTESIAN_POINT('Ctrl Pts',(87.4357400024264,50.3600751555862,10.4604794919955));
#77191=CARTESIAN_POINT('Ctrl Pts',(87.4945378015802,50.355488558338,10.4406158728676));
#77192=CARTESIAN_POINT('Ctrl Pts',(87.5541752808107,50.3509019610898,10.424023748181));
#77193=CARTESIAN_POINT('Ctrl Pts',(87.6169219690562,50.3460762408991,10.4065665905601));
#77194=CARTESIAN_POINT('Ctrl Pts',(87.680597661316,50.3412505207085,10.3927315331494));
#77195=CARTESIAN_POINT('Ctrl Pts',(87.7447481675762,50.3364248005179,10.3825853756929));
#77196=CARTESIAN_POINT('Ctrl Pts',(87.8088986738363,50.3315990803272,10.3724392182365));
#77197=CARTESIAN_POINT('Ctrl Pts',(87.8735233419441,50.3267733601366,10.3659819481964));
#77198=CARTESIAN_POINT('Ctrl Pts',(87.9381664171364,50.321947639946,10.3632169531008));
#77199=CARTESIAN_POINT('Ctrl Pts',(87.9997399437425,50.3173510670004,10.3605832526065));
#77200=CARTESIAN_POINT('Ctrl Pts',(88.061583113388,50.3127544940547,10.3612882410334));
#77201=CARTESIAN_POINT('Ctrl Pts',(88.1233033296202,50.3081579211091,10.3653640019816));
#77202=CARTESIAN_POINT('Ctrl Pts',(88.1860903420984,50.3034818992072,10.3695102099687));
#77203=CARTESIAN_POINT('Ctrl Pts',(88.2487495844209,50.2988058773052,10.3771449384457));
#77204=CARTESIAN_POINT('Ctrl Pts',(88.310864002806,50.2941298554033,10.3882466166265));
#77205=CARTESIAN_POINT('Ctrl Pts',(88.3717550718666,50.2895459281934,10.3991296462092));
#77206=CARTESIAN_POINT('Ctrl Pts',(88.4321220576025,50.2849620009836,10.413344206161));
#77207=CARTESIAN_POINT('Ctrl Pts',(88.4915762679907,50.2803780737737,10.4308176596342));
#77208=CARTESIAN_POINT('Ctrl Pts',(88.5509941564265,50.275796946991,10.4482804381706));
#77209=CARTESIAN_POINT('Ctrl Pts',(88.6094998876824,50.2712158202084,10.4689980192556));
#77210=CARTESIAN_POINT('Ctrl Pts',(88.66671722287,50.2666346934257,10.4928471913919));
#77211=CARTESIAN_POINT('Ctrl Pts',(88.7239206342945,50.2620546814541,10.5166905598636));
#77212=CARTESIAN_POINT('Ctrl Pts',(88.7798358022469,50.2574746694826,10.5436638107564));
#77213=CARTESIAN_POINT('Ctrl Pts',(88.8341057955293,50.2528946575111,10.5735953347145));
#77214=CARTESIAN_POINT('Ctrl Pts',(88.8903517785809,50.2481478856737,10.6046166761119));
#77215=CARTESIAN_POINT('Ctrl Pts',(88.9448299322576,50.2434011138363,10.6388156448567));
#77216=CARTESIAN_POINT('Ctrl Pts',(88.997172346362,50.238654341999,10.6759500228874));
#77217=CARTESIAN_POINT('Ctrl Pts',(89.0477400437914,50.2340685137344,10.7118253263981));
#77218=CARTESIAN_POINT('Ctrl Pts',(89.0963141523153,50.2294826854698,10.7504397723638));
#77219=CARTESIAN_POINT('Ctrl Pts',(89.1425959842488,50.2248968572052,10.7915333021095));
#77220=CARTESIAN_POINT('Ctrl Pts',(89.1913142670116,50.2200696135814,10.8347901508174));
#77221=CARTESIAN_POINT('Ctrl Pts',(89.2374917905969,50.2152423699577,10.8807938651008));
#77222=CARTESIAN_POINT('Ctrl Pts',(89.2808257891941,50.210415126334,10.9291986538108));
#77223=CARTESIAN_POINT('Ctrl Pts',(89.3241597877912,50.2055878827102,10.9776034425208));
#77224=CARTESIAN_POINT('Ctrl Pts',(89.3646499174546,50.2007606390865,11.0284087492997));
#77225=CARTESIAN_POINT('Ctrl Pts',(89.4020459495463,50.1959333954627,11.0812330215473));
#77226=CARTESIAN_POINT('Ctrl Pts',(89.4376669307682,50.1913352831803,11.1315499216178));
#77227=CARTESIAN_POINT('Ctrl Pts',(89.4706273049234,50.1867371708979,11.1839051611084));
#77228=CARTESIAN_POINT('Ctrl Pts',(89.5006871383485,50.1821390586154,11.2379860717119));
#77229=CARTESIAN_POINT('Ctrl Pts',(89.5312550424806,50.1774632291306,11.2929810567915));
#77230=CARTESIAN_POINT('Ctrl Pts',(89.558823061198,50.1727873996458,11.3497602120251));
#77231=CARTESIAN_POINT('Ctrl Pts',(89.5831833051602,50.168111570161,11.4079616344198));
#77232=CARTESIAN_POINT('Ctrl Pts',(89.6070727119168,50.1635261155711,11.4650381339636));
#77233=CARTESIAN_POINT('Ctrl Pts',(89.6278770357406,50.1589406609812,11.5234819186271));
#77234=CARTESIAN_POINT('Ctrl Pts',(89.6454464357721,50.1543552063913,11.5829268335005));
#77235=CARTESIAN_POINT('Ctrl Pts',(89.6630050729331,50.1497725608134,11.642335332906));
#77236=CARTESIAN_POINT('Ctrl Pts',(89.6773325718359,50.1451899152354,11.7027432594939));
#77237=CARTESIAN_POINT('Ctrl Pts',(89.6883283361337,50.1406072696574,11.7637674928092));
#77238=CARTESIAN_POINT('Ctrl Pts',(89.6993213992027,50.1360257498561,11.8247767348592));
#77239=CARTESIAN_POINT('Ctrl Pts',(89.7069842622872,50.1314442300548,11.8864014825308));
#77240=CARTESIAN_POINT('Ctrl Pts',(89.7112674612321,50.1268627102534,11.9482485844018));
#77241=CARTESIAN_POINT('Ctrl Pts',(89.7157037728269,50.1221174136473,12.012306551045));
#77242=CARTESIAN_POINT('Ctrl Pts',(89.7165141093847,50.1173721170411,12.0766024957849));
#77243=CARTESIAN_POINT('Ctrl Pts',(89.7137023404252,50.112626820435,12.1406965562169));
#77244=CARTESIAN_POINT('Ctrl Pts',(89.7109841953776,50.1080395287142,12.2026564666653));
#77245=CARTESIAN_POINT('Ctrl Pts',(89.7048815061111,50.1034522369935,12.2644272088208));
#77246=CARTESIAN_POINT('Ctrl Pts',(89.6954506739318,50.0988649452727,12.3256165685985));
#77247=CARTESIAN_POINT('Ctrl Pts',(89.6855325877313,50.0940406462239,12.3899673420278));
#77248=CARTESIAN_POINT('Ctrl Pts',(89.6719332443629,50.089216347175,12.4536743970219));
#77249=CARTESIAN_POINT('Ctrl Pts',(89.654778475292,50.0843920481261,12.5162967463427));
#77250=CARTESIAN_POINT('Ctrl Pts',(89.637623706221,50.0795677490773,12.5789190956634));
#77251=CARTESIAN_POINT('Ctrl Pts',(89.6169137902823,50.0747434500284,12.6404561514783));
#77252=CARTESIAN_POINT('Ctrl Pts',(89.5928329021536,50.0699191509795,12.7004915328548));
#77253=CARTESIAN_POINT('Ctrl Pts',(89.5698820994029,50.0653212501343,12.7577095303252));
#77254=CARTESIAN_POINT('Ctrl Pts',(89.5437758042981,50.0607233492891,12.8137977326738));
#77255=CARTESIAN_POINT('Ctrl Pts',(89.5146466153835,50.0561254484439,12.8683850021316));
#77256=CARTESIAN_POINT('Ctrl Pts',(89.4850235558929,50.0514495925294,12.9238977709671));
#77257=CARTESIAN_POINT('Ctrl Pts',(89.4522742532069,50.0467737366149,12.9778577101907));
#77258=CARTESIAN_POINT('Ctrl Pts',(89.4165900779081,50.0420978807004,13.0298938574792));
#77259=CARTESIAN_POINT('Ctrl Pts',(89.381597103485,50.0375125959054,13.0809220669277));
#77260=CARTESIAN_POINT('Ctrl Pts',(89.3437822413148,50.0329273111103,13.1300999082551));
#77261=CARTESIAN_POINT('Ctrl Pts',(89.3033718855931,50.0283420263153,13.1771029407434));
#77262=CARTESIAN_POINT('Ctrl Pts',(89.2629861465548,50.0237595347276,13.2240773405024));
#77263=CARTESIAN_POINT('Ctrl Pts',(89.220008380139,50.01917704314,13.2688791733253));
#77264=CARTESIAN_POINT('Ctrl Pts',(89.1747059368798,50.0145945515523,13.3112161772442));
#77265=CARTESIAN_POINT('Ctrl Pts',(89.1294144657396,50.0100131698307,13.3535429272649));
#77266=CARTESIAN_POINT('Ctrl Pts',(89.0817998070938,50.0054317881091,13.3934056861967));
#77267=CARTESIAN_POINT('Ctrl Pts',(89.0321654642234,50.0008504063874,13.4305497170413));
#77268=CARTESIAN_POINT('Ctrl Pts',(88.9807535278566,49.9961049480632,13.46902401608));
#77269=CARTESIAN_POINT('Ctrl Pts',(88.9271749221276,49.9913594897389,13.5045807549041));
#77270=CARTESIAN_POINT('Ctrl Pts',(88.8718013827731,49.9866140314147,13.5369846413257));
#77271=CARTESIAN_POINT('Ctrl Pts',(88.818274586487,49.9820268371705,13.5683078373428));
#77272=CARTESIAN_POINT('Ctrl Pts',(88.7630712069238,49.9774396429263,13.5966850075563));
#77273=CARTESIAN_POINT('Ctrl Pts',(88.7065513627189,49.9728524486821,13.6219508788583));
#77274=CARTESIAN_POINT('Ctrl Pts',(88.6471065079281,49.9680278583178,13.6485243075688));
#77275=CARTESIAN_POINT('Ctrl Pts',(88.5862058221421,49.9632032679535,13.6716554140613));
#77276=CARTESIAN_POINT('Ctrl Pts',(88.5242881493081,49.9583786775892,13.69121078983));
#77277=CARTESIAN_POINT('Ctrl Pts',(88.4623704764741,49.9535540872249,13.7107661655987));
#77278=CARTESIAN_POINT('Ctrl Pts',(88.3994364620039,49.9487294968606,13.7267457263269));
#77279=CARTESIAN_POINT('Ctrl Pts',(88.3359359037635,49.9439049064963,13.739078448264));
#77280=CARTESIAN_POINT('Ctrl Pts',(88.275493887077,49.9393126953507,13.7508171574307));
#77281=CARTESIAN_POINT('Ctrl Pts',(88.2142892124175,49.9347204842051,13.7593007386264));
#77282=CARTESIAN_POINT('Ctrl Pts',(88.152704642768,49.9301282730595,13.7644388802127));
#77283=CARTESIAN_POINT('Ctrl Pts',(88.0899888039669,49.9254517059325,13.7696714061732));
#77284=CARTESIAN_POINT('Ctrl Pts',(88.0268794771053,49.9207751388056,13.771434151298));
#77285=CARTESIAN_POINT('Ctrl Pts',(87.96379294189,49.9160985716787,13.7696861005668));
#77286=CARTESIAN_POINT('Ctrl Pts',(87.9020151183292,49.911519018564,13.7679743126349));
#77287=CARTESIAN_POINT('Ctrl Pts',(87.8402596861978,49.9069394654494,13.7628960104431));
#77288=CARTESIAN_POINT('Ctrl Pts',(87.778921210903,49.9023599123347,13.7544650636751));
#77289=CARTESIAN_POINT('Ctrl Pts',(87.717620147725,49.8977831524225,13.7460392591863));
#77290=CARTESIAN_POINT('Ctrl Pts',(87.6567360416306,49.8932063925102,13.7342649337972));
#77291=CARTESIAN_POINT('Ctrl Pts',(87.5966586802207,49.888629632598,13.7192078230893));
#77292=CARTESIAN_POINT('Ctrl Pts',(87.5365957676149,49.8840539734116,13.7041543336663));
#77293=CARTESIAN_POINT('Ctrl Pts',(87.4773397093041,49.8794783142252,13.6858197501331));
#77294=CARTESIAN_POINT('Ctrl Pts',(87.4192683985301,49.8749026550389,13.6643205396359));
#77295=CARTESIAN_POINT('Ctrl Pts',(87.3589717827859,49.8701516556201,13.6419974748233));
#77296=CARTESIAN_POINT('Ctrl Pts',(87.2999531278244,49.8654006562012,13.6162624728202));
#77297=CARTESIAN_POINT('Ctrl Pts',(87.2426137837962,49.8606496567824,13.5873012385284));
#77298=CARTESIAN_POINT('Ctrl Pts',(87.1873193869315,49.8560680967416,13.5593728760791));
#77299=CARTESIAN_POINT('Ctrl Pts',(87.1335869555861,49.8514865367007,13.5284448610906));
#77300=CARTESIAN_POINT('Ctrl Pts',(87.0817498541583,49.8469049766599,13.4947298562196));
#77301=CARTESIAN_POINT('Ctrl Pts',(87.0298755271838,49.8423201264837,13.4609906397424));
#77302=CARTESIAN_POINT('Ctrl Pts',(86.9798996477705,49.8377352763076,13.4244607546482));
#77303=CARTESIAN_POINT('Ctrl Pts',(86.9321238428729,49.8331504261314,13.3853942068929));
#77304=CARTESIAN_POINT('Ctrl Pts',(86.884267715068,49.8285578676917,13.3462619786389));
#77305=CARTESIAN_POINT('Ctrl Pts',(86.838619409982,49.823965309252,13.3045849297218));
#77306=CARTESIAN_POINT('Ctrl Pts',(86.7954439568676,49.8193727508123,13.2606540677553));
#77307=CARTESIAN_POINT('Ctrl Pts',(86.7907994973359,49.8188787212126,13.2559283475629));
#77308=CARTESIAN_POINT('Ctrl Pts',(86.7861836137786,49.8183846916129,13.2511765776306));
#77309=CARTESIAN_POINT('Ctrl Pts',(86.7815966074234,49.8178906620131,13.2463991417826));
#77310=CARTESIAN_POINT('Ctrl Pts',(86.7393784611865,49.8133436846882,13.2024283099049));
#77311=CARTESIAN_POINT('Ctrl Pts',(86.6994265036506,49.8087967073632,13.1560896518755));
#77312=CARTESIAN_POINT('Ctrl Pts',(86.6620215912074,49.8042497300383,13.1076487355204));
#77313=CARTESIAN_POINT('Ctrl Pts',(86.6246693612079,49.7997091568421,13.0592760451198));
#77314=CARTESIAN_POINT('Ctrl Pts',(86.5898573866485,49.795168583646,13.008807368977));
#77315=CARTESIAN_POINT('Ctrl Pts',(86.5578291487055,49.7906280104498,12.9565443911159));
#77316=CARTESIAN_POINT('Ctrl Pts',(86.5258336294948,49.7860920757167,12.9043348029664));
#77317=CARTESIAN_POINT('Ctrl Pts',(86.4966164826327,49.7815561409836,12.8503349873008));
#77318=CARTESIAN_POINT('Ctrl Pts',(86.4703790443116,49.7770202062506,12.7948771545973));
#77319=CARTESIAN_POINT('Ctrl Pts',(86.4434889842422,49.7723714461105,12.7380398812909));
#77320=CARTESIAN_POINT('Ctrl Pts',(86.4197291914862,49.7677226859705,12.6796715411922));
#77321=CARTESIAN_POINT('Ctrl Pts',(86.3992664835047,49.7630739258305,12.6201569339147));
#77322=CARTESIAN_POINT('Ctrl Pts',(86.3793118303186,49.7585405866251,12.5621199747398));
#77323=CARTESIAN_POINT('Ctrl Pts',(86.3624925481563,49.7540072474198,12.5029935460392));
#77324=CARTESIAN_POINT('Ctrl Pts',(86.3489136999958,49.7494739082145,12.4431524452241));
#77325=CARTESIAN_POINT('Ctrl Pts',(86.3348162661056,49.7447674376071,12.3810259708212));
#77326=CARTESIAN_POINT('Ctrl Pts',(86.3242119685148,49.7400609669997,12.3181297082135));
#77327=CARTESIAN_POINT('Ctrl Pts',(86.3171600745083,49.7353544963923,12.2548945272111));
#77328=CARTESIAN_POINT('Ctrl Pts',(86.3101081805018,49.730648025785,12.1916593462086));
#77329=CARTESIAN_POINT('Ctrl Pts',(86.3066087018371,49.7259415551776,12.1280858736035));
#77330=CARTESIAN_POINT('Ctrl Pts',(86.3066605689277,49.7212350845702,12.0646074153347));
#77331=CARTESIAN_POINT('',(87.4571200021394,49.5646,10.4541712921126));
#77332=CARTESIAN_POINT('Ctrl Pts',(86.3066605689282,49.7212350845237,12.0646074147082));
#77333=CARTESIAN_POINT('Ctrl Pts',(86.3067280594444,49.7151109317192,11.9820079870988));
#77334=CARTESIAN_POINT('Ctrl Pts',(86.3128039761533,49.7089867789146,11.8996672994486));
#77335=CARTESIAN_POINT('Ctrl Pts',(86.3247540055513,49.70286262611,11.8183121282626));
#77336=CARTESIAN_POINT('Ctrl Pts',(86.3318997838979,49.6992005565833,11.7696640453768));
#77337=CARTESIAN_POINT('Ctrl Pts',(86.3411450603446,49.6955384870566,11.7213677890819));
#77338=CARTESIAN_POINT('Ctrl Pts',(86.352453256211,49.6918764175298,11.6735748042403));
#77339=CARTESIAN_POINT('Ctrl Pts',(86.3666577103926,49.6872764177229,11.6135410666397));
#77340=CARTESIAN_POINT('Ctrl Pts',(86.3841544769797,49.682676417916,11.5541587182232));
#77341=CARTESIAN_POINT('Ctrl Pts',(86.4048668634738,49.6780764181091,11.4958147815381));
#77342=CARTESIAN_POINT('Ctrl Pts',(86.4259196253528,49.6734008245648,11.4365120543286));
#77343=CARTESIAN_POINT('Ctrl Pts',(86.4502946188797,49.6687252310205,11.3782827131778));
#77344=CARTESIAN_POINT('Ctrl Pts',(86.4778572181742,49.6640496374763,11.3215216281614));
#77345=CARTESIAN_POINT('Ctrl Pts',(86.5049010407252,49.659462046851,11.2658288869006));
#77346=CARTESIAN_POINT('Ctrl Pts',(86.5350132812281,49.6548744562257,11.2115500870572));
#77347=CARTESIAN_POINT('Ctrl Pts',(86.5680176299229,49.6502868656004,11.1590398491407));
#77348=CARTESIAN_POINT('Ctrl Pts',(86.6010023848879,49.6457019984954,11.1065607850378));
#77349=CARTESIAN_POINT('Ctrl Pts',(86.6368755734356,49.6411171313903,11.0558486302588));
#77350=CARTESIAN_POINT('Ctrl Pts',(86.6754156395653,49.6365322642853,11.0072322012063));
#77351=CARTESIAN_POINT('Ctrl Pts',(86.7139469229305,49.63194844201,10.9586268511866));
#77352=CARTESIAN_POINT('Ctrl Pts',(86.7551435616937,49.6273646197347,10.9121166767737));
#77353=CARTESIAN_POINT('Ctrl Pts',(86.798742713684,49.6227807974595,10.8679987031002));
#77354=CARTESIAN_POINT('Ctrl Pts',(86.8438579691743,49.6180375787584,10.822346584581));
#77355=CARTESIAN_POINT('Ctrl Pts',(86.8915455481405,49.6132943600573,10.7792565633214));
#77356=CARTESIAN_POINT('Ctrl Pts',(86.9414732651338,49.6085511413563,10.7390156749206));
#77357=CARTESIAN_POINT('Ctrl Pts',(86.9897857092911,49.6039613763435,10.7000766688778));
#77358=CARTESIAN_POINT('Ctrl Pts',(87.0401950753472,49.5993716113308,10.6638054910064));
#77359=CARTESIAN_POINT('Ctrl Pts',(87.0923693508009,49.5947818463181,10.6304190841503));
#77360=CARTESIAN_POINT('Ctrl Pts',(87.1471602095597,49.5899619007728,10.5953583212242));
#77361=CARTESIAN_POINT('Ctrl Pts',(87.203897118866,49.5851419552276,10.5634796281792));
#77362=CARTESIAN_POINT('Ctrl Pts',(87.2621673652706,49.5803220096824,10.5349792552796));
#77363=CARTESIAN_POINT('Ctrl Pts',(87.3204376116753,49.5755020641371,10.50647888238));
#77364=CARTESIAN_POINT('Ctrl Pts',(87.3802405748965,49.5706821185919,10.4813570068324));
#77365=CARTESIAN_POINT('Ctrl Pts',(87.4411435901739,49.5658621730467,10.4597501726755));
#77366=CARTESIAN_POINT('Ctrl Pts',(87.4464597044757,49.5654414486978,10.4578641511122));
#77367=CARTESIAN_POINT('Ctrl Pts',(87.4517852306617,49.5650207243489,10.4560045037934));
#77368=CARTESIAN_POINT('Ctrl Pts',(87.4571200021394,49.5646,10.4541712921126));
#77369=CARTESIAN_POINT('',(86.3679792906019,49.5646,11.6129461576271));
#77370=CARTESIAN_POINT('Origin',(88.011,49.5646,12.066));
#77371=CARTESIAN_POINT('',(86.3092266939895,49.5985899145734,12.0662160011593));
#77372=CARTESIAN_POINT('Ctrl Pts',(86.3679792906019,49.5646,11.6129461576271));
#77373=CARTESIAN_POINT('Ctrl Pts',(86.3470351830164,49.5704400412141,11.6889009322794));
#77374=CARTESIAN_POINT('Ctrl Pts',(86.3313737199885,49.5762800824281,11.7662671947601));
#77375=CARTESIAN_POINT('Ctrl Pts',(86.3211280276762,49.5821201236421,11.8443977600419));
#77376=CARTESIAN_POINT('Ctrl Pts',(86.3114965890295,49.5876100404708,11.9178442117801));
#77377=CARTESIAN_POINT('Ctrl Pts',(86.3066506132027,49.5930999572995,11.9919661813803));
#77378=CARTESIAN_POINT('Ctrl Pts',(86.3066600136595,49.5985898741282,12.0662157799485));
#77379=CARTESIAN_POINT('',(86.3073293460377,50.3923399468998,12.0666353777397));
#77380=CARTESIAN_POINT('Ctrl Pts',(86.3092810471104,49.5985899154299,12.0662160058438));
#77381=CARTESIAN_POINT('Ctrl Pts',(86.3121893889261,49.629264691781,12.4804454596203));
#77382=CARTESIAN_POINT('Ctrl Pts',(86.6701468888325,49.7019442162931,13.4633634721033));
#77383=CARTESIAN_POINT('Ctrl Pts',(88.3227306481849,49.8166284889665,14.0573743541845));
#77384=CARTESIAN_POINT('Ctrl Pts',(89.8516815299995,49.9426427334496,12.8834028378848));
#77385=CARTESIAN_POINT('Ctrl Pts',(89.696794108141,50.0686569779329,10.9633757853075));
#77386=CARTESIAN_POINT('Ctrl Pts',(87.9986885115237,50.1946712224162,10.0514601738819));
#77387=CARTESIAN_POINT('Ctrl Pts',(86.5545658312753,50.3025655349151,10.8497041618736));
#77388=CARTESIAN_POINT('Ctrl Pts',(86.310277298106,50.368455099253,11.7432630818391));
#77389=CARTESIAN_POINT('Ctrl Pts',(86.3092109631531,50.3923399154298,12.0666342497661));
#77390=CARTESIAN_POINT('',(86.3066604225581,51.1860899153758,12.0672001521734));
#77391=CARTESIAN_POINT('Ctrl Pts',(86.306660118584,50.3923399580925,12.0666357789217));
#77392=CARTESIAN_POINT('Ctrl Pts',(86.3066852637277,50.3973113147805,12.1340426553562));
#77393=CARTESIAN_POINT('Ctrl Pts',(86.3107135546021,50.4022826714685,12.2013277506436));
#77394=CARTESIAN_POINT('Ctrl Pts',(86.3186766764168,50.4072540281564,12.26803119575));
#77395=CARTESIAN_POINT('Ctrl Pts',(86.3266622759845,50.4122394176485,12.3349229267581));
#77396=CARTESIAN_POINT('Ctrl Pts',(86.3386048135703,50.4172248071405,12.4012293743328));
#77397=CARTESIAN_POINT('Ctrl Pts',(86.354385126363,50.4222101966325,12.4665021798249));
#77398=CARTESIAN_POINT('Ctrl Pts',(86.3702327072629,50.4272168377765,12.5320532293634));
#77399=CARTESIAN_POINT('Ctrl Pts',(86.3899506940518,50.4322234789205,12.5965614717567));
#77400=CARTESIAN_POINT('Ctrl Pts',(86.4133699848707,50.4372301200645,12.6595934386076));
#77401=CARTESIAN_POINT('Ctrl Pts',(86.4281351142681,50.4403866505038,12.6993331196222));
#77402=CARTESIAN_POINT('Ctrl Pts',(86.4443705175168,50.4435431809432,12.738486425967));
#77403=CARTESIAN_POINT('Ctrl Pts',(86.4620244619462,50.4466997113825,12.7769497999936));
#77404=CARTESIAN_POINT('Ctrl Pts',(86.4877325305886,50.4512963215923,12.8329610253403));
#77405=CARTESIAN_POINT('Ctrl Pts',(86.5165354926491,50.455892931802,12.8876913198559));
#77406=CARTESIAN_POINT('Ctrl Pts',(86.5482830806852,50.4604895420117,12.940776571217));
#77407=CARTESIAN_POINT('Ctrl Pts',(86.580579112399,50.4651655592556,12.9947788771415));
#77408=CARTESIAN_POINT('Ctrl Pts',(86.615922338754,50.4698415764995,13.0470782417727));
#77409=CARTESIAN_POINT('Ctrl Pts',(86.6541035914268,50.4745175937435,13.0973132269109));
#77410=CARTESIAN_POINT('Ctrl Pts',(86.6915330282512,50.4791015369032,13.1465590496897));
#77411=CARTESIAN_POINT('Ctrl Pts',(86.7316894162553,50.483685480063,13.1938206290306));
#77412=CARTESIAN_POINT('Ctrl Pts',(86.774331041167,50.4882694232228,13.2387850279821));
#77413=CARTESIAN_POINT('Ctrl Pts',(86.8169465414334,50.4928505580025,13.2837218792269));
#77414=CARTESIAN_POINT('Ctrl Pts',(86.8620439098941,50.4974316927822,13.3263639719743));
#77415=CARTESIAN_POINT('Ctrl Pts',(86.9093420809422,50.5020128275619,13.3664324915109));
#77416=CARTESIAN_POINT('Ctrl Pts',(86.9566286600696,50.5065928395888,13.4064911909827));
#77417=CARTESIAN_POINT('Ctrl Pts',(87.006114582701,50.5111728516158,13.4439772403373));
#77418=CARTESIAN_POINT('Ctrl Pts',(87.0574844918447,50.5157528636428,13.4786510578722));
#77419=CARTESIAN_POINT('Ctrl Pts',(87.110724638286,50.520499621328,13.5145872538671));
#77420=CARTESIAN_POINT('Ctrl Pts',(87.1659881523694,50.5252463790133,13.5475021178737));
#77421=CARTESIAN_POINT('Ctrl Pts',(87.2228918182155,50.5299931366985,13.5771784571666));
#77422=CARTESIAN_POINT('Ctrl Pts',(87.2778660422669,50.5345789453038,13.6058485560266));
#77423=CARTESIAN_POINT('Ctrl Pts',(87.3343704549797,50.539164753909,13.6314960940994));
#77424=CARTESIAN_POINT('Ctrl Pts',(87.3920374879344,50.5437505625142,13.6539736283256));
#77425=CARTESIAN_POINT('Ctrl Pts',(87.4527404486939,50.5485777947395,13.6776345106043));
#77426=CARTESIAN_POINT('Ctrl Pts',(87.5147312163883,50.5534050269647,13.6977821803525));
#77427=CARTESIAN_POINT('Ctrl Pts',(87.5775640365029,50.55823225919,13.7143046141862));
#77428=CARTESIAN_POINT('Ctrl Pts',(87.6403968566176,50.5630594914153,13.7308270480198));
#77429=CARTESIAN_POINT('Ctrl Pts',(87.7040710771906,50.5678867236405,13.743724193095));
#77430=CARTESIAN_POINT('Ctrl Pts',(87.7681330346237,50.5727139558658,13.7529470865231));
#77431=CARTESIAN_POINT('Ctrl Pts',(87.829144338054,50.5773113135149,13.76173078237));
#77432=CARTESIAN_POINT('Ctrl Pts',(87.8907579602646,50.5819086711641,13.7672183676022));
#77433=CARTESIAN_POINT('Ctrl Pts',(87.9525863601549,50.5865060288132,13.769338686897));
#77434=CARTESIAN_POINT('Ctrl Pts',(88.0154713713922,50.5911819526272,13.7714952412137));
#77435=CARTESIAN_POINT('Ctrl Pts',(88.0785780588376,50.5958578764412,13.7701681896364));
#77436=CARTESIAN_POINT('Ctrl Pts',(88.141489423131,50.6005338002552,13.7653373255628));
#77437=CARTESIAN_POINT('Ctrl Pts',(88.2031736195302,50.6051185141003,13.7606006937691));
#77438=CARTESIAN_POINT('Ctrl Pts',(88.2646695126617,50.6097032279454,13.7524957559121));
#77439=CARTESIAN_POINT('Ctrl Pts',(88.3255829859497,50.6142879417905,13.7410559335589));
#77440=CARTESIAN_POINT('Ctrl Pts',(88.3864592330113,50.6188698537662,13.7296231024574));
#77441=CARTESIAN_POINT('Ctrl Pts',(88.4467532667713,50.6234517657419,13.7148595218008));
#77442=CARTESIAN_POINT('Ctrl Pts',(88.5060783046827,50.6280336777176,13.6968501794563));
#77443=CARTESIAN_POINT('Ctrl Pts',(88.565388873419,50.6326144721806,13.6788452295291));
#77444=CARTESIAN_POINT('Ctrl Pts',(88.6237304286219,50.6371952666436,13.657596237216));
#77445=CARTESIAN_POINT('Ctrl Pts',(88.6807305571034,50.6417760611065,13.6332382768686));
#77446=CARTESIAN_POINT('Ctrl Pts',(88.73978652946,50.6465220727101,13.6080017893157));
#77447=CARTESIAN_POINT('Ctrl Pts',(88.7974019023001,50.6512680843136,13.5794279517199));
#77448=CARTESIAN_POINT('Ctrl Pts',(88.853186642118,50.6560140959171,13.5477207886231));
#77449=CARTESIAN_POINT('Ctrl Pts',(88.9070975956646,50.6606006909595,13.5170786559829));
#77450=CARTESIAN_POINT('Ctrl Pts',(88.9592985498954,50.6651872860019,13.4835107147741));
#77451=CARTESIAN_POINT('Ctrl Pts',(89.0094661784179,50.6697738810443,13.4472458601406));
#77452=CARTESIAN_POINT('Ctrl Pts',(89.0622493258862,50.6745996009284,13.40909031589));
#77453=CARTESIAN_POINT('Ctrl Pts',(89.1127808199414,50.6794253208125,13.3679493471259));
#77454=CARTESIAN_POINT('Ctrl Pts',(89.1607251442831,50.6842510406966,13.324136291585));
#77455=CARTESIAN_POINT('Ctrl Pts',(89.2086694686247,50.6890767605807,13.2803232360441));
#77456=CARTESIAN_POINT('Ctrl Pts',(89.2540262262617,50.6939024804649,13.2338386112796));
#77457=CARTESIAN_POINT('Ctrl Pts',(89.2965084889806,50.698728200349,13.1850365321824));
#77458=CARTESIAN_POINT('Ctrl Pts',(89.3369799397171,50.7033255045427,13.1385444007935));
#77459=CARTESIAN_POINT('Ctrl Pts',(89.3750090047662,50.7079228087365,13.0897584870719));
#77460=CARTESIAN_POINT('Ctrl Pts',(89.4103257087688,50.7125201129303,13.0389657734878));
#77461=CARTESIAN_POINT('Ctrl Pts',(89.4462464236706,50.7171960434262,12.9873043674968));
#77462=CARTESIAN_POINT('Ctrl Pts',(89.4793607081385,50.7218719739221,12.9335672105246));
#77463=CARTESIAN_POINT('Ctrl Pts',(89.5094254032387,50.726547904418,12.8780936808823));
#77464=CARTESIAN_POINT('Ctrl Pts',(89.538903282671,50.7311325680886,12.8237029074841));
#77465=CARTESIAN_POINT('Ctrl Pts',(89.5654492955193,50.7357172317592,12.7676434039417));
#77466=CARTESIAN_POINT('Ctrl Pts',(89.5888777580777,50.7403018954297,12.7102643992676));
#77467=CARTESIAN_POINT('Ctrl Pts',(89.6122919095732,50.7448837586003,12.6529204440358));
#77468=CARTESIAN_POINT('Ctrl Pts',(89.6325920947704,50.7494656217708,12.5942590561464));
#77469=CARTESIAN_POINT('Ctrl Pts',(89.6496399301992,50.7540474849414,12.5346512720102));
#77470=CARTESIAN_POINT('Ctrl Pts',(89.6666836130879,50.758628232054,12.4750580072374));
#77471=CARTESIAN_POINT('Ctrl Pts',(89.6804763789678,50.7632089791667,12.4145192930305));
#77472=CARTESIAN_POINT('Ctrl Pts',(89.6909297172832,50.7677897262794,12.3534212598063));
#77473=CARTESIAN_POINT('Ctrl Pts',(89.7017603019815,50.7725357861588,12.2901182838805));
#77474=CARTESIAN_POINT('Ctrl Pts',(89.709005657291,50.7772818460382,12.2262154088906));
#77475=CARTESIAN_POINT('Ctrl Pts',(89.7126256410867,50.7820279059176,12.1621509916559));
#77476=CARTESIAN_POINT('Ctrl Pts',(89.7161239626396,50.7866144578209,12.1002396836941));
#77477=CARTESIAN_POINT('Ctrl Pts',(89.7162368207152,50.7912010097241,12.0381780483506));
#77478=CARTESIAN_POINT('Ctrl Pts',(89.7129811514963,50.7957875616274,11.9763618632993));
#77479=CARTESIAN_POINT('Ctrl Pts',(89.7095556471097,50.8006133754949,11.911320976518));
#77480=CARTESIAN_POINT('Ctrl Pts',(89.7024006033697,50.8054391893624,11.8465524909059));
#77481=CARTESIAN_POINT('Ctrl Pts',(89.6915972956155,50.8102650032298,11.7825082619017));
#77482=CARTESIAN_POINT('Ctrl Pts',(89.6807939878612,50.8150908170973,11.7184640328975));
#77483=CARTESIAN_POINT('Ctrl Pts',(89.6663426356459,50.8199166309648,11.6551446748319));
#77484=CARTESIAN_POINT('Ctrl Pts',(89.6483851321419,50.8247424448323,11.5929833357685));
#77485=CARTESIAN_POINT('Ctrl Pts',(89.6312785310761,50.8293395912357,11.533767463761));
#77486=CARTESIAN_POINT('Ctrl Pts',(89.6109203559465,50.8339367376392,11.475359179951));
#77487=CARTESIAN_POINT('Ctrl Pts',(89.5874052368878,50.8385338840426,11.4181409376162));
#77488=CARTESIAN_POINT('Ctrl Pts',(89.5634870240488,50.8432098342623,11.3599418659886));
#77489=CARTESIAN_POINT('Ctrl Pts',(89.5363026713531,50.847885784482,11.3029745552547));
#77490=CARTESIAN_POINT('Ctrl Pts',(89.5060053913801,50.8525617347017,11.2476273982199));
#77491=CARTESIAN_POINT('Ctrl Pts',(89.4763006636678,50.8571462329866,11.1933627173364));
#77492=CARTESIAN_POINT('Ctrl Pts',(89.4436039334705,50.8617307312715,11.1406558549161));
#77493=CARTESIAN_POINT('Ctrl Pts',(89.4081078498387,50.8663152295564,11.0898522184018));
#77494=CARTESIAN_POINT('Ctrl Pts',(89.3726334678097,50.8708969249698,11.0390796422251));
#77495=CARTESIAN_POINT('Ctrl Pts',(89.3343634168964,50.8754786203832,10.9902084011517));
#77496=CARTESIAN_POINT('Ctrl Pts',(89.2935343242799,50.8800603157966,10.9435559957647));
#77497=CARTESIAN_POINT('Ctrl Pts',(89.2527151959571,50.8846408930524,10.8969149758442));
#77498=CARTESIAN_POINT('Ctrl Pts',(89.2093386008289,50.8892214703083,10.8524920995507));
#77499=CARTESIAN_POINT('Ctrl Pts',(89.1636808995905,50.8938020475641,10.810571157206));
#77500=CARTESIAN_POINT('Ctrl Pts',(89.1163721240079,50.89854826771,10.7671342692373));
#77501=CARTESIAN_POINT('Ctrl Pts',(89.0666144868449,50.903294487856,10.7263841734061));
#77502=CARTESIAN_POINT('Ctrl Pts',(89.0147545343136,50.9080407080019,10.6885924094717));
#77503=CARTESIAN_POINT('Ctrl Pts',(88.9646411013919,50.9126270867645,10.6520733820822));
#77504=CARTESIAN_POINT('Ctrl Pts',(88.9125651954624,50.917213465527,10.618316808786));
#77505=CARTESIAN_POINT('Ctrl Pts',(88.8588684810597,50.9217998442895,10.5875231234728));
#77506=CARTESIAN_POINT('Ctrl Pts',(88.8023646640735,50.9266259851272,10.555119636991));
#77507=CARTESIAN_POINT('Ctrl Pts',(88.7440664965507,50.9314521259648,10.525997620887));
#77508=CARTESIAN_POINT('Ctrl Pts',(88.6843977849398,50.9362782668025,10.500333924862));
#77509=CARTESIAN_POINT('Ctrl Pts',(88.6247290733289,50.9411044076401,10.4746702288369));
#77510=CARTESIAN_POINT('Ctrl Pts',(88.5636904532144,50.9459305484778,10.4524650017373));
#77511=CARTESIAN_POINT('Ctrl Pts',(88.5017229000459,50.9507566893155,10.4338339940525));
#77512=CARTESIAN_POINT('Ctrl Pts',(88.4426943609331,50.9553539346258,10.4160866228946));
#77513=CARTESIAN_POINT('Ctrl Pts',(88.3825806479584,50.9599511799362,10.4015091716729));
#77514=CARTESIAN_POINT('Ctrl Pts',(88.3217544155937,50.9645484252466,10.3902295715734));
#77515=CARTESIAN_POINT('Ctrl Pts',(88.2598870007897,50.9692243631029,10.3787568948836));
#77516=CARTESIAN_POINT('Ctrl Pts',(88.1972829246974,50.9739003009593,10.3706962760495));
#77517=CARTESIAN_POINT('Ctrl Pts',(88.1343515751703,50.9785762388156,10.3661296447955));
#77518=CARTESIAN_POINT('Ctrl Pts',(88.0726494942767,50.9831608393054,10.3616522157691));
#77519=CARTESIAN_POINT('Ctrl Pts',(88.0106333425797,50.9877454397952,10.3605335406842));
#77520=CARTESIAN_POINT('Ctrl Pts',(87.9486978124994,50.992330040285,10.3627991096078));
#77521=CARTESIAN_POINT('Ctrl Pts',(87.8868001349848,50.9969118388469,10.3650632939047));
#77522=CARTESIAN_POINT('Ctrl Pts',(87.824983489032,51.0014936374087,10.370707602465));
#77523=CARTESIAN_POINT('Ctrl Pts',(87.7636429740228,51.0060754359706,10.3797054417156));
#77524=CARTESIAN_POINT('Ctrl Pts',(87.7023174183853,51.0106561171498,10.3887010866249));
#77525=CARTESIAN_POINT('Ctrl Pts',(87.6414682666095,51.015236798329,10.401048564842));
#77526=CARTESIAN_POINT('Ctrl Pts',(87.5814838475592,51.0198174795082,10.4166696175743));
#77527=CARTESIAN_POINT('Ctrl Pts',(87.5193329771451,51.0245636006991,10.4328548543319));
#77528=CARTESIAN_POINT('Ctrl Pts',(87.4581110767645,51.0293097218899,10.4525545699957));
#77529=CARTESIAN_POINT('Ctrl Pts',(87.3982341983022,51.0340558430808,10.4756249159806));
#77530=CARTESIAN_POINT('Ctrl Pts',(87.3403713037556,51.0386423264952,10.4979192812041));
#77531=CARTESIAN_POINT('Ctrl Pts',(87.2837648329454,51.0432288099096,10.523360834546));
#77532=CARTESIAN_POINT('Ctrl Pts',(87.2287685056506,51.047815293324,10.5517712442144));
#77533=CARTESIAN_POINT('Ctrl Pts',(87.1709008636871,51.0526412334031,10.5816649388591));
#77534=CARTESIAN_POINT('Ctrl Pts',(87.1148166627409,51.0574671734822,10.6148456730932));
#77535=CARTESIAN_POINT('Ctrl Pts',(87.0608942929944,51.0622931135613,10.6510533645697));
#77536=CARTESIAN_POINT('Ctrl Pts',(87.006971923248,51.0671190536405,10.6872610560462));
#77537=CARTESIAN_POINT('Ctrl Pts',(86.9552118543247,51.0719449937196,10.7264952517081));
#77538=CARTESIAN_POINT('Ctrl Pts',(86.9059504698246,51.0767709337987,10.7684483164594));
#77539=CARTESIAN_POINT('Ctrl Pts',(86.8594551730849,51.0813258913644,10.808045664657));
#77540=CARTESIAN_POINT('Ctrl Pts',(86.814981848768,51.0858808489301,10.8502384811275));
#77541=CARTESIAN_POINT('Ctrl Pts',(86.7728402917496,51.0904358064958,10.894788929157));
#77542=CARTESIAN_POINT('Ctrl Pts',(86.7309866254985,51.094959646791,10.939035030039));
#77543=CARTESIAN_POINT('Ctrl Pts',(86.691433367289,51.0994834870863,10.9856063034794));
#77544=CARTESIAN_POINT('Ctrl Pts',(86.6544517062852,51.1040073273815,11.0342289195663));
#77545=CARTESIAN_POINT('Ctrl Pts',(86.6175059510488,51.1085267754468,11.0828043275966));
#77546=CARTESIAN_POINT('Ctrl Pts',(86.5831271644513,51.1130462235121,11.1334267183578));
#77547=CARTESIAN_POINT('Ctrl Pts',(86.5515477123081,51.1175656715774,11.1857876077042));
#77548=CARTESIAN_POINT('Ctrl Pts',(86.5199865423486,51.1220825032142,11.2381181839411));
#77549=CARTESIAN_POINT('Ctrl Pts',(86.4912217654906,51.126599334851,11.2921848154484));
#77550=CARTESIAN_POINT('Ctrl Pts',(86.4654423658546,51.1311161664877,11.3476502000175));
#77551=CARTESIAN_POINT('Ctrl Pts',(86.4392958994072,51.1356973122284,11.403905343159));
#77552=CARTESIAN_POINT('Ctrl Pts',(86.4162207877119,51.1402784579691,11.4615989149807));
#77553=CARTESIAN_POINT('Ctrl Pts',(86.3963648395834,51.1448596037098,11.5203553039326));
#77554=CARTESIAN_POINT('Ctrl Pts',(86.3767772798433,51.149378827133,11.5783174959802));
#77555=CARTESIAN_POINT('Ctrl Pts',(86.3603224833752,51.1538980505563,11.6373134175068));
#77556=CARTESIAN_POINT('Ctrl Pts',(86.34709206766,51.1584172739796,11.696967171791));
#77557=CARTESIAN_POINT('Ctrl Pts',(86.3335897275704,51.163029380879,11.7578469880641));
#77558=CARTESIAN_POINT('Ctrl Pts',(86.3234459251632,51.1676414877784,11.8194114230928));
#77559=CARTESIAN_POINT('Ctrl Pts',(86.3167026929446,51.1722535946777,11.8812529542731));
#77560=CARTESIAN_POINT('Ctrl Pts',(86.309959460726,51.1768657015771,11.9430944854533));
#77561=CARTESIAN_POINT('Ctrl Pts',(86.3066167724698,51.1814778084765,12.0052125352787));
#77562=CARTESIAN_POINT('Ctrl Pts',(86.3066604225581,51.1860899153758,12.0672001521734));
#77563=CARTESIAN_POINT('',(86.3066605642293,51.9798399154705,12.0646131774589));
#77564=CARTESIAN_POINT('Ctrl Pts',(86.3066604225586,51.1860899154298,12.0672001528987));
#77565=CARTESIAN_POINT('Ctrl Pts',(86.3067130919174,51.1916550030472,12.1419960166398));
#77566=CARTESIAN_POINT('Ctrl Pts',(86.3116895962548,51.1972200906646,12.2166201618318));
#77567=CARTESIAN_POINT('Ctrl Pts',(86.3215218299453,51.202785178282,12.2905848358831));
#77568=CARTESIAN_POINT('Ctrl Pts',(86.3296440530645,51.2073823923769,12.3516856604259));
#77569=CARTESIAN_POINT('Ctrl Pts',(86.3411018368618,51.2119796064718,12.4124707301463));
#77570=CARTESIAN_POINT('Ctrl Pts',(86.355858390661,51.2165768205668,12.4725477691915));
#77571=CARTESIAN_POINT('Ctrl Pts',(86.370867651638,51.221252762325,12.5336536323914));
#77572=CARTESIAN_POINT('Ctrl Pts',(86.3892897538642,51.2259287040833,12.5940264482924));
#77573=CARTESIAN_POINT('Ctrl Pts',(86.4110308607976,51.2306046458416,12.6532593883454));
#77574=CARTESIAN_POINT('Ctrl Pts',(86.4323471215974,51.2351892143417,12.7113348488997));
#77575=CARTESIAN_POINT('Ctrl Pts',(86.4568536557395,51.2397737828418,12.7683140811023));
#77576=CARTESIAN_POINT('Ctrl Pts',(86.4844112400724,51.2443583513419,12.8238268889811));
#77577=CARTESIAN_POINT('Ctrl Pts',(86.5119519809785,51.2489401177153,12.8793057669658));
#77578=CARTESIAN_POINT('Ctrl Pts',(86.5425398485158,51.2535218840886,12.9333195428286));
#77579=CARTESIAN_POINT('Ctrl Pts',(86.575987984843,51.258103650462,12.9855190873251));
#77580=CARTESIAN_POINT('Ctrl Pts',(86.6094279629091,51.2626842993068,13.0377058999458));
#77581=CARTESIAN_POINT('Ctrl Pts',(86.645726550323,51.2672649481516,13.0880789312246));
#77582=CARTESIAN_POINT('Ctrl Pts',(86.6846525901919,51.2718455969964,13.1363164878181));
#77583=CARTESIAN_POINT('Ctrl Pts',(86.7249850657803,51.2765917491438,13.1862969142964));
#77584=CARTESIAN_POINT('Ctrl Pts',(86.7681381789869,51.2813379012912,13.2339841049719));
#77585=CARTESIAN_POINT('Ctrl Pts',(86.8138095736111,51.2860840534386,13.2790580854034));
#77586=CARTESIAN_POINT('Ctrl Pts',(86.8579441928296,51.2906705045312,13.3226153925403));
#77587=CARTESIAN_POINT('Ctrl Pts',(86.9044298579653,51.2952569556239,13.3637322733405));
#77588=CARTESIAN_POINT('Ctrl Pts',(86.9529584541405,51.2998434067166,13.4021597669572));
#77589=CARTESIAN_POINT('Ctrl Pts',(87.0040217120299,51.3046694093913,13.4425943389673));
#77590=CARTESIAN_POINT('Ctrl Pts',(87.0573466385354,51.3094954120661,13.4800505052685));
#77591=CARTESIAN_POINT('Ctrl Pts',(87.1125404367764,51.3143214147408,13.5142904573503));
#77592=CARTESIAN_POINT('Ctrl Pts',(87.1677342350173,51.3191474174155,13.5485304094321));
#77593=CARTESIAN_POINT('Ctrl Pts',(87.2247962987226,51.3239734200903,13.5795539057566));
#77594=CARTESIAN_POINT('Ctrl Pts',(87.2833077818663,51.328799422765,13.6071809988667));
#77595=CARTESIAN_POINT('Ctrl Pts',(87.3390455384296,51.3333966496307,13.6334984344808));
#77596=CARTESIAN_POINT('Ctrl Pts',(87.3963272293104,51.3379938764964,13.6568423081311));
#77597=CARTESIAN_POINT('Ctrl Pts',(87.4548033372498,51.3425911033621,13.677030759466));
#77598=CARTESIAN_POINT('Ctrl Pts',(87.5142806677395,51.347267043524,13.6975648756108));
#77599=CARTESIAN_POINT('Ctrl Pts',(87.5749932626738,51.3519429836859,13.7148341864651));
#77600=CARTESIAN_POINT('Ctrl Pts',(87.6365484410715,51.3566189238478,13.7286968652211));
#77601=CARTESIAN_POINT('Ctrl Pts',(87.6969009554397,51.3612035055703,13.7422886951951));
#77602=CARTESIAN_POINT('Ctrl Pts',(87.7580629042249,51.3657880872928,13.7526056961669));
#77603=CARTESIAN_POINT('Ctrl Pts',(87.8196477612758,51.3703726690154,13.7595640396322));
#77604=CARTESIAN_POINT('Ctrl Pts',(87.8811949790187,51.3749544487425,13.7665181303112));
#77605=CARTESIAN_POINT('Ctrl Pts',(87.943164087736,51.3795362284697,13.770117576732));
#77606=CARTESIAN_POINT('Ctrl Pts',(88.005160423092,51.3841180081969,13.770329995905));
#77607=CARTESIAN_POINT('Ctrl Pts',(88.0671416385854,51.3886986705051,13.7705423632726));
#77608=CARTESIAN_POINT('Ctrl Pts',(88.1291495587205,51.3932793328133,13.7673693414617));
#77609=CARTESIAN_POINT('Ctrl Pts',(88.1907885410593,51.3978599951215,13.7608306452574));
#77610=CARTESIAN_POINT('Ctrl Pts',(88.2546542398407,51.4026061344654,13.7540557377823));
#77611=CARTESIAN_POINT('Ctrl Pts',(88.3181232497171,51.4073522738093,13.7436673270672));
#77612=CARTESIAN_POINT('Ctrl Pts',(88.3807627611592,51.4120984131532,13.7297458748439));
#77613=CARTESIAN_POINT('Ctrl Pts',(88.4412948875003,51.4166848778268,13.7162927829305));
#77614=CARTESIAN_POINT('Ctrl Pts',(88.5010519575863,51.4212713425004,13.6995408265212));
#77615=CARTESIAN_POINT('Ctrl Pts',(88.5596576912754,51.4258578071739,13.6796138241241));
#77616=CARTESIAN_POINT('Ctrl Pts',(88.6213239035269,51.430683783853,13.6586462040295));
#77617=CARTESIAN_POINT('Ctrl Pts',(88.6817146322155,51.4355097605321,13.634163065632));
#77618=CARTESIAN_POINT('Ctrl Pts',(88.7404170450196,51.4403357372112,13.6063654144504));
#77619=CARTESIAN_POINT('Ctrl Pts',(88.7991194578237,51.4451617138903,13.5785677632688));
#77620=CARTESIAN_POINT('Ctrl Pts',(88.8561330230062,51.4499876905693,13.5474559776151));
#77621=CARTESIAN_POINT('Ctrl Pts',(88.9110793882464,51.4548136672484,13.513284329513));
#77622=CARTESIAN_POINT('Ctrl Pts',(88.9634212821718,51.4594108914382,13.4807324259905));
#77623=CARTESIAN_POINT('Ctrl Pts',(89.0141024548446,51.464008115628,13.4452705771532));
#77624=CARTESIAN_POINT('Ctrl Pts',(89.0627805440023,51.4686053398177,13.4070937785473));
#77625=CARTESIAN_POINT('Ctrl Pts',(89.1122921272935,51.4732812803141,13.3682632949215));
#77626=CARTESIAN_POINT('Ctrl Pts',(89.1597308850862,51.4779572208106,13.326624211991));
#77627=CARTESIAN_POINT('Ctrl Pts',(89.2047646755216,51.482633161307,13.2824295027155));
#77628=CARTESIAN_POINT('Ctrl Pts',(89.2489185673613,51.4872177403293,13.239098297539));
#77629=CARTESIAN_POINT('Ctrl Pts',(89.2907602454635,51.4918023193517,13.1933108083627));
#77630=CARTESIAN_POINT('Ctrl Pts',(89.3300096325757,51.496386898374,13.1453462951123));
#77631=CARTESIAN_POINT('Ctrl Pts',(89.369235031301,51.5009686753996,13.0974110967477));
#77632=CARTESIAN_POINT('Ctrl Pts',(89.4058709588722,51.5055504524252,13.047301905739));
#77633=CARTESIAN_POINT('Ctrl Pts',(89.4396761443467,51.5101322294508,12.9953327230732));
#77634=CARTESIAN_POINT('Ctrl Pts',(89.4734730853234,51.5147128890605,12.9433762147888));
#77635=CARTESIAN_POINT('Ctrl Pts',(89.5044403772444,51.5192935486702,12.8895610418726));
#77636=CARTESIAN_POINT('Ctrl Pts',(89.5323799870813,51.5238742082799,12.8342302848161));
#77637=CARTESIAN_POINT('Ctrl Pts',(89.561328952019,51.5286203502342,12.7769006314902));
#77638=CARTESIAN_POINT('Ctrl Pts',(89.5870269692947,51.5333664921885,12.7179442826247));
#77639=CARTESIAN_POINT('Ctrl Pts',(89.609306880766,51.5381126341428,12.6577684940041));
#77640=CARTESIAN_POINT('Ctrl Pts',(89.6308372034223,51.5426990961573,12.5996172689975));
#77641=CARTESIAN_POINT('Ctrl Pts',(89.6491756941917,51.5472855581717,12.5403278862145));
#77642=CARTESIAN_POINT('Ctrl Pts',(89.6642222819317,51.5518720201862,12.4802836252188));
#77643=CARTESIAN_POINT('Ctrl Pts',(89.6800546512452,51.5566980021104,12.4171036583279));
#77644=CARTESIAN_POINT('Ctrl Pts',(89.692241730495,51.5615239840347,12.3530884374176));
#77645=CARTESIAN_POINT('Ctrl Pts',(89.7007284689377,51.5663499659589,12.2886938186422));
#77646=CARTESIAN_POINT('Ctrl Pts',(89.7092152073804,51.5711759478831,12.2242991998668));
#77647=CARTESIAN_POINT('Ctrl Pts',(89.7140016344315,51.5760019298073,12.1595258351518));
#77648=CARTESIAN_POINT('Ctrl Pts',(89.715096151996,51.5808279117316,12.0948295048961));
#77649=CARTESIAN_POINT('Ctrl Pts',(89.7161387876291,51.5854251341817,12.0331998870144));
#77650=CARTESIAN_POINT('Ctrl Pts',(89.7138359464523,51.5900223566319,11.9713871243631));
#77651=CARTESIAN_POINT('Ctrl Pts',(89.7081657511357,51.594619579082,11.9097846077624));
#77652=CARTESIAN_POINT('Ctrl Pts',(89.7023984650355,51.5992955197959,11.8471272709525));
#77653=CARTESIAN_POINT('Ctrl Pts',(89.6931473169984,51.6039714605098,11.784687976654));
#77654=CARTESIAN_POINT('Ctrl Pts',(89.6804446813148,51.6086474012236,11.7228829767708));
#77655=CARTESIAN_POINT('Ctrl Pts',(89.6679902433133,51.6132319784067,11.6622855890788));
#77656=CARTESIAN_POINT('Ctrl Pts',(89.6522180897161,51.6178165555898,11.6022984541811));
#77657=CARTESIAN_POINT('Ctrl Pts',(89.6332109188214,51.6224011327728,11.5433083409346));
#77658=CARTESIAN_POINT('Ctrl Pts',(89.6142153648411,51.6269829079271,11.484354281612));
#77659=CARTESIAN_POINT('Ctrl Pts',(89.591988869851,51.6315646830813,11.4263965191688));
#77660=CARTESIAN_POINT('Ctrl Pts',(89.5666643673551,51.6361464582355,11.3698080640071));
#77661=CARTESIAN_POINT('Ctrl Pts',(89.5413460412288,51.6407271159449,11.3132334101515));
#77662=CARTESIAN_POINT('Ctrl Pts',(89.5129314153614,51.6453077736542,11.2580278650513));
#77663=CARTESIAN_POINT('Ctrl Pts',(89.4816013057684,51.6498884313635,11.2045438867405));
#77664=CARTESIAN_POINT('Ctrl Pts',(89.449139329153,51.6546345751011,11.1491276856553));
#77665=CARTESIAN_POINT('Ctrl Pts',(89.4135474179629,51.6593807188387,11.0955603575894));
#77666=CARTESIAN_POINT('Ctrl Pts',(89.3750770503391,51.6641268625764,11.0442032313917));
#77667=CARTESIAN_POINT('Ctrl Pts',(89.3379010155446,51.6687133226397,10.9945740121148));
#77668=CARTESIAN_POINT('Ctrl Pts',(89.2980375462268,51.6732997827031,10.9470089810368));
#77669=CARTESIAN_POINT('Ctrl Pts',(89.2557543649582,51.6778862427664,10.901800100276));
#77670=CARTESIAN_POINT('Ctrl Pts',(89.2112629663549,51.6827122283411,10.8542302090333));
#77671=CARTESIAN_POINT('Ctrl Pts',(89.1640926474987,51.6875382139159,10.8092697662519));
#77672=CARTESIAN_POINT('Ctrl Pts',(89.1145965243496,51.6923641994907,10.7672122779132));
#77673=CARTESIAN_POINT('Ctrl Pts',(89.0651004012004,51.6971901850654,10.7251547895744));
#77674=CARTESIAN_POINT('Ctrl Pts',(89.0132790374135,51.7020161706401,10.6860005845717));
#77675=CARTESIAN_POINT('Ctrl Pts',(88.9595199021039,51.7068421562149,10.6499898196295));
#77676=CARTESIAN_POINT('Ctrl Pts',(88.9083090589371,51.7114393802768,10.6156860380462));
#77677=CARTESIAN_POINT('Ctrl Pts',(88.8551297687583,51.7160366043387,10.5840935275524));
#77678=CARTESIAN_POINT('Ctrl Pts',(88.8003006616581,51.7206338284007,10.5554440423784));
#77679=CARTESIAN_POINT('Ctrl Pts',(88.7445327374292,51.7253097689131,10.5263040033941));
#77680=CARTESIAN_POINT('Ctrl Pts',(88.6870583538989,51.7299857094255,10.5002090968762));
#77681=CARTESIAN_POINT('Ctrl Pts',(88.6282447727882,51.7346616499378,10.4773578986865));
#77682=CARTESIAN_POINT('Ctrl Pts',(88.5705803308158,51.7392462287928,10.4549531825118));
#77683=CARTESIAN_POINT('Ctrl Pts',(88.511629050097,51.7438308076477,10.4356667523341));
#77684=CARTESIAN_POINT('Ctrl Pts',(88.4517607190889,51.7484153865026,10.4196389144212));
#77685=CARTESIAN_POINT('Ctrl Pts',(88.3919289785141,51.7529971633465,10.4036208724309));
#77686=CARTESIAN_POINT('Ctrl Pts',(88.3311817897196,51.7575789401903,10.3908576050375));
#77687=CARTESIAN_POINT('Ctrl Pts',(88.2699046298808,51.7621607170341,10.3814397522717));
#77688=CARTESIAN_POINT('Ctrl Pts',(88.2086424146661,51.7667413764481,10.3720241963857));
#77689=CARTESIAN_POINT('Ctrl Pts',(88.1468509879067,51.7713220358619,10.3659525127385));
#77690=CARTESIAN_POINT('Ctrl Pts',(88.0849245316919,51.7759026952759,10.363263966666));
#77691=CARTESIAN_POINT('Ctrl Pts',(88.0207608959499,51.7806488373944,10.36047829312));
#77692=CARTESIAN_POINT('Ctrl Pts',(87.9564528657858,51.7853949795129,10.3613249675671));
#77693=CARTESIAN_POINT('Ctrl Pts',(87.8924404019637,51.7901411216314,10.3657887021569));
#77694=CARTESIAN_POINT('Ctrl Pts',(87.8305815886813,51.794727583417,10.3701022577997));
#77695=CARTESIAN_POINT('Ctrl Pts',(87.768999282998,51.7993140452026,10.3777931994341));
#77696=CARTESIAN_POINT('Ctrl Pts',(87.7080839810922,51.8039005069881,10.3887949674864));
#77697=CARTESIAN_POINT('Ctrl Pts',(87.6439874767223,51.8087264892731,10.4003712849629));
#77698=CARTESIAN_POINT('Ctrl Pts',(87.5806301815173,51.8135524715581,10.4156135763098));
#77699=CARTESIAN_POINT('Ctrl Pts',(87.5184502046144,51.8183784538431,10.4343843790078));
#77700=CARTESIAN_POINT('Ctrl Pts',(87.4562702277115,51.8232044361281,10.4531551817058));
#77701=CARTESIAN_POINT('Ctrl Pts',(87.3952681511434,51.8280304184131,10.4754542006095));
#77702=CARTESIAN_POINT('Ctrl Pts',(87.3358558974417,51.832856400698,10.5010861760529));
#77703=CARTESIAN_POINT('Ctrl Pts',(87.2792598719986,51.8374536243207,10.5255031581393));
#77704=CARTESIAN_POINT('Ctrl Pts',(87.2238739591252,51.8420508479433,10.5530444637661));
#77705=CARTESIAN_POINT('Ctrl Pts',(87.1700656849818,51.8466480715659,10.5835681083352));
#77706=CARTESIAN_POINT('Ctrl Pts',(87.1153360671562,51.8513240121332,10.6146144005367));
#77707=CARTESIAN_POINT('Ctrl Pts',(87.0622391480133,51.8559999527005,10.6487460015799));
#77708=CARTESIAN_POINT('Ctrl Pts',(87.0111409577233,51.8606758932678,10.6857620744316));
#77709=CARTESIAN_POINT('Ctrl Pts',(86.9610411635716,51.8652604716757,10.7220548984953));
#77710=CARTESIAN_POINT('Ctrl Pts',(86.9128631272666,51.8698450500836,10.7611201770715));
#77711=CARTESIAN_POINT('Ctrl Pts',(86.8669252958447,51.8744296284915,10.8027233450617));
#77712=CARTESIAN_POINT('Ctrl Pts',(86.8210155408074,51.8790114048868,10.8443010859365));
#77713=CARTESIAN_POINT('Ctrl Pts',(86.7773436523091,51.883593181282,10.8884132995929));
#77714=CARTESIAN_POINT('Ctrl Pts',(86.7361948612738,51.8881749576772,10.9347853015995));
#77715=CARTESIAN_POINT('Ctrl Pts',(86.6950561058497,51.8927556166417,10.9811459941273));
#77716=CARTESIAN_POINT('Ctrl Pts',(86.6564395640461,51.8973362756061,11.029765000343));
#77717=CARTESIAN_POINT('Ctrl Pts',(86.6205920273553,51.9019169345705,11.0803324570597));
#77718=CARTESIAN_POINT('Ctrl Pts',(86.5834494414185,51.9066630771214,11.1327267435319));
#77719=CARTESIAN_POINT('Ctrl Pts',(86.5492801490811,51.9114092196723,11.1872125204093));
#77720=CARTESIAN_POINT('Ctrl Pts',(86.5183099409665,51.9161553622232,11.2434118750781));
#77721=CARTESIAN_POINT('Ctrl Pts',(86.4883817075303,51.9207418235624,11.2977204350745));
#77722=CARTESIAN_POINT('Ctrl Pts',(86.4614408643829,51.9253282849016,11.3536285849229));
#77723=CARTESIAN_POINT('Ctrl Pts',(86.4376432980279,51.9299147462408,11.4107721587422));
#77724=CARTESIAN_POINT('Ctrl Pts',(86.4126029355551,51.9347407293975,11.4708999793805));
#77725=CARTESIAN_POINT('Ctrl Pts',(86.391043382755,51.9395667125543,11.5323951949942));
#77726=CARTESIAN_POINT('Ctrl Pts',(86.3730867843619,51.944392695711,11.5948151810192));
#77727=CARTESIAN_POINT('Ctrl Pts',(86.3551301859688,51.9492186788678,11.6572351670442));
#77728=CARTESIAN_POINT('Ctrl Pts',(86.3407766097187,51.9540446620245,11.7205792744149));
#77729=CARTESIAN_POINT('Ctrl Pts',(86.3300854400862,51.9588706451812,11.7843955293858));
#77730=CARTESIAN_POINT('Ctrl Pts',(86.3146007869758,51.9658604019308,11.8768243846938));
#77731=CARTESIAN_POINT('Ctrl Pts',(86.3067370918222,51.9728501586803,11.9705644153934));
#77732=CARTESIAN_POINT('Ctrl Pts',(86.3066605642297,51.9798399154299,12.064613176913));
#77733=CARTESIAN_POINT('',(86.3066600304637,52.7735899153848,12.0656777559288));
#77734=CARTESIAN_POINT('Ctrl Pts',(86.3066605642293,51.9798399154705,12.0646131774589));
#77735=CARTESIAN_POINT('Ctrl Pts',(86.3066110592266,51.9843615272388,12.1254524887725));
#77736=CARTESIAN_POINT('Ctrl Pts',(86.3098234268039,51.9888831390072,12.1864087974373));
#77737=CARTESIAN_POINT('Ctrl Pts',(86.3163087196424,51.9934047507755,12.2470974872272));
#77738=CARTESIAN_POINT('Ctrl Pts',(86.3227874283413,51.9979217720151,12.3077245633292));
#77739=CARTESIAN_POINT('Ctrl Pts',(86.3325324283883,52.0024387932547,12.3680840389148));
#77740=CARTESIAN_POINT('Ctrl Pts',(86.345502752508,52.0069558144942,12.4277924186555));
#77741=CARTESIAN_POINT('Ctrl Pts',(86.3584650054124,52.0114700248672,12.4874636428725));
#77742=CARTESIAN_POINT('Ctrl Pts',(86.3746484952788,52.0159842352402,12.5464840613476));
#77743=CARTESIAN_POINT('Ctrl Pts',(86.393960872915,52.0204984456132,12.6044786876713));
#77744=CARTESIAN_POINT('Ctrl Pts',(86.4132688196422,52.0250116202745,12.662460008077));
#77745=CARTESIAN_POINT('Ctrl Pts',(86.435704063534,52.0295247949358,12.7194155048757));
#77746=CARTESIAN_POINT('Ctrl Pts',(86.4611245850067,52.0340379695971,12.7749859191827));
#77747=CARTESIAN_POINT('Ctrl Pts',(86.4865669549605,52.0385550232509,12.8306040952616));
#77748=CARTESIAN_POINT('Ctrl Pts',(86.5149995091763,52.0430720769047,12.8848343315321));
#77749=CARTESIAN_POINT('Ctrl Pts',(86.5462328952534,52.0475891305585,12.9373392935316));
#77750=CARTESIAN_POINT('Ctrl Pts',(86.5774796251288,52.0521081140271,12.9898666871568));
#77751=CARTESIAN_POINT('Ctrl Pts',(86.6115292756043,52.0566270974958,13.0406669021523));
#77752=CARTESIAN_POINT('Ctrl Pts',(86.6481492710332,52.0611460809645,13.0894318375713));
#77753=CARTESIAN_POINT('Ctrl Pts',(86.6848359186587,52.0656732894526,13.1382855302397));
#77754=CARTESIAN_POINT('Ctrl Pts',(86.7241019130956,52.0702004979407,13.185096144303));
#77755=CARTESIAN_POINT('Ctrl Pts',(86.7656752921718,52.0747277064288,13.2295897935582));
#77756=CARTESIAN_POINT('Ctrl Pts',(86.7967664476536,52.078113434174,13.2628649084919));
#77757=CARTESIAN_POINT('Ctrl Pts',(86.8291472898651,52.0814991619193,13.2948448699306));
#77758=CARTESIAN_POINT('Ctrl Pts',(86.862692146513,52.0848848896645,13.325429993775));
#77759=CARTESIAN_POINT('Ctrl Pts',(86.9082401705004,52.0894821133216,13.3669592204204));
#77760=CARTESIAN_POINT('Ctrl Pts',(86.9561374912916,52.0940793369787,13.4060996032432));
#77761=CARTESIAN_POINT('Ctrl Pts',(87.0061034332076,52.0986765606358,13.4425746349722));
#77762=CARTESIAN_POINT('Ctrl Pts',(87.0569249272226,52.1033525011988,13.4796742179207));
#77763=CARTESIAN_POINT('Ctrl Pts',(87.1098862220447,52.1080284417618,13.5140158871587));
#77764=CARTESIAN_POINT('Ctrl Pts',(87.1646536219269,52.1127043823248,13.5453487228921));
#77765=CARTESIAN_POINT('Ctrl Pts',(87.2183509342208,52.1172889607641,13.5760693535784));
#77766=CARTESIAN_POINT('Ctrl Pts',(87.2737839451832,52.1218735392034,13.6038974062373));
#77767=CARTESIAN_POINT('Ctrl Pts',(87.3306078061622,52.1264581176428,13.6286392092113));
#77768=CARTESIAN_POINT('Ctrl Pts',(87.3873969373941,52.1310398940682,13.6533658904294));
#77769=CARTESIAN_POINT('Ctrl Pts',(87.4455747673341,52.1356216704936,13.6750098593511));
#77770=CARTESIAN_POINT('Ctrl Pts',(87.5047735561091,52.140203446919,13.693424229605));
#77771=CARTESIAN_POINT('Ctrl Pts',(87.5639579071159,52.1447841059124,13.711834108848));
#77772=CARTESIAN_POINT('Ctrl Pts',(87.6241622368029,52.1493647649057,13.7270158019066));
#77773=CARTESIAN_POINT('Ctrl Pts',(87.6850025666825,52.153945423899,13.73887193445));
#77774=CARTESIAN_POINT('Ctrl Pts',(87.7480408493917,52.1586915664197,13.7511563884723));
#77775=CARTESIAN_POINT('Ctrl Pts',(87.811761406716,52.1634377089405,13.7598702251828));
#77776=CARTESIAN_POINT('Ctrl Pts',(87.8757268866723,52.1681838514612,13.7649632192636));
#77777=CARTESIAN_POINT('Ctrl Pts',(87.9375402859127,52.1727703128257,13.7698848625728));
#77778=CARTESIAN_POINT('Ctrl Pts',(87.9995818583249,52.1773567741903,13.7714255110949));
#77779=CARTESIAN_POINT('Ctrl Pts',(88.0614555531867,52.1819432355548,13.769592989171));
#77780=CARTESIAN_POINT('Ctrl Pts',(88.1265605179797,52.1867692186536,13.7676647662711));
#77781=CARTESIAN_POINT('Ctrl Pts',(88.1914789475542,52.1915952017524,13.7620014384124));
#77782=CARTESIAN_POINT('Ctrl Pts',(88.2557571753501,52.1964211848512,13.7526738750317));
#77783=CARTESIAN_POINT('Ctrl Pts',(88.320035403146,52.20124716795,13.7433463116511));
#77784=CARTESIAN_POINT('Ctrl Pts',(88.3836728097494,52.2060731510488,13.7303547181766));
#77785=CARTESIAN_POINT('Ctrl Pts',(88.4462330406866,52.2108991341476,13.7138310095075));
#77786=CARTESIAN_POINT('Ctrl Pts',(88.5058278141434,52.2154963577379,13.6980905517112));
#77787=CARTESIAN_POINT('Ctrl Pts',(88.5646899250684,52.2200935813282,13.6790806940928));
#77788=CARTESIAN_POINT('Ctrl Pts',(88.6224348357162,52.2246908049185,13.656887261019));
#77789=CARTESIAN_POINT('Ctrl Pts',(88.6811684964101,52.2293667454899,13.6343138159627));
#77790=CARTESIAN_POINT('Ctrl Pts',(88.738745800749,52.2340426860612,13.6084467899394));
#77791=CARTESIAN_POINT('Ctrl Pts',(88.7947749495291,52.2387186266326,13.5794304292205));
#77792=CARTESIAN_POINT('Ctrl Pts',(88.8497093567838,52.2433032050036,13.5509810129526));
#77793=CARTESIAN_POINT('Ctrl Pts',(88.9031550888766,52.2478877833747,13.5195044688184));
#77794=CARTESIAN_POINT('Ctrl Pts',(88.9547623926716,52.2524723617457,13.4851854641937));
#77795=CARTESIAN_POINT('Ctrl Pts',(89.0063381549831,52.2570541381025,13.4508874347458));
#77796=CARTESIAN_POINT('Ctrl Pts',(89.0560772939649,52.2616359144592,13.4137506708428));
#77797=CARTESIAN_POINT('Ctrl Pts',(89.1036569456197,52.266217690816,13.3740044475418));
#77798=CARTESIAN_POINT('Ctrl Pts',(89.1512249932506,52.2707983497404,13.3342679177989));
#77799=CARTESIAN_POINT('Ctrl Pts',(89.1966342085771,52.2753790086648,13.2919235182363));
#77800=CARTESIAN_POINT('Ctrl Pts',(89.2395945159105,52.2799596675893,13.2472410215848));
#77801=CARTESIAN_POINT('Ctrl Pts',(89.2841068333612,52.2847058101761,13.2009442979601));
#77802=CARTESIAN_POINT('Ctrl Pts',(89.325989464459,52.2894519527629,13.1521376824791));
#77803=CARTESIAN_POINT('Ctrl Pts',(89.3649629946575,52.2941980953497,13.1011613616717));
#77804=CARTESIAN_POINT('Ctrl Pts',(89.4026252824094,52.2987845566454,13.0519001104328));
#77805=CARTESIAN_POINT('Ctrl Pts',(89.4375708857887,52.3033710179412,13.000613318739));
#77806=CARTESIAN_POINT('Ctrl Pts',(89.4695915607741,52.307957479237,12.947637961092));
#77807=CARTESIAN_POINT('Ctrl Pts',(89.5032844735889,52.3127834624693,12.8918960347477));
#77808=CARTESIAN_POINT('Ctrl Pts',(89.5337382689994,52.3176094457016,12.8342849041646));
#77809=CARTESIAN_POINT('Ctrl Pts',(89.5607664177231,52.3224354289339,12.7752241437639));
#77810=CARTESIAN_POINT('Ctrl Pts',(89.5877945664468,52.3272614121663,12.7161633833633));
#77811=CARTESIAN_POINT('Ctrl Pts',(89.6113969050988,52.3320873953986,12.6556536249518));
#77812=CARTESIAN_POINT('Ctrl Pts',(89.631447580047,52.3369133786309,12.5941330096858));
#77813=CARTESIAN_POINT('Ctrl Pts',(89.6505478195558,52.3415106022077,12.535528574207));
#77814=CARTESIAN_POINT('Ctrl Pts',(89.6665039718338,52.3461078257845,12.4757663456097));
#77815=CARTESIAN_POINT('Ctrl Pts',(89.6791795669483,52.3507050493613,12.4152159332221));
#77816=CARTESIAN_POINT('Ctrl Pts',(89.6920722027953,52.3553809899344,12.3536287327593));
#77817=CARTESIAN_POINT('Ctrl Pts',(89.70157062529,52.3600569305074,12.2912265774969));
#77818=CARTESIAN_POINT('Ctrl Pts',(89.7075835073716,52.3647328710804,12.2284168652413));
#77819=CARTESIAN_POINT('Ctrl Pts',(89.7134789050183,52.3693174494369,12.1668343787055));
#77820=CARTESIAN_POINT('Ctrl Pts',(89.7160236929141,52.3739020277933,12.1048606492721));
#77821=CARTESIAN_POINT('Ctrl Pts',(89.71518330836,52.3784866061497,12.0428896753089));
#77822=CARTESIAN_POINT('Ctrl Pts',(89.7143434374343,52.3830683824915,11.9809565769287));
#77823=CARTESIAN_POINT('Ctrl Pts',(89.710122503393,52.3876501588333,11.9190267386236));
#77824=CARTESIAN_POINT('Ctrl Pts',(89.70253800403,52.392231935175,11.8574957637787));
#77825=CARTESIAN_POINT('Ctrl Pts',(89.6949553544229,52.3968125940841,11.7959797954986));
#77826=CARTESIAN_POINT('Ctrl Pts',(89.6840108302165,52.4013932529931,11.7348630025654));
#77827=CARTESIAN_POINT('Ctrl Pts',(89.669773736496,52.4059739119022,11.6745354081002));
#77828=CARTESIAN_POINT('Ctrl Pts',(89.6550223047996,52.4107200545032,11.6120283819732));
#77829=CARTESIAN_POINT('Ctrl Pts',(89.6367359211655,52.4154661971042,11.5503692487821));
#77830=CARTESIAN_POINT('Ctrl Pts',(89.6150488293952,52.4202123397052,11.489977267362));
#77831=CARTESIAN_POINT('Ctrl Pts',(89.5940913877346,52.4247988009849,11.4316171404813));
#77832=CARTESIAN_POINT('Ctrl Pts',(89.5699587204277,52.4293852622646,11.3744407070064));
#77833=CARTESIAN_POINT('Ctrl Pts',(89.5428209755857,52.4339717235443,11.3188056917002));
#77834=CARTESIAN_POINT('Ctrl Pts',(89.5142659972748,52.438797706806,11.2602652099966));
#77835=CARTESIAN_POINT('Ctrl Pts',(89.4823837675879,52.4436236900676,11.2034321253496));
#77836=CARTESIAN_POINT('Ctrl Pts',(89.4474256066323,52.4484496733293,11.148690721615));
#77837=CARTESIAN_POINT('Ctrl Pts',(89.4124674456766,52.4532756565909,11.0939493178805));
#77838=CARTESIAN_POINT('Ctrl Pts',(89.3744337956266,52.4581016398525,11.0413000750128));
#77839=CARTESIAN_POINT('Ctrl Pts',(89.3336244852963,52.4629276231142,10.9910863725421));
#77840=CARTESIAN_POINT('Ctrl Pts',(89.2947496043837,52.467524846715,10.9432528833718));
#77841=CARTESIAN_POINT('Ctrl Pts',(89.2531966879137,52.4721220703158,10.8974328229279));
#77842=CARTESIAN_POINT('Ctrl Pts',(89.2092022313909,52.4767192939166,10.8539413181327));
#77843=CARTESIAN_POINT('Ctrl Pts',(89.1644544701387,52.4813952344866,10.8097051205094));
#77844=CARTESIAN_POINT('Ctrl Pts',(89.1171810309949,52.4860711750567,10.7678784429161));
#77845=CARTESIAN_POINT('Ctrl Pts',(89.0676746417971,52.4907471156267,10.7287589832109));
#77846=CARTESIAN_POINT('Ctrl Pts',(89.0191355472001,52.4953316940081,10.6904038701442));
#77847=CARTESIAN_POINT('Ctrl Pts',(88.9684503945638,52.4999162723895,10.6546514656367));
#77848=CARTESIAN_POINT('Ctrl Pts',(88.9159314434978,52.5045008507709,10.6217445107707));
#77849=CARTESIAN_POINT('Ctrl Pts',(88.8634445910991,52.509082627138,10.5888576680617));
#77850=CARTESIAN_POINT('Ctrl Pts',(88.8091265930975,52.513664403505,10.558813096353));
#77851=CARTESIAN_POINT('Ctrl Pts',(88.7533192950585,52.5182461798721,10.5318106701636));
#77852=CARTESIAN_POINT('Ctrl Pts',(88.6975256076543,52.5228268388067,10.5048148294958));
#77853=CARTESIAN_POINT('Ctrl Pts',(88.6402437992809,52.5274074977413,10.480859883103));
#77854=CARTESIAN_POINT('Ctrl Pts',(88.5818391276159,52.5319881566759,10.4600991543739));
#77855=CARTESIAN_POINT('Ctrl Pts',(88.5213244936232,52.5367342992527,10.4385884110609));
#77856=CARTESIAN_POINT('Ctrl Pts',(88.4596048389029,52.5414804418294,10.420507351753));
#77857=CARTESIAN_POINT('Ctrl Pts',(88.397105205341,52.5462265844062,10.4059706008602));
#77858=CARTESIAN_POINT('Ctrl Pts',(88.3367083364506,52.5508130457118,10.3919229306942));
#77859=CARTESIAN_POINT('Ctrl Pts',(88.2755836749861,52.5553995070174,10.3811848686896));
#77860=CARTESIAN_POINT('Ctrl Pts',(88.2141240412226,52.559985968323,10.3738074992846));
#77861=CARTESIAN_POINT('Ctrl Pts',(88.1494547589547,52.5648119515354,10.3660448564696));
#77862=CARTESIAN_POINT('Ctrl Pts',(88.0844152000847,52.5696379347478,10.3620035979478));
#77863=CARTESIAN_POINT('Ctrl Pts',(88.0194645253132,52.5744639179602,10.3616810194652));
#77864=CARTESIAN_POINT('Ctrl Pts',(87.9545138505416,52.5792899011726,10.3613584409825));
#77865=CARTESIAN_POINT('Ctrl Pts',(87.8896527029231,52.584115884385,10.3647544313855));
#77866=CARTESIAN_POINT('Ctrl Pts',(87.8253321896315,52.5889418675974,10.3718033467767));
#77867=CARTESIAN_POINT('Ctrl Pts',(87.7640605755197,52.5935390911885,10.3785181318687));
#77868=CARTESIAN_POINT('Ctrl Pts',(87.7030279223271,52.5981363147797,10.3885748725647));
#77869=CARTESIAN_POINT('Ctrl Pts',(87.6426272497201,52.6027335383709,10.4019458084391));
#77870=CARTESIAN_POINT('Ctrl Pts',(87.5811923532064,52.6074094789421,10.4155456911273));
#77871=CARTESIAN_POINT('Ctrl Pts',(87.5204118209124,52.6120854195133,10.4325743699693));
#77872=CARTESIAN_POINT('Ctrl Pts',(87.46069453033,52.6167613600846,10.4529473890628));
#77873=CARTESIAN_POINT('Ctrl Pts',(87.4021440430775,52.6213459384561,10.4729223441067));
#77874=CARTESIAN_POINT('Ctrl Pts',(87.3446161271531,52.6259305168276,10.4961119538344));
#77875=CARTESIAN_POINT('Ctrl Pts',(87.2884840837042,52.6305150951992,10.522385544801));
#77876=CARTESIAN_POINT('Ctrl Pts',(87.2323863471824,52.6350968715562,10.5486430778065));
#77877=CARTESIAN_POINT('Ctrl Pts',(87.1776832515823,52.6396786479133,10.5779806392638));
#77878=CARTESIAN_POINT('Ctrl Pts',(87.1247281323297,52.6442604242704,10.6102194491696));
#77879=CARTESIAN_POINT('Ctrl Pts',(87.0717859281054,52.648841083195,10.6424503964711));
#77880=CARTESIAN_POINT('Ctrl Pts',(87.020591288557,52.6534217421196,10.6775809229875));
#77881=CARTESIAN_POINT('Ctrl Pts',(86.9714711392208,52.6580024010442,10.7153873304285));
#77882=CARTESIAN_POINT('Ctrl Pts',(86.9205764455857,52.6627485436305,10.7545595550686));
#77883=CARTESIAN_POINT('Ctrl Pts',(86.8719095003477,52.6674946862169,10.7966043995105));
#77884=CARTESIAN_POINT('Ctrl Pts',(86.8257971440967,52.6722408288033,10.841226949203));
#77885=CARTESIAN_POINT('Ctrl Pts',(86.7812362120673,52.6768272900989,10.8843481983753));
#77886=CARTESIAN_POINT('Ctrl Pts',(86.739060998119,52.6814137513944,10.9298760088617));
#77887=CARTESIAN_POINT('Ctrl Pts',(86.6995274846004,52.68600021269,10.9775080721698));
#77888=CARTESIAN_POINT('Ctrl Pts',(86.6579293850988,52.6908261959218,11.0276276576205));
#77889=CARTESIAN_POINT('Ctrl Pts',(86.6192568617795,52.6956521791536,11.0800767945419));
#77890=CARTESIAN_POINT('Ctrl Pts',(86.5837566909408,52.7004781623853,11.1344682655187));
#77891=CARTESIAN_POINT('Ctrl Pts',(86.5482565201021,52.7053041456171,11.1888597364954));
#77892=CARTESIAN_POINT('Ctrl Pts',(86.5159289571537,52.7101301288489,11.2451929409941));
#77893=CARTESIAN_POINT('Ctrl Pts',(86.4869635332425,52.7149561120806,11.3030532891523));
#77894=CARTESIAN_POINT('Ctrl Pts',(86.4574999237459,52.7198650989407,11.3619087959349));
#77895=CARTESIAN_POINT('Ctrl Pts',(86.4314063174814,52.7247740858009,11.4225592194157));
#77896=CARTESIAN_POINT('Ctrl Pts',(86.4088885715127,52.729683072661,11.4846104521835));
#77897=CARTESIAN_POINT('Ctrl Pts',(86.3864229191759,52.7345807028357,11.5465181326575));
#77898=CARTESIAN_POINT('Ctrl Pts',(86.3675168111418,52.7394783330105,11.6098198038362));
#77899=CARTESIAN_POINT('Ctrl Pts',(86.3523292230594,52.7443759631853,11.6740993884629));
#77900=CARTESIAN_POINT('Ctrl Pts',(86.3371938783017,52.7492567461502,11.738157859691));
#77901=CARTESIAN_POINT('Ctrl Pts',(86.325751674089,52.7541375291151,11.803187158091));
#77902=CARTESIAN_POINT('Ctrl Pts',(86.3181120088452,52.75901831208,11.8687562801913));
#77903=CARTESIAN_POINT('Ctrl Pts',(86.3105092552082,52.7638755131816,11.9340086002363));
#77904=CARTESIAN_POINT('Ctrl Pts',(86.3066724870618,52.7687327142832,11.9997951539516));
#77905=CARTESIAN_POINT('Ctrl Pts',(86.3066600304638,52.7735899153848,12.0656777559288));
#77906=CARTESIAN_POINT('',(86.3066607114372,53.5673399154776,12.0675572608337));
#77907=CARTESIAN_POINT('Ctrl Pts',(86.3066600304636,52.7735899154298,12.0656777565391));
#77908=CARTESIAN_POINT('Ctrl Pts',(86.3066478884484,52.7783244602588,12.129896660799));
#77909=CARTESIAN_POINT('Ctrl Pts',(86.3102696895027,52.7830590050878,12.1940683671357));
#77910=CARTESIAN_POINT('Ctrl Pts',(86.3174835015953,52.7877935499168,12.2577725351328));
#77911=CARTESIAN_POINT('Ctrl Pts',(86.3247131691019,52.7925385009175,12.3216167200773));
#77912=CARTESIAN_POINT('Ctrl Pts',(86.3355505626445,52.7972834519183,12.3849908574272));
#77913=CARTESIAN_POINT('Ctrl Pts',(86.3499021437454,52.8020284029191,12.4474823030581));
#77914=CARTESIAN_POINT('Ctrl Pts',(86.3642700270975,52.8067787438056,12.5100447339854));
#77915=CARTESIAN_POINT('Ctrl Pts',(86.3821599224672,52.8115290846921,12.5717220352282));
#77916=CARTESIAN_POINT('Ctrl Pts',(86.4034285223832,52.8162794255786,12.6321172846264));
#77917=CARTESIAN_POINT('Ctrl Pts',(86.4247516027314,52.8210419346674,12.6926672390503));
#77918=CARTESIAN_POINT('Ctrl Pts',(86.4494705067647,52.8258044437561,12.7519281542938));
#77919=CARTESIAN_POINT('Ctrl Pts',(86.4773939614703,52.8305669528449,12.8095236070127));
#77920=CARTESIAN_POINT('Ctrl Pts',(86.4977263091968,52.8340347540845,12.851461497023));
#77921=CARTESIAN_POINT('Ctrl Pts',(86.5197567014376,52.8375025553242,12.8925168392184));
#77922=CARTESIAN_POINT('Ctrl Pts',(86.5433968215242,52.8409703565639,12.9325539487693));
#77923=CARTESIAN_POINT('Ctrl Pts',(86.5747362525636,52.8455675801571,12.985630677195));
#77924=CARTESIAN_POINT('Ctrl Pts',(86.6090230548098,52.8501648037503,13.037114053001));
#77925=CARTESIAN_POINT('Ctrl Pts',(86.6460701587727,52.8547620273435,13.0866573196364));
#77926=CARTESIAN_POINT('Ctrl Pts',(86.6837516099672,52.8594379679145,13.1370489018124));
#77927=CARTESIAN_POINT('Ctrl Pts',(86.7242885925132,52.8641139084855,13.185432804658));
#77928=CARTESIAN_POINT('Ctrl Pts',(86.7674358396594,52.8687898490565,13.2314711556776));
#77929=CARTESIAN_POINT('Ctrl Pts',(86.8097400420211,52.8733744274301,13.2766099732558));
#77930=CARTESIAN_POINT('Ctrl Pts',(86.8545530587904,52.8779590058036,13.3194936839307));
#77931=CARTESIAN_POINT('Ctrl Pts',(86.901602145811,52.8825435841772,13.359835861584));
#77932=CARTESIAN_POINT('Ctrl Pts',(86.9486224772492,52.8871253605364,13.400153382801));
#77933=CARTESIAN_POINT('Ctrl Pts',(86.9978757834375,52.8917071368955,13.4379321203825));
#77934=CARTESIAN_POINT('Ctrl Pts',(87.049053695795,52.8962889132547,13.4729236452013));
#77935=CARTESIAN_POINT('Ctrl Pts',(87.1002191265607,52.9008695721813,13.5079066360665));
#77936=CARTESIAN_POINT('Ctrl Pts',(87.1533078116675,52.905450231108,13.5401034764192));
#77937=CARTESIAN_POINT('Ctrl Pts',(87.2079813162425,52.9100308900346,13.569308294774));
#77938=CARTESIAN_POINT('Ctrl Pts',(87.2646299889455,52.914777032619,13.5995681840786));
#77939=CARTESIAN_POINT('Ctrl Pts',(87.3229796991594,52.9195231752034,13.6266153986706));
#77940=CARTESIAN_POINT('Ctrl Pts',(87.3826271432278,52.9242693177877,13.6502734576051));
#77941=CARTESIAN_POINT('Ctrl Pts',(87.4402677827277,52.9288557790853,13.6731355545081));
#77942=CARTESIAN_POINT('Ctrl Pts',(87.4991196905869,52.9334422403829,13.6928328422381));
#77943=CARTESIAN_POINT('Ctrl Pts',(87.5588019903555,52.9380287016805,13.7092564607126));
#77944=CARTESIAN_POINT('Ctrl Pts',(87.6216011200086,52.9428546849083,13.7265377811367));
#77945=CARTESIAN_POINT('Ctrl Pts',(87.6853191247605,52.947680668136,13.740193984382));
#77946=CARTESIAN_POINT('Ctrl Pts',(87.749501534727,52.9525066513638,13.7501595495261));
#77947=CARTESIAN_POINT('Ctrl Pts',(87.8136839446935,52.9573326345915,13.7601251146701));
#77948=CARTESIAN_POINT('Ctrl Pts',(87.8783301074432,52.9621586178193,13.7664000561262));
#77949=CARTESIAN_POINT('Ctrl Pts',(87.9429841694157,52.9669846010471,13.7689822906859));
#77950=CARTESIAN_POINT('Ctrl Pts',(88.0045735212603,52.9715818246389,13.7714421230305));
#77951=CARTESIAN_POINT('Ctrl Pts',(88.066422914334,52.9761790482308,13.7705615739378));
#77952=CARTESIAN_POINT('Ctrl Pts',(88.1281395648571,52.9807762718227,13.7663097241224));
#77953=CARTESIAN_POINT('Ctrl Pts',(88.1909129723994,52.9854522123939,13.7619850710666));
#77954=CARTESIAN_POINT('Ctrl Pts',(88.2535485227054,52.990128152965,13.7541724628825));
#77955=CARTESIAN_POINT('Ctrl Pts',(88.3156293295559,52.9948040935361,13.7428946917366));
#77956=CARTESIAN_POINT('Ctrl Pts',(88.3764971528496,52.9993886719084,13.7318372745399));
#77957=CARTESIAN_POINT('Ctrl Pts',(88.4368311909235,53.0039732502806,13.7174489820524));
#77958=CARTESIAN_POINT('Ctrl Pts',(88.4962428750387,53.0085578286528,13.6998035952415));
#77959=CARTESIAN_POINT('Ctrl Pts',(88.5556182477674,53.0131396050106,13.6821689929838));
#77960=CARTESIAN_POINT('Ctrl Pts',(88.614071897359,53.0177213813683,13.6612813882623));
#77961=CARTESIAN_POINT('Ctrl Pts',(88.6712278545075,53.0223031577261,13.6372651003992));
#77962=CARTESIAN_POINT('Ctrl Pts',(88.7283698721008,53.0268838166513,13.6132546697797));
#77963=CARTESIAN_POINT('Ctrl Pts',(88.7842143564401,53.0314644755766,13.5861172678811));
#77964=CARTESIAN_POINT('Ctrl Pts',(88.8384047838757,53.0360451345018,13.5560255565659));
#77965=CARTESIAN_POINT('Ctrl Pts',(88.894552927535,53.0407912770875,13.5248467338506));
#77966=CARTESIAN_POINT('Ctrl Pts',(88.948924675794,53.0455374196733,13.4904962827174));
#77967=CARTESIAN_POINT('Ctrl Pts',(89.0011530118701,53.050283562259,13.4532173040604));
#77968=CARTESIAN_POINT('Ctrl Pts',(89.0516241550464,53.0548700235552,13.4171925556073));
#77969=CARTESIAN_POINT('Ctrl Pts',(89.1000934654956,53.0594564848514,13.3784336063825));
#77970=CARTESIAN_POINT('Ctrl Pts',(89.1462629006426,53.0640429461476,13.3372013931807));
#77971=CARTESIAN_POINT('Ctrl Pts',(89.1948434740714,53.068868929378,13.2938158816469));
#77972=CARTESIAN_POINT('Ctrl Pts',(89.2408769065255,53.0736949126085,13.247692144612));
#77973=CARTESIAN_POINT('Ctrl Pts',(89.2840616485871,53.0785208958389,13.1991764533808));
#77974=CARTESIAN_POINT('Ctrl Pts',(89.3272463906486,53.0833468790694,13.1506607621496));
#77975=CARTESIAN_POINT('Ctrl Pts',(89.3675821005486,53.0881728622998,13.0997536726613));
#77976=CARTESIAN_POINT('Ctrl Pts',(89.4048197737318,53.0929988455303,13.0468370272141));
#77977=CARTESIAN_POINT('Ctrl Pts',(89.4402923192196,53.0975960691222,12.9964287188472));
#77978=CARTESIAN_POINT('Ctrl Pts',(89.473099585584,53.1021932927141,12.9439901255787));
#77979=CARTESIAN_POINT('Ctrl Pts',(89.5030025514424,53.106790516306,12.8898344627953));
#77980=CARTESIAN_POINT('Ctrl Pts',(89.5334175374574,53.1114664568771,12.8347515076803));
#77981=CARTESIAN_POINT('Ctrl Pts',(89.5608274449313,53.1161423974483,12.7778925068007));
#77982=CARTESIAN_POINT('Ctrl Pts',(89.5850253034763,53.1208183380194,12.7196200575383));
#77983=CARTESIAN_POINT('Ctrl Pts',(89.6087503652583,53.1254029163916,12.6624861811512));
#77984=CARTESIAN_POINT('Ctrl Pts',(89.6293875637479,53.1299874947638,12.6039940863905));
#77985=CARTESIAN_POINT('Ctrl Pts',(89.6467881246946,53.1345720731361,12.5445102367852));
#77986=CARTESIAN_POINT('Ctrl Pts',(89.6641780507214,53.1391538494938,12.4850627426728));
#77987=CARTESIAN_POINT('Ctrl Pts',(89.67833511902,53.1437356258516,12.424625183169));
#77988=CARTESIAN_POINT('Ctrl Pts',(89.6891598475981,53.1483174022094,12.3635808486939));
#77989=CARTESIAN_POINT('Ctrl Pts',(89.6999819361733,53.1528980611346,12.3025514020959));
#77990=CARTESIAN_POINT('Ctrl Pts',(89.7074732095439,53.1574787200599,12.2409159753006));
#77991=CARTESIAN_POINT('Ctrl Pts',(89.7115853466096,53.1620593789851,12.1790677429547));
#77992=CARTESIAN_POINT('Ctrl Pts',(89.715846041231,53.1668055215708,12.1149851438841));
#77993=CARTESIAN_POINT('Ctrl Pts',(89.7164786690044,53.1715516641565,12.0506746448662));
#77994=CARTESIAN_POINT('Ctrl Pts',(89.7134883946887,53.1762978067422,11.9865764420948));
#77995=CARTESIAN_POINT('Ctrl Pts',(89.7105987264652,53.1808842680384,11.9246347871911));
#77996=CARTESIAN_POINT('Ctrl Pts',(89.7043262066928,53.1854707293346,11.8628918872255));
#77997=CARTESIAN_POINT('Ctrl Pts',(89.6947283959729,53.1900571906308,11.8017396658699));
#77998=CARTESIAN_POINT('Ctrl Pts',(89.6846293521585,53.1948831738613,11.7373938498458));
#77999=CARTESIAN_POINT('Ctrl Pts',(89.670848301016,53.1997091570917,11.6737027307551));
#78000=CARTESIAN_POINT('Ctrl Pts',(89.6535125923678,53.2045351403222,11.6111074637751));
#78001=CARTESIAN_POINT('Ctrl Pts',(89.6361768837197,53.2093611235526,11.5485121967951));
#78002=CARTESIAN_POINT('Ctrl Pts',(89.6152867992471,53.214187106783,11.487013370594));
#78003=CARTESIAN_POINT('Ctrl Pts',(89.5910280729863,53.2190130900135,11.4270272899605));
#78004=CARTESIAN_POINT('Ctrl Pts',(89.5679192507301,53.2236103136057,11.369884649399));
#78005=CARTESIAN_POINT('Ctrl Pts',(89.541659099045,53.2282075371979,11.3138799422366));
#78006=CARTESIAN_POINT('Ctrl Pts',(89.512381111906,53.2328047607902,11.2593838630353));
#78007=CARTESIAN_POINT('Ctrl Pts',(89.4826018059495,53.2374807013613,11.2039546626513));
#78008=CARTESIAN_POINT('Ctrl Pts',(89.4497004554622,53.2421566419324,11.1500867673443));
#78009=CARTESIAN_POINT('Ctrl Pts',(89.4138694256987,53.2468325825035,11.09815072969));
#78010=CARTESIAN_POINT('Ctrl Pts',(89.3787384907302,53.2514171608761,11.0472294591209));
#78011=CARTESIAN_POINT('Ctrl Pts',(89.3407916345206,53.2560017392486,10.9981656719112));
#78012=CARTESIAN_POINT('Ctrl Pts',(89.3002560358696,53.2605863176212,10.9512831258235));
#78013=CARTESIAN_POINT('Ctrl Pts',(89.2597452118706,53.2651680939793,10.9044292335314));
#78014=CARTESIAN_POINT('Ctrl Pts',(89.2166491149424,53.2697498703374,10.8597543232163));
#78015=CARTESIAN_POINT('Ctrl Pts',(89.1712357965721,53.2743316466955,10.8175498680553));
#78016=CARTESIAN_POINT('Ctrl Pts',(89.1258335538883,53.2789123056211,10.7753557059831));
#78017=CARTESIAN_POINT('Ctrl Pts',(89.0781155843645,53.2834929645467,10.7356311493715));
#78018=CARTESIAN_POINT('Ctrl Pts',(89.0283859930401,53.2880736234723,10.6986300512423));
#78019=CARTESIAN_POINT('Ctrl Pts',(88.9768598403684,53.2928197660577,10.660292229023));
#78020=CARTESIAN_POINT('Ctrl Pts',(88.923174365156,53.2975659086431,10.6248788099224));
#78021=CARTESIAN_POINT('Ctrl Pts',(88.8677021869033,53.3023120512284,10.5926242167881));
#78022=CARTESIAN_POINT('Ctrl Pts',(88.8140963387823,53.306898512525,10.5614548112371));
#78023=CARTESIAN_POINT('Ctrl Pts',(88.7588226143968,53.3114849738215,10.5332352153234));
#78024=CARTESIAN_POINT('Ctrl Pts',(88.7022414979199,53.3160714351181,10.508129650082));
#78025=CARTESIAN_POINT('Ctrl Pts',(88.6427055067527,53.3208974183479,10.4817129795827));
#78026=CARTESIAN_POINT('Ctrl Pts',(88.58172242412,53.3257234015777,10.4587447481971));
#78027=CARTESIAN_POINT('Ctrl Pts',(88.5197319482119,53.3305493848074,10.4393572486657));
#78028=CARTESIAN_POINT('Ctrl Pts',(88.4577414723038,53.3353753680372,10.4199697491342));
#78029=CARTESIAN_POINT('Ctrl Pts',(88.3947442504564,53.340201351267,10.4041630641035));
#78030=CARTESIAN_POINT('Ctrl Pts',(88.3311907710474,53.3450273344968,10.3920069576799));
#78031=CARTESIAN_POINT('Ctrl Pts',(88.2706498323445,53.3496245580888,10.3804270709342));
#78032=CARTESIAN_POINT('Ctrl Pts',(88.2093556183969,53.3542217816809,10.3721118964261));
#78033=CARTESIAN_POINT('Ctrl Pts',(88.1476919645212,53.3588190052729,10.3671503473128));
#78034=CARTESIAN_POINT('Ctrl Pts',(88.0849724610756,53.363494945844,10.3621038429761));
#78035=CARTESIAN_POINT('Ctrl Pts',(88.0218712499876,53.3681708864152,10.3605270842887));
#78036=CARTESIAN_POINT('Ctrl Pts',(87.9588039789972,53.3728468269863,10.3624594483865));
#78037=CARTESIAN_POINT('Ctrl Pts',(87.8969689658722,53.3774314053587,10.3643540564372));
#78038=CARTESIAN_POINT('Ctrl Pts',(87.8351671116439,53.382015983731,10.3696218762146));
#78039=CARTESIAN_POINT('Ctrl Pts',(87.7737936335629,53.3866005621034,10.3782476558091));
#78040=CARTESIAN_POINT('Ctrl Pts',(87.7124576658829,53.3911823384613,10.3868681634774));
#78041=CARTESIAN_POINT('Ctrl Pts',(87.6515500582537,53.3957641148193,10.3988424907949));
#78042=CARTESIAN_POINT('Ctrl Pts',(87.5914610742573,53.4003458911772,10.4141035367231));
#78043=CARTESIAN_POINT('Ctrl Pts',(87.5313867451412,53.4049265501026,10.4293608606913));
#78044=CARTESIAN_POINT('Ctrl Pts',(87.4721311364827,53.409507209028,10.4479031867508));
#78045=CARTESIAN_POINT('Ctrl Pts',(87.4140724617767,53.4140878679534,10.4696127193846));
#78046=CARTESIAN_POINT('Ctrl Pts',(87.353916324206,53.418834010539,10.4921065437499));
#78047=CARTESIAN_POINT('Ctrl Pts',(87.2950458257325,53.4235801531245,10.518000653331));
#78048=CARTESIAN_POINT('Ctrl Pts',(87.2378600183096,53.4283262957101,10.5471091532596));
#78049=CARTESIAN_POINT('Ctrl Pts',(87.1825981951091,53.4329127570064,10.5752383141332));
#78050=CARTESIAN_POINT('Ctrl Pts',(87.1289099154122,53.4374992183028,10.6063686662655));
#78051=CARTESIAN_POINT('Ctrl Pts',(87.0771286709566,53.4420856795992,10.6402864325571));
#78052=CARTESIAN_POINT('Ctrl Pts',(87.0226432188333,53.4469116628293,10.6759755097672));
#78053=CARTESIAN_POINT('Ctrl Pts',(86.9702699727955,53.4517376460594,10.714750748264));
#78054=CARTESIAN_POINT('Ctrl Pts',(86.9203585665297,53.4565636292896,10.756314503708));
#78055=CARTESIAN_POINT('Ctrl Pts',(86.8704471602638,53.4613896125197,10.7978782591519));
#78056=CARTESIAN_POINT('Ctrl Pts',(86.8229980143172,53.4662155957499,10.8422300325295));
#78057=CARTESIAN_POINT('Ctrl Pts',(86.7783140833319,53.47104157898,10.8890291989824));
#78058=CARTESIAN_POINT('Ctrl Pts',(86.7362981532647,53.4755794110246,10.9330340674335));
#78059=CARTESIAN_POINT('Ctrl Pts',(86.6965446275607,53.4801172430691,10.9793934087281));
#78060=CARTESIAN_POINT('Ctrl Pts',(86.6593331863823,53.4846550751137,11.0278421793559));
#78061=CARTESIAN_POINT('Ctrl Pts',(86.6221740909261,53.4891865237426,11.0762227965929));
#78062=CARTESIAN_POINT('Ctrl Pts',(86.5875503140188,53.4937179723716,11.1266866120252));
#78063=CARTESIAN_POINT('Ctrl Pts',(86.5557041194029,53.4982494210005,11.1789325079132));
#78064=CARTESIAN_POINT('Ctrl Pts',(86.5238903094915,53.5027762615553,11.2311252744424));
#78065=CARTESIAN_POINT('Ctrl Pts',(86.4948487563883,53.5073031021101,11.2850960865296));
#78066=CARTESIAN_POINT('Ctrl Pts',(86.4687795277154,53.511829942665,11.3405133698914));
#78067=CARTESIAN_POINT('Ctrl Pts',(86.4421402312034,53.5164557737287,11.3971424885313));
#78068=CARTESIAN_POINT('Ctrl Pts',(86.4186051288118,53.5210816047925,11.4552816346984));
#78069=CARTESIAN_POINT('Ctrl Pts',(86.3983382336703,53.5257074358562,11.5145502171383));
#78070=CARTESIAN_POINT('Ctrl Pts',(86.378515920084,53.5302317931049,11.5725186636484));
#78071=CARTESIAN_POINT('Ctrl Pts',(86.3618200008801,53.5347561503536,11.631566963447));
#78072=CARTESIAN_POINT('Ctrl Pts',(86.3483543202793,53.5392805076024,11.6913212318451));
#78073=CARTESIAN_POINT('Ctrl Pts',(86.3344356204183,53.5439570755736,11.7530857836639));
#78074=CARTESIAN_POINT('Ctrl Pts',(86.3239685799923,53.5486336435449,11.8156040867182));
#78075=CARTESIAN_POINT('Ctrl Pts',(86.3170104412882,53.5533102115161,11.8784521112473));
#78076=CARTESIAN_POINT('Ctrl Pts',(86.3100523025842,53.5579867794874,11.9413001357764));
#78077=CARTESIAN_POINT('Ctrl Pts',(86.306603075047,53.5626633474586,12.0044772662455));
#78078=CARTESIAN_POINT('Ctrl Pts',(86.3066607114366,53.5673399154299,12.0675572601897));
#78079=CARTESIAN_POINT('',(86.3066601203479,54.3610899154771,12.0653595099723));
#78080=CARTESIAN_POINT('Ctrl Pts',(86.3066607114372,53.5673399154776,12.0675572608336));
#78081=CARTESIAN_POINT('Ctrl Pts',(86.3067358739435,53.5734385352263,12.1498186326717));
#78082=CARTESIAN_POINT('Ctrl Pts',(86.3127703680478,53.579537154975,12.231815876902));
#78083=CARTESIAN_POINT('Ctrl Pts',(86.324628267231,53.5856357747237,12.312830335489));
#78084=CARTESIAN_POINT('Ctrl Pts',(86.332029821036,53.5894424576368,12.363398557141));
#78085=CARTESIAN_POINT('Ctrl Pts',(86.3416992924877,53.59324914055,12.4135844802534));
#78086=CARTESIAN_POINT('Ctrl Pts',(86.3535945960656,53.5970558234632,12.4632180290585));
#78087=CARTESIAN_POINT('Ctrl Pts',(86.3679602187063,53.6016530470553,12.5231590661058));
#78088=CARTESIAN_POINT('Ctrl Pts',(86.3856112274446,53.6062502706474,12.5824428301661));
#78089=CARTESIAN_POINT('Ctrl Pts',(86.4064706649311,53.6108474942395,12.6406829112678));
#78090=CARTESIAN_POINT('Ctrl Pts',(86.4276872727553,53.6155234348106,12.6999202210557));
#78091=CARTESIAN_POINT('Ctrl Pts',(86.4522231863206,53.6201993753817,12.7580772322774));
#78092=CARTESIAN_POINT('Ctrl Pts',(86.4799432088402,53.6248753159529,12.8147589317287));
#78093=CARTESIAN_POINT('Ctrl Pts',(86.5071216157924,53.6294598943253,12.8703331396263));
#78094=CARTESIAN_POINT('Ctrl Pts',(86.5373605891585,53.6340444726977,12.9244886896752));
#78095=CARTESIAN_POINT('Ctrl Pts',(86.5704835546859,53.6386290510701,12.9768716739365));
#78096=CARTESIAN_POINT('Ctrl Pts',(86.6035862760337,53.6432108274281,13.02922264263));
#78097=CARTESIAN_POINT('Ctrl Pts',(86.639569222979,53.6477926037861,13.0798027643285));
#78098=CARTESIAN_POINT('Ctrl Pts',(86.6782106069416,53.652374380144,13.128283987148));
#78099=CARTESIAN_POINT('Ctrl Pts',(86.7168425667998,53.6569550390695,13.1767533860611));
#78100=CARTESIAN_POINT('Ctrl Pts',(86.758131359452,53.6615356979949,13.2231245043846));
#78101=CARTESIAN_POINT('Ctrl Pts',(86.8018139552308,53.6661163569204,13.267101138429));
#78102=CARTESIAN_POINT('Ctrl Pts',(86.8470746549347,53.6708624995059,13.3126664990031));
#78103=CARTESIAN_POINT('Ctrl Pts',(86.8949050649616,53.6756086420914,13.3556605960175));
#78104=CARTESIAN_POINT('Ctrl Pts',(86.9449715152674,53.6803547846769,13.395796264598));
#78105=CARTESIAN_POINT('Ctrl Pts',(86.9933535081046,53.6849412459733,13.4345815912572));
#78106=CARTESIAN_POINT('Ctrl Pts',(87.0438229889342,53.6895277072697,13.4706975393349));
#78107=CARTESIAN_POINT('Ctrl Pts',(87.0960478619781,53.6941141685661,13.5039281695305));
#78108=CARTESIAN_POINT('Ctrl Pts',(87.1510001106102,53.6989401517961,13.5388942258609));
#78109=CARTESIAN_POINT('Ctrl Pts',(87.207895568258,53.7037661350262,13.5706650130704));
#78110=CARTESIAN_POINT('Ctrl Pts',(87.266319061639,53.7085921182562,13.5990444010667));
#78111=CARTESIAN_POINT('Ctrl Pts',(87.3247425550201,53.7134181014862,13.6274237890629));
#78112=CARTESIAN_POINT('Ctrl Pts',(87.3846934562525,53.7182440847163,13.6524115999727));
#78113=CARTESIAN_POINT('Ctrl Pts',(87.4457366346986,53.7230700679463,13.6738719362711));
#78114=CARTESIAN_POINT('Ctrl Pts',(87.5038862648798,53.7276672915384,13.6943150169081));
#78115=CARTESIAN_POINT('Ctrl Pts',(87.563265695465,53.7322645151305,13.7116414710749));
#78116=CARTESIAN_POINT('Ctrl Pts',(87.6235085536853,53.7368617387226,13.7257063639792));
#78117=CARTESIAN_POINT('Ctrl Pts',(87.6847829335868,53.7415376792937,13.740012086127));
#78118=CARTESIAN_POINT('Ctrl Pts',(87.74695011912,53.7462136198648,13.7509432366428));
#78119=CARTESIAN_POINT('Ctrl Pts',(87.8096049207595,53.7508895604359,13.7583991425363));
#78120=CARTESIAN_POINT('Ctrl Pts',(87.8710355236841,53.7554741388083,13.7657093690856));
#78121=CARTESIAN_POINT('Ctrl Pts',(87.9329343295529,53.7600587171808,13.7696788707333));
#78122=CARTESIAN_POINT('Ctrl Pts',(87.9949082391577,53.7646432955532,13.7702640320188));
#78123=CARTESIAN_POINT('Ctrl Pts',(88.0568442713882,53.7692250719111,13.7708488356639));
#78124=CARTESIAN_POINT('Ctrl Pts',(88.1188548083692,53.7738068482691,13.7680533955879));
#78125=CARTESIAN_POINT('Ctrl Pts',(88.1805439489161,53.7783886246271,13.7618861061362));
#78126=CARTESIAN_POINT('Ctrl Pts',(88.2422180443265,53.7829692835525,13.755720320802));
#78127=CARTESIAN_POINT('Ctrl Pts',(88.303570392612,53.787549942478,13.7461843691937));
#78128=CARTESIAN_POINT('Ctrl Pts',(88.3642094798163,53.7921306014034,13.7333385675885));
#78129=CARTESIAN_POINT('Ctrl Pts',(88.4270392514299,53.7968767439889,13.7200286907704));
#78130=CARTESIAN_POINT('Ctrl Pts',(88.4891026577919,53.8016228865744,13.7031652957325));
#78131=CARTESIAN_POINT('Ctrl Pts',(88.5499774633923,53.80636902916,13.6828729478704));
#78132=CARTESIAN_POINT('Ctrl Pts',(88.608804170509,53.8109554904564,13.6632633246015));
#78133=CARTESIAN_POINT('Ctrl Pts',(88.6665205270712,53.8155419517528,13.6404520908354));
#78134=CARTESIAN_POINT('Ctrl Pts',(88.7227649895615,53.8201284130492,13.6146011220564));
#78135=CARTESIAN_POINT('Ctrl Pts',(88.7819467454341,53.8249543962792,13.5874001202937));
#78136=CARTESIAN_POINT('Ctrl Pts',(88.8394980822379,53.8297803795093,13.5568334774783));
#78137=CARTESIAN_POINT('Ctrl Pts',(88.8950290374551,53.8346063627394,13.5231436087552));
#78138=CARTESIAN_POINT('Ctrl Pts',(88.9505599926724,53.8394323459695,13.4894537400321));
#78139=CARTESIAN_POINT('Ctrl Pts',(89.0040700763058,53.8442583291995,13.4526410764199));
#78140=CARTESIAN_POINT('Ctrl Pts',(89.0552091036478,53.8490843124296,13.41299746973));
#78141=CARTESIAN_POINT('Ctrl Pts',(89.1039240559726,53.8536815360217,13.3752330359843));
#78142=CARTESIAN_POINT('Ctrl Pts',(89.1506877066357,53.8582787596138,13.3347449665407));
#78143=CARTESIAN_POINT('Ctrl Pts',(89.1951795727132,53.8628759832058,13.291762446467));
#78144=CARTESIAN_POINT('Ctrl Pts',(89.2404332606208,53.867551923777,13.2480439486744));
#78145=CARTESIAN_POINT('Ctrl Pts',(89.283336156128,53.8722278643481,13.2017450224899));
#78146=CARTESIAN_POINT('Ctrl Pts',(89.3235839074266,53.8769038049192,13.1531514713069));
#78147=CARTESIAN_POINT('Ctrl Pts',(89.3630452665553,53.8814883832916,13.1055073790856));
#78148=CARTESIAN_POINT('Ctrl Pts',(89.3999539646657,53.886072961664,13.0556579346042));
#78149=CARTESIAN_POINT('Ctrl Pts',(89.4340601429617,53.8906575400365,13.003909731858));
#78150=CARTESIAN_POINT('Ctrl Pts',(89.4681454761555,53.8952393163944,12.9521931567121));
#78151=CARTESIAN_POINT('Ctrl Pts',(89.4994314063208,53.8998210927524,12.8985805485348));
#78152=CARTESIAN_POINT('Ctrl Pts',(89.5277102494122,53.9044028691103,12.8434090653755));
#78153=CARTESIAN_POINT('Ctrl Pts',(89.5559821956811,53.9089835280358,12.7882510377853));
#78154=CARTESIAN_POINT('Ctrl Pts',(89.581248278671,53.9135641869612,12.731535342748));
#78155=CARTESIAN_POINT('Ctrl Pts',(89.6033468146777,53.9181448458867,12.6736236149013));
#78156=CARTESIAN_POINT('Ctrl Pts',(89.6262436957873,53.9228909884722,12.6136197328818));
#78157=CARTESIAN_POINT('Ctrl Pts',(89.6457395154445,53.9276371310577,12.552332266648));
#78158=CARTESIAN_POINT('Ctrl Pts',(89.6617099036571,53.9323832736432,12.4901835093074));
#78159=CARTESIAN_POINT('Ctrl Pts',(89.6771429771701,53.9369697349396,12.430125711838));
#78160=CARTESIAN_POINT('Ctrl Pts',(89.6892840571562,53.941556196236,12.369264193803));
#78161=CARTESIAN_POINT('Ctrl Pts',(89.69807303788,53.9461426575324,12.3079904966283));
#78162=CARTESIAN_POINT('Ctrl Pts',(89.7073210116099,53.9509686407625,12.2435168608772));
#78163=CARTESIAN_POINT('Ctrl Pts',(89.7128571017517,53.9557946239926,12.1785874551594));
#78164=CARTESIAN_POINT('Ctrl Pts',(89.7146734512133,53.9606206072226,12.1136613809167));
#78165=CARTESIAN_POINT('Ctrl Pts',(89.7164898006749,53.9654465904527,12.0487353066739));
#78166=CARTESIAN_POINT('Ctrl Pts',(89.7145865057904,53.9702725736828,11.9838132093474));
#78167=CARTESIAN_POINT('Ctrl Pts',(89.709018817693,53.9750985569129,11.919347586585));
#78168=CARTESIAN_POINT('Ctrl Pts',(89.7037150472789,53.979695780505,11.8579377416451));
#78169=CARTESIAN_POINT('Ctrl Pts',(89.6950647092455,53.984293004097,11.7966899299085));
#78170=CARTESIAN_POINT('Ctrl Pts',(89.6830865172788,53.9888902276891,11.7359977055616));
#78171=CARTESIAN_POINT('Ctrl Pts',(89.6709032260674,53.9935661682602,11.6742662651626));
#78172=CARTESIAN_POINT('Ctrl Pts',(89.6552769954437,53.9982421088314,11.6131101540597));
#78173=CARTESIAN_POINT('Ctrl Pts',(89.6362828548449,54.0029180494025,11.5529400840574));
#78174=CARTESIAN_POINT('Ctrl Pts',(89.6176598366806,54.0075026277749,11.493945664132));
#78175=CARTESIAN_POINT('Ctrl Pts',(89.5957994952143,54.0120872061473,11.4358996084322));
#78176=CARTESIAN_POINT('Ctrl Pts',(89.5708238834506,54.0166717845197,11.3791781248263));
#78177=CARTESIAN_POINT('Ctrl Pts',(89.5458635363458,54.0212535608777,11.3224913084034));
#78178=CARTESIAN_POINT('Ctrl Pts',(89.5177918990106,54.0258353372356,11.2671279237597));
#78179=CARTESIAN_POINT('Ctrl Pts',(89.4867795774909,54.0304171135936,11.2134453247675));
#78180=CARTESIAN_POINT('Ctrl Pts',(89.4557748194517,54.0349977725191,11.1597758182261));
#78181=CARTESIAN_POINT('Ctrl Pts',(89.4218310554884,54.0395784314445,11.1077867241655));
#78182=CARTESIAN_POINT('Ctrl Pts',(89.3851644054752,54.04415909037,11.0578100266691));
#78183=CARTESIAN_POINT('Ctrl Pts',(89.3471731138449,54.0489052329555,11.0060278407147));
#78184=CARTESIAN_POINT('Ctrl Pts',(89.3062587244168,54.053651375541,10.956406744));
#78185=CARTESIAN_POINT('Ctrl Pts',(89.2627085564407,54.0583975181265,10.9092802736474));
#78186=CARTESIAN_POINT('Ctrl Pts',(89.2206236092914,54.0629839794229,10.8637393467971));
#78187=CARTESIAN_POINT('Ctrl Pts',(89.1760778662624,54.0675704407193,10.8205281563628));
#78188=CARTESIAN_POINT('Ctrl Pts',(89.1293676683184,54.0721569020157,10.7799095700301));
#78189=CARTESIAN_POINT('Ctrl Pts',(89.0802180914697,54.0769828852457,10.7371697312301));
#78190=CARTESIAN_POINT('Ctrl Pts',(89.028672291556,54.0818088684758,10.6973011153504));
#78191=CARTESIAN_POINT('Ctrl Pts',(88.9751117077413,54.0866348517059,10.6605593393543));
#78192=CARTESIAN_POINT('Ctrl Pts',(88.9215511239265,54.091460834936,10.6238175633582));
#78193=CARTESIAN_POINT('Ctrl Pts',(88.8659763507109,54.096286818166,10.5902028964001));
#78194=CARTESIAN_POINT('Ctrl Pts',(88.8087975090945,54.1011128013961,10.5599143549975));
#78195=CARTESIAN_POINT('Ctrl Pts',(88.7543290397454,54.1057100249882,10.531061540873));
#78196=CARTESIAN_POINT('Ctrl Pts',(88.6981815237835,54.1103072485803,10.5051081356642));
#78197=CARTESIAN_POINT('Ctrl Pts',(88.6406957446929,54.1149044721723,10.4822518809117));
#78198=CARTESIAN_POINT('Ctrl Pts',(88.5822256526191,54.1195804127435,10.4590042648755));
#78199=CARTESIAN_POINT('Ctrl Pts',(88.5223714607889,54.1242563533146,10.4389611930283));
#78200=CARTESIAN_POINT('Ctrl Pts',(88.4615189127579,54.1289322938857,10.4222824011262));
#78201=CARTESIAN_POINT('Ctrl Pts',(88.4018553495955,54.1335168722581,10.4059294925575));
#78202=CARTESIAN_POINT('Ctrl Pts',(88.3412326071423,54.1381014506306,10.3928107194147));
#78203=CARTESIAN_POINT('Ctrl Pts',(88.2800329469916,54.142686029003,10.3830275970673));
#78204=CARTESIAN_POINT('Ctrl Pts',(88.2188706910073,54.1472678053609,10.3732504539939));
#78205=CARTESIAN_POINT('Ctrl Pts',(88.1571327181066,54.1518495817189,10.366804999472));
#78206=CARTESIAN_POINT('Ctrl Pts',(88.0952117853512,54.1564313580769,10.3637417320489));
#78207=CARTESIAN_POINT('Ctrl Pts',(88.0333059542634,54.1610120170023,10.3606792117147));
#78208=CARTESIAN_POINT('Ctrl Pts',(87.9712177600988,54.1655926759278,10.36099726613));
#78209=CARTESIAN_POINT('Ctrl Pts',(87.9093433328666,54.1701733348532,10.3646943961688));
#78210=CARTESIAN_POINT('Ctrl Pts',(87.8452335925824,54.1749194774387,10.3685250909678));
#78211=CARTESIAN_POINT('Ctrl Pts',(87.7813539444909,54.1796656200243,10.3759837142419));
#78212=CARTESIAN_POINT('Ctrl Pts',(87.7181404417955,54.1844117626098,10.3870097931291));
#78213=CARTESIAN_POINT('Ctrl Pts',(87.6570537217279,54.1889982239062,10.3976649058141));
#78214=CARTESIAN_POINT('Ctrl Pts',(87.5965895299048,54.1935846852026,10.4116510313652));
#78215=CARTESIAN_POINT('Ctrl Pts',(87.5371294420067,54.198171146499,10.4288617865717));
#78216=CARTESIAN_POINT('Ctrl Pts',(87.4745641289013,54.202997129729,10.4469713509256));
#78217=CARTESIAN_POINT('Ctrl Pts',(87.4131112825313,54.2078231129591,10.468651380767));
#78218=CARTESIAN_POINT('Ctrl Pts',(87.3531925442499,54.2126490961892,10.4937200673037));
#78219=CARTESIAN_POINT('Ctrl Pts',(87.2932738059684,54.2174750794192,10.5187887538404));
#78220=CARTESIAN_POINT('Ctrl Pts',(87.2348897243538,54.2223010626493,10.5472457436092));
#78221=CARTESIAN_POINT('Ctrl Pts',(87.1784299465193,54.2271270458794,10.5788544315881));
#78222=CARTESIAN_POINT('Ctrl Pts',(87.1246464561318,54.2317242694714,10.608964815144));
#78223=CARTESIAN_POINT('Ctrl Pts',(87.0723881077518,54.2363214930635,10.6420584371157));
#78224=CARTESIAN_POINT('Ctrl Pts',(87.0220058687739,54.2409187166556,10.6779562528507));
#78225=CARTESIAN_POINT('Ctrl Pts',(86.9707609487516,54.2455946572267,10.7144687368853));
#78226=CARTESIAN_POINT('Ctrl Pts',(86.9214575001497,54.2502705977978,10.7538821732325));
#78227=CARTESIAN_POINT('Ctrl Pts',(86.8744389471863,54.254946538369,10.7959591310407));
#78228=CARTESIAN_POINT('Ctrl Pts',(86.8283390796325,54.2595311167414,10.8372139562058));
#78229=CARTESIAN_POINT('Ctrl Pts',(86.7844360200587,54.2641156951138,10.8810287992545));
#78230=CARTESIAN_POINT('Ctrl Pts',(86.7430223918915,54.2687002734862,10.9271375759402));
#78231=CARTESIAN_POINT('Ctrl Pts',(86.7016340750124,54.2732820498441,10.9732181717446));
#78232=CARTESIAN_POINT('Ctrl Pts',(86.6627325120772,54.2778638262021,11.0215895432681));
#78233=CARTESIAN_POINT('Ctrl Pts',(86.6265731589287,54.28244560256,11.0719491173378));
#78234=CARTESIAN_POINT('Ctrl Pts',(86.5904226245513,54.2870262614855,11.1222964093971));
#78235=CARTESIAN_POINT('Ctrl Pts',(86.5570132690835,54.2916069204109,11.1746305281004));
#78236=CARTESIAN_POINT('Ctrl Pts',(86.5265586935049,54.2961875793364,11.2286178631168));
#78237=CARTESIAN_POINT('Ctrl Pts',(86.4950038974746,54.3009337219219,11.2845555773123));
#78238=CARTESIAN_POINT('Ctrl Pts',(86.4666218026833,54.3056798645074,11.3422677701031));
#78239=CARTESIAN_POINT('Ctrl Pts',(86.441598119318,54.3104260070929,11.4013553035554));
#78240=CARTESIAN_POINT('Ctrl Pts',(86.4174163436591,54.3150124683893,11.4584548702869));
#78241=CARTESIAN_POINT('Ctrl Pts',(86.3963706809794,54.3195989296857,11.5168381751189));
#78242=CARTESIAN_POINT('Ctrl Pts',(86.3785787226685,54.3241853909821,11.5761269461223));
#78243=CARTESIAN_POINT('Ctrl Pts',(86.3598576026394,54.3290113742121,11.6385119955326));
#78244=CARTESIAN_POINT('Ctrl Pts',(86.3447395068377,54.3338373574422,11.7018990541506));
#78245=CARTESIAN_POINT('Ctrl Pts',(86.3333003915963,54.3386633406723,11.7658352792848));
#78246=CARTESIAN_POINT('Ctrl Pts',(86.3218612763549,54.3434893239023,11.8297715044191));
#78247=CARTESIAN_POINT('Ctrl Pts',(86.3141011422701,54.3483153071324,11.8942562434794));
#78248=CARTESIAN_POINT('Ctrl Pts',(86.3100325565661,54.3531412903625,11.9588338114055));
#78249=CARTESIAN_POINT('Ctrl Pts',(86.3077988381869,54.3557908320516,11.9942879251569));
#78250=CARTESIAN_POINT('Ctrl Pts',(86.3066734788713,54.3584403737407,12.0298125996632));
#78251=CARTESIAN_POINT('Ctrl Pts',(86.3066601203481,54.3610899154298,12.0653595093375));
#78252=CARTESIAN_POINT('',(86.3066603887547,55.1548399153721,12.0648488527018));
#78253=CARTESIAN_POINT('Ctrl Pts',(86.3066601203479,54.3610899154771,12.0653595099723));
#78254=CARTESIAN_POINT('Ctrl Pts',(86.306637159949,54.3656439064994,12.1264569851298));
#78255=CARTESIAN_POINT('Ctrl Pts',(86.3099038103981,54.3701978975217,12.1876878311977));
#78256=CARTESIAN_POINT('Ctrl Pts',(86.3164768878567,54.374751888544,12.2486643315267));
#78257=CARTESIAN_POINT('Ctrl Pts',(86.3230390949028,54.379298348275,12.3095399902466));
#78258=CARTESIAN_POINT('Ctrl Pts',(86.3328968232668,54.383844808006,12.3701616257491));
#78259=CARTESIAN_POINT('Ctrl Pts',(86.3460148865128,54.3883912677371,12.4301420155186));
#78260=CARTESIAN_POINT('Ctrl Pts',(86.3591209808625,54.3929335792868,12.4900676792935));
#78261=CARTESIAN_POINT('Ctrl Pts',(86.3754814072012,54.3974758908366,12.5493527512415));
#78262=CARTESIAN_POINT('Ctrl Pts',(86.3950094588118,54.4020182023863,12.6076173985299));
#78263=CARTESIAN_POINT('Ctrl Pts',(86.4145271930971,54.4065581140803,12.6658512626488));
#78264=CARTESIAN_POINT('Ctrl Pts',(86.4372090708181,54.4110980257744,12.7230652790075));
#78265=CARTESIAN_POINT('Ctrl Pts',(86.4629183718369,54.4156379374684,12.7788941773812));
#78266=CARTESIAN_POINT('Ctrl Pts',(86.4886239629771,54.4201771940485,12.8347150195872));
#78267=CARTESIAN_POINT('Ctrl Pts',(86.5173558919771,54.4247164506286,12.8891506693967));
#78268=CARTESIAN_POINT('Ctrl Pts',(86.5489299526732,54.4292557072087,12.9418573013396));
#78269=CARTESIAN_POINT('Ctrl Pts',(86.5805334836223,54.4337992005906,12.9946131280248));
#78270=CARTESIAN_POINT('Ctrl Pts',(86.6149841758236,54.4383426939726,13.0456362678403));
#78271=CARTESIAN_POINT('Ctrl Pts',(86.6520533418262,54.4428861873546,13.0946101379231));
#78272=CARTESIAN_POINT('Ctrl Pts',(86.6891405886908,54.4474318968716,13.1436078955082));
#78273=CARTESIAN_POINT('Ctrl Pts',(86.7288485154797,54.4519776063886,13.1905539970893));
#78274=CARTESIAN_POINT('Ctrl Pts',(86.770908834505,54.4565233159056,13.2351658294961));
#78275=CARTESIAN_POINT('Ctrl Pts',(86.813045320444,54.4610772572352,13.2798584493449));
#78276=CARTESIAN_POINT('Ctrl Pts',(86.8575423259244,54.4656311985648,13.3222080033695));
#78277=CARTESIAN_POINT('Ctrl Pts',(86.904096329719,54.4701851398943,13.3619703315734));
#78278=CARTESIAN_POINT('Ctrl Pts',(86.9346638294139,54.4731752715448,13.3880783965339));
#78279=CARTESIAN_POINT('Ctrl Pts',(86.9661174748064,54.4761654031953,13.4130718722357));
#78280=CARTESIAN_POINT('Ctrl Pts',(86.998364778829,54.4791555348458,13.4368919521407));
#78281=CARTESIAN_POINT('Ctrl Pts',(87.0479438891033,54.4837527584379,13.4735144979362));
#78282=CARTESIAN_POINT('Ctrl Pts',(87.0996140482451,54.4883499820299,13.5075191659228));
#78283=CARTESIAN_POINT('Ctrl Pts',(87.1530676211808,54.492947205622,13.5386597940372));
#78284=CARTESIAN_POINT('Ctrl Pts',(87.2074364647569,54.4976231461931,13.5703336344529));
#78285=CARTESIAN_POINT('Ctrl Pts',(87.2636500006559,54.5022990867642,13.5990440400659));
#78286=CARTESIAN_POINT('Ctrl Pts',(87.321350487704,54.5069750273354,13.6245757555505));
#78287=CARTESIAN_POINT('Ctrl Pts',(87.3779235773261,54.5115596057078,13.6496086123289));
#78288=CARTESIAN_POINT('Ctrl Pts',(87.4359255464466,54.5161441840802,13.6715856614817));
#78289=CARTESIAN_POINT('Ctrl Pts',(87.4949934502638,54.5207287624526,13.6903497395048));
#78290=CARTESIAN_POINT('Ctrl Pts',(87.554025252807,54.5253105388106,13.7091023492503));
#78291=CARTESIAN_POINT('Ctrl Pts',(87.6141212141056,54.5298923151685,13.7246457278236));
#78292=CARTESIAN_POINT('Ctrl Pts',(87.6749004332037,54.5344740915265,13.7368716039239));
#78293=CARTESIAN_POINT('Ctrl Pts',(87.7356648290827,54.5390547504519,13.7490944983005));
#78294=CARTESIAN_POINT('Ctrl Pts',(87.7971116531336,54.5436354093774,13.7580013960368));
#78295=CARTESIAN_POINT('Ctrl Pts',(87.8588489460954,54.5482160683028,13.7635349458541));
#78296=CARTESIAN_POINT('Ctrl Pts',(87.9228165979135,54.5529622108883,13.7692684040451));
#78297=CARTESIAN_POINT('Ctrl Pts',(87.9870955344131,54.5577083534738,13.7713799967936));
#78298=CARTESIAN_POINT('Ctrl Pts',(88.0512455570579,54.5624544960594,13.7698647630423));
#78299=CARTESIAN_POINT('Ctrl Pts',(88.1132372883896,54.5670409573558,13.7684005084755));
#78300=CARTESIAN_POINT('Ctrl Pts',(88.1751081224645,54.5716274186521,13.7635497258958));
#78301=CARTESIAN_POINT('Ctrl Pts',(88.2364649154011,54.5762138799485,13.7553609464893));
#78302=CARTESIAN_POINT('Ctrl Pts',(88.3010259864812,54.5810398631786,13.7467445188043));
#78303=CARTESIAN_POINT('Ctrl Pts',(88.3650172194607,54.5858658464087,13.7344319998631));
#78304=CARTESIAN_POINT('Ctrl Pts',(88.4279946468341,54.5906918296387,13.718540559294));
#78305=CARTESIAN_POINT('Ctrl Pts',(88.4909720742074,54.5955178128688,13.7026491187249));
#78306=CARTESIAN_POINT('Ctrl Pts',(88.5529351009836,54.6003437960989,13.6831790245952));
#78307=CARTESIAN_POINT('Ctrl Pts',(88.6134632606434,54.605169779329,13.6603063868576));
#78308=CARTESIAN_POINT('Ctrl Pts',(88.6711222847858,54.609767002921,13.6385179502204));
#78309=CARTESIAN_POINT('Ctrl Pts',(88.7277161566771,54.6143642265131,13.6135528454747));
#78310=CARTESIAN_POINT('Ctrl Pts',(88.7828712094735,54.6189614501052,13.5855360053602));
#78311=CARTESIAN_POINT('Ctrl Pts',(88.8389706668758,54.6236373906763,13.5570394406963));
#78312=CARTESIAN_POINT('Ctrl Pts',(88.8935810387959,54.6283133312474,13.5253857475867));
#78313=CARTESIAN_POINT('Ctrl Pts',(88.9463274463073,54.6329892718186,13.4907587177428));
#78314=CARTESIAN_POINT('Ctrl Pts',(88.9980432530891,54.637573850191,13.4568082579993));
#78315=CARTESIAN_POINT('Ctrl Pts',(89.0479668336628,54.6421584285634,13.4199999000623));
#78316=CARTESIAN_POINT('Ctrl Pts',(89.0957692908299,54.6467430069358,13.3805533162532));
#78317=CARTESIAN_POINT('Ctrl Pts',(89.1435425319678,54.6513247832938,13.3411308415091));
#78318=CARTESIAN_POINT('Ctrl Pts',(89.1891968284483,54.6559065596517,13.2990736614473));
#78319=CARTESIAN_POINT('Ctrl Pts',(89.2324346190519,54.6604883360097,13.254643052805));
#78320=CARTESIAN_POINT('Ctrl Pts',(89.2756618645504,54.6650689949351,13.2102232801798));
#78321=CARTESIAN_POINT('Ctrl Pts',(89.3164734192652,54.6696496538606,13.1634315927237));
#78322=CARTESIAN_POINT('Ctrl Pts',(89.3546085029542,54.674230312786,13.1145661764473));
#78323=CARTESIAN_POINT('Ctrl Pts',(89.3941212777851,54.6789764553715,13.0639354185317));
#78324=CARTESIAN_POINT('Ctrl Pts',(89.4307600872057,54.6837225979571,13.011078648429));
#78325=CARTESIAN_POINT('Ctrl Pts',(89.4642820001852,54.6884687405426,12.9563629953776));
#78326=CARTESIAN_POINT('Ctrl Pts',(89.4966760873183,54.693055201839,12.9034882195979));
#78327=CARTESIAN_POINT('Ctrl Pts',(89.5261595060493,54.6976416631354,12.848878163558));
#78328=CARTESIAN_POINT('Ctrl Pts',(89.5525597877001,54.7022281244318,12.7928894390111));
#78329=CARTESIAN_POINT('Ctrl Pts',(89.58033878948,54.7070541076618,12.733976776661));
#78330=CARTESIAN_POINT('Ctrl Pts',(89.604703547265,54.7118800908919,12.6735380920378));
#78331=CARTESIAN_POINT('Ctrl Pts',(89.6255116903145,54.716706074122,12.6120099243034));
#78332=CARTESIAN_POINT('Ctrl Pts',(89.646319833364,54.721532057352,12.550481756569));
#78333=CARTESIAN_POINT('Ctrl Pts',(89.6635712641648,54.7263580405821,12.4878647509873));
#78334=CARTESIAN_POINT('Ctrl Pts',(89.6771858758965,54.7311840238122,12.4246076722034));
#78335=CARTESIAN_POINT('Ctrl Pts',(89.6901551323704,54.7357812474042,12.3643490842458));
#78336=CARTESIAN_POINT('Ctrl Pts',(89.69987786545,54.7403784709963,12.3032623323918));
#78337=CARTESIAN_POINT('Ctrl Pts',(89.7062563573408,54.7449756945884,12.2417291054314));
#78338=CARTESIAN_POINT('Ctrl Pts',(89.7127440663715,54.7496516351595,12.1791422621653));
#78339=CARTESIAN_POINT('Ctrl Pts',(89.7157717268321,54.7543275757306,12.1160940085744));
#78340=CARTESIAN_POINT('Ctrl Pts',(89.7152904121643,54.7590035163018,12.0529989767782));
#78341=CARTESIAN_POINT('Ctrl Pts',(89.7148185018005,54.7635880946742,11.9911367452594));
#78342=CARTESIAN_POINT('Ctrl Pts',(89.7109735093815,54.7681726730466,11.9292300804759));
#78343=CARTESIAN_POINT('Ctrl Pts',(89.7037615928417,54.772757251419,11.8676744459228));
#78344=CARTESIAN_POINT('Ctrl Pts',(89.6965540840997,54.777339027777,11.8061564331013));
#78345=CARTESIAN_POINT('Ctrl Pts',(89.68598379068,54.7819208041349,11.7449895296412));
#78346=CARTESIAN_POINT('Ctrl Pts',(89.6721088198636,54.7865025804929,11.6845654392017));
#78347=CARTESIAN_POINT('Ctrl Pts',(89.6582372329626,54.7910832394183,11.6241560853704));
#78348=CARTESIAN_POINT('Ctrl Pts',(89.6410626825035,54.7956638983438,11.5644896808385));
#78349=CARTESIAN_POINT('Ctrl Pts',(89.6206942339859,54.8002445572692,11.5059470483316));
#78350=CARTESIAN_POINT('Ctrl Pts',(89.5995899425547,54.8049906998547,11.4452894692081));
#78351=CARTESIAN_POINT('Ctrl Pts',(89.5750566958746,54.8097368424403,11.3858389830133));
#78352=CARTESIAN_POINT('Ctrl Pts',(89.5472711615009,54.8144829850258,11.3279988116943));
#78353=CARTESIAN_POINT('Ctrl Pts',(89.5204204557523,54.8190694463222,11.272104640301));
#78354=CARTESIAN_POINT('Ctrl Pts',(89.4905331613785,54.8236559076186,11.2177145691873));
#78355=CARTESIAN_POINT('Ctrl Pts',(89.4578153286656,54.8282423689149,11.1651669187146));
#78356=CARTESIAN_POINT('Ctrl Pts',(89.4233888499944,54.833068352145,11.1098750360249));
#78357=CARTESIAN_POINT('Ctrl Pts',(89.3858284459847,54.8378943353751,11.0566238194046));
#78358=CARTESIAN_POINT('Ctrl Pts',(89.3454236407146,54.8427203186052,11.0057696558286));
#78359=CARTESIAN_POINT('Ctrl Pts',(89.3050188354446,54.8475463018352,10.9549154922525));
#78360=CARTESIAN_POINT('Ctrl Pts',(89.2617701181232,54.8523722850653,10.906458813634));
#78361=CARTESIAN_POINT('Ctrl Pts',(89.2160110555889,54.8571982682954,10.8607103287971));
#78362=CARTESIAN_POINT('Ctrl Pts',(89.1724210487852,54.8617954918875,10.8171303982902));
#78363=CARTESIAN_POINT('Ctrl Pts',(89.1263743736857,54.8663927154796,10.7758287457457));
#78364=CARTESIAN_POINT('Ctrl Pts',(89.078138693113,54.8709899390716,10.7370944934793));
#78365=CARTESIAN_POINT('Ctrl Pts',(89.0290770864174,54.8756658796428,10.6976970054004));
#78366=CARTESIAN_POINT('Ctrl Pts',(88.9777511130749,54.8803418202139,10.6609561089882));
#78367=CARTESIAN_POINT('Ctrl Pts',(88.9244825766025,54.885017760785,10.6271378044289));
#78368=CARTESIAN_POINT('Ctrl Pts',(88.8722548426254,54.8896023391574,10.5939802684603));
#78369=CARTESIAN_POINT('Ctrl Pts',(88.8181602237876,54.8941869175299,10.5636324295897));
#78370=CARTESIAN_POINT('Ctrl Pts',(88.7625342973995,54.8987714959023,10.5363036133166));
#78371=CARTESIAN_POINT('Ctrl Pts',(88.7069423686088,54.9033532722602,10.5089914999401));
#78372=CARTESIAN_POINT('Ctrl Pts',(88.6498214439763,54.9079350486182,10.4846949744478));
#78373=CARTESIAN_POINT('Ctrl Pts',(88.5915321193561,54.9125168249761,10.4635776792631));
#78374=CARTESIAN_POINT('Ctrl Pts',(88.5332570107039,54.9170974839016,10.4424655342974));
#78375=CARTESIAN_POINT('Ctrl Pts',(88.4738145461388,54.9216781428271,10.4245312537248));
#78376=CARTESIAN_POINT('Ctrl Pts',(88.413583819887,54.9262588017525,10.4098897670852));
#78377=CARTESIAN_POINT('Ctrl Pts',(88.3511771619209,54.931004944338,10.3947193332269));
#78378=CARTESIAN_POINT('Ctrl Pts',(88.287924747194,54.9357510869235,10.3830843629789));
#78379=CARTESIAN_POINT('Ctrl Pts',(88.2242611552639,54.9404972295091,10.3750551412729));
#78380=CARTESIAN_POINT('Ctrl Pts',(88.16273948896,54.9450836908055,10.3672960582005));
#78381=CARTESIAN_POINT('Ctrl Pts',(88.1008344072298,54.9496701521019,10.3629038996506));
#78382=CARTESIAN_POINT('Ctrl Pts',(88.038941901592,54.9542566133983,10.3618890629612));
#78383=CARTESIAN_POINT('Ctrl Pts',(87.9738171409165,54.9590825966283,10.3608212277549));
#78384=CARTESIAN_POINT('Ctrl Pts',(87.9087069497816,54.9639085798584,10.3634931243255));
#78385=CARTESIAN_POINT('Ctrl Pts',(87.8440677739317,54.9687345630885,10.3698548212196));
#78386=CARTESIAN_POINT('Ctrl Pts',(87.7794285980819,54.9735605463185,10.3762165181138));
#78387=CARTESIAN_POINT('Ctrl Pts',(87.7152610657229,54.9783865295486,10.386267838606));
#78388=CARTESIAN_POINT('Ctrl Pts',(87.6520071361564,54.9832125127787,10.399897074215));
#78389=CARTESIAN_POINT('Ctrl Pts',(87.591751548138,54.9878097363708,10.4128802613702));
#78390=CARTESIAN_POINT('Ctrl Pts',(87.5320774958243,54.9924069599628,10.4291630827193));
#78391=CARTESIAN_POINT('Ctrl Pts',(87.4733730569773,54.9970041835549,10.4486774886449));
#78392=CARTESIAN_POINT('Ctrl Pts',(87.4136634383757,55.0016801241261,10.4685260343075));
#78393=CARTESIAN_POINT('Ctrl Pts',(87.3549574890073,55.0063560646972,10.491717854363));
#78394=CARTESIAN_POINT('Ctrl Pts',(87.2976532270897,55.0110320052683,10.5181268730356));
#78395=CARTESIAN_POINT('Ctrl Pts',(87.2414686208403,55.0156165836407,10.5440198915635));
#78396=CARTESIAN_POINT('Ctrl Pts',(87.1866319045675,55.0202011620131,10.573005295817));
#78397=CARTESIAN_POINT('Ctrl Pts',(87.1335009537733,55.0247857403855,10.6049146980853));
#78398=CARTESIAN_POINT('Ctrl Pts',(87.0804024756907,55.0293675167435,10.6368045978827));
#78399=CARTESIAN_POINT('Ctrl Pts',(87.0290081313791,55.0339492931015,10.6716146905955));
#78400=CARTESIAN_POINT('Ctrl Pts',(86.9796509870481,55.0385310694594,10.7091307914603));
#78401=CARTESIAN_POINT('Ctrl Pts',(86.9303058802488,55.0431117283849,10.7466377426618));
#78402=CARTESIAN_POINT('Ctrl Pts',(86.8829973922011,55.0476923873103,10.7868490839957));
#78403=CARTESIAN_POINT('Ctrl Pts',(86.8380276978842,55.0522730462358,10.829508668017));
#78404=CARTESIAN_POINT('Ctrl Pts',(86.7914334011402,55.0570191888213,10.8737093980209));
#78405=CARTESIAN_POINT('Ctrl Pts',(86.7473505848034,55.0617653314068,10.920538297274));
#78406=CARTESIAN_POINT('Ctrl Pts',(86.7060740121473,55.0665114739923,10.9696683887497));
#78407=CARTESIAN_POINT('Ctrl Pts',(86.6661861664865,55.0710979352887,11.0171455260211));
#78408=CARTESIAN_POINT('Ctrl Pts',(86.628918981345,55.0756843965851,11.0667709944056));
#78409=CARTESIAN_POINT('Ctrl Pts',(86.5944959770564,55.0802708578815,11.1182177525482));
#78410=CARTESIAN_POINT('Ctrl Pts',(86.5582752764576,55.0850968411115,11.1723512502478));
#78411=CARTESIAN_POINT('Ctrl Pts',(86.5252043061989,55.0899228243416,11.2285009336578));
#78412=CARTESIAN_POINT('Ctrl Pts',(86.4954886934164,55.0947488075717,11.2862562502865));
#78413=CARTESIAN_POINT('Ctrl Pts',(86.4657730806339,55.0995747908017,11.3440115669152));
#78414=CARTESIAN_POINT('Ctrl Pts',(86.4394130175949,55.1044007740318,11.4033718931378));
#78415=CARTESIAN_POINT('Ctrl Pts',(86.416554373818,55.1092267572618,11.4639053390463));
#78416=CARTESIAN_POINT('Ctrl Pts',(86.3916467123487,55.1144853350552,11.5298649205931));
#78417=CARTESIAN_POINT('Ctrl Pts',(86.3708096801981,55.1197439128485,11.5974413574462));
#78418=CARTESIAN_POINT('Ctrl Pts',(86.3542262509689,55.1250024906418,11.666155555095));
#78419=CARTESIAN_POINT('Ctrl Pts',(86.3377777976361,55.1302182678031,11.7343104739421));
#78420=CARTESIAN_POINT('Ctrl Pts',(86.3255140956074,55.1354340449644,11.8035845018164));
#78421=CARTESIAN_POINT('Ctrl Pts',(86.317567286777,55.1406498221257,11.8734890097));
#78422=CARTESIAN_POINT('Ctrl Pts',(86.3103605653991,55.1453798532078,11.9368833006832));
#78423=CARTESIAN_POINT('Ctrl Pts',(86.3067036515886,55.1501098842899,12.0007957452571));
#78424=CARTESIAN_POINT('Ctrl Pts',(86.3066603887547,55.154839915372,12.0648488527018));
#78425=CARTESIAN_POINT('',(86.3066604846332,55.9485899154847,12.0672852856579));
#78426=CARTESIAN_POINT('Ctrl Pts',(86.3066603887541,55.1548399154298,12.0648488534838));
#78427=CARTESIAN_POINT('Ctrl Pts',(86.3066182940265,55.1594422377324,12.1271725549211));
#78428=CARTESIAN_POINT('Ctrl Pts',(86.3099990779096,55.164044560035,12.1895184871938));
#78429=CARTESIAN_POINT('Ctrl Pts',(86.3167835349057,55.1686468823377,12.2514869402501));
#78430=CARTESIAN_POINT('Ctrl Pts',(86.3235683082009,55.1732494192058,12.313458282347));
#78431=CARTESIAN_POINT('Ctrl Pts',(86.3337570130611,55.177851956074,12.3750516114809));
#78432=CARTESIAN_POINT('Ctrl Pts',(86.3472786724264,55.1824544929422,12.435873194185));
#78433=CARTESIAN_POINT('Ctrl Pts',(86.3608164302688,55.1870625094511,12.4967671892192));
#78434=CARTESIAN_POINT('Ctrl Pts',(86.3776949568103,55.1916705259599,12.5568871118524));
#78435=CARTESIAN_POINT('Ctrl Pts',(86.3977925109203,55.1962785424688,12.6158512824183));
#78436=CARTESIAN_POINT('Ctrl Pts',(86.4179021109743,55.2008893209012,12.6748507945534));
#78437=CARTESIAN_POINT('Ctrl Pts',(86.4412343924767,55.2055000993337,12.7326927090471));
#78438=CARTESIAN_POINT('Ctrl Pts',(86.4676193647064,55.2101108777661,12.7890152489407));
#78439=CARTESIAN_POINT('Ctrl Pts',(86.4940582244476,55.2147310730505,12.8454528195224));
#78440=CARTESIAN_POINT('Ctrl Pts',(86.5235619915821,55.2193512683348,12.9003643732525));
#78441=CARTESIAN_POINT('Ctrl Pts',(86.5559149500569,55.2239714636191,12.9534132819787));
#78442=CARTESIAN_POINT('Ctrl Pts',(86.5822199636318,55.2277279763278,12.9965454198097));
#78443=CARTESIAN_POINT('Ctrl Pts',(86.6104075793017,55.2314844890364,13.0384466472158));
#78444=CARTESIAN_POINT('Ctrl Pts',(86.6403421930249,55.2352410017451,13.078952127091));
#78445=CARTESIAN_POINT('Ctrl Pts',(86.6769761999087,55.2398382253372,13.1285227693683));
#78446=CARTESIAN_POINT('Ctrl Pts',(86.7163780016629,55.2444354489293,13.1762052693987));
#78447=CARTESIAN_POINT('Ctrl Pts',(86.7583258449082,55.2490326725214,13.2216739578121));
#78448=CARTESIAN_POINT('Ctrl Pts',(86.8009919493891,55.2537086130925,13.2679211939122));
#78449=CARTESIAN_POINT('Ctrl Pts',(86.8462918675474,55.2583845536636,13.3118776089568));
#78450=CARTESIAN_POINT('Ctrl Pts',(86.8939468716422,55.2630604942347,13.3532323582112));
#78451=CARTESIAN_POINT('Ctrl Pts',(86.9406707548454,55.2676450726072,13.3937790859005));
#78452=CARTESIAN_POINT('Ctrl Pts',(86.9896581177633,55.2722296509796,13.4318245506194));
#78453=CARTESIAN_POINT('Ctrl Pts',(87.040608194221,55.276814229352,13.4671119080491));
#78454=CARTESIAN_POINT('Ctrl Pts',(87.0915271308794,55.28139600571,13.5023776984606));
#78455=CARTESIAN_POINT('Ctrl Pts',(87.1444059848795,55.2859777820679,13.5348884348643));
#78456=CARTESIAN_POINT('Ctrl Pts',(87.1989124640647,55.2905595584259,13.5644287335668));
#78457=CARTESIAN_POINT('Ctrl Pts',(87.253405649866,55.2951402173513,13.593961827795));
#78458=CARTESIAN_POINT('Ctrl Pts',(87.3095252254899,55.2997208762768,13.62052568002));
#78459=CARTESIAN_POINT('Ctrl Pts',(87.3669133706643,55.3043015352022,13.643950331763));
#78460=CARTESIAN_POINT('Ctrl Pts',(87.4263747547465,55.3090476777877,13.6682212366693));
#78461=CARTESIAN_POINT('Ctrl Pts',(87.4871976074236,55.3137938203733,13.6891215020663));
#78462=CARTESIAN_POINT('Ctrl Pts',(87.5489626077904,55.3185399629588,13.70651707818));
#78463=CARTESIAN_POINT('Ctrl Pts',(87.608649559573,55.3231264242552,13.7233273899514));
#78464=CARTESIAN_POINT('Ctrl Pts',(87.6692157346942,55.3277128855516,13.7368650644912));
#78465=CARTESIAN_POINT('Ctrl Pts',(87.7302710777268,55.332299346848,13.7470610065668));
#78466=CARTESIAN_POINT('Ctrl Pts',(87.7945149560764,55.337125330078,13.7577894183622));
#78467=CARTESIAN_POINT('Ctrl Pts',(87.8592998566214,55.3419513133081,13.7648174111248));
#78468=CARTESIAN_POINT('Ctrl Pts',(87.924166980079,55.3467772965382,13.7681265705732));
#78469=CARTESIAN_POINT('Ctrl Pts',(87.9890341035366,55.3516032797682,13.7714357300217));
#78470=CARTESIAN_POINT('Ctrl Pts',(88.0539828024207,55.3564292629983,13.7710261376193));
#78471=CARTESIAN_POINT('Ctrl Pts',(88.1185594280151,55.3612552462284,13.7669426225023));
#78472=CARTESIAN_POINT('Ctrl Pts',(88.1800750140681,55.3658524698204,13.7630526727989));
#78473=CARTESIAN_POINT('Ctrl Pts',(88.2415055803598,55.3704496934125,13.755813314009));
#78474=CARTESIAN_POINT('Ctrl Pts',(88.3024572463992,55.3750469170046,13.7452342031776));
#78475=CARTESIAN_POINT('Ctrl Pts',(88.3644525708386,55.3797228575757,13.7344739491781));
#78476=CARTESIAN_POINT('Ctrl Pts',(88.4259519052912,55.3843987981468,13.7202584340412));
#78477=CARTESIAN_POINT('Ctrl Pts',(88.4865429209327,55.389074738718,13.7026532210431));
#78478=CARTESIAN_POINT('Ctrl Pts',(88.5459500617308,55.3936593170904,13.6853919925213));
#78479=CARTESIAN_POINT('Ctrl Pts',(88.6044835471508,55.3982438954628,13.6648724848301));
#78480=CARTESIAN_POINT('Ctrl Pts',(88.661764461642,55.4028284738352,13.6412080659595));
#78481=CARTESIAN_POINT('Ctrl Pts',(88.7190103670358,55.4074102501932,13.6175581103696));
#78482=CARTESIAN_POINT('Ctrl Pts',(88.7750047499725,55.4119920265511,13.5907672488416));
#78483=CARTESIAN_POINT('Ctrl Pts',(88.8293864271967,55.4165738029091,13.5609978232025));
#78484=CARTESIAN_POINT('Ctrl Pts',(88.8837548414746,55.4211544618345,13.5312356579186));
#78485=CARTESIAN_POINT('Ctrl Pts',(88.936510884512,55.42573512076,13.498496614923));
#78486=CARTESIAN_POINT('Ctrl Pts',(88.9873176893197,55.4303157796854,13.4629891213326));
#78487=CARTESIAN_POINT('Ctrl Pts',(89.039959971545,55.4350619222709,13.4261988625124));
#78488=CARTESIAN_POINT('Ctrl Pts',(89.0905089670408,55.4398080648565,13.3864365744015));
#78489=CARTESIAN_POINT('Ctrl Pts',(89.1386246186138,55.444554207442,13.3439818289381));
#78490=CARTESIAN_POINT('Ctrl Pts',(89.1851214462405,55.4491406687384,13.3029554494294));
#78491=CARTESIAN_POINT('Ctrl Pts',(89.2293457516953,55.4537271300347,13.2594153413936));
#78492=CARTESIAN_POINT('Ctrl Pts',(89.2710279210297,55.4583135913311,13.2136517214842));
#78493=CARTESIAN_POINT('Ctrl Pts',(89.3148868870606,55.4631395745612,13.165498156468));
#78494=CARTESIAN_POINT('Ctrl Pts',(89.3559305024903,55.4679655577913,13.1148829645452));
#78495=CARTESIAN_POINT('Ctrl Pts',(89.3938944449276,55.4727915410214,13.0621816048233));
#78496=CARTESIAN_POINT('Ctrl Pts',(89.431858387365,55.4776175242514,13.0094802451013));
#78497=CARTESIAN_POINT('Ctrl Pts',(89.4667423740536,55.4824435074815,12.9546933057325));
#78498=CARTESIAN_POINT('Ctrl Pts',(89.4983380083971,55.4872694907116,12.8982262218755));
#78499=CARTESIAN_POINT('Ctrl Pts',(89.5284359570816,55.4918667143036,12.8444357717834));
#78500=CARTESIAN_POINT('Ctrl Pts',(89.555673881669,55.4964639378957,12.788900033247));
#78501=CARTESIAN_POINT('Ctrl Pts',(89.5798462549563,55.5010611614878,12.7319551515752));
#78502=CARTESIAN_POINT('Ctrl Pts',(89.6044325250584,55.5057371020589,12.674035218556));
#78503=CARTESIAN_POINT('Ctrl Pts',(89.6258469327725,55.51041304263,12.6146578478582));
#78504=CARTESIAN_POINT('Ctrl Pts',(89.6439209125508,55.5150889832012,12.5542050070967));
#78505=CARTESIAN_POINT('Ctrl Pts',(89.6616417487194,55.5196735615736,12.4949333414091));
#78506=CARTESIAN_POINT('Ctrl Pts',(89.6761513659806,55.524258139946,12.4346283655096));
#78507=CARTESIAN_POINT('Ctrl Pts',(89.6873394838569,55.5288427183184,12.3736699050319));
#78508=CARTESIAN_POINT('Ctrl Pts',(89.6985207637504,55.5334244946764,12.3127487013035));
#78509=CARTESIAN_POINT('Ctrl Pts',(89.7063844778368,55.5380062710343,12.2511753045915));
#78510=CARTESIAN_POINT('Ctrl Pts',(89.7108711075708,55.5425880473923,12.1893412066015));
#78511=CARTESIAN_POINT('Ctrl Pts',(89.7153566430773,55.5471687063177,12.1275221891014));
#78512=CARTESIAN_POINT('Ctrl Pts',(89.7164666924284,55.5517493652432,12.065443104027));
#78513=CARTESIAN_POINT('Ctrl Pts',(89.7141936434196,55.5563300241686,12.0035000110784));
#78514=CARTESIAN_POINT('Ctrl Pts',(89.7118384768648,55.5610761667541,11.9393191244186));
#78515=CARTESIAN_POINT('Ctrl Pts',(89.7058510494495,55.5658223093397,11.8752848272459));
#78516=CARTESIAN_POINT('Ctrl Pts',(89.6962817888767,55.5705684519252,11.8118344482814));
#78517=CARTESIAN_POINT('Ctrl Pts',(89.6870344806762,55.5751549132216,11.7505188215132));
#78518=CARTESIAN_POINT('Ctrl Pts',(89.674442722707,55.5797413745179,11.689748945489));
#78519=CARTESIAN_POINT('Ctrl Pts',(89.6586040938518,55.5843278358143,11.6299087417493));
#78520=CARTESIAN_POINT('Ctrl Pts',(89.6419383133507,55.5891538190444,11.5669434617502));
#78521=CARTESIAN_POINT('Ctrl Pts',(89.6216774252868,55.5939798022745,11.5050082340056));
#78522=CARTESIAN_POINT('Ctrl Pts',(89.597993492667,55.5988057855046,11.4445287699076));
#78523=CARTESIAN_POINT('Ctrl Pts',(89.5743095600472,55.6036317687346,11.3840493058095));
#78524=CARTESIAN_POINT('Ctrl Pts',(89.547202923624,55.6084577519647,11.3250261619207));
#78525=CARTESIAN_POINT('Ctrl Pts',(89.5169011640017,55.6132837351948,11.2678543241623));
#78526=CARTESIAN_POINT('Ctrl Pts',(89.488035758223,55.6178809587869,11.2133925266766));
#78527=CARTESIAN_POINT('Ctrl Pts',(89.4561528251404,55.6224781823789,11.1603868536909));
#78528=CARTESIAN_POINT('Ctrl Pts',(89.4214232898435,55.627075405971,11.1091922977594));
#78529=CARTESIAN_POINT('Ctrl Pts',(89.3860990903874,55.6317513465421,11.0571211517064));
#78530=CARTESIAN_POINT('Ctrl Pts',(89.3478300524464,55.6364272871133,11.0069242420028));
#78531=CARTESIAN_POINT('Ctrl Pts',(89.3068456453556,55.6411032276844,10.9589503628957));
#78532=CARTESIAN_POINT('Ctrl Pts',(89.266662023794,55.6456878060568,10.9119138351105));
#78533=CARTESIAN_POINT('Ctrl Pts',(89.2238685352838,55.6502723844292,10.867014654133));
#78534=CARTESIAN_POINT('Ctrl Pts',(89.1787244633868,55.6548569628016,10.8245514858811));
#78535=CARTESIAN_POINT('Ctrl Pts',(89.1336079827603,55.6594387391596,10.7821142703782));
#78536=CARTESIAN_POINT('Ctrl Pts',(89.0861441374107,55.6640205155175,10.7421104634781));
#78537=CARTESIAN_POINT('Ctrl Pts',(89.0366295450226,55.6686022918755,10.7048024125878));
#78538=CARTESIAN_POINT('Ctrl Pts',(88.9871270285655,55.6731829508009,10.6675034606202));
#78539=CARTESIAN_POINT('Ctrl Pts',(88.9355751643183,55.6777636097264,10.6328992657033));
#78540=CARTESIAN_POINT('Ctrl Pts',(88.8823025615691,55.6823442686518,10.6012110453027));
#78541=CARTESIAN_POINT('Ctrl Pts',(88.8271054004916,55.6870904112373,10.5683780370499));
#78542=CARTESIAN_POINT('Ctrl Pts',(88.7700612585478,55.6918365538228,10.538676078001));
#78543=CARTESIAN_POINT('Ctrl Pts',(88.7115648967786,55.6965826964084,10.5123000093321));
#78544=CARTESIAN_POINT('Ctrl Pts',(88.6550366120927,55.7011691577048,10.48681134861));
#78545=CARTESIAN_POINT('Ctrl Pts',(88.5971527987433,55.7057556190011,10.4644284454721));
#78546=CARTESIAN_POINT('Ctrl Pts',(88.5382889240096,55.7103420802975,10.4452775604019));
#78547=CARTESIAN_POINT('Ctrl Pts',(88.4763509605202,55.7151680635276,10.4251265454436));
#78548=CARTESIAN_POINT('Ctrl Pts',(88.4133283838417,55.7199940467577,10.4085545555291));
#78549=CARTESIAN_POINT('Ctrl Pts',(88.3496721698896,55.7248200299878,10.3956479422163));
#78550=CARTESIAN_POINT('Ctrl Pts',(88.2860159559375,55.7296460132178,10.3827413289034));
#78551=CARTESIAN_POINT('Ctrl Pts',(88.2217267571155,55.7344719964479,10.3735001077978));
#78552=CARTESIAN_POINT('Ctrl Pts',(88.1572598488965,55.739297979678,10.3679473234906));
#78553=CARTESIAN_POINT('Ctrl Pts',(88.0958487794327,55.74389520327,10.3626577504022));
#78554=CARTESIAN_POINT('Ctrl Pts',(88.0340243279118,55.7484924268621,10.3606930660133));
#78555=CARTESIAN_POINT('Ctrl Pts',(87.9721774406511,55.7530896504542,10.3621022200597));
#78556=CARTESIAN_POINT('Ctrl Pts',(87.9092715663668,55.7577655910253,10.3635355026583));
#78557=CARTESIAN_POINT('Ctrl Pts',(87.8463430009672,55.7624415315965,10.3684593898906));
#78558=CARTESIAN_POINT('Ctrl Pts',(87.7838092377672,55.7671174721676,10.3768702852782));
#78559=CARTESIAN_POINT('Ctrl Pts',(87.7224973083379,55.77170205054,10.385116841987));
#78560=CARTESIAN_POINT('Ctrl Pts',(87.6615654206068,55.7762866289124,10.3967152974373));
#78561=CARTESIAN_POINT('Ctrl Pts',(87.6014051252175,55.7808712072848,10.4116098180441));
#78562=CARTESIAN_POINT('Ctrl Pts',(87.5412815987531,55.7854529836428,10.4264952353793));
#78563=CARTESIAN_POINT('Ctrl Pts',(87.4819292226512,55.7900347600007,10.4446726013306));
#78564=CARTESIAN_POINT('Ctrl Pts',(87.4237292855877,55.7946165363587,10.4660350180102));
#78565=CARTESIAN_POINT('Ctrl Pts',(87.3655435426919,55.7991971952841,10.4873922246889));
#78566=CARTESIAN_POINT('Ctrl Pts',(87.3085101585382,55.8037778542096,10.5119327647239));
#78567=CARTESIAN_POINT('Ctrl Pts',(87.2529932198747,55.808358513135,10.5395005545746));
#78568=CARTESIAN_POINT('Ctrl Pts',(87.1954706426435,55.8131046557205,10.5680642751067));
#78569=CARTESIAN_POINT('Ctrl Pts',(87.1395767259984,55.817850798306,10.5998779605821));
#78570=CARTESIAN_POINT('Ctrl Pts',(87.0856892780369,55.8225969408916,10.6347156455057));
#78571=CARTESIAN_POINT('Ctrl Pts',(87.0336148428542,55.827183402188,10.6683812361785));
#78572=CARTESIAN_POINT('Ctrl Pts',(86.9834143832994,55.8317698634844,10.7048701942512));
#78573=CARTESIAN_POINT('Ctrl Pts',(86.9353976264655,55.8363563247808,10.7439355652439));
#78574=CARTESIAN_POINT('Ctrl Pts',(86.8848732574003,55.8411823080108,10.7850410740672));
#78575=CARTESIAN_POINT('Ctrl Pts',(86.8367674101936,55.8460082912409,10.8289990481498));
#78576=CARTESIAN_POINT('Ctrl Pts',(86.7913972393957,55.850834274471,10.8754774500554));
#78577=CARTESIAN_POINT('Ctrl Pts',(86.7460270685979,55.8556602577011,10.9219558519611));
#78578=CARTESIAN_POINT('Ctrl Pts',(86.7033929411827,55.8604862409311,10.9709541420561));
#78579=CARTESIAN_POINT('Ctrl Pts',(86.6637611582523,55.8653122241612,11.022102333135));
#78580=CARTESIAN_POINT('Ctrl Pts',(86.6259913092781,55.8699114787058,11.0708475398733));
#78581=CARTESIAN_POINT('Ctrl Pts',(86.5907903728854,55.8745107332503,11.1217484975243));
#78582=CARTESIAN_POINT('Ctrl Pts',(86.5584127681868,55.8791099877949,11.1745039710839));
#78583=CARTESIAN_POINT('Ctrl Pts',(86.5260846539442,55.883702212196,11.2271788058047));
#78584=CARTESIAN_POINT('Ctrl Pts',(86.4965715781281,55.8882944365972,11.281702107454));
#78585=CARTESIAN_POINT('Ctrl Pts',(86.4700867789411,55.8928866609983,11.3377409246938));
#78586=CARTESIAN_POINT('Ctrl Pts',(86.4433152665828,55.8975285988676,11.3943863943342));
#78587=CARTESIAN_POINT('Ctrl Pts',(86.4196383236701,55.9021705367369,11.4525799769534));
#78588=CARTESIAN_POINT('Ctrl Pts',(86.3992298158745,55.9068124746062,11.5119497232524));
#78589=CARTESIAN_POINT('Ctrl Pts',(86.3790787614473,55.9113958544196,11.5705705200782));
#78590=CARTESIAN_POINT('Ctrl Pts',(86.3621143073747,55.915979234233,11.6303374781457));
#78591=CARTESIAN_POINT('Ctrl Pts',(86.3484555539935,55.9205626140464,11.6908722875434));
#78592=CARTESIAN_POINT('Ctrl Pts',(86.334535040707,55.9252338309437,11.752567201786));
#78593=CARTESIAN_POINT('Ctrl Pts',(86.3240484533583,55.9299050478409,11.8150591982026));
#78594=CARTESIAN_POINT('Ctrl Pts',(86.3170678817167,55.9345762647382,11.8779340162383));
#78595=CARTESIAN_POINT('Ctrl Pts',(86.3100873100751,55.9392474816354,11.9408088342741));
#78596=CARTESIAN_POINT('Ctrl Pts',(86.3066128093318,55.9439186985327,12.0040659176332));
#78597=CARTESIAN_POINT('Ctrl Pts',(86.3066604846326,55.9485899154299,12.067285284916));
#78598=CARTESIAN_POINT('',(86.3066600510811,56.7423399153589,12.0664172756536));
#78599=CARTESIAN_POINT('Ctrl Pts',(86.3066604846332,55.9485899154847,12.0672852856579));
#78600=CARTESIAN_POINT('Ctrl Pts',(86.3067146504435,55.9538970682025,12.1391112882315));
#78601=CARTESIAN_POINT('Ctrl Pts',(86.3113132460109,55.9592042209202,12.2107507526871));
#78602=CARTESIAN_POINT('Ctrl Pts',(86.3203621123175,55.964511373638,12.2816811728741));
#78603=CARTESIAN_POINT('Ctrl Pts',(86.3295034461463,55.9698727584823,12.3533364087442));
#78604=CARTESIAN_POINT('Ctrl Pts',(86.3431863562652,55.9752341433265,12.4242678780687));
#78605=CARTESIAN_POINT('Ctrl Pts',(86.3612643699134,55.9805955281708,12.4939569913238));
#78606=CARTESIAN_POINT('Ctrl Pts',(86.3733255626821,55.9841725083287,12.5404518023802));
#78607=CARTESIAN_POINT('Ctrl Pts',(86.3873420993332,55.9877494884866,12.586394033035));
#78608=CARTESIAN_POINT('Ctrl Pts',(86.4032587884797,55.9913264686445,12.6316350699695));
#78609=CARTESIAN_POINT('Ctrl Pts',(86.4237153120338,55.9959236922366,12.6897799724135));
#78610=CARTESIAN_POINT('Ctrl Pts',(86.4473721617171,56.0005209158287,12.7469330672877));
#78611=CARTESIAN_POINT('Ctrl Pts',(86.4741130321229,56.0051181394207,12.8027179131592));
#78612=CARTESIAN_POINT('Ctrl Pts',(86.5013117790042,56.0097940799919,12.8594579474081));
#78613=CARTESIAN_POINT('Ctrl Pts',(86.5317010679247,56.014470020563,12.9147819035902));
#78614=CARTESIAN_POINT('Ctrl Pts',(86.5651057779538,56.0191459611341,12.968310774763));
#78615=CARTESIAN_POINT('Ctrl Pts',(86.597857800527,56.0237305395065,13.0207937568169));
#78616=CARTESIAN_POINT('Ctrl Pts',(86.6335081862367,56.0283151178789,13.0715507180151));
#78617=CARTESIAN_POINT('Ctrl Pts',(86.6718448854607,56.0328996962513,13.1202477957308));
#78618=CARTESIAN_POINT('Ctrl Pts',(86.7101581539617,56.0374814726093,13.1689151106407));
#78619=CARTESIAN_POINT('Ctrl Pts',(86.751154166243,56.0420632489673,13.2155246392687));
#78620=CARTESIAN_POINT('Ctrl Pts',(86.7945785585489,56.0466450253252,13.2597728897818));
#78621=CARTESIAN_POINT('Ctrl Pts',(86.8379923602402,56.0512256842507,13.3040103487527));
#78622=CARTESIAN_POINT('Ctrl Pts',(86.88383300986,56.0558063431762,13.3458873096701));
#78623=CARTESIAN_POINT('Ctrl Pts',(86.9318083981857,56.0603870021016,13.3851362030411));
#78624=CARTESIAN_POINT('Ctrl Pts',(86.9815169744614,56.0651331446871,13.4258030257173));
#78625=CARTESIAN_POINT('Ctrl Pts',(87.0335170748689,56.0698792872726,13.4636478412017));
#78626=CARTESIAN_POINT('Ctrl Pts',(87.0874472546661,56.0746254298581,13.4984193388063));
#78627=CARTESIAN_POINT('Ctrl Pts',(87.1395629839962,56.0792118911545,13.5320209689951));
#78628=CARTESIAN_POINT('Ctrl Pts',(87.193480479509,56.0837983524509,13.5627526119449));
#78629=CARTESIAN_POINT('Ctrl Pts',(87.2488471905413,56.0883848137473,13.5904336425815));
#78630=CARTESIAN_POINT('Ctrl Pts',(87.3071053555355,56.0932107969774,13.6195602787853));
#78631=CARTESIAN_POINT('Ctrl Pts',(87.3669676662476,56.0980367802074,13.6453086724651));
#78632=CARTESIAN_POINT('Ctrl Pts',(87.4280009735009,56.1028627634375,13.6675264502034));
#78633=CARTESIAN_POINT('Ctrl Pts',(87.4890342807541,56.1076887466675,13.6897442279417));
#78634=CARTESIAN_POINT('Ctrl Pts',(87.5512379416981,56.1125147298976,13.7084312774101));
#78635=CARTESIAN_POINT('Ctrl Pts',(87.6141651528457,56.1173407131277,13.7234971914558));
#78636=CARTESIAN_POINT('Ctrl Pts',(87.6741095094423,56.1219379367197,13.7378489560986));
#78637=CARTESIAN_POINT('Ctrl Pts',(87.7349564804357,56.1265351603118,13.7489741038072));
#78638=CARTESIAN_POINT('Ctrl Pts',(87.7963267255002,56.1311323839039,13.7567661638487));
#78639=CARTESIAN_POINT('Ctrl Pts',(87.8587477961767,56.135808324475,13.7646916451638));
#78640=CARTESIAN_POINT('Ctrl Pts',(87.9217097357451,56.1404842650461,13.7691686055733));
#78641=CARTESIAN_POINT('Ctrl Pts',(87.9847991470731,56.1451602056173,13.7701385949816));
#78642=CARTESIAN_POINT('Ctrl Pts',(88.046655867941,56.1497447839897,13.7710896319752));
#78643=CARTESIAN_POINT('Ctrl Pts',(88.1086345907267,56.1543293623621,13.7686695011596));
#78644=CARTESIAN_POINT('Ctrl Pts',(88.1703398149164,56.1589139407345,13.762875263236));
#78645=CARTESIAN_POINT('Ctrl Pts',(88.2320073259479,56.1634957170924,13.7570845666498));
#78646=CARTESIAN_POINT('Ctrl Pts',(88.2934011640666,56.1680774934504,13.7479238994837));
#78647=CARTESIAN_POINT('Ctrl Pts',(88.3541283927722,56.1726592698084,13.7354423445191));
#78648=CARTESIAN_POINT('Ctrl Pts',(88.4148408109383,56.1772399287338,13.7229638336349));
#78649=CARTESIAN_POINT('Ctrl Pts',(88.4748864440305,56.1818205876593,13.707166145203));
#78650=CARTESIAN_POINT('Ctrl Pts',(88.5338820615718,56.1864012465847,13.6881495570034));
#78651=CARTESIAN_POINT('Ctrl Pts',(88.5950089905418,56.1911473891702,13.6684459640151));
#78652=CARTESIAN_POINT('Ctrl Pts',(88.6550080113801,56.1958935317557,13.6452865598798));
#78653=CARTESIAN_POINT('Ctrl Pts',(88.7134719454762,56.2006396743412,13.618838691371));
#78654=CARTESIAN_POINT('Ctrl Pts',(88.7699688934998,56.2052261356376,13.5932806464742));
#78655=CARTESIAN_POINT('Ctrl Pts',(88.8250319802325,56.209812596934,13.5646522221337));
#78656=CARTESIAN_POINT('Ctrl Pts',(88.8783182356818,56.2143990582304,13.5331516328089));
#78657=CARTESIAN_POINT('Ctrl Pts',(88.9343872960256,56.2192250414605,13.5000059664672));
#78658=CARTESIAN_POINT('Ctrl Pts',(88.9884883099577,56.2240510246906,13.4636802687804));
#78659=CARTESIAN_POINT('Ctrl Pts',(89.0402583257664,56.2288770079207,13.4244557903887));
#78660=CARTESIAN_POINT('Ctrl Pts',(89.0920283415751,56.2337029911507,13.385231311997));
#78661=CARTESIAN_POINT('Ctrl Pts',(89.1414669162095,56.2385289743808,13.343108532046));
#78662=CARTESIAN_POINT('Ctrl Pts',(89.1882557510482,56.2433549576109,13.2984137828765));
#78663=CARTESIAN_POINT('Ctrl Pts',(89.2328267172351,56.2479521812029,13.2558376392124));
#78664=CARTESIAN_POINT('Ctrl Pts',(89.2751765111576,56.252549404795,13.2107530770504));
#78665=CARTESIAN_POINT('Ctrl Pts',(89.3150099307752,56.2571466283871,13.1634210386354));
#78666=CARTESIAN_POINT('Ctrl Pts',(89.3555254069417,56.2618225689582,13.1152785469105));
#78667=CARTESIAN_POINT('Ctrl Pts',(89.3934370743049,56.2664985095293,13.0648111863052));
#78668=CARTESIAN_POINT('Ctrl Pts',(89.428471601609,56.2711744501005,13.0123345572428));
#78669=CARTESIAN_POINT('Ctrl Pts',(89.4628215968074,56.2757590284729,12.9608832577669));
#78670=CARTESIAN_POINT('Ctrl Pts',(89.4944055762479,56.2803436068453,12.9075009446471));
#78671=CARTESIAN_POINT('Ctrl Pts',(89.5230065515739,56.2849281852177,12.8525182919663));
#78672=CARTESIAN_POINT('Ctrl Pts',(89.5515900464819,56.2895099615757,12.7975692437251));
#78673=CARTESIAN_POINT('Ctrl Pts',(89.5771939179111,56.2940917379336,12.7410222460178));
#78674=CARTESIAN_POINT('Ctrl Pts',(89.5996462730734,56.2986735142916,12.683234035557));
#78675=CARTESIAN_POINT('Ctrl Pts',(89.6220931524138,56.303254173217,12.6254599188493));
#78676=CARTESIAN_POINT('Ctrl Pts',(89.6413898570269,56.3078348321425,12.5664456646026));
#78677=CARTESIAN_POINT('Ctrl Pts',(89.6574127686622,56.3124154910679,12.5065676233974));
#78678=CARTESIAN_POINT('Ctrl Pts',(89.6740145337125,56.3171616336534,12.4445263917917));
#78679=CARTESIAN_POINT('Ctrl Pts',(89.6871012226801,56.321907776239,12.3815583119947));
#78680=CARTESIAN_POINT('Ctrl Pts',(89.6965925739576,56.3266539188245,12.3180962320605));
#78681=CARTESIAN_POINT('Ctrl Pts',(89.7057645940771,56.3312403801209,12.256769297995));
#78682=CARTESIAN_POINT('Ctrl Pts',(89.7115793988327,56.3358268414173,12.194981611144));
#78683=CARTESIAN_POINT('Ctrl Pts',(89.7140174858883,56.3404133027136,12.1331288191363));
#78684=CARTESIAN_POINT('Ctrl Pts',(89.7165828988469,56.3452392859437,12.0680458460833));
#78685=CARTESIAN_POINT('Ctrl Pts',(89.7154092342088,56.3500652691738,12.002891425418));
#78686=CARTESIAN_POINT('Ctrl Pts',(89.7105359120319,56.3548912524039,11.9381230305569));
#78687=CARTESIAN_POINT('Ctrl Pts',(89.705662589855,56.3597172356339,11.8733546356957));
#78688=CARTESIAN_POINT('Ctrl Pts',(89.6970897723693,56.364543218864,11.8089728987431));
#78689=CARTESIAN_POINT('Ctrl Pts',(89.6849189735046,56.3693692020941,11.7454222313675));
#78690=CARTESIAN_POINT('Ctrl Pts',(89.6733250907644,56.3739664256862,11.6848839714062));
#78691=CARTESIAN_POINT('Ctrl Pts',(89.6584190714499,56.3785636492783,11.6248512021979));
#78692=CARTESIAN_POINT('Ctrl Pts',(89.6402600214436,56.3831608728703,11.5657134639774));
#78693=CARTESIAN_POINT('Ctrl Pts',(89.6217900390822,56.3878368134415,11.5055631267377));
#78694=CARTESIAN_POINT('Ctrl Pts',(89.5999545824805,56.3925127540126,11.4463392983937));
#78695=CARTESIAN_POINT('Ctrl Pts',(89.5748705397008,56.3971886945837,11.3884427915993));
#78696=CARTESIAN_POINT('Ctrl Pts',(89.5502766086465,56.4017732729561,11.3316775122184));
#78697=CARTESIAN_POINT('Ctrl Pts',(89.5225601086229,56.4063578513286,11.276188641823));
#78698=CARTESIAN_POINT('Ctrl Pts',(89.4918811517115,56.410942429701,11.2223378341387));
#78699=CARTESIAN_POINT('Ctrl Pts',(89.4612209452442,56.4155242060589,11.1685199391302));
#78700=CARTESIAN_POINT('Ctrl Pts',(89.4276021235109,56.4201059824169,11.1163385630737));
#78701=CARTESIAN_POINT('Ctrl Pts',(89.391231154141,56.4246877587749,11.0661316102913));
#78702=CARTESIAN_POINT('Ctrl Pts',(89.3548690551524,56.4292684177003,11.0159369022971));
#78703=CARTESIAN_POINT('Ctrl Pts',(89.3157564394869,56.4338490766258,10.9677160737162));
#78704=CARTESIAN_POINT('Ctrl Pts',(89.2741424368487,56.4384297355512,10.9217771109474));
#78705=CARTESIAN_POINT('Ctrl Pts',(89.2310250615346,56.4431758781367,10.8741785293722));
#78706=CARTESIAN_POINT('Ctrl Pts',(89.1852224485135,56.4479220207223,10.8290303163191));
#78707=CARTESIAN_POINT('Ctrl Pts',(89.1370547088028,56.4526681633078,10.7866346775127));
#78708=CARTESIAN_POINT('Ctrl Pts',(89.0905075455144,56.4572546246042,10.7456654160507));
#78709=CARTESIAN_POINT('Ctrl Pts',(89.0417523445954,56.4618410859006,10.7072667105503));
#78710=CARTESIAN_POINT('Ctrl Pts',(88.9911109199524,56.466427547197,10.6716695441216));
#78711=CARTESIAN_POINT('Ctrl Pts',(88.9378248132396,56.471253530427,10.6342133623027));
#78712=CARTESIAN_POINT('Ctrl Pts',(88.8824506108117,56.4760795136571,10.599859705636));
#78713=CARTESIAN_POINT('Ctrl Pts',(88.8253940271616,56.4809054968872,10.5688235895114));
#78714=CARTESIAN_POINT('Ctrl Pts',(88.7683374435115,56.4857314801172,10.5377874733868));
#78715=CARTESIAN_POINT('Ctrl Pts',(88.7095990976767,56.4905574633473,10.5100691043642));
#78716=CARTESIAN_POINT('Ctrl Pts',(88.6496074103387,56.4953834465774,10.4858242467813));
#78717=CARTESIAN_POINT('Ctrl Pts',(88.5924594288372,56.4999806701695,10.4627286358035));
#78718=CARTESIAN_POINT('Ctrl Pts',(88.5339396220379,56.5045778937615,10.4426897984422));
#78719=CARTESIAN_POINT('Ctrl Pts',(88.4744073098968,56.5091751173536,10.4258693647352));
#78720=CARTESIAN_POINT('Ctrl Pts',(88.4138556425571,56.5138510579247,10.408760919427));
#78721=CARTESIAN_POINT('Ctrl Pts',(88.3522569258906,56.5185269984959,10.3949824175572));
#78722=CARTESIAN_POINT('Ctrl Pts',(88.290011291034,56.523202939067,10.3846530592779));
#78723=CARTESIAN_POINT('Ctrl Pts',(88.2289818602702,56.5277875174394,10.3745255241119));
#78724=CARTESIAN_POINT('Ctrl Pts',(88.1673310901714,56.5323720958118,10.3677136478994));
#78725=CARTESIAN_POINT('Ctrl Pts',(88.1054496582838,56.5369566741842,10.3642790776246));
#78726=CARTESIAN_POINT('Ctrl Pts',(88.0436060472497,56.5415384505422,10.3608466064994));
#78727=CARTESIAN_POINT('Ctrl Pts',(87.9815325611732,56.5461202269001,10.3607873765511));
#78728=CARTESIAN_POINT('Ctrl Pts',(87.9196250684157,56.5507020032581,10.3641112088394));
#78729=CARTESIAN_POINT('Ctrl Pts',(87.8577326740479,56.5552826621835,10.3674342304906));
#78730=CARTESIAN_POINT('Ctrl Pts',(87.7960067007206,56.559863321109,10.3741386491852));
#78731=CARTESIAN_POINT('Ctrl Pts',(87.7348410219715,56.5644439800344,10.3841822172262));
#78732=CARTESIAN_POINT('Ctrl Pts',(87.6714656348476,56.56919012262,10.3945886252922));
#78733=CARTESIAN_POINT('Ctrl Pts',(87.6086923845848,56.5739362652055,10.4085800352604));
#78734=CARTESIAN_POINT('Ctrl Pts',(87.5469487884302,56.578682407791,10.4260514310989));
#78735=CARTESIAN_POINT('Ctrl Pts',(87.4872825207273,56.5832688690874,10.4429350116834));
#78736=CARTESIAN_POINT('Ctrl Pts',(87.4285781946293,56.5878553303838,10.4630678778013));
#78737=CARTESIAN_POINT('Ctrl Pts',(87.3712044154017,56.5924417916802,10.4863049517301));
#78738=CARTESIAN_POINT('Ctrl Pts',(87.3108343657043,56.5972677749102,10.5107555514079));
#78739=CARTESIAN_POINT('Ctrl Pts',(87.2519382325376,56.6020937581403,10.5386432103078));
#78740=CARTESIAN_POINT('Ctrl Pts',(87.1949167139219,56.6069197413704,10.5697437031765));
#78741=CARTESIAN_POINT('Ctrl Pts',(87.1378951953061,56.6117457246004,10.6008441960452));
#78742=CARTESIAN_POINT('Ctrl Pts',(87.0827488005417,56.6165717078305,10.6351571148539));
#78743=CARTESIAN_POINT('Ctrl Pts',(87.0298407653942,56.6213976910606,10.6724070207023));
#78744=CARTESIAN_POINT('Ctrl Pts',(86.9797608584156,56.6259657078196,10.7076657827155));
#78745=CARTESIAN_POINT('Ctrl Pts',(86.9314747164261,56.6305337245787,10.7457045104822));
#78746=CARTESIAN_POINT('Ctrl Pts',(86.8853106759136,56.6351017413377,10.7863131706398));
#78747=CARTESIAN_POINT('Ctrl Pts',(86.8392274476728,56.6396617615738,10.826850743474));
#78748=CARTESIAN_POINT('Ctrl Pts',(86.7952593321464,56.6442217818098,10.8699489816961));
#78749=CARTESIAN_POINT('Ctrl Pts',(86.7537043789943,56.6487818020459,10.9153555905494));
#78750=CARTESIAN_POINT('Ctrl Pts',(86.7121899853957,56.6533373714916,10.9607178804554));
#78751=CARTESIAN_POINT('Ctrl Pts',(86.6730844345984,56.6578929409373,11.0083836984446));
#78752=CARTESIAN_POINT('Ctrl Pts',(86.6366501883998,56.6624485103831,11.0580627842199));
#78753=CARTESIAN_POINT('Ctrl Pts',(86.6002376828568,56.6670013614779,11.1077122260199));
#78754=CARTESIAN_POINT('Ctrl Pts',(86.566493627052,56.6715542125726,11.1593721388688));
#78755=CARTESIAN_POINT('Ctrl Pts',(86.5356399060811,56.6761070636674,11.212719607121));
#78756=CARTESIAN_POINT('Ctrl Pts',(86.5047928926333,56.6806589249836,11.2660554777648));
#78757=CARTESIAN_POINT('Ctrl Pts',(86.4768352248621,56.6852107862998,11.3210777286816));
#78758=CARTESIAN_POINT('Ctrl Pts',(86.4519440347309,56.6897626476159,11.3774367619756));
#78759=CARTESIAN_POINT('Ctrl Pts',(86.4270313025592,56.6943184483331,11.433844571104));
#78760=CARTESIAN_POINT('Ctrl Pts',(86.405190560342,56.6988742490503,11.4915910011074));
#78761=CARTESIAN_POINT('Ctrl Pts',(86.3865511661085,56.7034300497675,11.5503054957936));
#78762=CARTESIAN_POINT('Ctrl Pts',(86.3679040418857,56.7079877398321,11.6090443401136));
#78763=CARTESIAN_POINT('Ctrl Pts',(86.3524610408587,56.7125454298968,11.6687515484091));
#78764=CARTESIAN_POINT('Ctrl Pts',(86.3403010154367,56.7171031199614,11.7290434173679));
#78765=CARTESIAN_POINT('Ctrl Pts',(86.3281186032256,56.7216692008018,11.7894462845612));
#78766=CARTESIAN_POINT('Ctrl Pts',(86.3192313151102,56.7262352816421,11.8504354504348));
#78767=CARTESIAN_POINT('Ctrl Pts',(86.3136663080636,56.7308013624825,11.9116200342736));
#78768=CARTESIAN_POINT('Ctrl Pts',(86.3089786900743,56.7346475467746,11.9631581461708));
#78769=CARTESIAN_POINT('Ctrl Pts',(86.3066474220475,56.7384937310667,12.0148346679399));
#78770=CARTESIAN_POINT('Ctrl Pts',(86.3066600510811,56.7423399153589,12.0664172756536));
#78771=CARTESIAN_POINT('',(86.3066607042565,57.5360899153607,12.064450618022));
#78772=CARTESIAN_POINT('Ctrl Pts',(86.3066600510813,56.7423399154299,12.0664172766061));
#78773=CARTESIAN_POINT('Ctrl Pts',(86.3066656024584,56.7440305888012,12.0890915258513));
#78774=CARTESIAN_POINT('Ctrl Pts',(86.3071236157404,56.7457212621725,12.1117596676896));
#78775=CARTESIAN_POINT('Ctrl Pts',(86.3080334792289,56.7474119355438,12.1344095368553));
#78776=CARTESIAN_POINT('Ctrl Pts',(86.3105075501914,56.7520091591358,12.1959983183745));
#78777=CARTESIAN_POINT('Ctrl Pts',(86.316332099658,56.7566063827279,12.2575791385552));
#78778=CARTESIAN_POINT('Ctrl Pts',(86.3255065323334,56.7612036063199,12.3187579989896));
#78779=CARTESIAN_POINT('Ctrl Pts',(86.334838056264,56.765879546891,12.3809844080103));
#78780=CARTESIAN_POINT('Ctrl Pts',(86.3476353350051,56.7705554874621,12.4427944287638));
#78781=CARTESIAN_POINT('Ctrl Pts',(86.363842306128,56.7752314280333,12.5037743335537));
#78782=CARTESIAN_POINT('Ctrl Pts',(86.3797326127225,56.7798160064057,12.5635627650787));
#78783=CARTESIAN_POINT('Ctrl Pts',(86.3989004305176,56.7844005847781,12.6225527122926));
#78784=CARTESIAN_POINT('Ctrl Pts',(86.4212411365165,56.7889851631505,12.6803627524318));
#78785=CARTESIAN_POINT('Ctrl Pts',(86.4435681882649,56.7935669395084,12.7381374600814));
#78786=CARTESIAN_POINT('Ctrl Pts',(86.4690640999206,56.7981487158664,12.7947332167309));
#78787=CARTESIAN_POINT('Ctrl Pts',(86.4975748797646,56.8027304922244,12.8497852008303));
#78788=CARTESIAN_POINT('Ctrl Pts',(86.5260787062199,56.8073111511498,12.9048237585048));
#78789=CARTESIAN_POINT('Ctrl Pts',(86.5575957072175,56.8118918100753,12.9583188392258));
#78790=CARTESIAN_POINT('Ctrl Pts',(86.5919252586688,56.8164724690008,13.0099288713223));
#78791=CARTESIAN_POINT('Ctrl Pts',(86.6274950202983,56.8212186115863,13.0634033987121));
#78792=CARTESIAN_POINT('Ctrl Pts',(86.6660841703194,56.8259647541718,13.1148535493639));
#78793=CARTESIAN_POINT('Ctrl Pts',(86.7074210320166,56.8307108967573,13.1639329259255));
#78794=CARTESIAN_POINT('Ctrl Pts',(86.7473671383277,56.8352973580538,13.2113610545574));
#78795=CARTESIAN_POINT('Ctrl Pts',(86.7898785758916,56.8398838193502,13.2565750775701));
#78796=CARTESIAN_POINT('Ctrl Pts',(86.8346714059086,56.8444702806466,13.2992987773946));
#78797=CARTESIAN_POINT('Ctrl Pts',(86.8818034828019,56.8492962638767,13.3442536664812));
#78798=CARTESIAN_POINT('Ctrl Pts',(86.9314612880865,56.8541222471067,13.3864505667847));
#78799=CARTESIAN_POINT('Ctrl Pts',(86.9832755413533,56.8589482303368,13.4256165903296));
#78800=CARTESIAN_POINT('Ctrl Pts',(87.0350897946201,56.8637742135669,13.4647826138744));
#78801=CARTESIAN_POINT('Ctrl Pts',(87.0890599143759,56.868600196797,13.5009174644516));
#78802=CARTESIAN_POINT('Ctrl Pts',(87.1447853658042,56.8734261800271,13.5338034756414));
#78803=CARTESIAN_POINT('Ctrl Pts',(87.1978693380795,56.8780234036192,13.5651306351619));
#78804=CARTESIAN_POINT('Ctrl Pts',(87.2527639172621,56.8826206272113,13.5936386685382));
#78805=CARTESIAN_POINT('Ctrl Pts',(87.3091377740607,56.8872178508033,13.6191143716416));
#78806=CARTESIAN_POINT('Ctrl Pts',(87.3664769047068,56.8918937913745,13.6450262881131));
#78807=CARTESIAN_POINT('Ctrl Pts',(87.4253460398766,56.8965697319456,13.667800702114));
#78808=CARTESIAN_POINT('Ctrl Pts',(87.4853671899815,56.9012456725167,13.6872603074868));
#78809=CARTESIAN_POINT('Ctrl Pts',(87.5442155997233,56.9058302508891,13.7063396958088));
#78810=CARTESIAN_POINT('Ctrl Pts',(87.6041709039119,56.9104148292616,13.7222324806806));
#78811=CARTESIAN_POINT('Ctrl Pts',(87.6648559138243,56.914999407634,13.7348196748617));
#78812=CARTESIAN_POINT('Ctrl Pts',(87.7255038341156,56.9195811839919,13.7473991759689));
#78813=CARTESIAN_POINT('Ctrl Pts',(87.7868800784062,56.9241629603499,13.7566769892163));
#78814=CARTESIAN_POINT('Ctrl Pts',(87.8485946274706,56.9287447367078,13.7625846075494));
#78815=CARTESIAN_POINT('Ctrl Pts',(87.9102941252017,56.9333253956333,13.7684907850954));
#78816=CARTESIAN_POINT('Ctrl Pts',(87.9723312574121,56.9379060545587,13.7710283509263));
#78817=CARTESIAN_POINT('Ctrl Pts',(88.0343102442518,56.9424867134842,13.7701805855346));
#78818=CARTESIAN_POINT('Ctrl Pts',(88.0985283215272,56.9472328560697,13.7693021932565));
#78819=CARTESIAN_POINT('Ctrl Pts',(88.162683389576,56.9519789986552,13.7647891294288));
#78820=CARTESIAN_POINT('Ctrl Pts',(88.2263370755343,56.9567251412407,13.7566817499164));
#78821=CARTESIAN_POINT('Ctrl Pts',(88.2878491691474,56.9613116025371,13.7488471386128));
#78822=CARTESIAN_POINT('Ctrl Pts',(88.3488925782536,56.9658980638335,13.7376564100642));
#78823=CARTESIAN_POINT('Ctrl Pts',(88.4090812385715,56.9704845251299,13.7231982871996));
#78824=CARTESIAN_POINT('Ctrl Pts',(88.472413172837,56.9753105083599,13.7079851078063));
#78825=CARTESIAN_POINT('Ctrl Pts',(88.5347980142919,56.98013649159,13.6891540808148));
#78826=CARTESIAN_POINT('Ctrl Pts',(88.5958062067336,56.98496247482,13.6668674324146));
#78827=CARTESIAN_POINT('Ctrl Pts',(88.6568143991754,56.9897884580501,13.6445807840144));
#78828=CARTESIAN_POINT('Ctrl Pts',(88.7164453783511,56.9946144412802,13.618838842067));
#78829=CARTESIAN_POINT('Ctrl Pts',(88.7742990285047,56.9994404245102,13.5898600423542));
#78830=CARTESIAN_POINT('Ctrl Pts',(88.8294103193431,57.0040376481023,13.5622548859833));
#78831=CARTESIAN_POINT('Ctrl Pts',(88.8831352735712,57.0086348716944,13.5315995098839));
#78832=CARTESIAN_POINT('Ctrl Pts',(88.935115061289,57.0132320952865,13.4980566291522));
#78833=CARTESIAN_POINT('Ctrl Pts',(88.9879848844333,57.0179080358576,13.4639394030169));
#78834=CARTESIAN_POINT('Ctrl Pts',(89.0390486978894,57.0225839764287,13.4268350102305));
#78835=CARTESIAN_POINT('Ctrl Pts',(89.0879525219152,57.0272599169998,13.3869648372082));
#78836=CARTESIAN_POINT('Ctrl Pts',(89.1359008246249,57.0318444953722,13.3478736789349));
#78837=CARTESIAN_POINT('Ctrl Pts',(89.1817723724914,57.0364290737447,13.3061241854332));
#78838=CARTESIAN_POINT('Ctrl Pts',(89.2252626151182,57.0410136521171,13.2619687024024));
#78839=CARTESIAN_POINT('Ctrl Pts',(89.2687262772663,57.045595428475,13.2178402064339));
#78840=CARTESIAN_POINT('Ctrl Pts',(89.3098111635798,57.050177204833,13.1713089986429));
#78841=CARTESIAN_POINT('Ctrl Pts',(89.3482481738866,57.054758981191,13.1226655842966));
#78842=CARTESIAN_POINT('Ctrl Pts',(89.386675809933,57.0593396401164,13.0740340334129));
#78843=CARTESIAN_POINT('Ctrl Pts',(89.422456536485,57.0639202990419,13.0232916978276));
#78844=CARTESIAN_POINT('Ctrl Pts',(89.455361636629,57.0685009579673,12.9707620119314));
#78845=CARTESIAN_POINT('Ctrl Pts',(89.4894554863603,57.0732471005528,12.9163346067715));
#78846=CARTESIAN_POINT('Ctrl Pts',(89.5204615954466,57.0779932431384,12.859988695644));
#78847=CARTESIAN_POINT('Ctrl Pts',(89.5481760948056,57.0827393857239,12.8021144538441));
#78848=CARTESIAN_POINT('Ctrl Pts',(89.5749581554726,57.0873258470203,12.7461873582519));
#78849=CARTESIAN_POINT('Ctrl Pts',(89.5986664570931,57.0919123083167,12.6888336605941));
#78850=CARTESIAN_POINT('Ctrl Pts',(89.6191661368895,57.0964987696131,12.6304258248537));
#78851=CARTESIAN_POINT('Ctrl Pts',(89.640736385612,57.1013247528431,12.5689677163967));
#78852=CARTESIAN_POINT('Ctrl Pts',(89.6587535020052,57.1061507360732,12.5063429645986));
#78853=CARTESIAN_POINT('Ctrl Pts',(89.6731207849723,57.1109767193033,12.4430004400036));
#78854=CARTESIAN_POINT('Ctrl Pts',(89.6874880679395,57.1158027025334,12.3796579154086));
#78855=CARTESIAN_POINT('Ctrl Pts',(89.6982054868738,57.1206286857634,12.3155982698893));
#78856=CARTESIAN_POINT('Ctrl Pts',(89.7052395320091,57.1254546689935,12.251276128461));
#78857=CARTESIAN_POINT('Ctrl Pts',(89.7119401516968,57.1300518925856,12.1900029636012));
#78858=CARTESIAN_POINT('Ctrl Pts',(89.7153262699519,57.1346491161777,12.1282400540699));
#78859=CARTESIAN_POINT('Ctrl Pts',(89.7153399582779,57.1392463397698,12.0663771169298));
#78860=CARTESIAN_POINT('Ctrl Pts',(89.7153538809853,57.1439222803409,12.0034549179486));
#78861=CARTESIAN_POINT('Ctrl Pts',(89.711878644327,57.148598220912,11.9404297504446));
#78862=CARTESIAN_POINT('Ctrl Pts',(89.7049082415433,57.1532741614831,11.8777190800113));
#78863=CARTESIAN_POINT('Ctrl Pts',(89.6980740319627,57.1578587398555,11.8162336999011));
#78864=CARTESIAN_POINT('Ctrl Pts',(89.6878800694191,57.162443318228,11.7550511677618));
#78865=CARTESIAN_POINT('Ctrl Pts',(89.6743731671188,57.1670278966004,11.6945642148242));
#78866=CARTESIAN_POINT('Ctrl Pts',(89.6608745200019,57.1716096729583,11.6341142304588));
#78867=CARTESIAN_POINT('Ctrl Pts',(89.6440670587452,57.1761914493163,11.5743594781124));
#78868=CARTESIAN_POINT('Ctrl Pts',(89.6240488833731,57.1807732256743,11.5156836042342));
#78869=CARTESIAN_POINT('Ctrl Pts',(89.6040355901599,57.1853538845997,11.4570220405981));
#78870=CARTESIAN_POINT('Ctrl Pts',(89.580813301596,57.1899345435252,11.3994393146546));
#78871=CARTESIAN_POINT('Ctrl Pts',(89.5545296859893,57.1945152024506,11.3433030067382));
#78872=CARTESIAN_POINT('Ctrl Pts',(89.5272965325583,57.1992613450361,11.2851386845454));
#78873=CARTESIAN_POINT('Ctrl Pts',(89.4967768149411,57.2040074876216,11.228527843375));
#78874=CARTESIAN_POINT('Ctrl Pts',(89.4631877493251,57.2087536302072,11.1738533885566));
#78875=CARTESIAN_POINT('Ctrl Pts',(89.4307287688681,57.2133400915035,11.1210184249186));
#78876=CARTESIAN_POINT('Ctrl Pts',(89.3954040667084,57.2179265527999,11.0699920041341));
#78877=CARTESIAN_POINT('Ctrl Pts',(89.35745340832,57.2225130140963,11.0210894512813));
#78878=CARTESIAN_POINT('Ctrl Pts',(89.3175208265065,57.2273389973264,10.9696330266604));
#78879=CARTESIAN_POINT('Ctrl Pts',(89.2746809083428,57.2321649805565,10.9205288778271));
#78880=CARTESIAN_POINT('Ctrl Pts',(89.2292583089208,57.2369909637865,10.8741017122483));
#78881=CARTESIAN_POINT('Ctrl Pts',(89.1838357094989,57.2418169470166,10.8276745466695));
#78882=CARTESIAN_POINT('Ctrl Pts',(89.1358309598696,57.2466429302467,10.7839247436333));
#78883=CARTESIAN_POINT('Ctrl Pts',(89.0856078244774,57.2514689134767,10.7431270434498));
#78884=CARTESIAN_POINT('Ctrl Pts',(89.0377653492997,57.2560661370688,10.7042632221631));
#78885=CARTESIAN_POINT('Ctrl Pts',(88.9877136477779,57.2606633606609,10.6679183467968));
#78886=CARTESIAN_POINT('Ctrl Pts',(88.9357487091222,57.265260584253,10.6343524663603));
#78887=CARTESIAN_POINT('Ctrl Pts',(88.8828939892964,57.2699365248241,10.6002118467025));
#78888=CARTESIAN_POINT('Ctrl Pts',(88.8280602477108,57.2746124653952,10.5689466936973));
#78889=CARTESIAN_POINT('Ctrl Pts',(88.7715949479891,57.2792884059663,10.5407884865719));
#78890=CARTESIAN_POINT('Ctrl Pts',(88.7162329116333,57.2838729843387,10.513180456609));
#78891=CARTESIAN_POINT('Ctrl Pts',(88.6593029784183,57.2884575627112,10.4885592906041));
#78892=CARTESIAN_POINT('Ctrl Pts',(88.6011604815904,57.2930421410836,10.4670986767255));
#78893=CARTESIAN_POINT('Ctrl Pts',(88.5430535204439,57.2976239174415,10.4456511792003));
#78894=CARTESIAN_POINT('Ctrl Pts',(88.4837359417387,57.3022056937995,10.4273605794718));
#78895=CARTESIAN_POINT('Ctrl Pts',(88.4235832643108,57.3067874701574,10.412352550992));
#78896=CARTESIAN_POINT('Ctrl Pts',(88.3634452572971,57.3113681290829,10.3973481827648));
#78897=CARTESIAN_POINT('Ctrl Pts',(88.3024730495601,57.3159487880083,10.3856249196992));
#78898=CARTESIAN_POINT('Ctrl Pts',(88.2410555482283,57.3205294469338,10.377258077642));
#78899=CARTESIAN_POINT('Ctrl Pts',(88.1774192410267,57.3252755895193,10.3685889699787));
#78900=CARTESIAN_POINT('Ctrl Pts',(88.1133054177713,57.3300217321048,10.3635235806528));
#78901=CARTESIAN_POINT('Ctrl Pts',(88.0491535831273,57.3347678746903,10.3620871091237));
#78902=CARTESIAN_POINT('Ctrl Pts',(87.98716010076,57.3393543359867,10.3606989668686));
#78903=CARTESIAN_POINT('Ctrl Pts',(87.9251316496256,57.3439407972831,10.3626993294924));
#78904=CARTESIAN_POINT('Ctrl Pts',(87.8634631894947,57.3485272585795,10.3680577968771));
#78905=CARTESIAN_POINT('Ctrl Pts',(87.7985741748093,57.3533532418095,10.3736961032022));
#78906=CARTESIAN_POINT('Ctrl Pts',(87.7340844211728,57.3581792250396,10.3830527958237));
#78907=CARTESIAN_POINT('Ctrl Pts',(87.6704428147227,57.3630052082697,10.396031246054));
#78908=CARTESIAN_POINT('Ctrl Pts',(87.6068012082727,57.3678311914997,10.4090096962842));
#78909=CARTESIAN_POINT('Ctrl Pts',(87.5440083556983,57.3726571747298,10.4256096637016));
#78910=CARTESIAN_POINT('Ctrl Pts',(87.4824923775355,57.3774831579599,10.4456745608993));
#78911=CARTESIAN_POINT('Ctrl Pts',(87.4238923591315,57.382080381552,10.4647883485716));
#78912=CARTESIAN_POINT('Ctrl Pts',(87.3662102788873,57.386677605144,10.4871244272184));
#78913=CARTESIAN_POINT('Ctrl Pts',(87.3098251536625,57.3912748287361,10.5125751802988));
#78914=CARTESIAN_POINT('Ctrl Pts',(87.2524745616443,57.3959507693072,10.5384617195351));
#78915=CARTESIAN_POINT('Ctrl Pts',(87.1964662910824,57.4006267098784,10.567570526405));
#78916=CARTESIAN_POINT('Ctrl Pts',(87.1421832764163,57.4053026504495,10.5997352434089));
#78917=CARTESIAN_POINT('Ctrl Pts',(87.0889608859171,57.4098872288219,10.6312715009142));
#78918=CARTESIAN_POINT('Ctrl Pts',(87.0373973977466,57.4144718071943,10.6657450530811));
#78919=CARTESIAN_POINT('Ctrl Pts',(86.9878314633255,57.4190563855668,10.7029515851741));
#78920=CARTESIAN_POINT('Ctrl Pts',(86.9382958227402,57.4236381619247,10.7401353772827));
#78921=CARTESIAN_POINT('Ctrl Pts',(86.890755721362,57.4282199382827,10.7800485322924));
#78922=CARTESIAN_POINT('Ctrl Pts',(86.8455204210706,57.4328017146406,10.8224437340038));
#78923=CARTESIAN_POINT('Ctrl Pts',(86.8002961530495,57.4373823735661,10.864828596106));
#78924=CARTESIAN_POINT('Ctrl Pts',(86.7573759414981,57.4419630324916,10.9096939552778));
#78925=CARTESIAN_POINT('Ctrl Pts',(86.7170340035995,57.446543691417,10.9567539336291));
#78926=CARTESIAN_POINT('Ctrl Pts',(86.6752346484066,57.4512898340025,11.005514029275));
#78927=CARTESIAN_POINT('Ctrl Pts',(86.6362038491661,57.456035976588,11.0566299486358));
#78928=CARTESIAN_POINT('Ctrl Pts',(86.600201163264,57.4607821191736,11.1097461226931));
#78929=CARTESIAN_POINT('Ctrl Pts',(86.5654097674134,57.46536858047,11.1610752330469));
#78930=CARTESIAN_POINT('Ctrl Pts',(86.5334461592334,57.4699550417664,11.2142716422571));
#78931=CARTESIAN_POINT('Ctrl Pts',(86.504499024632,57.4745415030628,11.2689870472726));
#78932=CARTESIAN_POINT('Ctrl Pts',(86.4740401638422,57.4793674862928,11.3265598926465));
#78933=CARTESIAN_POINT('Ctrl Pts',(86.4469217568009,57.4841934695229,11.3858141584882));
#78934=CARTESIAN_POINT('Ctrl Pts',(86.4233060989873,57.489019452753,11.4463203147696));
#78935=CARTESIAN_POINT('Ctrl Pts',(86.3996904411738,57.493845435983,11.5068264710511));
#78936=CARTESIAN_POINT('Ctrl Pts',(86.3795776596723,57.4986714192131,11.5685838776753));
#78937=CARTESIAN_POINT('Ctrl Pts',(86.3630684141364,57.5034974024432,11.6311479287007));
#78938=CARTESIAN_POINT('Ctrl Pts',(86.3429813041155,57.5093692671442,11.7072707880753));
#78939=CARTESIAN_POINT('Ctrl Pts',(86.3281593659612,57.5152411318451,11.7848369403936));
#78940=CARTESIAN_POINT('Ctrl Pts',(86.3187675222516,57.5211129965461,11.8632092781867));
#78941=CARTESIAN_POINT('Ctrl Pts',(86.3107825017104,57.5261053028176,11.929842065794));
#78942=CARTESIAN_POINT('Ctrl Pts',(86.3067219701062,57.5310976090892,11.9970574272591));
#78943=CARTESIAN_POINT('Ctrl Pts',(86.3066607042565,57.5360899153607,12.064450618022));
#78944=CARTESIAN_POINT('',(86.3066600816788,58.3298399155007,12.0665276521619));
#78945=CARTESIAN_POINT('Ctrl Pts',(86.3066607042556,57.5360899154299,12.064450618956));
#78946=CARTESIAN_POINT('Ctrl Pts',(86.3066050417779,57.5406256283189,12.1256800683038));
#78947=CARTESIAN_POINT('Ctrl Pts',(86.3098532065461,57.5451613412079,12.1869899608666));
#78948=CARTESIAN_POINT('Ctrl Pts',(86.3164045293079,57.5496970540969,12.2479918303384));
#78949=CARTESIAN_POINT('Ctrl Pts',(86.3229518351935,57.5542299859601,12.3089562971408));
#78950=CARTESIAN_POINT('Ctrl Pts',(86.3327982305187,57.5587629178234,12.369612598124));
#78951=CARTESIAN_POINT('Ctrl Pts',(86.3458910537401,57.5632958496866,12.4295753466414));
#78952=CARTESIAN_POINT('Ctrl Pts',(86.3589809092653,57.5678277540889,12.4895245036498));
#78953=CARTESIAN_POINT('Ctrl Pts',(86.3753156211357,57.5723596584911,12.5487799113382));
#78954=CARTESIAN_POINT('Ctrl Pts',(86.3947914680293,57.5768915628934,12.6069665579176));
#78955=CARTESIAN_POINT('Ctrl Pts',(86.4142844559702,57.5814274559072,12.6652044156236));
#78956=CARTESIAN_POINT('Ctrl Pts',(86.4369239375402,57.5859633489211,12.7223711372686));
#78957=CARTESIAN_POINT('Ctrl Pts',(86.4625567634577,57.5904992419349,12.7781084038307));
#78958=CARTESIAN_POINT('Ctrl Pts',(86.4882003017455,57.5950370305714,12.8338689638932));
#78959=CARTESIAN_POINT('Ctrl Pts',(86.5168394326287,57.5995748192078,12.8881984172555));
#78960=CARTESIAN_POINT('Ctrl Pts',(86.5482748589299,57.6041126078443,12.9407628234451));
#78961=CARTESIAN_POINT('Ctrl Pts',(86.5797695730835,57.6086589548423,12.9934263671721));
#78962=CARTESIAN_POINT('Ctrl Pts',(86.6140708247473,57.6132053018403,13.0443177814376));
#78963=CARTESIAN_POINT('Ctrl Pts',(86.6509363382424,57.6177516488383,13.0931327429143));
#78964=CARTESIAN_POINT('Ctrl Pts',(86.6827229109502,57.621671648201,13.1352224949642));
#78965=CARTESIAN_POINT('Ctrl Pts',(86.7164150464297,57.6255916475637,13.1757689032637));
#78966=CARTESIAN_POINT('Ctrl Pts',(86.7518355149009,57.6295116469264,13.2145989879262));
#78967=CARTESIAN_POINT('Ctrl Pts',(86.7933752699446,57.6341088705185,13.2601374089248));
#78968=CARTESIAN_POINT('Ctrl Pts',(86.8374738665761,57.6387060941105,13.3035129384981));
#78969=CARTESIAN_POINT('Ctrl Pts',(86.8838772211828,57.6433033177026,13.3444244510613));
#78970=CARTESIAN_POINT('Ctrl Pts',(86.9310751275051,57.6479792582738,13.3860364800585));
#78971=CARTESIAN_POINT('Ctrl Pts',(86.9806571749383,57.6526551988449,13.425098860696));
#78972=CARTESIAN_POINT('Ctrl Pts',(87.0323141331252,57.657331139416,13.4613310752576));
#78973=CARTESIAN_POINT('Ctrl Pts',(87.0829617770989,57.6619157177884,13.4968553563595));
#78974=CARTESIAN_POINT('Ctrl Pts',(87.135603541871,57.6665002961608,13.5296587664414));
#78975=CARTESIAN_POINT('Ctrl Pts',(87.1899138315338,57.6710848745332,13.5595167690901));
#78976=CARTESIAN_POINT('Ctrl Pts',(87.2441909276934,57.6756666508912,13.5893565230477));
#78977=CARTESIAN_POINT('Ctrl Pts',(87.3001340815269,57.6802484272491,13.6162541943417));
#78978=CARTESIAN_POINT('Ctrl Pts',(87.3573906041994,57.6848302036071,13.6400297307615));
#78979=CARTESIAN_POINT('Ctrl Pts',(87.4146331627901,57.6894108625325,13.6637994686536));
#78980=CARTESIAN_POINT('Ctrl Pts',(87.4731879844347,57.693991521458,13.6844483881265));
#78981=CARTESIAN_POINT('Ctrl Pts',(87.5326816613113,57.6985721803834,13.7018442476208));
#78982=CARTESIAN_POINT('Ctrl Pts',(87.5943246428098,57.703318322969,13.7198685604764));
#78983=CARTESIAN_POINT('Ctrl Pts',(87.6569750735685,57.7080644655545,13.7344000444749));
#78984=CARTESIAN_POINT('Ctrl Pts',(87.720202066041,57.71281060814,13.745348503797));
#78985=CARTESIAN_POINT('Ctrl Pts',(87.7813018220297,57.7173970694364,13.7559286083832));
#78986=CARTESIAN_POINT('Ctrl Pts',(87.842939424396,57.7219835307328,13.763162982944));
#78987=CARTESIAN_POINT('Ctrl Pts',(87.9047197787231,57.7265699920292,13.7670230304629));
#78988=CARTESIAN_POINT('Ctrl Pts',(87.9697265311326,57.7313959752592,13.7710846639075));
#78989=CARTESIAN_POINT('Ctrl Pts',(88.0348907105068,57.7362219584893,13.7714098521451));
#78990=CARTESIAN_POINT('Ctrl Pts',(88.0997540577899,57.7410479417194,13.7680274829819));
#78991=CARTESIAN_POINT('Ctrl Pts',(88.164617405073,57.7458739249494,13.7646451138188));
#78992=CARTESIAN_POINT('Ctrl Pts',(88.2291792845965,57.7506999081795,13.7575553349039));
#78993=CARTESIAN_POINT('Ctrl Pts',(88.292993067447,57.7555258914096,13.7468494119081));
#78994=CARTESIAN_POINT('Ctrl Pts',(88.3537819707718,57.7601231150016,13.7366509674824));
#78995=CARTESIAN_POINT('Ctrl Pts',(88.4141416957318,57.7647203385937,13.7231296364321));
#78996=CARTESIAN_POINT('Ctrl Pts',(88.4736814457111,57.7693175621858,13.7063355496345));
#78997=CARTESIAN_POINT('Ctrl Pts',(88.534240678245,57.7739935027569,13.6892539023665));
#78998=CARTESIAN_POINT('Ctrl Pts',(88.5939510524028,57.778669443328,13.6687863615603));
#78999=CARTESIAN_POINT('Ctrl Pts',(88.6524091731495,57.7833453838992,13.6450405657233));
#79000=CARTESIAN_POINT('Ctrl Pts',(88.7097250932282,57.7879299622716,13.6217587338919));
#79001=CARTESIAN_POINT('Ctrl Pts',(88.7658367606141,57.792514540644,13.5953258018849));
#79002=CARTESIAN_POINT('Ctrl Pts',(88.8203789346954,57.7970991190164,13.5658935214446));
#79003=CARTESIAN_POINT('Ctrl Pts',(88.8748877735497,57.8016808953744,13.5364792295014));
#79004=CARTESIAN_POINT('Ctrl Pts',(88.9278285740933,57.8062626717323,13.5040694652369));
#79005=CARTESIAN_POINT('Ctrl Pts',(88.9788587726644,57.8108444480903,13.4688628699116));
#79006=CARTESIAN_POINT('Ctrl Pts',(89.0298765256688,57.8154251070157,13.4336648609928));
#79007=CARTESIAN_POINT('Ctrl Pts',(89.078984182906,57.8200057659412,13.3956716640504));
#79008=CARTESIAN_POINT('Ctrl Pts',(89.1258681095012,57.8245864248666,13.3551252592425));
#79009=CARTESIAN_POINT('Ctrl Pts',(89.1744457932388,57.8293325674521,13.3131140504448));
#79010=CARTESIAN_POINT('Ctrl Pts',(89.2206355167396,57.8340787100377,13.2683619561433));
#79011=CARTESIAN_POINT('Ctrl Pts',(89.2641277917142,57.8388248526232,13.2211820519873));
#79012=CARTESIAN_POINT('Ctrl Pts',(89.3061567936393,57.8434113139196,13.1755894890836));
#79013=CARTESIAN_POINT('Ctrl Pts',(89.3456667041477,57.847997775216,13.1277303502242));
#79014=CARTESIAN_POINT('Ctrl Pts',(89.3824191995577,57.8525842365124,13.0779210516066));
#79015=CARTESIAN_POINT('Ctrl Pts',(89.4210910459005,57.8574102197424,13.0255105276109));
#79016=CARTESIAN_POINT('Ctrl Pts',(89.4567092137119,57.8622362029725,12.9709411026307));
#79017=CARTESIAN_POINT('Ctrl Pts',(89.4890494131044,57.8670621862026,12.9146134385111));
#79018=CARTESIAN_POINT('Ctrl Pts',(89.521389612497,57.8718881694327,12.8582857743915));
#79019=CARTESIAN_POINT('Ctrl Pts',(89.5504516227279,57.8767141526627,12.8002004852554));
#79020=CARTESIAN_POINT('Ctrl Pts',(89.5760698670492,57.8815401358928,12.7407822958958));
#79021=CARTESIAN_POINT('Ctrl Pts',(89.600473763948,57.8861373594849,12.6841806276139));
#79022=CARTESIAN_POINT('Ctrl Pts',(89.6218532476306,57.890734583077,12.6261371915674));
#79023=CARTESIAN_POINT('Ctrl Pts',(89.6400384665074,57.895331806669,12.5670074951927));
#79024=CARTESIAN_POINT('Ctrl Pts',(89.6585350658217,57.9000077472402,12.5068653374971));
#79025=CARTESIAN_POINT('Ctrl Pts',(89.6737266845588,57.9046836878113,12.4455998192272));
#79026=CARTESIAN_POINT('Ctrl Pts',(89.6854849511396,57.9093596283824,12.3836082240857));
#79027=CARTESIAN_POINT('Ctrl Pts',(89.6970134754747,57.9139442067548,12.3228278694097));
#79028=CARTESIAN_POINT('Ctrl Pts',(89.7052415086695,57.9185287851273,12.2613500800785));
#79029=CARTESIAN_POINT('Ctrl Pts',(89.7100984345194,57.9231133634997,12.1995640124199));
#79030=CARTESIAN_POINT('Ctrl Pts',(89.7149523919008,57.9276951398576,12.1378157073297));
#79031=CARTESIAN_POINT('Ctrl Pts',(89.7164392875279,57.9322769162156,12.0757600039394));
#79032=CARTESIAN_POINT('Ctrl Pts',(89.7145401980228,57.9368586925736,12.0137924400075));
#79033=CARTESIAN_POINT('Ctrl Pts',(89.7126415716797,57.941439351499,11.9518399891159));
#79034=CARTESIAN_POINT('Ctrl Pts',(89.7073586151196,57.9460200104245,11.8899761435903));
#79035=CARTESIAN_POINT('Ctrl Pts',(89.6987245058285,57.9506006693499,11.8285956444673));
#79036=CARTESIAN_POINT('Ctrl Pts',(89.6897784754732,57.9553468119354,11.7649976762386));
#79037=CARTESIAN_POINT('Ctrl Pts',(89.6772345425004,57.9600929545209,11.701919231053));
#79038=CARTESIAN_POINT('Ctrl Pts',(89.6611878623258,57.9648390971065,11.6397901284197));
#79039=CARTESIAN_POINT('Ctrl Pts',(89.6456810636508,57.9694255584029,11.579751324386));
#79040=CARTESIAN_POINT('Ctrl Pts',(89.6269037144614,57.9740120196993,11.5205994743882));
#79041=CARTESIAN_POINT('Ctrl Pts',(89.6049923762338,57.9785984809957,11.462706422951));
#79042=CARTESIAN_POINT('Ctrl Pts',(89.5819367470676,57.9834244642257,11.4017899827332));
#79043=CARTESIAN_POINT('Ctrl Pts',(89.5554110680201,57.9882504474558,11.3422680172752));
#79044=CARTESIAN_POINT('Ctrl Pts',(89.5256302890324,57.9930764306859,11.2845462757491));
#79045=CARTESIAN_POINT('Ctrl Pts',(89.4958495100446,57.9979024139159,11.226824534223));
#79046=CARTESIAN_POINT('Ctrl Pts',(89.4628140273237,58.002728397146,11.170903535179));
#79047=CARTESIAN_POINT('Ctrl Pts',(89.4267908525366,58.0075543803761,11.1171527533508));
#79048=CARTESIAN_POINT('Ctrl Pts',(89.3924752361952,58.0121516039682,11.0659498480499));
#79049=CARTESIAN_POINT('Ctrl Pts',(89.3553079222439,58.0167488275602,11.0165058032694));
#79050=CARTESIAN_POINT('Ctrl Pts',(89.3154954527141,58.0213460511523,10.9691561417193));
#79051=CARTESIAN_POINT('Ctrl Pts',(89.2750012853581,58.0260219917234,10.9209957251034));
#79052=CARTESIAN_POINT('Ctrl Pts',(89.231770741624,58.0306979322946,10.8750025832539));
#79053=CARTESIAN_POINT('Ctrl Pts',(89.1860679593757,58.0353738728657,10.8315000500411));
#79054=CARTESIAN_POINT('Ctrl Pts',(89.1412581539756,58.0399584512381,10.788847503483));
#79055=CARTESIAN_POINT('Ctrl Pts',(89.0940722366443,58.0445430296105,10.748589481712));
#79056=CARTESIAN_POINT('Ctrl Pts',(89.0447988437096,58.0491276079829,10.7109963888075));
#79057=CARTESIAN_POINT('Ctrl Pts',(88.9955555658145,58.0537093843409,10.6734262721466));
#79058=CARTESIAN_POINT('Ctrl Pts',(88.9442277459688,58.0582911606988,10.6385181628915));
#79059=CARTESIAN_POINT('Ctrl Pts',(88.8911374198007,58.0628729370568,10.6065024981637));
#79060=CARTESIAN_POINT('Ctrl Pts',(88.8380600416362,58.0674535959822,10.574494641618));
#79061=CARTESIAN_POINT('Ctrl Pts',(88.7832214461921,58.0720342549077,10.5453780919779));
#79062=CARTESIAN_POINT('Ctrl Pts',(88.7269712591976,58.0766149138331,10.519339083185));
#79063=CARTESIAN_POINT('Ctrl Pts',(88.668688943862,58.0813610564187,10.4923593733817));
#79064=CARTESIAN_POINT('Ctrl Pts',(88.6088915929045,58.0861071990042,10.4686841263943));
#79065=CARTESIAN_POINT('Ctrl Pts',(88.5479919189739,58.0908533415897,10.4484665337135));
#79066=CARTESIAN_POINT('Ctrl Pts',(88.4891411802082,58.0954398028861,10.4289291505301));
#79067=CARTESIAN_POINT('Ctrl Pts',(88.429261647752,58.1000262641824,10.4126205088464));
#79068=CARTESIAN_POINT('Ctrl Pts',(88.3687397868389,58.1046127254788,10.3996275684852));
#79069=CARTESIAN_POINT('Ctrl Pts',(88.3050572510133,58.1094387087089,10.3859560888323));
#79070=CARTESIAN_POINT('Ctrl Pts',(88.2406640921925,58.114264691939,10.3759562329338));
#79071=CARTESIAN_POINT('Ctrl Pts',(88.1760177774279,58.119090675169,10.3696674946424));
#79072=CARTESIAN_POINT('Ctrl Pts',(88.1113714626634,58.1239166583991,10.363378756351));
#79073=CARTESIAN_POINT('Ctrl Pts',(88.0464726425025,58.1287426416292,10.3608010840659));
#79074=CARTESIAN_POINT('Ctrl Pts',(87.981776547289,58.1335686248593,10.3619105582712));
#79075=CARTESIAN_POINT('Ctrl Pts',(87.9201471546758,58.1381658484513,10.3629674415524));
#79076=CARTESIAN_POINT('Ctrl Pts',(87.8584486607663,58.1427630720434,10.3673741001395));
#79077=CARTESIAN_POINT('Ctrl Pts',(87.7970749734348,58.1473602956355,10.3751390008019));
#79078=CARTESIAN_POINT('Ctrl Pts',(87.7346504015503,58.1520362362066,10.3830368576956));
#79079=CARTESIAN_POINT('Ctrl Pts',(87.6725623959176,58.1567121767777,10.3944091294685));
#79080=CARTESIAN_POINT('Ctrl Pts',(87.6112258642168,58.1613881173488,10.4092092842007));
#79081=CARTESIAN_POINT('Ctrl Pts',(87.5510877738377,58.1659726957213,10.4237202618877));
#79082=CARTESIAN_POINT('Ctrl Pts',(87.491672574254,58.1705572740937,10.4415262487952));
#79083=CARTESIAN_POINT('Ctrl Pts',(87.433363993645,58.1751418524661,10.4625314222716));
#79084=CARTESIAN_POINT('Ctrl Pts',(87.3750910502248,58.179723628824,10.4835237577519));
#79085=CARTESIAN_POINT('Ctrl Pts',(87.3179238626078,58.184305405182,10.5077112305808));
#79086=CARTESIAN_POINT('Ctrl Pts',(87.2622306976248,58.18888718154,10.5349482806187));
#79087=CARTESIAN_POINT('Ctrl Pts',(87.206551115442,58.1934678404654,10.5621786879131));
#79088=CARTESIAN_POINT('Ctrl Pts',(87.1523452993283,58.1980484993908,10.5924569724198));
#79089=CARTESIAN_POINT('Ctrl Pts',(87.0999593449239,58.2026291583163,10.6255904192215));
#79090=CARTESIAN_POINT('Ctrl Pts',(87.0456808637864,58.2073753009018,10.6599208650002));
#79091=CARTESIAN_POINT('Ctrl Pts',(86.9933567783718,58.2121214434873,10.6973164608235));
#79092=CARTESIAN_POINT('Ctrl Pts',(86.9433396429249,58.2168675860728,10.7375135689326));
#79093=CARTESIAN_POINT('Ctrl Pts',(86.8950053057762,58.2214540473692,10.776358268022));
#79094=CARTESIAN_POINT('Ctrl Pts',(86.8488254862918,58.2260405086656,10.8178185438669));
#79095=CARTESIAN_POINT('Ctrl Pts',(86.8050828595243,58.230626969962,10.8616168857432));
#79096=CARTESIAN_POINT('Ctrl Pts',(86.7590558313697,58.2354529531921,10.9077025386552));
#79097=CARTESIAN_POINT('Ctrl Pts',(86.7157279710292,58.2402789364222,10.9563766851729));
#79098=CARTESIAN_POINT('Ctrl Pts',(86.6753805876875,58.2451049196523,11.0072764189582));
#79099=CARTESIAN_POINT('Ctrl Pts',(86.6350332043458,58.2499309028823,11.0581761527434));
#79100=CARTESIAN_POINT('Ctrl Pts',(86.5976666075079,58.2547568861124,11.1113008992694));
#79101=CARTESIAN_POINT('Ctrl Pts',(86.5635076182577,58.2595828693425,11.1662552359708));
#79102=CARTESIAN_POINT('Ctrl Pts',(86.5300585882811,58.2643085495008,11.2200674036025));
#79103=CARTESIAN_POINT('Ctrl Pts',(86.4995535605494,58.2690342296592,11.2758443580691));
#79104=CARTESIAN_POINT('Ctrl Pts',(86.4722214614649,58.2737599098175,11.3332412095758));
#79105=CARTESIAN_POINT('Ctrl Pts',(86.4449541705362,58.2784743847401,11.3905019652753));
#79106=CARTESIAN_POINT('Ctrl Pts',(86.4208450455069,58.2831888596626,11.4493745572213));
#79107=CARTESIAN_POINT('Ctrl Pts',(86.4000781682881,58.2879033345851,11.5094879267131));
#79108=CARTESIAN_POINT('Ctrl Pts',(86.3793403262532,58.2926112179704,11.5695172487714));
#79109=CARTESIAN_POINT('Ctrl Pts',(86.3619356072016,58.2973191013556,11.6307834624679));
#79110=CARTESIAN_POINT('Ctrl Pts',(86.3480005576707,58.3020269847408,11.6928945317842));
#79111=CARTESIAN_POINT('Ctrl Pts',(86.3340839774588,58.3067286283635,11.7549232799614));
#79112=CARTESIAN_POINT('Ctrl Pts',(86.3236280275323,58.3114302719862,11.8177942005056));
#79113=CARTESIAN_POINT('Ctrl Pts',(86.3167192903354,58.3161319156089,11.8811008046035));
#79114=CARTESIAN_POINT('Ctrl Pts',(86.310004973963,58.3207012488826,11.9426258787601));
#79115=CARTESIAN_POINT('Ctrl Pts',(86.3066408975656,58.3252705821562,12.0045620015264));
#79116=CARTESIAN_POINT('Ctrl Pts',(86.3066600816785,58.3298399154298,12.0665276512002));
#79117=CARTESIAN_POINT('',(86.3066604718792,59.1235899153792,12.0672682606086));
#79118=CARTESIAN_POINT('Ctrl Pts',(86.3066600816788,58.3298399155007,12.0665276521619));
#79119=CARTESIAN_POINT('Ctrl Pts',(86.3066808163434,58.3347785551241,12.1335015396935));
#79120=CARTESIAN_POINT('Ctrl Pts',(86.3106535093132,58.3397171947475,12.2003619829515));
#79121=CARTESIAN_POINT('Ctrl Pts',(86.3185129173098,58.3446558343709,12.2666547047214));
#79122=CARTESIAN_POINT('Ctrl Pts',(86.3263921235412,58.3496069146701,12.3331144211136));
#79123=CARTESIAN_POINT('Ctrl Pts',(86.3381775155799,58.3545579949693,12.3990031909576));
#79124=CARTESIAN_POINT('Ctrl Pts',(86.3537529409633,58.3595090752684,12.4638781483247));
#79125=CARTESIAN_POINT('Ctrl Pts',(86.3693917803471,58.3644803134638,12.5290172384823));
#79126=CARTESIAN_POINT('Ctrl Pts',(86.388851417852,58.3694515516592,12.5931338941111));
#79127=CARTESIAN_POINT('Ctrl Pts',(86.4119657193583,58.3744227898545,12.6558001398209));
#79128=CARTESIAN_POINT('Ctrl Pts',(86.4292844558749,58.3781475645116,12.7027537627818));
#79129=CARTESIAN_POINT('Ctrl Pts',(86.4486538909255,58.3818723391686,12.7488935214905));
#79130=CARTESIAN_POINT('Ctrl Pts',(86.4699872979162,58.3855971138257,12.7940485475684));
#79131=CARTESIAN_POINT('Ctrl Pts',(86.4963176000006,58.3901943374178,12.8497801743908));
#79132=CARTESIAN_POINT('Ctrl Pts',(86.5257292004784,58.3947915610099,12.9041959859528));
#79133=CARTESIAN_POINT('Ctrl Pts',(86.5580676803332,58.3993887846019,12.9569335048519));
#79134=CARTESIAN_POINT('Ctrl Pts',(86.590959882971,58.4040647251731,13.0105740335975));
#79135=CARTESIAN_POINT('Ctrl Pts',(86.6268800000254,58.4087406657442,13.0624777348097));
#79136=CARTESIAN_POINT('Ctrl Pts',(86.6656148451287,58.4134166063153,13.1122856305292));
#79137=CARTESIAN_POINT('Ctrl Pts',(86.7035928584113,58.4180011846877,13.1611203404698));
#79138=CARTESIAN_POINT('Ctrl Pts',(86.7442762687742,58.4225857630601,13.2079399862667));
#79139=CARTESIAN_POINT('Ctrl Pts',(86.7874198018873,58.4271703414326,13.2524342941716));
#79140=CARTESIAN_POINT('Ctrl Pts',(86.8305369664244,58.4317521177905,13.2969014079305));
#79141=CARTESIAN_POINT('Ctrl Pts',(86.8761109186961,58.4363338941485,13.3390456371465));
#79142=CARTESIAN_POINT('Ctrl Pts',(86.9238574195489,58.4409156705064,13.3785912712532));
#79143=CARTESIAN_POINT('Ctrl Pts',(86.971592275684,58.4454963294319,13.4181272607213));
#79144=CARTESIAN_POINT('Ctrl Pts',(87.0214982366928,58.4500769883573,13.4550655886343));
#79145=CARTESIAN_POINT('Ctrl Pts',(87.0732572142,58.4546576472828,13.4891701596366));
#79146=CARTESIAN_POINT('Ctrl Pts',(87.1268860678927,58.4594037898683,13.5245068130372));
#79147=CARTESIAN_POINT('Ctrl Pts',(87.1825039376427,58.4641499324538,13.5568006679624));
#79148=CARTESIAN_POINT('Ctrl Pts',(87.2397254403287,58.4688960750393,13.5858389352836));
#79149=CARTESIAN_POINT('Ctrl Pts',(87.2950217578459,58.4734825363357,13.6139002264865));
#79150=CARTESIAN_POINT('Ctrl Pts',(87.3518149960678,58.4780689976321,13.6389213833942));
#79151=CARTESIAN_POINT('Ctrl Pts',(87.4097358913649,58.4826554589285,13.6607590122859));
#79152=CARTESIAN_POINT('Ctrl Pts',(87.4706816295519,58.4874814421586,13.6837370827429));
#79153=CARTESIAN_POINT('Ctrl Pts',(87.5328754240038,58.4923074253887,13.7031897934175));
#79154=CARTESIAN_POINT('Ctrl Pts',(87.5958707470284,58.4971334086187,13.7190101448349));
#79155=CARTESIAN_POINT('Ctrl Pts',(87.658866070053,58.5019593918488,13.7348304962524));
#79156=CARTESIAN_POINT('Ctrl Pts',(87.7226622706541,58.5067853750789,13.7470184428211));
#79157=CARTESIAN_POINT('Ctrl Pts',(87.7868056147989,58.511611358309,13.7555300273284));
#79158=CARTESIAN_POINT('Ctrl Pts',(87.847908457664,58.5162085819011,13.7636381485625));
#79159=CARTESIAN_POINT('Ctrl Pts',(87.9095771487089,58.5208058054932,13.7684439092126));
#79160=CARTESIAN_POINT('Ctrl Pts',(87.9714234063106,58.5254030290852,13.7698804326689));
#79161=CARTESIAN_POINT('Ctrl Pts',(88.0343286401543,58.5300789696564,13.7713415533162));
#79162=CARTESIAN_POINT('Ctrl Pts',(88.0974170654511,58.5347549102275,13.7693168058526));
#79163=CARTESIAN_POINT('Ctrl Pts',(88.1602714651954,58.5394308507986,13.7637905834579));
#79164=CARTESIAN_POINT('Ctrl Pts',(88.2218977663205,58.544015429171,13.7583723367359));
#79165=CARTESIAN_POINT('Ctrl Pts',(88.2832985734276,58.5486000075434,13.7495882603519));
#79166=CARTESIAN_POINT('Ctrl Pts',(88.3440801824787,58.5531845859159,13.7374761223661));
#79167=CARTESIAN_POINT('Ctrl Pts',(88.404824642869,58.5577663622738,13.725371387108));
#79168=CARTESIAN_POINT('Ctrl Pts',(88.4649501574056,58.5623481386318,13.7099427227589));
#79169=CARTESIAN_POINT('Ctrl Pts',(88.5240709248393,58.5669299149897,13.691279379579));
#79170=CARTESIAN_POINT('Ctrl Pts',(88.5831772735275,58.5715105739152,13.6726205881328));
#79171=CARTESIAN_POINT('Ctrl Pts',(88.6412788763462,58.5760912328406,13.6507288371036));
#79172=CARTESIAN_POINT('Ctrl Pts',(88.6980048538477,58.5806718917661,13.6257433014409));
#79173=CARTESIAN_POINT('Ctrl Pts',(88.7567801483862,58.5854180343516,13.5998551231766));
#79174=CARTESIAN_POINT('Ctrl Pts',(88.8140779633559,58.5901641769371,13.570645520284));
#79175=CARTESIAN_POINT('Ctrl Pts',(88.8695104987765,58.5949103195226,13.5383228447221));
#79176=CARTESIAN_POINT('Ctrl Pts',(88.9230780378227,58.599496780819,13.5070876473402));
#79177=CARTESIAN_POINT('Ctrl Pts',(88.9749034236237,58.6040832421154,13.4729458901017));
#79178=CARTESIAN_POINT('Ctrl Pts',(89.024665899943,58.6086697034118,13.436130022623));
#79179=CARTESIAN_POINT('Ctrl Pts',(89.077027156407,58.6134956866419,13.3973914946881));
#79180=CARTESIAN_POINT('Ctrl Pts',(89.1271036276571,58.6183216698719,13.3556922974774));
#79181=CARTESIAN_POINT('Ctrl Pts',(89.1745632251013,58.623147653102,13.3113495319756));
#79182=CARTESIAN_POINT('Ctrl Pts',(89.2220228225455,58.627973636332,13.2670067664738));
#79183=CARTESIAN_POINT('Ctrl Pts',(89.2668651547817,58.6327996195621,13.2200209548678));
#79184=CARTESIAN_POINT('Ctrl Pts',(89.308807187647,58.6376256027922,13.1707494463867));
#79185=CARTESIAN_POINT('Ctrl Pts',(89.3487610983417,58.6422228263842,13.1238134894205));
#79186=CARTESIAN_POINT('Ctrl Pts',(89.3862475413485,58.6468200499763,13.0746109551229));
#79187=CARTESIAN_POINT('Ctrl Pts',(89.4209997287398,58.6514172735684,13.0234317733154));
#79188=CARTESIAN_POINT('Ctrl Pts',(89.4563469681558,58.6560932141395,12.9713762646333));
#79189=CARTESIAN_POINT('Ctrl Pts',(89.4888650187903,58.6607691547106,12.9172761223816));
#79190=CARTESIAN_POINT('Ctrl Pts',(89.5183144710356,58.6654450952818,12.8614733942796));
#79191=CARTESIAN_POINT('Ctrl Pts',(89.5471885167574,58.6700296736542,12.806760983699));
#79192=CARTESIAN_POINT('Ctrl Pts',(89.573112550046,58.6746142520266,12.7504123935714));
#79193=CARTESIAN_POINT('Ctrl Pts',(89.5959047560652,58.679198830399,12.6927788683434));
#79194=CARTESIAN_POINT('Ctrl Pts',(89.618683031885,58.683780606757,12.6351805677223));
#79195=CARTESIAN_POINT('Ctrl Pts',(89.6383330890393,58.6883623831149,12.5762993615891));
#79196=CARTESIAN_POINT('Ctrl Pts',(89.654720650441,58.6929441594729,12.5165077789716));
#79197=CARTESIAN_POINT('Ctrl Pts',(89.6711042151408,58.6975248183983,12.4567307787023));
#79198=CARTESIAN_POINT('Ctrl Pts',(89.6842267291334,58.7021054773238,12.3960443334303));
#79199=CARTESIAN_POINT('Ctrl Pts',(89.6940039516866,58.7066861362492,12.3348355151524));
#79200=CARTESIAN_POINT('Ctrl Pts',(89.7041343921065,58.7114322788347,12.2714154300149));
#79201=CARTESIAN_POINT('Ctrl Pts',(89.710673050288,58.7161784214203,12.2074350701328));
#79202=CARTESIAN_POINT('Ctrl Pts',(89.7135846248931,58.7209245640058,12.1433332443245));
#79203=CARTESIAN_POINT('Ctrl Pts',(89.7163982412135,58.7255110253022,12.0813880882738));
#79204=CARTESIAN_POINT('Ctrl Pts',(89.7158250532987,58.7300974865985,12.0193300375764));
#79205=CARTESIAN_POINT('Ctrl Pts',(89.7118863692065,58.7346839478949,11.9575546467217));
#79206=CARTESIAN_POINT('Ctrl Pts',(89.7077419924965,58.739509931125,11.8925531169954));
#79207=CARTESIAN_POINT('Ctrl Pts',(89.6998710301739,58.7443359143551,11.8278652203452));
#79208=CARTESIAN_POINT('Ctrl Pts',(89.6883597610478,58.7491618975852,11.76394194661));
#79209=CARTESIAN_POINT('Ctrl Pts',(89.6768484919216,58.7539878808152,11.7000186728747));
#79210=CARTESIAN_POINT('Ctrl Pts',(89.6616971423962,58.7588138640453,11.6368606341129));
#79211=CARTESIAN_POINT('Ctrl Pts',(89.6430524117444,58.7636398472754,11.5748994390969));
#79212=CARTESIAN_POINT('Ctrl Pts',(89.6252914723598,58.7682370708675,11.5158753078596));
#79213=CARTESIAN_POINT('Ctrl Pts',(89.6042879819519,58.7728342944595,11.4576947597245));
#79214=CARTESIAN_POINT('Ctrl Pts',(89.5801408112597,58.7774315180516,11.4007391864545));
#79215=CARTESIAN_POINT('Ctrl Pts',(89.5555801752897,58.7821074586227,11.3428083787678));
#79216=CARTESIAN_POINT('Ctrl Pts',(89.5277672508755,58.7867833991939,11.2861454257539));
#79217=CARTESIAN_POINT('Ctrl Pts',(89.4968595440726,58.791459339765,11.2311369867526));
#79218=CARTESIAN_POINT('Ctrl Pts',(89.4665557363157,58.7960439181374,11.1772033458286));
#79219=CARTESIAN_POINT('Ctrl Pts',(89.4332772563873,58.8006284965098,11.1248606110418));
#79220=CARTESIAN_POINT('Ctrl Pts',(89.3972205760408,58.8052130748822,11.0744520434386));
#79221=CARTESIAN_POINT('Ctrl Pts',(89.3611859329093,58.8097948512402,11.0240742846739));
#79222=CARTESIAN_POINT('Ctrl Pts',(89.3223767517619,58.8143766275981,10.9756287622745));
#79223=CARTESIAN_POINT('Ctrl Pts',(89.2810331703959,58.8189584039561,10.9294303445481));
#79224=CARTESIAN_POINT('Ctrl Pts',(89.2396996721633,58.8235390628815,10.8832431939831));
#79225=CARTESIAN_POINT('Ctrl Pts',(89.1958333400602,58.828119721807,10.8393024393121));
#79226=CARTESIAN_POINT('Ctrl Pts',(89.1497136693969,58.8327003807324,10.79788880033));
#79227=CARTESIAN_POINT('Ctrl Pts',(89.1019278515643,58.8374465233179,10.7549790271307));
#79228=CARTESIAN_POINT('Ctrl Pts',(89.0517231568139,58.8421926659035,10.7147828939027));
#79229=CARTESIAN_POINT('Ctrl Pts',(88.999449090322,58.846938808489,10.6775680674078));
#79230=CARTESIAN_POINT('Ctrl Pts',(88.9489337552998,58.8515252697854,10.6416053127506));
#79231=CARTESIAN_POINT('Ctrl Pts',(88.8964865766668,58.8561117310817,10.6084266501165));
#79232=CARTESIAN_POINT('Ctrl Pts',(88.8424514255881,58.8606981923781,10.5782287264208));
#79233=CARTESIAN_POINT('Ctrl Pts',(88.7855943595217,58.8655241756082,10.5464537557145));
#79234=CARTESIAN_POINT('Ctrl Pts',(88.7269794878156,58.8703501588383,10.5179796826691));
#79235=CARTESIAN_POINT('Ctrl Pts',(88.6670324941007,58.8751761420684,10.4929786389613));
#79236=CARTESIAN_POINT('Ctrl Pts',(88.6070855003858,58.8800021252984,10.4679775952535));
#79237=CARTESIAN_POINT('Ctrl Pts',(88.5458070216668,58.8848281085285,10.4464497226561));
#79238=CARTESIAN_POINT('Ctrl Pts',(88.4836392311151,58.8896540917586,10.4285058800683));
#79239=CARTESIAN_POINT('Ctrl Pts',(88.4244182973144,58.8942513153507,10.4114126054869));
#79240=CARTESIAN_POINT('Ctrl Pts',(88.3641473198731,58.8988485389428,10.3975010250991));
#79241=CARTESIAN_POINT('Ctrl Pts',(88.303200341452,58.9034457625348,10.3868949419243));
#79242=CARTESIAN_POINT('Ctrl Pts',(88.2412097848958,58.908121703106,10.3761072537416));
#79243=CARTESIAN_POINT('Ctrl Pts',(88.1785203426625,58.9127976436771,10.368739564741));
#79244=CARTESIAN_POINT('Ctrl Pts',(88.1155422865393,58.9174735842482,10.3648692742987));
#79245=CARTESIAN_POINT('Ctrl Pts',(88.0537947451307,58.9220581626206,10.3610746046301));
#79246=CARTESIAN_POINT('Ctrl Pts',(87.9917702991426,58.9266427409931,10.3606419255504));
#79247=CARTESIAN_POINT('Ctrl Pts',(87.9298638954832,58.9312273193655,10.3635923613471));
#79248=CARTESIAN_POINT('Ctrl Pts',(87.8679953279395,58.9358090957234,10.3665409938887));
#79249=CARTESIAN_POINT('Ctrl Pts',(87.8062451670857,58.9403908720814,10.3728686171715));
#79250=CARTESIAN_POINT('Ctrl Pts',(87.7450081908972,58.9449726484394,10.3825442705286));
#79251=CARTESIAN_POINT('Ctrl Pts',(87.6837861495685,58.9495533073648,10.3922175641263));
#79252=CARTESIAN_POINT('Ctrl Pts',(87.6230775470304,58.9541339662903,10.4052371874353));
#79253=CARTESIAN_POINT('Ctrl Pts',(87.563269819836,58.9587146252157,10.4215205925977));
#79254=CARTESIAN_POINT('Ctrl Pts',(87.5013014424476,58.9634607678013,10.4383922619221));
#79255=CARTESIAN_POINT('Ctrl Pts',(87.4403008556013,58.9682069103868,10.4587679559189));
#79256=CARTESIAN_POINT('Ctrl Pts',(87.3806825029854,58.9729530529723,10.4824992300105));
#79257=CARTESIAN_POINT('Ctrl Pts',(87.3230699762016,58.9775395142687,10.5054320787766));
#79258=CARTESIAN_POINT('Ctrl Pts',(87.2667485944832,58.9821259755651,10.5314979983285));
#79259=CARTESIAN_POINT('Ctrl Pts',(87.2120700803616,58.9867124368615,10.5605147562641));
#79260=CARTESIAN_POINT('Ctrl Pts',(87.1545360524603,58.9915384200915,10.5910468763755));
#79261=CARTESIAN_POINT('Ctrl Pts',(87.0988217469623,58.9963644033216,10.6248461690274));
#79262=CARTESIAN_POINT('Ctrl Pts',(87.0453026656082,59.0011903865517,10.661648372398));
#79263=CARTESIAN_POINT('Ctrl Pts',(86.9917835842541,59.0060163697817,10.6984505757685));
#79264=CARTESIAN_POINT('Ctrl Pts',(86.9404601916607,59.0108423530118,10.7382552315939));
#79265=CARTESIAN_POINT('Ctrl Pts',(86.8916654569177,59.0156683362419,10.7807509905615));
#79266=CARTESIAN_POINT('Ctrl Pts',(86.8458789933511,59.0201967901109,10.8206268199917));
#79267=CARTESIAN_POINT('Ctrl Pts',(86.8021189271895,59.02472524398,10.8630459958341));
#79268=CARTESIAN_POINT('Ctrl Pts',(86.7606873677575,59.029253697849,10.9077715435827));
#79269=CARTESIAN_POINT('Ctrl Pts',(86.7193124721653,59.0337759583817,10.952435922471));
#79270=CARTESIAN_POINT('Ctrl Pts',(86.6802601326207,59.0382982189143,10.9994000478932));
#79271=CARTESIAN_POINT('Ctrl Pts',(86.6437985928296,59.042820479447,11.0483875257097));
#79272=CARTESIAN_POINT('Ctrl Pts',(86.6073725997099,59.0473383311886,11.0973272452091));
#79273=CARTESIAN_POINT('Ctrl Pts',(86.5735327161805,59.0518561829303,11.1482859914009));
#79274=CARTESIAN_POINT('Ctrl Pts',(86.5425080117181,59.0563740346719,11.2009531134372));
#79275=CARTESIAN_POINT('Ctrl Pts',(86.5115013763062,59.0608892551784,11.253589561696));
#79276=CARTESIAN_POINT('Ctrl Pts',(86.4833069364353,59.065404475685,11.3079319621111));
#79277=CARTESIAN_POINT('Ctrl Pts',(86.4581100863428,59.0699196961915,11.3636412941652));
#79278=CARTESIAN_POINT('Ctrl Pts',(86.432903837136,59.0744366009988,11.4193714073244));
#79279=CARTESIAN_POINT('Ctrl Pts',(86.4106976423061,59.0789535058061,11.4764689979253));
#79280=CARTESIAN_POINT('Ctrl Pts',(86.391629846485,59.0834704106135,11.5345725435163));
#79281=CARTESIAN_POINT('Ctrl Pts',(86.3725597501086,59.0879878603914,11.5926830993781));
#79282=CARTESIAN_POINT('Ctrl Pts',(86.3566289553476,59.0925053101694,11.651799347088));
#79283=CARTESIAN_POINT('Ctrl Pts',(86.3439257959816,59.0970227599473,11.7115448774579));
#79284=CARTESIAN_POINT('Ctrl Pts',(86.3312035786438,59.1015469870495,11.7713800413276));
#79285=CARTESIAN_POINT('Ctrl Pts',(86.3217187612233,59.1060712141517,11.8318458547642));
#79286=CARTESIAN_POINT('Ctrl Pts',(86.3155082094182,59.110595441254,11.89255714581));
#79287=CARTESIAN_POINT('Ctrl Pts',(86.309562232134,59.114926932629,11.9506820868425));
#79288=CARTESIAN_POINT('Ctrl Pts',(86.3066171358679,59.1192584240041,12.0090315885683));
#79289=CARTESIAN_POINT('Ctrl Pts',(86.3066604718792,59.1235899153792,12.0672682606086));
#79290=CARTESIAN_POINT('',(86.306660521223,59.9173399154754,12.0646670776546));
#79291=CARTESIAN_POINT('Ctrl Pts',(86.3066604718797,59.1235899154298,12.0672682612888));
#79292=CARTESIAN_POINT('Ctrl Pts',(86.3067208101713,59.1296208038615,12.1483532367145));
#79293=CARTESIAN_POINT('Ctrl Pts',(86.3125682407869,59.1356516922933,12.2292263611692));
#79294=CARTESIAN_POINT('Ctrl Pts',(86.3241094256459,59.1416825807251,12.3092591740417));
#79295=CARTESIAN_POINT('Ctrl Pts',(86.3329070361332,59.1462798043172,12.3702665595444));
#79296=CARTESIAN_POINT('Ctrl Pts',(86.3450365252776,59.1508770279093,12.4309213061331));
#79297=CARTESIAN_POINT('Ctrl Pts',(86.3604567637294,59.1554742515014,12.490831567567));
#79298=CARTESIAN_POINT('Ctrl Pts',(86.376141038629,59.1601501920726,12.5517676557197));
#79299=CARTESIAN_POINT('Ctrl Pts',(86.3952298350125,59.1648261326437,12.6119329851159));
#79300=CARTESIAN_POINT('Ctrl Pts',(86.4176248208747,59.1695020732149,12.6709217917609));
#79301=CARTESIAN_POINT('Ctrl Pts',(86.4395822359172,59.1740866515873,12.7287580287803));
#79302=CARTESIAN_POINT('Ctrl Pts',(86.46471761521,59.1786712299597,12.7854628065256));
#79303=CARTESIAN_POINT('Ctrl Pts',(86.4928876476361,59.1832558083321,12.8406674907341));
#79304=CARTESIAN_POINT('Ctrl Pts',(86.5210404630291,59.1878375846901,12.8958384348011));
#79305=CARTESIAN_POINT('Ctrl Pts',(86.552224023004,59.1924193610481,12.9495106507903));
#79306=CARTESIAN_POINT('Ctrl Pts',(86.5862476177626,59.197001137406,13.0013370969382));
#79307=CARTESIAN_POINT('Ctrl Pts',(86.6202629146324,59.2015817963315,13.0531509033257));
#79308=CARTESIAN_POINT('Ctrl Pts',(86.6571165920408,59.206162455257,13.1031194081535));
#79309=CARTESIAN_POINT('Ctrl Pts',(86.6965739473985,59.2107431141824,13.1509234940043));
#79310=CARTESIAN_POINT('Ctrl Pts',(86.7374567630855,59.2154892567679,13.2004545792279));
#79311=CARTESIAN_POINT('Ctrl Pts',(86.7811346619707,59.2202353993534,13.2476613758826));
#79312=CARTESIAN_POINT('Ctrl Pts',(86.8273017694101,59.2249815419388,13.292227276853));
#79313=CARTESIAN_POINT('Ctrl Pts',(86.8719156105713,59.2295680032352,13.3352937832333));
#79314=CARTESIAN_POINT('Ctrl Pts',(86.9188533668513,59.2341544645316,13.375893995501));
#79315=CARTESIAN_POINT('Ctrl Pts',(86.9678041871651,59.238740925828,13.4137823754908));
#79316=CARTESIAN_POINT('Ctrl Pts',(87.0193113999516,59.243566909058,13.4536494264976));
#79317=CARTESIAN_POINT('Ctrl Pts',(87.0730471767966,59.2483928922881,13.4905132611832));
#79318=CARTESIAN_POINT('Ctrl Pts',(87.1286161204782,59.2532188755181,13.5241404338266));
#79319=CARTESIAN_POINT('Ctrl Pts',(87.1841850641597,59.2580448587481,13.55776760647));
#79320=CARTESIAN_POINT('Ctrl Pts',(87.2415865657944,59.2628708419781,13.5881578822621));
#79321=CARTESIAN_POINT('Ctrl Pts',(87.3003998211841,59.2676968252082,13.6151359596455));
#79322=CARTESIAN_POINT('Ctrl Pts',(87.3564252303735,59.2722940488002,13.6408352312558));
#79323=CARTESIAN_POINT('Ctrl Pts',(87.4139615870079,59.2768912723923,13.6635440501566));
#79324=CARTESIAN_POINT('Ctrl Pts',(87.4726573842561,59.2814884959844,13.683084433069));
#79325=CARTESIAN_POINT('Ctrl Pts',(87.5323582132914,59.2861644365555,13.7029594005151));
#79326=CARTESIAN_POINT('Ctrl Pts',(87.5932581198193,59.2908403771266,13.7195560987896));
#79327=CARTESIAN_POINT('Ctrl Pts',(87.6549628777595,59.2955163176978,13.7327370528031));
#79328=CARTESIAN_POINT('Ctrl Pts',(87.7154619996849,59.3001008960702,13.7456604669866));
#79329=CARTESIAN_POINT('Ctrl Pts',(87.7767342825985,59.3046854744426,13.7553003040122));
#79330=CARTESIAN_POINT('Ctrl Pts',(87.8383922972793,59.309270052815,13.7615770158154));
#79331=CARTESIAN_POINT('Ctrl Pts',(87.9000126276553,59.313851829173,13.7678498914017));
#79332=CARTESIAN_POINT('Ctrl Pts',(87.9620177169563,59.318433605531,13.7707636660454));
#79333=CARTESIAN_POINT('Ctrl Pts',(88.0240125672906,59.3230153818889,13.7702903240623));
#79334=CARTESIAN_POINT('Ctrl Pts',(88.0859922979299,59.3275960408144,13.7698170975209));
#79335=CARTESIAN_POINT('Ctrl Pts',(88.1479612857555,59.3321766997399,13.7659583981145));
#79336=CARTESIAN_POINT('Ctrl Pts',(88.2095241310749,59.3367573586653,13.7587383155647));
#79337=CARTESIAN_POINT('Ctrl Pts',(88.2733110330491,59.3415035012509,13.7512573959377));
#79338=CARTESIAN_POINT('Ctrl Pts',(88.3366613006586,59.3462496438364,13.7401675764964));
#79339=CARTESIAN_POINT('Ctrl Pts',(88.3991430395344,59.3509957864219,13.7255541016975));
#79340=CARTESIAN_POINT('Ctrl Pts',(88.4595226155632,59.3555822477183,13.711432289012));
#79341=CARTESIAN_POINT('Ctrl Pts',(88.5190906943802,59.3601687090147,13.6940203911597));
#79342=CARTESIAN_POINT('Ctrl Pts',(88.5774723889305,59.3647551703111,13.6734463811211));
#79343=CARTESIAN_POINT('Ctrl Pts',(88.6389029910079,59.3695811535412,13.6517979203569));
#79344=CARTESIAN_POINT('Ctrl Pts',(88.6990192978616,59.3744071367713,13.6266482549287));
#79345=CARTESIAN_POINT('Ctrl Pts',(88.7574107238353,59.3792331200013,13.5982029457431));
#79346=CARTESIAN_POINT('Ctrl Pts',(88.8158021498089,59.3840591032314,13.5697576365574));
#79347=CARTESIAN_POINT('Ctrl Pts',(88.8724681673767,59.3888850864615,13.5380170677901));
#79348=CARTESIAN_POINT('Ctrl Pts',(88.9270332583123,59.3937110696915,13.5032396826089));
#79349=CARTESIAN_POINT('Ctrl Pts',(88.9790118731136,59.3983082932836,13.4701108033724));
#79350=CARTESIAN_POINT('Ctrl Pts',(89.0292976813082,59.4029055168757,13.4340905273487));
#79351=CARTESIAN_POINT('Ctrl Pts',(89.077550498505,59.4075027404678,13.3953776249579));
#79352=CARTESIAN_POINT('Ctrl Pts',(89.1266295352504,59.4121786810389,13.3560018523225));
#79353=CARTESIAN_POINT('Ctrl Pts',(89.1736048068095,59.41685462161,13.3138405801563));
#79354=CARTESIAN_POINT('Ctrl Pts',(89.2181469897109,59.4215305621812,13.269150439817));
#79355=CARTESIAN_POINT('Ctrl Pts',(89.2618188724656,59.4261151405536,13.2253334905331));
#79356=CARTESIAN_POINT('Ctrl Pts',(89.3031515140972,59.430699718926,13.1790859841457));
#79357=CARTESIAN_POINT('Ctrl Pts',(89.3418679434624,59.4352842972984,13.1306902613737));
#79358=CARTESIAN_POINT('Ctrl Pts',(89.3805607100203,59.4398660736563,13.0823241172246));
#79359=CARTESIAN_POINT('Ctrl Pts',(89.4166401175261,59.4444478500143,13.0318127567608));
#79360=CARTESIAN_POINT('Ctrl Pts',(89.4498683830425,59.4490296263722,12.9794728304009));
#79361=CARTESIAN_POINT('Ctrl Pts',(89.48308854464,59.4536102852977,12.9271456690323));
#79362=CARTESIAN_POINT('Ctrl Pts',(89.5134586719212,59.4581909442231,12.8729912566345));
#79363=CARTESIAN_POINT('Ctrl Pts',(89.5407845388671,59.4627716031486,12.8173548430955));
#79364=CARTESIAN_POINT('Ctrl Pts',(89.5690975966409,59.4675177457341,12.7597084747671));
#79365=CARTESIAN_POINT('Ctrl Pts',(89.5941419113378,59.4722638883196,12.7004714694172));
#79366=CARTESIAN_POINT('Ctrl Pts',(89.6157548396587,59.4770100309051,12.6400529071366));
#79367=CARTESIAN_POINT('Ctrl Pts',(89.636640613202,59.4815964922015,12.5816670932909));
#79368=CARTESIAN_POINT('Ctrl Pts',(89.6543221614587,59.4861829534979,12.5221784973082));
#79369=CARTESIAN_POINT('Ctrl Pts',(89.668703658964,59.4907694147943,12.4619714821262));
#79370=CARTESIAN_POINT('Ctrl Pts',(89.6838362113392,59.4955953980243,12.3986202344377));
#79371=CARTESIAN_POINT('Ctrl Pts',(89.6953144554487,59.5004213812544,12.3344741049122));
#79372=CARTESIAN_POINT('Ctrl Pts',(89.7030883862101,59.5052473644845,12.269989531234));
#79373=CARTESIAN_POINT('Ctrl Pts',(89.7108623169714,59.5100733477146,12.2055049575557));
#79374=CARTESIAN_POINT('Ctrl Pts',(89.7149319710093,59.5148993309447,12.1406825912867));
#79375=CARTESIAN_POINT('Ctrl Pts',(89.715310791279,59.5197253141747,12.0759780924933));
#79376=CARTESIAN_POINT('Ctrl Pts',(89.7156716548375,59.5243225377668,12.014340694644));
#79377=CARTESIAN_POINT('Ctrl Pts',(89.7126852185318,59.5289197613589,11.9525571694224));
#79378=CARTESIAN_POINT('Ctrl Pts',(89.7063339580072,59.533516984951,11.8910211257674));
#79379=CARTESIAN_POINT('Ctrl Pts',(89.6998739466177,59.5381929255221,11.8284314175772));
#79380=CARTESIAN_POINT('Ctrl Pts',(89.689932698466,59.5428688660932,11.7660982755586));
#79381=CARTESIAN_POINT('Ctrl Pts',(89.6765471903453,59.5475448066643,11.704437567863));
#79382=CARTESIAN_POINT('Ctrl Pts',(89.6634232187934,59.5521293850367,11.6439816354941));
#79383=CARTESIAN_POINT('Ctrl Pts',(89.64698848327,59.5567139634091,11.5841726179499));
#79384=CARTESIAN_POINT('Ctrl Pts',(89.627329955385,59.5612985417816,11.5253963458087));
#79385=CARTESIAN_POINT('Ctrl Pts',(89.6076834424499,59.5658803181395,11.4666559967013));
#79386=CARTESIAN_POINT('Ctrl Pts',(89.5848172051553,59.5704620944975,11.4089476231853));
#79387=CARTESIAN_POINT('Ctrl Pts',(89.5588682950506,59.5750438708554,11.3526427425356));
#79388=CARTESIAN_POINT('Ctrl Pts',(89.5329257135297,59.5796245297809,11.2963515938752));
#79389=CARTESIAN_POINT('Ctrl Pts',(89.5039021646468,59.5842051887063,11.2414637206838));
#79390=CARTESIAN_POINT('Ctrl Pts',(89.4719823521895,59.5887858476318,11.188329559464));
#79391=CARTESIAN_POINT('Ctrl Pts',(89.4389093852451,59.5935319902173,11.1332758413385));
#79392=CARTESIAN_POINT('Ctrl Pts',(89.402727128262,59.5982781328028,11.0801055039213));
#79393=CARTESIAN_POINT('Ctrl Pts',(89.3636910405609,59.6030242753883,11.0291770718265));
#79394=CARTESIAN_POINT('Ctrl Pts',(89.325968300003,59.6076107366847,10.9799620980914));
#79395=CARTESIAN_POINT('Ctrl Pts',(89.285581120993,59.6121971979811,10.9328409141891));
#79396=CARTESIAN_POINT('Ctrl Pts',(89.2428004393584,59.6167836592775,10.8881025031029));
#79397=CARTESIAN_POINT('Ctrl Pts',(89.1977855926613,59.6216096425075,10.841027687098));
#79398=CARTESIAN_POINT('Ctrl Pts',(89.1501208566216,59.6264356257376,10.796591789907));
#79399=CARTESIAN_POINT('Ctrl Pts',(89.1001625715059,59.6312616089677,10.7550843930937));
#79400=CARTESIAN_POINT('Ctrl Pts',(89.0502042863902,59.6360875921977,10.7135769962803));
#79401=CARTESIAN_POINT('Ctrl Pts',(88.9979530194548,59.6409135754278,10.6749984224819));
#79402=CARTESIAN_POINT('Ctrl Pts',(88.9437988718105,59.6457395586579,10.6395845274434));
#79403=CARTESIAN_POINT('Ctrl Pts',(88.8922117209045,59.65033678225,10.6058493099763));
#79404=CARTESIAN_POINT('Ctrl Pts',(88.8386862339935,59.6549340058421,10.5748469706846));
#79405=CARTESIAN_POINT('Ctrl Pts',(88.7835435850918,59.6595312294341,10.5468057251511));
#79406=CARTESIAN_POINT('Ctrl Pts',(88.7274567439725,59.6642071700053,10.5182843371811));
#79407=CARTESIAN_POINT('Ctrl Pts',(88.6696972310118,59.6688831105764,10.4928267710902));
#79408=CARTESIAN_POINT('Ctrl Pts',(88.6106344820152,59.6735590511475,10.4706275282623));
#79409=CARTESIAN_POINT('Ctrl Pts',(88.5527257473881,59.6781436295199,10.448862031673));
#79410=CARTESIAN_POINT('Ctrl Pts',(88.4935647453181,59.6827282078923,10.4302288637889));
#79411=CARTESIAN_POINT('Ctrl Pts',(88.433522793536,59.6873127862648,10.4148642319474));
#79412=CARTESIAN_POINT('Ctrl Pts',(88.3735175383491,59.6918945626227,10.3995089907014));
#79413=CARTESIAN_POINT('Ctrl Pts',(88.3126328931943,59.6964763389807,10.3874184503386));
#79414=CARTESIAN_POINT('Ctrl Pts',(88.2512553141907,59.7010581153387,10.3786789814611));
#79415=CARTESIAN_POINT('Ctrl Pts',(88.1898927043381,59.7056387742641,10.3699416440204));
#79416=CARTESIAN_POINT('Ctrl Pts',(88.1280379030294,59.7102194331896,10.3645538273662));
#79417=CARTESIAN_POINT('Ctrl Pts',(88.0660855024955,59.714800092115,10.3625504342615));
#79418=CARTESIAN_POINT('Ctrl Pts',(88.0018949719991,59.7195462347006,10.3604746653635));
#79419=CARTESIAN_POINT('Ctrl Pts',(87.9376002344375,59.7242923772861,10.3620326202201));
#79420=CARTESIAN_POINT('Ctrl Pts',(87.873641054749,59.7290385198716,10.3672041453549));
#79421=CARTESIAN_POINT('Ctrl Pts',(87.81183374557,59.733624981168,10.3722016774447));
#79422=CARTESIAN_POINT('Ctrl Pts',(87.7503402854361,59.7382114424644,10.3805733297022));
#79423=CARTESIAN_POINT('Ctrl Pts',(87.6895504103278,59.7427979037608,10.3922482272154));
#79424=CARTESIAN_POINT('Ctrl Pts',(87.625585863617,59.7476238869908,10.404532830959));
#79425=CARTESIAN_POINT('Ctrl Pts',(87.5624010317684,59.7524498702209,10.4204750091404));
#79426=CARTESIAN_POINT('Ctrl Pts',(87.5004324769044,59.757275853451,10.4399324614396));
#79427=CARTESIAN_POINT('Ctrl Pts',(87.4384639220403,59.762101836681,10.4593899137387));
#79428=CARTESIAN_POINT('Ctrl Pts',(87.3777122228942,59.7669278199111,10.4823623385896));
#79429=CARTESIAN_POINT('Ctrl Pts',(87.3185871172308,59.7717538031412,10.5086499316547));
#79430=CARTESIAN_POINT('Ctrl Pts',(87.2622646399899,59.7763510267333,10.5336914490525));
#79431=CARTESIAN_POINT('Ctrl Pts',(87.2071867605101,59.7809482503253,10.5618437133064));
#79432=CARTESIAN_POINT('Ctrl Pts',(87.1537194119223,59.7855454739174,10.5929606831774));
#79433=CARTESIAN_POINT('Ctrl Pts',(87.0993365568175,59.7902214144885,10.6246104602561));
#79434=CARTESIAN_POINT('Ctrl Pts',(87.0466204281995,59.7948973550596,10.6593272975581));
#79435=CARTESIAN_POINT('Ctrl Pts',(86.9959348123226,59.7995732956308,10.6969063215523));
#79436=CARTESIAN_POINT('Ctrl Pts',(86.9462395318102,59.8041578740032,10.7337510970663));
#79437=CARTESIAN_POINT('Ctrl Pts',(86.8984965586452,59.8087424523756,10.7733469001858));
#79438=CARTESIAN_POINT('Ctrl Pts',(86.8530217257735,59.813327030748,10.8154556577156));
#79439=CARTESIAN_POINT('Ctrl Pts',(86.8075746863276,59.817908807106,10.8575386791063));
#79440=CARTESIAN_POINT('Ctrl Pts',(86.7643934111796,59.8224905834639,10.9021312643472));
#79441=CARTESIAN_POINT('Ctrl Pts',(86.7237600754219,59.8270723598219,10.9489555907789));
#79442=CARTESIAN_POINT('Ctrl Pts',(86.6831366495782,59.8316530187473,10.9957684973987));
#79443=CARTESIAN_POINT('Ctrl Pts',(86.6450602630228,59.8362336776727,11.0448116804123));
#79444=CARTESIAN_POINT('Ctrl Pts',(86.6097742646436,59.8408143365982,11.0957725657482));
#79445=CARTESIAN_POINT('Ctrl Pts',(86.5732135029048,59.8455604791837,11.1485744949083));
#79446=CARTESIAN_POINT('Ctrl Pts',(86.5396489876384,59.8503066217692,11.2034348978998));
#79447=CARTESIAN_POINT('Ctrl Pts',(86.5093023154406,59.8550527643547,11.2599733876671));
#79448=CARTESIAN_POINT('Ctrl Pts',(86.4799766399047,59.8596392256511,11.3146096718499));
#79449=CARTESIAN_POINT('Ctrl Pts',(86.4536558654889,59.8642256869475,11.3708124034107));
#79450=CARTESIAN_POINT('Ctrl Pts',(86.4304918409927,59.8688121482439,11.4282157144369));
#79451=CARTESIAN_POINT('Ctrl Pts',(86.4061181056582,59.873638131474,11.4886168381923));
#79452=CARTESIAN_POINT('Ctrl Pts',(86.3852400924201,59.8784641147041,11.5503467708357));
#79453=CARTESIAN_POINT('Ctrl Pts',(86.3679750425218,59.8832900979342,11.6129615637679));
#79454=CARTESIAN_POINT('Ctrl Pts',(86.3507099926235,59.8881160811642,11.6755763567001));
#79455=CARTESIAN_POINT('Ctrl Pts',(86.3370579666174,59.8929420643943,11.739075360146));
#79456=CARTESIAN_POINT('Ctrl Pts',(86.3270733459061,59.8977680476244,11.8030059711094));
#79457=CARTESIAN_POINT('Ctrl Pts',(86.3135757387981,59.9042920035595,11.8894299118791));
#79458=CARTESIAN_POINT('Ctrl Pts',(86.3067291470103,59.9108159594947,11.9769188414441));
#79459=CARTESIAN_POINT('Ctrl Pts',(86.3066605212234,59.9173399154298,12.0646670770413));
#79460=CARTESIAN_POINT('',(86.3066600524911,60.7110899153719,12.0655770041428));
#79461=CARTESIAN_POINT('Ctrl Pts',(86.306660521223,59.9173399154754,12.0646670776546));
#79462=CARTESIAN_POINT('Ctrl Pts',(86.3066129479909,59.9218624984084,12.1254965309288));
#79463=CARTESIAN_POINT('Ctrl Pts',(86.3098261904978,59.9263850813415,12.1864461177575));
#79464=CARTESIAN_POINT('Ctrl Pts',(86.3163123336439,59.9309076642745,12.24713130348));
#79465=CARTESIAN_POINT('Ctrl Pts',(86.3227916386046,59.9354254791567,12.3077525102656));
#79466=CARTESIAN_POINT('Ctrl Pts',(86.3325369576799,59.939943294039,12.3681093485899));
#79467=CARTESIAN_POINT('Ctrl Pts',(86.3455083588812,59.9444611089212,12.4278182264114));
#79468=CARTESIAN_POINT('Ctrl Pts',(86.3584711803611,59.9489759355686,12.4874876107709));
#79469=CARTESIAN_POINT('Ctrl Pts',(86.3746557460688,59.9534907622159,12.5465093713017));
#79470=CARTESIAN_POINT('Ctrl Pts',(86.3939707165961,59.9580055888633,12.6045082471181));
#79471=CARTESIAN_POINT('Ctrl Pts',(86.4132804969975,59.9625192023316,12.6624915380562));
#79472=CARTESIAN_POINT('Ctrl Pts',(86.4357188476173,59.9670328157999,12.7194519911633));
#79473=CARTESIAN_POINT('Ctrl Pts',(86.4611447048284,59.9715464292682,12.775029900377));
#79474=CARTESIAN_POINT('Ctrl Pts',(86.4865916952581,59.9760637943181,12.8306540043007));
#79475=CARTESIAN_POINT('Ctrl Pts',(86.5150309359955,59.980581159368,12.8848927886205));
#79476=CARTESIAN_POINT('Ctrl Pts',(86.5462739446734,59.985098524418,12.9374082960631));
#79477=CARTESIAN_POINT('Ctrl Pts',(86.5775291932197,59.9896176592064,12.989944377161));
#79478=CARTESIAN_POINT('Ctrl Pts',(86.6115901042272,59.9941367939947,13.0407553994953));
#79479=CARTESIAN_POINT('Ctrl Pts',(86.6482248598373,59.9986559287831,13.0895324874935));
#79480=CARTESIAN_POINT('Ctrl Pts',(86.684927495256,60.0031834369862,13.1383999535858));
#79481=CARTESIAN_POINT('Ctrl Pts',(86.7242131612465,60.0077109451894,13.1852255552867));
#79482=CARTESIAN_POINT('Ctrl Pts',(86.76581046214,60.0122384533925,13.2297344415304));
#79483=CARTESIAN_POINT('Ctrl Pts',(86.8011641645117,60.0160863996309,13.2675627112343));
#79484=CARTESIAN_POINT('Ctrl Pts',(86.8381868570541,60.0199343458693,13.303718035511));
#79485=CARTESIAN_POINT('Ctrl Pts',(86.876693414237,60.0237822921076,13.3380547964198));
#79486=CARTESIAN_POINT('Ctrl Pts',(86.9226980208934,60.0283795156997,13.3790776583694));
#79487=CARTESIAN_POINT('Ctrl Pts',(86.9710253567054,60.0329767392918,13.4176858363108));
#79488=CARTESIAN_POINT('Ctrl Pts',(87.0213917046313,60.0375739628839,13.4536059445453));
#79489=CARTESIAN_POINT('Ctrl Pts',(87.0726204615035,60.042249903455,13.4901411027878));
#79490=CARTESIAN_POINT('Ctrl Pts',(87.1259583820144,60.0469258440261,13.5238948469401));
#79491=CARTESIAN_POINT('Ctrl Pts',(87.1810690153139,60.0516017845973,13.5546199636771));
#79492=CARTESIAN_POINT('Ctrl Pts',(87.2351028537838,60.0561863629697,13.584744748956));
#79493=CARTESIAN_POINT('Ctrl Pts',(87.2908402888454,60.0607709413421,13.6119579340704));
#79494=CARTESIAN_POINT('Ctrl Pts',(87.3479343506829,60.0653555197145,13.6360696737074));
#79495=CARTESIAN_POINT('Ctrl Pts',(87.4049935176242,60.0699372960725,13.6601666766691));
#79496=CARTESIAN_POINT('Ctrl Pts',(87.4634071992927,60.0745190724304,13.6811657951226));
#79497=CARTESIAN_POINT('Ctrl Pts',(87.5228060535599,60.0791008487884,13.6989242193866));
#79498=CARTESIAN_POINT('Ctrl Pts',(87.5821904212602,60.0836815077139,13.7166783126141));
#79499=CARTESIAN_POINT('Ctrl Pts',(87.6425589970882,60.0882621666393,13.7311931348913));
#79500=CARTESIAN_POINT('Ctrl Pts',(87.7035267489651,60.0928428255648,13.7423755651697));
#79501=CARTESIAN_POINT('Ctrl Pts',(87.7666970587904,60.0975889681503,13.7539619787004));
#79502=CARTESIAN_POINT('Ctrl Pts',(87.8305101056303,60.1023351107358,13.7619704463725));
#79503=CARTESIAN_POINT('Ctrl Pts',(87.8945280086709,60.1070812533213,13.7663555836459));
#79504=CARTESIAN_POINT('Ctrl Pts',(87.9563920654883,60.1116677146177,13.7705931854502));
#79505=CARTESIAN_POINT('Ctrl Pts',(88.0184468831037,60.1162541759141,13.7714474754972));
#79506=CARTESIAN_POINT('Ctrl Pts',(88.080296521582,60.1208406372105,13.768930658511));
#79507=CARTESIAN_POINT('Ctrl Pts',(88.1453761764165,60.1256666204406,13.7662824040543));
#79508=CARTESIAN_POINT('Ctrl Pts',(88.2102279920796,60.1304926036707,13.759901336269));
#79509=CARTESIAN_POINT('Ctrl Pts',(88.2743991136333,60.1353185869007,13.7498633384385));
#79510=CARTESIAN_POINT('Ctrl Pts',(88.3385702351869,60.1401445701308,13.739825340608));
#79511=CARTESIAN_POINT('Ctrl Pts',(88.4020600455273,60.1449705533608,13.7261306249994));
#79512=CARTESIAN_POINT('Ctrl Pts',(88.4644336759938,60.1497965365909,13.7089159251388));
#79513=CARTESIAN_POINT('Ctrl Pts',(88.5238506925549,60.154393760183,13.6925172307056));
#79514=CARTESIAN_POINT('Ctrl Pts',(88.5824989273805,60.158990983775,13.6728574407152));
#79515=CARTESIAN_POINT('Ctrl Pts',(88.6399948155849,60.1635882073671,13.6500266277962));
#79516=CARTESIAN_POINT('Ctrl Pts',(88.698475189868,60.1682641479382,13.6268048892268));
#79517=CARTESIAN_POINT('Ctrl Pts',(88.7557628470377,60.1729400885094,13.6003025620697));
#79518=CARTESIAN_POINT('Ctrl Pts',(88.8114676074206,60.1776160290805,13.5706682176049));
#79519=CARTESIAN_POINT('Ctrl Pts',(88.8660839644523,60.1822006074529,13.5416128922331));
#79520=CARTESIAN_POINT('Ctrl Pts',(88.9191782532287,60.1867851858253,13.50954709097));
#79521=CARTESIAN_POINT('Ctrl Pts',(88.9704027846842,60.1913697641977,13.4746593386409));
#79522=CARTESIAN_POINT('Ctrl Pts',(89.0215960085983,60.1959515405557,13.4397929090983));
#79523=CARTESIAN_POINT('Ctrl Pts',(89.0709213212645,60.2005333169136,13.4021082343319));
#79524=CARTESIAN_POINT('Ctrl Pts',(89.1180584145327,60.2051150932716,13.3618381466882));
#79525=CARTESIAN_POINT('Ctrl Pts',(89.1651840117092,60.209695752197,13.3215778803675));
#79526=CARTESIAN_POINT('Ctrl Pts',(89.2101220620533,60.2142764111225,13.2787337834054));
#79527=CARTESIAN_POINT('Ctrl Pts',(89.2525854916771,60.2188570700479,13.2335788206614));
#79528=CARTESIAN_POINT('Ctrl Pts',(89.2965829808909,60.2236032126334,13.1867925623708));
#79529=CARTESIAN_POINT('Ctrl Pts',(89.3379231818021,60.2283493552189,13.1375256536989));
#79530=CARTESIAN_POINT('Ctrl Pts',(89.376330459886,60.2330954978045,13.0861213510693));
#79531=CARTESIAN_POINT('Ctrl Pts',(89.4134455467713,60.2376819591008,13.0364465171951));
#79532=CARTESIAN_POINT('Ctrl Pts',(89.4478217102424,60.2422684203972,12.9847763170237));
#79533=CARTESIAN_POINT('Ctrl Pts',(89.4792544464154,60.2468548816936,12.9314500079042));
#79534=CARTESIAN_POINT('Ctrl Pts',(89.5123287160632,60.2516808649237,12.8753388021398));
#79535=CARTESIAN_POINT('Ctrl Pts',(89.5421433905218,60.2565068481538,12.8173943355545));
#79536=CARTESIAN_POINT('Ctrl Pts',(89.5685165929858,60.2613328313839,12.7580382201685));
#79537=CARTESIAN_POINT('Ctrl Pts',(89.5948897954498,60.2661588146139,12.6986821047824));
#79538=CARTESIAN_POINT('Ctrl Pts',(89.617821369533,60.270984797844,12.6379149741709));
#79539=CARTESIAN_POINT('Ctrl Pts',(89.6371903157418,60.2758107810741,12.5761763347977));
#79540=CARTESIAN_POINT('Ctrl Pts',(89.6556411416605,60.2804080046662,12.5173642096953));
#79541=CARTESIAN_POINT('Ctrl Pts',(89.6709352658989,60.2850052282582,12.4574291402083));
#79542=CARTESIAN_POINT('Ctrl Pts',(89.6829403152594,60.2896024518503,12.3967422225998));
#79543=CARTESIAN_POINT('Ctrl Pts',(89.6951509237362,60.2942783924214,12.3350161798051));
#79544=CARTESIAN_POINT('Ctrl Pts',(89.7039585120003,60.2989543329926,12.2725127767161));
#79545=CARTESIAN_POINT('Ctrl Pts',(89.7092762649574,60.3036302735637,12.2096403964156));
#79546=CARTESIAN_POINT('Ctrl Pts',(89.7144901154814,60.3082148519361,12.1479964660525));
#79547=CARTESIAN_POINT('Ctrl Pts',(89.7163492335356,60.3127994303085,12.0859983790548));
#79548=CARTESIAN_POINT('Ctrl Pts',(89.714823416698,60.3173840086809,12.0240404919991));
#79549=CARTESIAN_POINT('Ctrl Pts',(89.7132985324129,60.3219657850389,11.9621204725249));
#79550=CARTESIAN_POINT('Ctrl Pts',(89.7083928279001,60.3265475613969,11.900241112112));
#79551=CARTESIAN_POINT('Ctrl Pts',(89.7001281757988,60.3311293377548,11.8387977963955));
#79552=CARTESIAN_POINT('Ctrl Pts',(89.6918655393329,60.3357099966803,11.7773694658623));
#79553=CARTESIAN_POINT('Ctrl Pts',(89.680245649347,60.3402906556057,11.7163774731916));
#79554=CARTESIAN_POINT('Ctrl Pts',(89.6653421208768,60.3448713145311,11.6562110510363));
#79555=CARTESIAN_POINT('Ctrl Pts',(89.6499001785061,60.3496174571167,11.5938710202554));
#79556=CARTESIAN_POINT('Ctrl Pts',(89.630932879344,60.3543635997022,11.5324179319364));
#79557=CARTESIAN_POINT('Ctrl Pts',(89.6085790965537,60.3591097422877,11.4722695343384));
#79558=CARTESIAN_POINT('Ctrl Pts',(89.5869773941715,60.3636962035841,11.4141447956368));
#79559=CARTESIAN_POINT('Ctrl Pts',(89.5622137536472,60.3682826648805,11.3572388002696));
#79560=CARTESIAN_POINT('Ctrl Pts',(89.5344622696087,60.3728691261769,11.3019073690456));
#79561=CARTESIAN_POINT('Ctrl Pts',(89.5052615006662,60.3776951094069,11.2436863263013));
#79562=CARTESIAN_POINT('Ctrl Pts',(89.4727525700976,60.382521092637,11.1872093800826));
#79563=CARTESIAN_POINT('Ctrl Pts',(89.4371910333326,60.3873470758671,11.1328580107821));
#79564=CARTESIAN_POINT('Ctrl Pts',(89.4016294965676,60.3921730590971,11.0785066414816));
#79565=CARTESIAN_POINT('Ctrl Pts',(89.3630158010626,60.3969990423272,11.0262813241333));
#79566=CARTESIAN_POINT('Ctrl Pts',(89.3216535555268,60.4018250255573,10.9765221007359));
#79567=CARTESIAN_POINT('Ctrl Pts',(89.2822519492771,60.4064222491494,10.929121547352));
#79568=CARTESIAN_POINT('Ctrl Pts',(89.2401947425895,60.4110194727414,10.883763922235));
#79569=CARTESIAN_POINT('Ctrl Pts',(89.1957219022323,60.4156166963335,10.8407617170644));
#79570=CARTESIAN_POINT('Ctrl Pts',(89.1504875658173,60.4202926369046,10.7970231971127));
#79571=CARTESIAN_POINT('Ctrl Pts',(89.1027543586077,60.4249685774758,10.7557219872247));
#79572=CARTESIAN_POINT('Ctrl Pts',(89.0528182834772,60.4296445180469,10.717152529078));
#79573=CARTESIAN_POINT('Ctrl Pts',(89.0038578985954,60.4342290964193,10.6793366712916));
#79574=CARTESIAN_POINT('Ctrl Pts',(88.9527803764849,60.4388136747917,10.6441471011552));
#79575=CARTESIAN_POINT('Ctrl Pts',(88.8999006426985,60.4433982531641,10.6118230908826));
#79576=CARTESIAN_POINT('Ctrl Pts',(88.8470532280844,60.4479800295221,10.5795188364821));
#79577=CARTESIAN_POINT('Ctrl Pts',(88.7924062192987,60.45256180588,10.5500769341547));
#79578=CARTESIAN_POINT('Ctrl Pts',(88.7363036518768,60.457143582238,10.5236934649123));
#79579=CARTESIAN_POINT('Ctrl Pts',(88.6802147671027,60.4617242411635,10.4973164302368));
#79580=CARTESIAN_POINT('Ctrl Pts',(88.6226714888481,60.4663049000889,10.4739965644364));
#79581=CARTESIAN_POINT('Ctrl Pts',(88.5640407484093,60.4708855590144,10.4538831412708));
#79582=CARTESIAN_POINT('Ctrl Pts',(88.5032918783133,60.4756317015999,10.4330430883919));
#79583=CARTESIAN_POINT('Ctrl Pts',(88.4413759981938,60.4803778441854,10.4156458388827));
#79584=CARTESIAN_POINT('Ctrl Pts',(88.3787193918396,60.4851239867709,10.4018013085977));
#79585=CARTESIAN_POINT('Ctrl Pts',(88.3181708316499,60.4897104480673,10.3884225697219));
#79586=CARTESIAN_POINT('Ctrl Pts',(88.2569311322003,60.4942969093637,10.3783612868975));
#79587=CARTESIAN_POINT('Ctrl Pts',(88.195393654796,60.4988833706601,10.3716641963085));
#79588=CARTESIAN_POINT('Ctrl Pts',(88.1306424632386,60.5037093538902,10.3646173589356));
#79589=CARTESIAN_POINT('Ctrl Pts',(88.0655621813225,60.5085353371202,10.3612957739798));
#79590=CARTESIAN_POINT('Ctrl Pts',(88.0006119117509,60.5133613203503,10.3616916584073));
#79591=CARTESIAN_POINT('Ctrl Pts',(87.9356616421792,60.5181873035804,10.3620875428348));
#79592=CARTESIAN_POINT('Ctrl Pts',(87.8708420267378,60.5230132868104,10.3662007783859));
#79593=CARTESIAN_POINT('Ctrl Pts',(87.8066034188971,60.5278392700405,10.3739607353157));
#79594=CARTESIAN_POINT('Ctrl Pts',(87.7454098279936,60.5324364936326,10.3813528573705));
#79595=CARTESIAN_POINT('Ctrl Pts',(87.6844921499851,60.5370337172246,10.3920840873396));
#79596=CARTESIAN_POINT('Ctrl Pts',(87.6242430734256,60.5416309408167,10.4061223191612));
#79597=CARTESIAN_POINT('Ctrl Pts',(87.5629623687099,60.5463068813878,10.4204009237161));
#79598=CARTESIAN_POINT('Ctrl Pts',(87.5023739153509,60.550982821959,10.4381008764927));
#79599=CARTESIAN_POINT('Ctrl Pts',(87.442885631628,60.5556587625301,10.4591332040118));
#79600=CARTESIAN_POINT('Ctrl Pts',(87.3845596767063,60.5602433409025,10.4797545854));
#79601=CARTESIAN_POINT('Ctrl Pts',(87.3272917890264,60.5648279192749,10.5035791137684));
#79602=CARTESIAN_POINT('Ctrl Pts',(87.2714538014706,60.5694124976473,10.530471994446));
#79603=CARTESIAN_POINT('Ctrl Pts',(87.2156499411203,60.5739942740053,10.5573484386633));
#79604=CARTESIAN_POINT('Ctrl Pts',(87.1612747056924,60.5785760503632,10.587289296267));
#79605=CARTESIAN_POINT('Ctrl Pts',(87.1086794314454,60.5831578267212,10.6201118898188));
#79606=CARTESIAN_POINT('Ctrl Pts',(87.0560969844655,60.5877384856466,10.6529264783895));
#79607=CARTESIAN_POINT('Ctrl Pts',(87.0052940685559,60.5923191445721,10.6886211383305));
#79608=CARTESIAN_POINT('Ctrl Pts',(86.9565951148436,60.5968998034975,10.7269685687938));
#79609=CARTESIAN_POINT('Ctrl Pts',(86.9061368332193,60.601645946083,10.7667013617673));
#79610=CARTESIAN_POINT('Ctrl Pts',(86.8579379388001,60.6063920886686,10.8092819568575));
#79611=CARTESIAN_POINT('Ctrl Pts',(86.812321990022,60.6111382312541,10.8544118422521));
#79612=CARTESIAN_POINT('Ctrl Pts',(86.7682407641002,60.6157246925505,10.8980233581185));
#79613=CARTESIAN_POINT('Ctrl Pts',(86.7265717301612,60.6203111538469,10.9440148987681));
#79614=CARTESIAN_POINT('Ctrl Pts',(86.6875675109478,60.6248976151433,10.9920813426888));
#79615=CARTESIAN_POINT('Ctrl Pts',(86.6465263474752,60.6297235983733,11.0426579936841));
#79616=CARTESIAN_POINT('Ctrl Pts',(86.6084363492216,60.6345495816034,11.09553169276));
#79617=CARTESIAN_POINT('Ctrl Pts',(86.5735399942341,60.6393755648335,11.1503125165082));
#79618=CARTESIAN_POINT('Ctrl Pts',(86.5386436392466,60.6442015480636,11.2050933402564));
#79619=CARTESIAN_POINT('Ctrl Pts',(86.5069411762764,60.6490275312937,11.261780685355));
#79620=CARTESIAN_POINT('Ctrl Pts',(86.4786175389448,60.6538535145238,11.3199578908329));
#79621=CARTESIAN_POINT('Ctrl Pts',(86.4496369214494,60.6587914387174,11.3794845441073));
#79622=CARTESIAN_POINT('Ctrl Pts',(86.4240874916357,60.663729362911,11.4407864007869));
#79623=CARTESIAN_POINT('Ctrl Pts',(86.4021724737663,60.6686672871046,11.503462155555));
#79624=CARTESIAN_POINT('Ctrl Pts',(86.3803110941619,60.6735931254451,11.5659845078132));
#79625=CARTESIAN_POINT('Ctrl Pts',(86.3620665597285,60.6785189637856,11.6298737052834));
#79626=CARTESIAN_POINT('Ctrl Pts',(86.3475949281985,60.6834448021261,11.6947071200453));
#79627=CARTESIAN_POINT('Ctrl Pts',(86.3331772318557,60.6883522820657,11.7592989032843));
#79628=CARTESIAN_POINT('Ctrl Pts',(86.3225045213705,60.6932597620053,11.8248275188846));
#79629=CARTESIAN_POINT('Ctrl Pts',(86.3156830782276,60.6981672419449,11.8908561438356));
#79630=CARTESIAN_POINT('Ctrl Pts',(86.3096955324728,60.7024747997539,11.9488130020448));
#79631=CARTESIAN_POINT('Ctrl Pts',(86.3066745521873,60.7067823575629,12.007154655696));
#79632=CARTESIAN_POINT('Ctrl Pts',(86.3066600524911,60.7110899153719,12.0655770041428));
#79633=CARTESIAN_POINT('',(86.3066607115161,61.5048399155016,12.0675573471538));
#79634=CARTESIAN_POINT('Ctrl Pts',(86.3066600524909,60.7110899154298,12.0655770049287));
#79635=CARTESIAN_POINT('Ctrl Pts',(86.3066441759981,60.7158064996465,12.1295468780701));
#79636=CARTESIAN_POINT('Ctrl Pts',(86.3102341532229,60.7205230838632,12.1934773303318));
#79637=CARTESIAN_POINT('Ctrl Pts',(86.3173906533801,60.7252396680799,12.256950822574));
#79638=CARTESIAN_POINT('Ctrl Pts',(86.3245616248092,60.729965789776,12.3205526655672));
#79639=CARTESIAN_POINT('Ctrl Pts',(86.3353134694598,60.7346919114722,12.383695239678));
#79640=CARTESIAN_POINT('Ctrl Pts',(86.3495552008937,60.7394180331683,12.4459684396404));
#79641=CARTESIAN_POINT('Ctrl Pts',(86.3638114807984,60.7441489827776,12.5083052540469));
#79642=CARTESIAN_POINT('Ctrl Pts',(86.3815646199732,60.7488799323869,12.5697704781106));
#79643=CARTESIAN_POINT('Ctrl Pts',(86.4026737719427,60.7536108819962,12.6299694847622));
#79644=CARTESIAN_POINT('Ctrl Pts',(86.4238362968947,60.7583537934736,12.6903207003012));
#79645=CARTESIAN_POINT('Ctrl Pts',(86.4483716155272,60.763096704951,12.7493988686388));
#79646=CARTESIAN_POINT('Ctrl Pts',(86.4760907903572,60.7678396164284,12.8068296388197));
#79647=CARTESIAN_POINT('Ctrl Pts',(86.4995229647787,60.7718489972879,12.8553782638165));
#79648=CARTESIAN_POINT('Ctrl Pts',(86.5252294344248,60.7758583781474,12.9027499362615));
#79649=CARTESIAN_POINT('Ctrl Pts',(86.5530718782772,60.7798677590069,12.9487346302768));
#79650=CARTESIAN_POINT('Ctrl Pts',(86.5849964931304,60.784464982599,13.0014614545943));
#79651=CARTESIAN_POINT('Ctrl Pts',(86.6198506742157,60.7890622061911,13.0525624218208));
#79652=CARTESIAN_POINT('Ctrl Pts',(86.6574435278868,60.7936594297831,13.1016928658635));
#79653=CARTESIAN_POINT('Ctrl Pts',(86.6956800735201,60.7983353703543,13.1516645568146));
#79654=CARTESIAN_POINT('Ctrl Pts',(86.7367497681312,60.8030113109254,13.1995971051849));
#79655=CARTESIAN_POINT('Ctrl Pts',(86.7804036226425,60.8076872514965,13.2451553721349));
#79656=CARTESIAN_POINT('Ctrl Pts',(86.8232045338646,60.8122718298689,13.28982348589));
#79657=CARTESIAN_POINT('Ctrl Pts',(86.8684891614438,60.8168564082413,13.3322088797932));
#79658=CARTESIAN_POINT('Ctrl Pts',(86.9159816096461,60.8214409866138,13.3720281621721));
#79659=CARTESIAN_POINT('Ctrl Pts',(86.9634450312912,60.8260227629717,13.4118231076992));
#79660=CARTESIAN_POINT('Ctrl Pts',(87.0131132086595,60.8306045393297,13.4490547251605));
#79661=CARTESIAN_POINT('Ctrl Pts',(87.0646750440703,60.8351863156876,13.4834780116054));
#79662=CARTESIAN_POINT('Ctrl Pts',(87.1162243042556,60.8397669746131,13.5178929026821));
#79663=CARTESIAN_POINT('Ctrl Pts',(87.1696658824878,60.8443476335385,13.5495005398805));
#79664=CARTESIAN_POINT('Ctrl Pts',(87.2246590873795,60.848928292464,13.5780988078625));
#79665=CARTESIAN_POINT('Ctrl Pts',(87.2816390101152,60.8536744350495,13.6077302342032));
#79666=CARTESIAN_POINT('Ctrl Pts',(87.3402843297241,60.858420577635,13.6341303665783));
#79667=CARTESIAN_POINT('Ctrl Pts',(87.4001898151027,60.8631667202205,13.6571271959293));
#79668=CARTESIAN_POINT('Ctrl Pts',(87.4580798142295,60.8677531815169,13.6793503099335));
#79669=CARTESIAN_POINT('Ctrl Pts',(87.5171460004979,60.8723396428133,13.6983954101024));
#79670=CARTESIAN_POINT('Ctrl Pts',(87.5770063166188,60.8769261041097,13.7141578560275));
#79671=CARTESIAN_POINT('Ctrl Pts',(87.6399927593417,60.8817520873398,13.7307434750448));
#79672=CARTESIAN_POINT('Ctrl Pts',(87.7038579222001,60.8865780705699,13.743694034646));
#79673=CARTESIAN_POINT('Ctrl Pts',(87.7681466383619,60.8914040538,13.7529490449747));
#79674=CARTESIAN_POINT('Ctrl Pts',(87.8324353545238,60.8962300370301,13.7622040553035));
#79675=CARTESIAN_POINT('Ctrl Pts',(87.8971469717572,60.9010560202601,13.767763537989));
#79676=CARTESIAN_POINT('Ctrl Pts',(87.9618256413461,60.9058820034902,13.7696304523138));
#79677=CARTESIAN_POINT('Ctrl Pts',(88.0234384343382,60.9104792270823,13.7714088717921));
#79678=CARTESIAN_POINT('Ctrl Pts',(88.0852743034678,60.9150764506744,13.7698442377821));
#79679=CARTESIAN_POINT('Ctrl Pts',(88.1469401469759,60.9196736742664,13.7649099776151));
#79680=CARTESIAN_POINT('Ctrl Pts',(88.2096618775458,60.9243496148376,13.7598912294857));
#79681=CARTESIAN_POINT('Ctrl Pts',(88.2722071777644,60.9290255554087,13.751386264506));
#79682=CARTESIAN_POINT('Ctrl Pts',(88.3341594390292,60.9337014959798,13.7394224847797));
#79683=CARTESIAN_POINT('Ctrl Pts',(88.3949012283648,60.9382860743522,13.7276924627764));
#79684=CARTESIAN_POINT('Ctrl Pts',(88.4550724211052,60.9428706527246,13.7126376736548));
#79685=CARTESIAN_POINT('Ctrl Pts',(88.5142852884022,60.947455231097,13.6943361919695));
#79686=CARTESIAN_POINT('Ctrl Pts',(88.5734619658261,60.952037007455,13.6760458958312));
#79687=CARTESIAN_POINT('Ctrl Pts',(88.6316809938509,60.9566187838129,13.6545129917608));
#79688=CARTESIAN_POINT('Ctrl Pts',(88.6885678013138,60.9612005601709,13.6298659502089));
#79689=CARTESIAN_POINT('Ctrl Pts',(88.7454407348635,60.9657812190963,13.6052249197328));
#79690=CARTESIAN_POINT('Ctrl Pts',(88.800981625966,60.9703618780218,13.5774714617722));
#79691=CARTESIAN_POINT('Ctrl Pts',(88.8548358826594,60.9749425369472,13.546782171265));
#79692=CARTESIAN_POINT('Ctrl Pts',(88.9106357108641,60.9796886795328,13.5149841808523));
#79693=CARTESIAN_POINT('Ctrl Pts',(88.9646241698028,60.9844348221183,13.4800344054183));
#79694=CARTESIAN_POINT('Ctrl Pts',(89.0164369541746,60.9891809647038,13.4421799906916));
#79695=CARTESIAN_POINT('Ctrl Pts',(89.0665065266532,60.9937674260002,13.405599166388));
#79696=CARTESIAN_POINT('Ctrl Pts',(89.1145441448782,60.9983538872966,13.3663064515924));
#79697=CARTESIAN_POINT('Ctrl Pts',(89.1602546708257,61.002940348593,13.3245660638939));
#79698=CARTESIAN_POINT('Ctrl Pts',(89.2083523691176,61.007766331823,13.2806458391209));
#79699=CARTESIAN_POINT('Ctrl Pts',(89.253872793751,61.0125923150531,13.2340157312277));
#79700=CARTESIAN_POINT('Ctrl Pts',(89.2965182439904,61.0174182982832,13.1850253258831));
#79701=CARTESIAN_POINT('Ctrl Pts',(89.3391636942298,61.0222442815133,13.1360349205385));
#79702=CARTESIAN_POINT('Ctrl Pts',(89.3789338344764,61.0270702647434,13.084684777428));
#79703=CARTESIAN_POINT('Ctrl Pts',(89.4155838991065,61.0318962479734,13.0313594698198));
#79704=CARTESIAN_POINT('Ctrl Pts',(89.4504966896689,61.0364934715655,12.9805618705524));
#79705=CARTESIAN_POINT('Ctrl Pts',(89.4827219064413,61.0410906951576,12.9277635922223));
#79706=CARTESIAN_POINT('Ctrl Pts',(89.5120240072541,61.0456879187497,12.8732804749569));
#79707=CARTESIAN_POINT('Ctrl Pts',(89.5418278397772,61.0503638593209,12.8178644584508));
#79708=CARTESIAN_POINT('Ctrl Pts',(89.5686071321136,61.055039799892,12.7607057451108));
#79709=CARTESIAN_POINT('Ctrl Pts',(89.5921589373602,61.0597157404631,12.7021691995107));
#79710=CARTESIAN_POINT('Ctrl Pts',(89.6152505689416,61.0643003188355,12.6447763869047));
#79711=CARTESIAN_POINT('Ctrl Pts',(89.6352395023911,61.068884897208,12.5860595950058));
#79712=CARTESIAN_POINT('Ctrl Pts',(89.6519810261474,61.0734694755804,12.52638691057));
#79713=CARTESIAN_POINT('Ctrl Pts',(89.6687123177759,61.0780512519384,12.4667506970397));
#79714=CARTESIAN_POINT('Ctrl Pts',(89.6821999979823,61.0826330282963,12.4061602385123));
#79715=CARTESIAN_POINT('Ctrl Pts',(89.6923488305763,61.0872148046543,12.3449999023654));
#79716=CARTESIAN_POINT('Ctrl Pts',(89.702495188009,61.0917954635798,12.2838544823869));
#79717=CARTESIAN_POINT('Ctrl Pts',(89.7093042310432,61.0963761225052,12.2221399626512));
#79718=CARTESIAN_POINT('Ctrl Pts',(89.7127319905835,61.1009567814307,12.1602500282483));
#79719=CARTESIAN_POINT('Ctrl Pts',(89.716283583442,61.1057029240162,12.0961242205725));
#79720=CARTESIAN_POINT('Ctrl Pts',(89.7162048105288,61.1104490666017,12.0318106582684));
#79721=CARTESIAN_POINT('Ctrl Pts',(89.7125057054581,61.1151952091872,11.9677494534695));
#79722=CARTESIAN_POINT('Ctrl Pts',(89.7089310546901,61.1197816704836,11.9058435517568));
#79723=CARTESIAN_POINT('Ctrl Pts',(89.7019759578328,61.12436813178,11.8441738117826));
#79724=CARTESIAN_POINT('Ctrl Pts',(89.6917023071775,61.1289545930764,11.7831314965425));
#79725=CARTESIAN_POINT('Ctrl Pts',(89.6808921285736,61.1337805763064,11.7189013263454));
#79726=CARTESIAN_POINT('Ctrl Pts',(89.6664074097455,61.1386065595365,11.6553665410596));
#79727=CARTESIAN_POINT('Ctrl Pts',(89.6483803725037,61.1434325427665,11.5929668602099));
#79728=CARTESIAN_POINT('Ctrl Pts',(89.6303533352618,61.1482585259965,11.5305671793602));
#79729=CARTESIAN_POINT('Ctrl Pts',(89.6087842677816,61.1530845092265,11.469303188463));
#79730=CARTESIAN_POINT('Ctrl Pts',(89.5838634976358,61.1579104924566,11.4095891123657));
#79731=CARTESIAN_POINT('Ctrl Pts',(89.5601240134756,61.1625077160486,11.3527055828697));
#79732=CARTESIAN_POINT('Ctrl Pts',(89.5332459797793,61.1671049396407,11.2969947751641));
#79733=CARTESIAN_POINT('Ctrl Pts',(89.5033669827431,61.1717021632328,11.2428258845067));
#79734=CARTESIAN_POINT('Ctrl Pts',(89.4729763759632,61.1763781038039,11.1877294750227));
#79735=CARTESIAN_POINT('Ctrl Pts',(89.4394811858226,61.181054044375,11.1342288091747));
#79736=CARTESIAN_POINT('Ctrl Pts',(89.4030778646249,61.1857299849461,11.0826922890461));
#79737=CARTESIAN_POINT('Ctrl Pts',(89.3673858201031,61.1903145633186,11.0321627299177));
#79738=CARTESIAN_POINT('Ctrl Pts',(89.3288985729185,61.1948991416909,10.9835216884461));
#79739=CARTESIAN_POINT('Ctrl Pts',(89.2878468691759,61.1994837200633,10.9370903896787));
#79740=CARTESIAN_POINT('Ctrl Pts',(89.2468202555196,61.2040654964213,10.8906874689125));
#79741=CARTESIAN_POINT('Ctrl Pts',(89.2032326296158,61.2086472727792,10.8464919934662));
#79742=CARTESIAN_POINT('Ctrl Pts',(89.157355250644,61.2132290491372,10.8047924536696));
#79743=CARTESIAN_POINT('Ctrl Pts',(89.1114890605367,61.2178097080626,10.7631030838196));
#79744=CARTESIAN_POINT('Ctrl Pts',(89.0633346024734,61.2223903669881,10.7239087834454));
#79745=CARTESIAN_POINT('Ctrl Pts',(89.0131987708498,61.2269710259135,10.6874600262208));
#79746=CARTESIAN_POINT('Ctrl Pts',(88.9612517017919,61.231717168499,10.6496944991057));
#79747=CARTESIAN_POINT('Ctrl Pts',(88.9071777901919,61.2364633110846,10.6148770812555));
#79748=CARTESIAN_POINT('Ctrl Pts',(88.8513522257904,61.2412094536701,10.5832380594954));
#79749=CARTESIAN_POINT('Ctrl Pts',(88.7974048810022,61.2457959149665,10.5526635147692));
#79750=CARTESIAN_POINT('Ctrl Pts',(88.7418223909129,61.2503823762629,10.5250570482046));
#79751=CARTESIAN_POINT('Ctrl Pts',(88.6849670341506,61.2549688375592,10.5005788833422));
#79752=CARTESIAN_POINT('Ctrl Pts',(88.6251424808521,61.2597948207893,10.474822378382));
#79753=CARTESIAN_POINT('Ctrl Pts',(88.563909069067,61.2646208040195,10.4525301083734));
#79754=CARTESIAN_POINT('Ctrl Pts',(88.5017079334239,61.2694467872496,10.4338294943007));
#79755=CARTESIAN_POINT('Ctrl Pts',(88.4395067977809,61.2742727704797,10.4151288802279));
#79756=CARTESIAN_POINT('Ctrl Pts',(88.3763385864904,61.2790987537098,10.400019997572));
#79757=CARTESIAN_POINT('Ctrl Pts',(88.3126545320565,61.2839247369399,10.3885676231544));
#79758=CARTESIAN_POINT('Ctrl Pts',(88.2519892078063,61.2885219605319,10.377658110347));
#79759=CARTESIAN_POINT('Ctrl Pts',(88.1906067665736,61.293119184124,10.3700214422995));
#79760=CARTESIAN_POINT('Ctrl Pts',(88.1288920036934,61.297716407716,10.3657422809865));
#79761=CARTESIAN_POINT('Ctrl Pts',(88.0661205161181,61.3023923482871,10.3613898487861));
#79762=CARTESIAN_POINT('Ctrl Pts',(88.00300572438,61.3070682888583,10.3605111721684));
#79763=CARTESIAN_POINT('Ctrl Pts',(87.9399636863555,61.3117442294294,10.3631410282282));
#79764=CARTESIAN_POINT('Ctrl Pts',(87.8781534131749,61.3163288078018,10.3657195000951));
#79765=CARTESIAN_POINT('Ctrl Pts',(87.8164136091926,61.3209133861742,10.371670610537));
#79766=CARTESIAN_POINT('Ctrl Pts',(87.7551392987735,61.3254979645465,10.3809747369348));
#79767=CARTESIAN_POINT('Ctrl Pts',(87.6939024381457,61.3300797409045,10.3902731768126));
#79768=CARTESIAN_POINT('Ctrl Pts',(87.6331310091896,61.3346615172624,10.4029204929095));
#79769=CARTESIAN_POINT('Ctrl Pts',(87.5732145093823,61.3392432936203,10.4188452714439));
#79770=CARTESIAN_POINT('Ctrl Pts',(87.5133126223886,61.3438239525457,10.434766166143));
#79771=CARTESIAN_POINT('Ctrl Pts',(87.4542657423754,61.3484046114711,10.4539628057942));
#79772=CARTESIAN_POINT('Ctrl Pts',(87.3964507567196,61.3529852703965,10.476313218529));
#79773=CARTESIAN_POINT('Ctrl Pts',(87.3365471118574,61.3577314129821,10.4994710758182));
#79774=CARTESIAN_POINT('Ctrl Pts',(87.2779666392387,61.3624775555676,10.5260147893731));
#79775=CARTESIAN_POINT('Ctrl Pts',(87.221106310152,61.3672236981532,10.5557540616382));
#79776=CARTESIAN_POINT('Ctrl Pts',(87.1661590147529,61.3718101594495,10.5844927728689));
#79777=CARTESIAN_POINT('Ctrl Pts',(87.1128183638655,61.3763966207459,10.6162150862082));
#79778=CARTESIAN_POINT('Ctrl Pts',(87.0614154641582,61.3809830820422,10.6507035487609));
#79779=CARTESIAN_POINT('Ctrl Pts',(87.007328115342,61.3858090652724,10.6869931260968));
#79780=CARTESIAN_POINT('Ctrl Pts',(86.9553869805493,61.3906350485025,10.7263453120269));
#79781=CARTESIAN_POINT('Ctrl Pts',(86.9059383797233,61.3954610317326,10.7684586129947));
#79782=CARTESIAN_POINT('Ctrl Pts',(86.8564897788974,61.4002870149628,10.8105719139625));
#79783=CARTESIAN_POINT('Ctrl Pts',(86.8095341270401,61.4051129981929,10.8554458263333));
#79784=CARTESIAN_POINT('Ctrl Pts',(86.7653705924827,61.4099389814231,10.9027363949955));
#79785=CARTESIAN_POINT('Ctrl Pts',(86.7238082338614,61.4144807203876,10.9472416093955));
#79786=CARTESIAN_POINT('Ctrl Pts',(86.684538764033,61.4190224593521,10.9940794473683));
#79787=CARTESIAN_POINT('Ctrl Pts',(86.6478391663862,61.4235641983167,11.0429812429377));
#79788=CARTESIAN_POINT('Ctrl Pts',(86.6111914874166,61.4280995121132,11.0918138574614));
#79789=CARTESIAN_POINT('Ctrl Pts',(86.5771067908207,61.4326348259098,11.1427042334525));
#79790=CARTESIAN_POINT('Ctrl Pts',(86.5458242256299,61.4371701397064,11.1953480685148));
#79791=CARTESIAN_POINT('Ctrl Pts',(86.5145737630342,61.441700799302,11.2479378797553));
#79792=CARTESIAN_POINT('Ctrl Pts',(86.4861199992106,61.4462314588977,11.302277137944));
#79793=CARTESIAN_POINT('Ctrl Pts',(86.4606595426181,61.4507621184934,11.3580315672256));
#79794=CARTESIAN_POINT('Ctrl Pts',(86.4352075425464,61.4552912732607,11.4137674780457));
#79795=CARTESIAN_POINT('Ctrl Pts',(86.4127471112947,61.459820428028,11.4709171613093));
#79796=CARTESIAN_POINT('Ctrl Pts',(86.3934286111655,61.4643495827954,11.5291223252694));
#79797=CARTESIAN_POINT('Ctrl Pts',(86.3741152572093,61.4688775310604,11.5873119842038));
#79798=CARTESIAN_POINT('Ctrl Pts',(86.3579423331523,61.4734054793255,11.6465560683486));
#79799=CARTESIAN_POINT('Ctrl Pts',(86.3450108760953,61.4779334275906,11.7064793821891));
#79800=CARTESIAN_POINT('Ctrl Pts',(86.3320682999305,61.4824652692101,11.7664542210651));
#79801=CARTESIAN_POINT('Ctrl Pts',(86.3223728674377,61.4869971108295,11.8271089440921));
#79802=CARTESIAN_POINT('Ctrl Pts',(86.3159745177665,61.491528952449,11.8880577335792));
#79803=CARTESIAN_POINT('Ctrl Pts',(86.3097100891034,61.4959659401092,11.9477308310904));
#79804=CARTESIAN_POINT('Ctrl Pts',(86.3066060032365,61.5004029277695,12.0076853217731));
#79805=CARTESIAN_POINT('Ctrl Pts',(86.3066607115152,61.5048399154298,12.0675573461848));
#79806=CARTESIAN_POINT('',(86.3066600835977,62.2985899154715,12.0654661855251));
#79807=CARTESIAN_POINT('Ctrl Pts',(86.3066607115161,61.5048399155016,12.0675573471538));
#79808=CARTESIAN_POINT('Ctrl Pts',(86.3067344748707,61.5108223170385,12.1482829471039));
#79809=CARTESIAN_POINT('Ctrl Pts',(86.312547324273,61.5168047185754,12.2287530864269));
#79810=CARTESIAN_POINT('Ctrl Pts',(86.3239687341642,61.5227871201123,12.3082815380758));
#79811=CARTESIAN_POINT('Ctrl Pts',(86.3323475036833,61.5271758220436,12.3666237719092));
#79812=CARTESIAN_POINT('Ctrl Pts',(86.343743627015,61.531564523975,12.4244598713876));
#79813=CARTESIAN_POINT('Ctrl Pts',(86.3580897682031,61.5359532259064,12.481526895906));
#79814=CARTESIAN_POINT('Ctrl Pts',(86.3731175417349,61.5405504494983,12.541305362418));
#79815=CARTESIAN_POINT('Ctrl Pts',(86.3914232300308,61.5451476730902,12.6003902552955));
#79816=CARTESIAN_POINT('Ctrl Pts',(86.4129256062274,61.5497448966821,12.6583960394604));
#79817=CARTESIAN_POINT('Ctrl Pts',(86.4347961616233,61.5544208372532,12.7173950405132));
#79818=CARTESIAN_POINT('Ctrl Pts',(86.4599738701113,61.5590967778244,12.7752770930347));
#79819=CARTESIAN_POINT('Ctrl Pts',(86.4883191737899,61.5637727183955,12.8316487034484));
#79820=CARTESIAN_POINT('Ctrl Pts',(86.5161106446655,61.5683572967677,12.8869188810688));
#79821=CARTESIAN_POINT('Ctrl Pts',(86.546946802419,61.57294187514,12.9407366335863));
#79822=CARTESIAN_POINT('Ctrl Pts',(86.5806471688951,61.5775264535122,12.9927500278663));
#79823=CARTESIAN_POINT('Ctrl Pts',(86.6143269382942,61.58210822987,13.0447316324656));
#79824=CARTESIAN_POINT('Ctrl Pts',(86.6508671690947,61.5866900062277,13.0949106391781));
#79825=CARTESIAN_POINT('Ctrl Pts',(86.6900424575833,61.5912717825855,13.1429614694744));
#79826=CARTESIAN_POINT('Ctrl Pts',(86.7292081917555,61.5958524415108,13.1910005808312));
#79827=CARTESIAN_POINT('Ctrl Pts',(86.7710073863296,61.600433100436,13.2369121517682));
#79828=CARTESIAN_POINT('Ctrl Pts',(86.8151737513127,61.6050137593613,13.280402906185));
#79829=CARTESIAN_POINT('Ctrl Pts',(86.8609356971641,61.609759901947,13.3254648339533));
#79830=CARTESIAN_POINT('Ctrl Pts',(86.9092387544391,61.6145060445327,13.3679272309615));
#79831=CARTESIAN_POINT('Ctrl Pts',(86.9597460970713,61.6192521871183,13.4075066407503));
#79832=CARTESIAN_POINT('Ctrl Pts',(87.0085541486572,61.6238386484145,13.4457544236278));
#79833=CARTESIAN_POINT('Ctrl Pts',(87.0594200335514,61.6284251097108,13.4813099007641));
#79834=CARTESIAN_POINT('Ctrl Pts',(87.1120092877091,61.633011571007,13.5139608195026));
#79835=CARTESIAN_POINT('Ctrl Pts',(87.1673449467881,61.6378375542374,13.5483168897087));
#79836=CARTESIAN_POINT('Ctrl Pts',(87.224588351958,61.6426635374678,13.5794563917294));
#79837=CARTESIAN_POINT('Ctrl Pts',(87.2833221858692,61.6474895206983,13.607187799855));
#79838=CARTESIAN_POINT('Ctrl Pts',(87.3420560197804,61.6523155039287,13.6349192079806));
#79839=CARTESIAN_POINT('Ctrl Pts',(87.402279652622,61.6571414871591,13.6592423512942));
#79840=CARTESIAN_POINT('Ctrl Pts',(87.4635564771644,61.6619674703895,13.6800261537241));
#79841=CARTESIAN_POINT('Ctrl Pts',(87.5219286782211,61.6665646939814,13.6998247693217));
#79842=CARTESIAN_POINT('Ctrl Pts',(87.5814961302972,61.6711619175733,13.7164933458481));
#79843=CARTESIAN_POINT('Ctrl Pts',(87.6418908798614,61.6757591411652,13.7298910099615));
#79844=CARTESIAN_POINT('Ctrl Pts',(87.7033197519028,61.6804350817363,13.7435180785462));
#79845=CARTESIAN_POINT('Ctrl Pts',(87.7656040475827,61.6851110223075,13.7537609063011));
#79846=CARTESIAN_POINT('Ctrl Pts',(87.8283374885835,61.6897869628786,13.7605233083446));
#79847=CARTESIAN_POINT('Ctrl Pts',(87.889845194349,61.6943715412509,13.7671535812663));
#79848=CARTESIAN_POINT('Ctrl Pts',(87.9517841214331,61.6989561196231,13.770438154704));
#79849=CARTESIAN_POINT('Ctrl Pts',(88.0137607122301,61.7035406979953,13.7703377640796));
#79850=CARTESIAN_POINT('Ctrl Pts',(88.0756994240142,61.708122474353,13.7702374348123));
#79851=CARTESIAN_POINT('Ctrl Pts',(88.137675245877,61.7127042507108,13.766756244499));
#79852=CARTESIAN_POINT('Ctrl Pts',(88.1992923937076,61.7172860270686,13.7599069661796));
#79853=CARTESIAN_POINT('Ctrl Pts',(88.2608945139597,61.7218666859938,13.7530593583054));
#79854=CARTESIAN_POINT('Ctrl Pts',(88.3221376281278,61.7264473449191,13.7428453493028));
#79855=CARTESIAN_POINT('Ctrl Pts',(88.3826309133882,61.7310280038443,13.7293295824383));
#79856=CARTESIAN_POINT('Ctrl Pts',(88.4453096157339,61.73577414643,13.7153255367887));
#79857=CARTESIAN_POINT('Ctrl Pts',(88.5071826929468,61.7405202890157,13.6977766673657));
#79858=CARTESIAN_POINT('Ctrl Pts',(88.5678293132122,61.7452664316014,13.6768122024456));
#79859=CARTESIAN_POINT('Ctrl Pts',(88.6264355121557,61.7498528928976,13.6565530751195));
#79860=CARTESIAN_POINT('Ctrl Pts',(88.6838960142886,61.7544393541938,13.6331048151613));
#79861=CARTESIAN_POINT('Ctrl Pts',(88.7398510887762,61.75902581549,13.6066332873172));
#79862=CARTESIAN_POINT('Ctrl Pts',(88.798728343744,61.7638517987205,13.5787793186014));
#79863=CARTESIAN_POINT('Ctrl Pts',(88.8559380508016,61.7686777819509,13.5475779494007));
#79864=CARTESIAN_POINT('Ctrl Pts',(88.9110929527311,61.7735037651814,13.5132758935475));
#79865=CARTESIAN_POINT('Ctrl Pts',(88.9662478546607,61.7783297484119,13.4789738376944));
#79866=CARTESIAN_POINT('Ctrl Pts',(89.0193474662625,61.7831557316423,13.4415715316011));
#79867=CARTESIAN_POINT('Ctrl Pts',(89.0700448525328,61.7879817148728,13.4013646827454));
#79868=CARTESIAN_POINT('Ctrl Pts',(89.1183390983164,61.7925789384661,13.3630637054432));
#79869=CARTESIAN_POINT('Ctrl Pts',(89.1646520346834,61.7971761620594,13.3220608431329));
#79870=CARTESIAN_POINT('Ctrl Pts',(89.2086657334164,61.8017733856526,13.2785888118403));
#79871=CARTESIAN_POINT('Ctrl Pts',(89.25343306644,61.8064493262236,13.2343724210776));
#79872=CARTESIAN_POINT('Ctrl Pts',(89.2958212078182,61.8111252667946,13.1876017627667));
#79873=CARTESIAN_POINT('Ctrl Pts',(89.3355289857389,61.8158012073656,13.1385659893626));
#79874=CARTESIAN_POINT('Ctrl Pts',(89.3744609219252,61.8203857857392,13.0904883153909));
#79875=CARTESIAN_POINT('Ctrl Pts',(89.4108159590514,61.8249703641128,13.0402336599975));
#79876=CARTESIAN_POINT('Ctrl Pts',(89.444347644956,61.8295549424864,12.9881113622004));
#79877=CARTESIAN_POINT('Ctrl Pts',(89.4778588368781,61.8341367188456,12.936020920644));
#79878=CARTESIAN_POINT('Ctrl Pts',(89.5085498243185,61.8387184952047,12.8820655272747));
#79879=CARTESIAN_POINT('Ctrl Pts',(89.5362166653663,61.8433002715639,12.8265846167842));
#79880=CARTESIAN_POINT('Ctrl Pts',(89.5638767588505,61.8478809304905,12.7711172373281));
#79881=CARTESIAN_POINT('Ctrl Pts',(89.5885139430192,61.8524615894172,12.7141255346751));
#79882=CARTESIAN_POINT('Ctrl Pts',(89.6099705442328,61.8570422483438,12.6559729097814));
#79883=CARTESIAN_POINT('Ctrl Pts',(89.6322022996125,61.8617883909282,12.5957194279529));
#79884=CARTESIAN_POINT('Ctrl Pts',(89.6510190034195,61.8665345335125,12.5342200608254));
#79885=CARTESIAN_POINT('Ctrl Pts',(89.666300964409,61.8712806760969,12.4718984513726));
#79886=CARTESIAN_POINT('Ctrl Pts',(89.6810687724518,61.8758671373944,12.4116736172724));
#79887=CARTESIAN_POINT('Ctrl Pts',(89.6925358981186,61.880453598692,12.3506815257231));
#79888=CARTESIAN_POINT('Ctrl Pts',(89.7006465703345,61.8850400599896,12.2893143590479));
#79889=CARTESIAN_POINT('Ctrl Pts',(89.7091808117768,61.8898660432173,12.224742372522));
#79890=CARTESIAN_POINT('Ctrl Pts',(89.7139983552846,61.894692026445,12.1597557024171));
#79891=CARTESIAN_POINT('Ctrl Pts',(89.7150964225358,61.8995180096728,12.0948135089969));
#79892=CARTESIAN_POINT('Ctrl Pts',(89.7161944897869,61.9043439929005,12.0298713155767));
#79893=CARTESIAN_POINT('Ctrl Pts',(89.7135731842489,61.9091699761282,11.9649742431773));
#79894=CARTESIAN_POINT('Ctrl Pts',(89.7072927589168,61.913995959356,11.9005741506097));
#79895=CARTESIAN_POINT('Ctrl Pts',(89.7013100361987,61.9185931829462,11.8392267296193));
#79896=CARTESIAN_POINT('Ctrl Pts',(89.6919827429114,61.9231904065364,11.7780783495286));
#79897=CARTESIAN_POINT('Ctrl Pts',(89.6793339448426,61.9277876301266,11.7175223334476));
#79898=CARTESIAN_POINT('Ctrl Pts',(89.6664685649219,61.932463570698,11.6559294335428));
#79899=CARTESIAN_POINT('Ctrl Pts',(89.6501668201511,61.9371395112694,11.5949499113494));
#79900=CARTESIAN_POINT('Ctrl Pts',(89.6305082784108,61.9418154518407,11.5349936236174));
#79901=CARTESIAN_POINT('Ctrl Pts',(89.6112338407047,61.9464000302113,11.4762088089429));
#79902=CARTESIAN_POINT('Ctrl Pts',(89.5887327679586,61.9509846085819,11.4184081096921));
#79903=CARTESIAN_POINT('Ctrl Pts',(89.5631312670824,61.9555691869525,11.3619663606439));
#79904=CARTESIAN_POINT('Ctrl Pts',(89.5375454133977,61.9601509633086,11.3055591078095));
#79905=CARTESIAN_POINT('Ctrl Pts',(89.5088630987932,61.9647327396647,11.250509620908));
#79906=CARTESIAN_POINT('Ctrl Pts',(89.4772588716991,61.9693145160209,11.1971733448129));
#79907=CARTESIAN_POINT('Ctrl Pts',(89.4456623524432,61.9738951749445,11.143850076705));
#79908=CARTESIAN_POINT('Ctrl Pts',(89.4111455947277,61.9784758338682,11.0922396276918));
#79909=CARTESIAN_POINT('Ctrl Pts',(89.3739283774024,61.9830564927918,11.042671570965));
#79910=CARTESIAN_POINT('Ctrl Pts',(89.3353666283021,61.9878026353791,10.9913127885449));
#79911=CARTESIAN_POINT('Ctrl Pts',(89.2939058648324,61.9925487779664,10.9421472966084));
#79912=CARTESIAN_POINT('Ctrl Pts',(89.2498370780422,61.9972949205537,10.8955054337299));
#79913=CARTESIAN_POINT('Ctrl Pts',(89.2072509607485,62.0018813818483,10.8504328100428));
#79914=CARTESIAN_POINT('Ctrl Pts',(89.1622299681931,62.006467843143,10.807717000004));
#79915=CARTESIAN_POINT('Ctrl Pts',(89.1150733308866,62.0110543044376,10.7676175772813));
#79916=CARTESIAN_POINT('Ctrl Pts',(89.0654539999091,62.0158802876712,10.7254240146836));
#79917=CARTESIAN_POINT('Ctrl Pts',(89.0134703521095,62.0207062709048,10.6861280048536));
#79918=CARTESIAN_POINT('Ctrl Pts',(88.9595066307898,62.0255322541384,10.6499809298785));
#79919=CARTESIAN_POINT('Ctrl Pts',(88.9055429094701,62.030358237372,10.6138338549034));
#79920=CARTESIAN_POINT('Ctrl Pts',(88.8495997120712,62.0351842206056,10.5808359773451));
#79921=CARTESIAN_POINT('Ctrl Pts',(88.7920893358986,62.0400102038393,10.5511817650472));
#79922=CARTESIAN_POINT('Ctrl Pts',(88.7373050473324,62.0446074274305,10.5229332117974));
#79923=CARTESIAN_POINT('Ctrl Pts',(88.6808738862995,62.0492046510219,10.497602462629));
#79924=CARTESIAN_POINT('Ctrl Pts',(88.6231388027267,62.0538018746131,10.475383477454));
#79925=CARTESIAN_POINT('Ctrl Pts',(88.5644151373884,62.0584778151844,10.4527840427805));
#79926=CARTESIAN_POINT('Ctrl Pts',(88.5043429036074,62.0631537557556,10.4334042662798));
#79927=CARTESIAN_POINT('Ctrl Pts',(88.4433095882361,62.0678296963268,10.4173996070851));
#79928=CARTESIAN_POINT('Ctrl Pts',(88.3834687897197,62.0724142746984,10.4017076594928));
#79929=CARTESIAN_POINT('Ctrl Pts',(88.3227046445502,62.07699885307,10.3892602592979));
#79930=CARTESIAN_POINT('Ctrl Pts',(88.2614005138331,62.0815834314415,10.3801546873239));
#79931=CARTESIAN_POINT('Ctrl Pts',(88.2001338511333,62.0861652077986,10.3710546805169));
#79932=CARTESIAN_POINT('Ctrl Pts',(88.1383283597657,62.0907469841557,10.3652925266471));
#79933=CARTESIAN_POINT('Ctrl Pts',(88.0763773313464,62.0953287605128,10.3629143767426));
#79934=CARTESIAN_POINT('Ctrl Pts',(88.0144414119348,62.0999094194374,10.3605368068364));
#79935=CARTESIAN_POINT('Ctrl Pts',(87.9523605343781,62.104490078362,10.3615416220435));
#79936=CARTESIAN_POINT('Ctrl Pts',(87.8905307878683,62.1090707372866,10.3659229415911));
#79937=CARTESIAN_POINT('Ctrl Pts',(87.8264673424463,62.1138168798729,10.3704625433452));
#79938=CARTESIAN_POINT('Ctrl Pts',(87.7626741049852,62.1185630224592,10.3786273064894));
#79939=CARTESIAN_POINT('Ctrl Pts',(87.6995864330993,62.1233091650455,10.3903519385175));
#79940=CARTESIAN_POINT('Ctrl Pts',(87.6386213103571,62.127895626341,10.4016821019128));
#79941=CARTESIAN_POINT('Ctrl Pts',(87.5783155233266,62.1324820876365,10.4163361883729));
#79942=CARTESIAN_POINT('Ctrl Pts',(87.5190494476001,62.137068548932,10.4342036004472));
#79943=CARTESIAN_POINT('Ctrl Pts',(87.456688278664,62.1418945321637,10.4530041147239));
#79944=CARTESIAN_POINT('Ctrl Pts',(87.3954790026308,62.1467205153954,10.4753625706521));
#79945=CARTESIAN_POINT('Ctrl Pts',(87.3358412240052,62.1515464986272,10.5010925066327));
#79946=CARTESIAN_POINT('Ctrl Pts',(87.2762034453795,62.1563724818589,10.5268224426133));
#79947=CARTESIAN_POINT('Ctrl Pts',(87.2181377087964,62.1611984650906,10.5559234991368));
#79948=CARTESIAN_POINT('Ctrl Pts',(87.1620310203565,62.1660244483224,10.5881547756266));
#79949=CARTESIAN_POINT('Ctrl Pts',(87.1085838822509,62.1706216719236,10.6188582360121));
#79950=CARTESIAN_POINT('Ctrl Pts',(87.0566947915483,62.1752188955248,10.6525278821585));
#79951=CARTESIAN_POINT('Ctrl Pts',(87.0067127136938,62.179816119126,10.6889807981863));
#79952=CARTESIAN_POINT('Ctrl Pts',(86.9558748067559,62.184492059696,10.7260578872587));
#79953=CARTESIAN_POINT('Ctrl Pts',(86.907010340959,62.189168000266,10.7660142758366));
#79954=CARTESIAN_POINT('Ctrl Pts',(86.8604600931996,62.193843940836,10.8086087488535));
#79955=CARTESIAN_POINT('Ctrl Pts',(86.8148193806325,62.1984285192176,10.8503709777027));
#79956=CARTESIAN_POINT('Ctrl Pts',(86.7714036589527,62.2030130975992,10.8946687681268));
#79957=CARTESIAN_POINT('Ctrl Pts',(86.7305025904295,62.2075976759808,10.9412328153421));
#79958=CARTESIAN_POINT('Ctrl Pts',(86.6896265199272,62.2121794523479,10.9877684034226));
#79959=CARTESIAN_POINT('Ctrl Pts',(86.6512623903516,62.2167612287151,11.0365671201859));
#79960=CARTESIAN_POINT('Ctrl Pts',(86.6156622950455,62.2213430050822,11.0873235852784));
#79961=CARTESIAN_POINT('Ctrl Pts',(86.5800708821153,62.2259236640168,11.1380676715639));
#79962=CARTESIAN_POINT('Ctrl Pts',(86.5472424574208,62.2305043229514,11.1907681417634));
#79963=CARTESIAN_POINT('Ctrl Pts',(86.5173869186885,62.235084981886,11.245089043236));
#79964=CARTESIAN_POINT('Ctrl Pts',(86.4864528007921,62.2398311244626,11.3013723742943));
#79965=CARTESIAN_POINT('Ctrl Pts',(86.4587108181782,62.2445772670393,11.3593949809681));
#79966=CARTESIAN_POINT('Ctrl Pts',(86.4343422546599,62.2493234096159,11.4187556955376));
#79967=CARTESIAN_POINT('Ctrl Pts',(86.4107935576202,62.2539098709213,11.4761192525813));
#79968=CARTESIAN_POINT('Ctrl Pts',(86.390394981605,62.2584963322267,11.5347317794983));
#79969=CARTESIAN_POINT('Ctrl Pts',(86.3732599266061,62.263082793532,11.5942137267791));
#79970=CARTESIAN_POINT('Ctrl Pts',(86.3552300159058,62.2679087767443,11.6568020404916));
#79971=CARTESIAN_POINT('Ctrl Pts',(86.3408139925677,62.2727347599566,11.7203524477324));
#79972=CARTESIAN_POINT('Ctrl Pts',(86.3300827992189,62.2775607431689,11.7844112933401));
#79973=CARTESIAN_POINT('Ctrl Pts',(86.3193516058702,62.2823867263812,11.8484701389477));
#79974=CARTESIAN_POINT('Ctrl Pts',(86.3123052358886,62.2872127095934,11.9130367703652));
#79975=CARTESIAN_POINT('Ctrl Pts',(86.3089512152314,62.2920386928057,11.977655391406));
#79976=CARTESIAN_POINT('Ctrl Pts',(86.3074335323714,62.2942224336805,12.0068950961104));
#79977=CARTESIAN_POINT('Ctrl Pts',(86.3066692581048,62.2964061745552,12.0361742440832));
#79978=CARTESIAN_POINT('Ctrl Pts',(86.3066600835979,62.2985899154299,12.0654661849667));
#79979=CARTESIAN_POINT('',(86.3066604360558,63.0923399153734,12.0647808303758));
#79980=CARTESIAN_POINT('Ctrl Pts',(86.3066600835977,62.2985899154715,12.0654661855251));
#79981=CARTESIAN_POINT('Ctrl Pts',(86.3066409247245,62.3031501668908,12.126635812625));
#79982=CARTESIAN_POINT('Ctrl Pts',(86.3099191485247,62.3077104183102,12.1879386415856));
#79983=CARTESIAN_POINT('Ctrl Pts',(86.3165116107995,62.3122706697295,12.2489861592162));
#79984=CARTESIAN_POINT('Ctrl Pts',(86.3230929799242,62.3168232476042,12.3099309520609));
#79985=CARTESIAN_POINT('Ctrl Pts',(86.3329774650661,62.3213758254789,12.3706207754731));
#79986=CARTESIAN_POINT('Ctrl Pts',(86.3461299231414,62.3259284033536,12.4306676058837));
#79987=CARTESIAN_POINT('Ctrl Pts',(86.3592701199207,62.3304767371162,12.4906584580154));
#79988=CARTESIAN_POINT('Ctrl Pts',(86.3756721442038,62.3350250708789,12.5500070010703));
#79989=CARTESIAN_POINT('Ctrl Pts',(86.395249330378,62.3395734046416,12.6083325633003));
#79990=CARTESIAN_POINT('Ctrl Pts',(86.4148157428858,62.3441192353771,12.6666260279584));
#79991=CARTESIAN_POINT('Ctrl Pts',(86.4375536893511,62.3486650661125,12.7238971374533));
#79992=CARTESIAN_POINT('Ctrl Pts',(86.4633264760513,62.353210896848,12.7797797271346));
#79993=CARTESIAN_POINT('Ctrl Pts',(86.4890949221422,62.3577559619823,12.8356529051643));
#79994=CARTESIAN_POINT('Ctrl Pts',(86.5178969762771,62.3623010271166,12.8901375576983));
#79995=CARTESIAN_POINT('Ctrl Pts',(86.5495484264447,62.3668460922509,12.9428888947596));
#79996=CARTESIAN_POINT('Ctrl Pts',(86.581228963405,62.3713953341723,12.9956887088164));
#79997=CARTESIAN_POINT('Ctrl Pts',(86.6157638595154,62.3759445760937,13.0467515806393));
#79998=CARTESIAN_POINT('Ctrl Pts',(86.6529243586932,62.3804938180151,13.0957598691389));
#79999=CARTESIAN_POINT('Ctrl Pts',(86.6901020368947,62.3850451630174,13.1447908138076));
#80000=CARTESIAN_POINT('Ctrl Pts',(86.7299073996572,62.3895965080196,13.1917648882435));
#80001=CARTESIAN_POINT('Ctrl Pts',(86.7720720065963,62.3941478530219,13.2363983350811));
#80002=CARTESIAN_POINT('Ctrl Pts',(86.8143143084384,62.3987075845913,13.2811140260466));
#80003=CARTESIAN_POINT('Ctrl Pts',(86.8589241592856,62.4032673161608,13.3234801196338));
#80004=CARTESIAN_POINT('Ctrl Pts',(86.9055977174153,62.4078270477302,13.3632511820217));
#80005=CARTESIAN_POINT('Ctrl Pts',(86.9404885615714,62.4112356775831,13.3929820616739));
#80006=CARTESIAN_POINT('Ctrl Pts',(86.9765319281591,62.414644307436,13.4212635625407));
#80007=CARTESIAN_POINT('Ctrl Pts',(87.0135906687455,62.418052937289,13.4480092118096));
#80008=CARTESIAN_POINT('Ctrl Pts',(87.0635718411982,62.4226501608808,13.4840811043595));
#80009=CARTESIAN_POINT('Ctrl Pts',(87.1156149772854,62.4272473844726,13.5175121494062));
#80010=CARTESIAN_POINT('Ctrl Pts',(87.1694097378665,62.4318446080644,13.5480596028102));
#80011=CARTESIAN_POINT('Ctrl Pts',(87.2241256111526,62.4365205486355,13.5791301117522));
#80012=CARTESIAN_POINT('Ctrl Pts',(87.280653284269,62.4411964892067,13.6072169623774));
#80013=CARTESIAN_POINT('Ctrl Pts',(87.3386326569108,62.4458724297779,13.6321088696343));
#80014=CARTESIAN_POINT('Ctrl Pts',(87.3954791830314,62.4504570081495,13.6565144192564));
#80015=CARTESIAN_POINT('Ctrl Pts',(87.4537206998271,62.4550415865212,13.677848542848));
#80016=CARTESIAN_POINT('Ctrl Pts',(87.5129925462586,62.4596261648929,13.6959581011848));
#80017=CARTESIAN_POINT('Ctrl Pts',(87.5722281667676,62.4642079412499,13.7140565912742));
#80018=CARTESIAN_POINT('Ctrl Pts',(87.6324923824485,62.468789717607,13.7289342754822));
#80019=CARTESIAN_POINT('Ctrl Pts',(87.6934031180205,62.473371493964,13.7404871024158));
#80020=CARTESIAN_POINT('Ctrl Pts',(87.7542989982961,62.4779521528884,13.7520371117727));
#80021=CARTESIAN_POINT('Ctrl Pts',(87.8158405855425,62.4825328118127,13.760263778773));
#80022=CARTESIAN_POINT('Ctrl Pts',(87.8776353100951,62.4871134707371,13.7651140912507));
#80023=CARTESIAN_POINT('Ctrl Pts',(87.9416624683375,62.4918596133234,13.770139629058));
#80024=CARTESIAN_POINT('Ctrl Pts',(88.0059608294402,62.4966057559096,13.7715400797695));
#80025=CARTESIAN_POINT('Ctrl Pts',(88.0700901669213,62.5013518984959,13.7693153518281));
#80026=CARTESIAN_POINT('Ctrl Pts',(88.1320619090005,62.5059383597908,13.7671654736039));
#80027=CARTESIAN_POINT('Ctrl Pts',(88.1938753015951,62.5105248210857,13.7616306118411));
#80028=CARTESIAN_POINT('Ctrl Pts',(88.2551377616971,62.5151112823806,13.7527636434645));
#80029=CARTESIAN_POINT('Ctrl Pts',(88.3195995735795,62.5199372656126,13.7434336092721));
#80030=CARTESIAN_POINT('Ctrl Pts',(88.3834506984063,62.5247632488445,13.7304140131299));
#80031=CARTESIAN_POINT('Ctrl Pts',(88.4462484918887,62.5295892320764,13.7138269283844));
#80032=CARTESIAN_POINT('Ctrl Pts',(88.5090462853711,62.5344152153083,13.6972398436388));
#80033=CARTESIAN_POINT('Ctrl Pts',(88.5707901555195,62.5392411985402,13.6770855449223));
#80034=CARTESIAN_POINT('Ctrl Pts',(88.6310616095541,62.5440671817722,13.653544782347));
#80035=CARTESIAN_POINT('Ctrl Pts',(88.6884760971671,62.5486644054318,13.6311198907805));
#80036=CARTESIAN_POINT('Ctrl Pts',(88.744790359347,62.5532616290915,13.6055303074046));
#80037=CARTESIAN_POINT('Ctrl Pts',(88.7996321340302,62.5578588527511,13.5769050905914));
#80038=CARTESIAN_POINT('Ctrl Pts',(88.8554129482248,62.5625347933138,13.5477897326446));
#80039=CARTESIAN_POINT('Ctrl Pts',(88.9096698458675,62.5672107338765,13.5155339107476));
#80040=CARTESIAN_POINT('Ctrl Pts',(88.9620300039657,62.5718866744392,13.4803255520413));
#80041=CARTESIAN_POINT('Ctrl Pts',(89.0133671090328,62.5764712528796,13.4458051213207));
#80042=CARTESIAN_POINT('Ctrl Pts',(89.0628804852146,62.58105583132,13.408446791651));
#80043=CARTESIAN_POINT('Ctrl Pts',(89.1102436853043,62.5856404097604,13.3684738599751));
#80044=CARTESIAN_POINT('Ctrl Pts',(89.1575779378311,62.5902221861863,13.3285253590588));
#80045=CARTESIAN_POINT('Ctrl Pts',(89.202764231824,62.5948039626123,13.2859657523754));
#80046=CARTESIAN_POINT('Ctrl Pts',(89.24550791434,62.5993857390382,13.2410595921195));
#80047=CARTESIAN_POINT('Ctrl Pts',(89.288241172256,62.6039663980315,13.1961643838622));
#80048=CARTESIAN_POINT('Ctrl Pts',(89.3285326504828,62.6085470570248,13.1489241266734));
#80049=CARTESIAN_POINT('Ctrl Pts',(89.3661248830719,62.613127716018,13.0996398729148));
#80050=CARTESIAN_POINT('Ctrl Pts',(89.4050751943188,62.6178738585378,13.0485751478039));
#80051=CARTESIAN_POINT('Ctrl Pts',(89.4411270933243,62.6226200010576,12.9953163367531));
#80052=CARTESIAN_POINT('Ctrl Pts',(89.4740417248846,62.6273661435774,12.9402332336664));
#80053=CARTESIAN_POINT('Ctrl Pts',(89.5058489631424,62.6319526049405,12.887003368989));
#80054=CARTESIAN_POINT('Ctrl Pts',(89.534726516419,62.6365390663036,12.8320705261377));
#80055=CARTESIAN_POINT('Ctrl Pts',(89.5605058711942,62.6411255276667,12.7757932027955));
#80056=CARTESIAN_POINT('Ctrl Pts',(89.5876315178696,62.6459515107648,12.7165768724364));
#80057=CARTESIAN_POINT('Ctrl Pts',(89.6113262497302,62.6507774938629,12.6558723794506));
#80058=CARTESIAN_POINT('Ctrl Pts',(89.6314525334729,62.655603476961,12.5941178110623));
#80059=CARTESIAN_POINT('Ctrl Pts',(89.6515788172157,62.6604294600591,12.532363242674));
#80060=CARTESIAN_POINT('Ctrl Pts',(89.6681365624707,62.6652554431573,12.4695592451861));
#80061=CARTESIAN_POINT('Ctrl Pts',(89.6810506312657,62.6700814262554,12.4061554418334));
#80062=CARTESIAN_POINT('Ctrl Pts',(89.6933525516511,62.6746786497019,12.3457570845572));
#80063=CARTESIAN_POINT('Ctrl Pts',(89.7023989868417,62.6792758731483,12.2845665250379));
#80064=CARTESIAN_POINT('Ctrl Pts',(89.7080964470144,62.6838730965948,12.2229665095841));
#80065=CARTESIAN_POINT('Ctrl Pts',(89.7138914634168,62.6885490371841,12.1603117319957));
#80066=CARTESIAN_POINT('Ctrl Pts',(89.716221539061,62.6932249777735,12.0972338451252));
#80067=CARTESIAN_POINT('Ctrl Pts',(89.715042336769,62.6979009183628,12.0341479969423));
#80068=CARTESIAN_POINT('Ctrl Pts',(89.7138861746983,62.7024854965906,11.9722947717923));
#80069=CARTESIAN_POINT('Ctrl Pts',(89.7093566456306,62.7070700748183,11.9104344269658));
#80070=CARTESIAN_POINT('Ctrl Pts',(89.7014642814849,62.7116546530461,11.848962333629));
#80071=CARTESIAN_POINT('Ctrl Pts',(89.6935767410136,62.7162364292602,11.7875278109562));
#80072=CARTESIAN_POINT('Ctrl Pts',(89.6823305055283,62.7208182054742,11.7264815731116));
#80073=CARTESIAN_POINT('Ctrl Pts',(89.6677880115279,62.7253999816883,11.6662146570254));
#80074=CARTESIAN_POINT('Ctrl Pts',(89.6532490642397,62.7299806404708,11.6059624392023));
#80075=CARTESIAN_POINT('Ctrl Pts',(89.6354155736761,62.7345612992533,11.5464896604513));
#80076=CARTESIAN_POINT('Ctrl Pts',(89.614400811079,62.7391419580359,11.4881759137668));
#80077=CARTESIAN_POINT('Ctrl Pts',(89.5926268551138,62.7438881007611,11.4277554856698));
#80078=CARTESIAN_POINT('Ctrl Pts',(89.5674375055463,62.7486342434863,11.3685800056446));
#80079=CARTESIAN_POINT('Ctrl Pts',(89.5390138793376,62.7533803862115,11.3110507168348));
#80080=CARTESIAN_POINT('Ctrl Pts',(89.5115465516341,62.7579668473691,11.2554569718042));
#80081=CARTESIAN_POINT('Ctrl Pts',(89.4810594586578,62.7625533085266,11.2014008237734));
#80082=CARTESIAN_POINT('Ctrl Pts',(89.4477623803717,62.7671397696841,11.1492182931861));
#80083=CARTESIAN_POINT('Ctrl Pts',(89.4127264026994,62.7719657531932,11.0943105934524));
#80084=CARTESIAN_POINT('Ctrl Pts',(89.3745792636135,62.7767917367022,11.0414781006924));
#80085=CARTESIAN_POINT('Ctrl Pts',(89.3336144116812,62.7816177202113,10.991073977609));
#80086=CARTESIAN_POINT('Ctrl Pts',(89.2926495597488,62.7864437037204,10.9406698545257));
#80087=CARTESIAN_POINT('Ctrl Pts',(89.2488674889268,62.7912696872295,10.8926945275948));
#80088=CARTESIAN_POINT('Ctrl Pts',(89.2026051825974,62.7960956707386,10.847454996971));
#80089=CARTESIAN_POINT('Ctrl Pts',(89.1585357887037,62.8006928943761,10.8043598974653));
#80090=CARTESIAN_POINT('Ctrl Pts',(89.112035077645,62.8052901180137,10.7635701106697));
#80091=CARTESIAN_POINT('Ctrl Pts',(89.0633738939566,62.8098873416513,10.7253717805004));
#80092=CARTESIAN_POINT('Ctrl Pts',(89.013879498924,62.8145632822167,10.6865193913952));
#80093=CARTESIAN_POINT('Ctrl Pts',(88.9621502613259,62.8192392227821,10.6503484783872));
#80094=CARTESIAN_POINT('Ctrl Pts',(88.9085109073074,62.8239151633476,10.6171214658005));
#80095=CARTESIAN_POINT('Ctrl Pts',(88.8559196005661,62.8284997417617,10.5845436683414));
#80096=CARTESIAN_POINT('Ctrl Pts',(88.8014926022352,62.8330843201758,10.5547960464102));
#80097=CARTESIAN_POINT('Ctrl Pts',(88.7455677845218,62.83766889859,10.528084200763));
#80098=CARTESIAN_POINT('Ctrl Pts',(88.689677147101,62.8422506749882,10.5013886809393));
#80099=CARTESIAN_POINT('Ctrl Pts',(88.6322909638731,62.8468324513864,10.477725477324));
#80100=CARTESIAN_POINT('Ctrl Pts',(88.5737716187422,62.8514142277845,10.4572542336533));
#80101=CARTESIAN_POINT('Ctrl Pts',(88.5152665456981,62.8559948867486,10.4367879826456));
#80102=CARTESIAN_POINT('Ctrl Pts',(88.4556293396536,62.8605755457127,10.4195123142004));
#80103=CARTESIAN_POINT('Ctrl Pts',(88.3952403429229,62.8651562046769,10.405537957534));
#80104=CARTESIAN_POINT('Ctrl Pts',(88.3326696977595,62.8699023472223,10.3910587550351));
#80105=CARTESIAN_POINT('Ctrl Pts',(88.269292454637,62.8746484897677,10.3801241550034));
#80106=CARTESIAN_POINT('Ctrl Pts',(88.2055439439558,62.8793946323131,10.372799631033));
#80107=CARTESIAN_POINT('Ctrl Pts',(88.1439402149616,62.8839810936439,10.3657215364255));
#80108=CARTESIAN_POINT('Ctrl Pts',(88.0819903367574,62.8885675549747,10.3620144014998));
#80109=CARTESIAN_POINT('Ctrl Pts',(88.0200903916493,62.8931540163055,10.3616842427591));
#80110=CARTESIAN_POINT('Ctrl Pts',(87.9549578045197,62.8979799994582,10.3613368419188));
#80111=CARTESIAN_POINT('Ctrl Pts',(87.8898811525563,62.9028059826109,10.3647287827876));
#80112=CARTESIAN_POINT('Ctrl Pts',(87.8253163012447,62.9076319657636,10.3718050880679));
#80113=CARTESIAN_POINT('Ctrl Pts',(87.7607514499332,62.9124579489163,10.3788813933482));
#80114=CARTESIAN_POINT('Ctrl Pts',(87.696699025486,62.917283932069,10.3896418793765));
#80115=CARTESIAN_POINT('Ctrl Pts',(87.6335997244982,62.9221099152218,10.4039699558518));
#80116=CARTESIAN_POINT('Ctrl Pts',(87.5734914281143,62.9267071392979,10.4176188593088));
#80117=CARTESIAN_POINT('Ctrl Pts',(87.5140011306449,62.931304363374,10.4345607631823));
#80118=CARTESIAN_POINT('Ctrl Pts',(87.4555161334491,62.9359015874501,10.4547233292815));
#80119=CARTESIAN_POINT('Ctrl Pts',(87.3960297209697,62.9405775279607,10.4752311309594));
#80120=CARTESIAN_POINT('Ctrl Pts',(87.3375838976558,62.9452534684713,10.4990709003749));
#80121=CARTESIAN_POINT('Ctrl Pts',(87.2805752627201,62.949929408982,10.526112166822));
#80122=CARTESIAN_POINT('Ctrl Pts',(87.2246805005826,62.9545139878428,10.5526250829383));
#80123=CARTESIAN_POINT('Ctrl Pts',(87.1701677523669,62.9590985667036,10.5822152866476));
#80124=CARTESIAN_POINT('Ctrl Pts',(87.1173930091322,62.9636831455644,10.6147104418924));
#80125=CARTESIAN_POINT('Ctrl Pts',(87.0646505208948,62.968264922411,10.6471857366682));
#80126=CARTESIAN_POINT('Ctrl Pts',(87.013644363941,62.9728466992577,10.682562196162));
#80127=CARTESIAN_POINT('Ctrl Pts',(86.9647052149742,62.9774284761043,10.7206219644918));
#80128=CARTESIAN_POINT('Ctrl Pts',(86.9157780016,62.9820091355179,10.758672450562));
#80129=CARTESIAN_POINT('Ctrl Pts',(86.8689171971213,62.9865897949315,10.7994046339764));
#80130=CARTESIAN_POINT('Ctrl Pts',(86.8244221247348,62.9911704543451,10.8425590404392));
#80131=CARTESIAN_POINT('Ctrl Pts',(86.7783196059005,62.9959165964584,10.8872724599265));
#80132=CARTESIAN_POINT('Ctrl Pts',(86.7347574844944,63.0006627385718,10.934586106822));
#80133=CARTESIAN_POINT('Ctrl Pts',(86.6940268888191,63.0054088806851,10.9841697637677));
#80134=CARTESIAN_POINT('Ctrl Pts',(86.6546666430059,63.0099953424627,11.0320852163492));
#80135=CARTESIAN_POINT('Ctrl Pts',(86.6179506613849,63.0145818042403,11.0821198809277));
#80136=CARTESIAN_POINT('Ctrl Pts',(86.5840988331452,63.0191682660179,11.1339442636684));
#80137=CARTESIAN_POINT('Ctrl Pts',(86.5484791482572,63.0239942482991,11.1884750904727));
#80138=CARTESIAN_POINT('Ctrl Pts',(86.5160313015061,63.0288202305803,11.2449871385155));
#80139=CARTESIAN_POINT('Ctrl Pts',(86.4869563660697,63.0336462128615,11.3030676062215));
#80140=CARTESIAN_POINT('Ctrl Pts',(86.4578814306333,63.0384721951426,11.3611480739276));
#80141=CARTESIAN_POINT('Ctrl Pts',(86.4321795918688,63.0432981774238,11.4207963355849));
#80142=CARTESIAN_POINT('Ctrl Pts',(86.409991933047,63.048124159705,11.4815789145219));
#80143=CARTESIAN_POINT('Ctrl Pts',(86.3855797573436,63.0534339910998,11.5484555060827));
#80144=CARTESIAN_POINT('Ctrl Pts',(86.3653371628071,63.0587438224946,11.6169309864996));
#80145=CARTESIAN_POINT('Ctrl Pts',(86.3494450064644,63.0640536538894,11.6865137169054));
#80146=CARTESIAN_POINT('Ctrl Pts',(86.333693968622,63.0693163352671,11.7554785695136));
#80147=CARTESIAN_POINT('Ctrl Pts',(86.3222165491053,63.0745790166449,11.8255309165857));
#80148=CARTESIAN_POINT('Ctrl Pts',(86.3151423989973,63.0798416980226,11.8961711664021));
#80149=CARTESIAN_POINT('Ctrl Pts',(86.3095423218201,63.0840077704729,11.9520917850975));
#80150=CARTESIAN_POINT('Ctrl Pts',(86.3067007811299,63.0881738429231,12.0083803880777));
#80151=CARTESIAN_POINT('Ctrl Pts',(86.3066604360558,63.0923399153734,12.0647808303758));
#80152=CARTESIAN_POINT('',(86.3066604397214,63.8860899154862,12.067224283217));
#80153=CARTESIAN_POINT('Ctrl Pts',(86.3066604360553,63.0923399154299,12.0647808311405));
#80154=CARTESIAN_POINT('Ctrl Pts',(86.3066159630468,63.0969322453676,12.1269519630066));
#80155=CARTESIAN_POINT('Ctrl Pts',(86.3099776468474,63.1015245753052,12.1891522354369));
#80156=CARTESIAN_POINT('Ctrl Pts',(86.3167284964179,63.1061169052429,12.2509835337255));
#80157=CARTESIAN_POINT('Ctrl Pts',(86.3234790823301,63.1107090558246,12.312812417158));
#80158=CARTESIAN_POINT('Ctrl Pts',(86.3336185148868,63.1153012064062,12.3742718532793));
#80159=CARTESIAN_POINT('Ctrl Pts',(86.3470779954168,63.1198933569879,12.4349693730703));
#80160=CARTESIAN_POINT('Ctrl Pts',(86.3605524404198,63.1244906131985,12.495734377367));
#80161=CARTESIAN_POINT('Ctrl Pts',(86.3773541968501,63.1290878694091,12.5557352789889));
#80162=CARTESIAN_POINT('Ctrl Pts',(86.3973636303177,63.1336851256196,12.6145913798436));
#80163=CARTESIAN_POINT('Ctrl Pts',(86.417383747727,63.1382848365133,12.6734789066327));
#80164=CARTESIAN_POINT('Ctrl Pts',(86.440614764977,63.1428845474069,12.7312199457579));
#80165=CARTESIAN_POINT('Ctrl Pts',(86.466888688362,63.1474842583005,12.7874534585623));
#80166=CARTESIAN_POINT('Ctrl Pts',(86.4932165744992,63.1520934163199,12.8438024666842));
#80167=CARTESIAN_POINT('Ctrl Pts',(86.5225996154727,63.1567025743394,12.8986373151098));
#80168=CARTESIAN_POINT('Ctrl Pts',(86.5548239238879,63.1613117323588,12.9516218555111));
#80169=CARTESIAN_POINT('Ctrl Pts',(86.5847159075744,63.1655872896353,13.0007714911495));
#80170=CARTESIAN_POINT('Ctrl Pts',(86.6170520880028,63.1698628469118,13.048329009007));
#80171=CARTESIAN_POINT('Ctrl Pts',(86.6516306929192,63.1741384041883,13.0940515174672));
#80172=CARTESIAN_POINT('Ctrl Pts',(86.6888107827956,63.1787356285181,13.143213910746));
#80173=CARTESIAN_POINT('Ctrl Pts',(86.7287376134219,63.1833328528479,13.1904576611463));
#80174=CARTESIAN_POINT('Ctrl Pts',(86.7711858425798,63.1879300771777,13.2354595720504));
#80175=CARTESIAN_POINT('Ctrl Pts',(86.814360893162,63.1926060176566,13.2812320298921));
#80176=CARTESIAN_POINT('Ctrl Pts',(86.8601442563419,63.1972819581355,13.3246846734459));
#80177=CARTESIAN_POINT('Ctrl Pts',(86.9082537831574,63.2019578986144,13.365509760194));
#80178=CARTESIAN_POINT('Ctrl Pts',(86.955423316475,63.2065424776949,13.4055371813104));
#80179=CARTESIAN_POINT('Ctrl Pts',(87.0048285241927,63.2111270567754,13.4430384546965));
#80180=CARTESIAN_POINT('Ctrl Pts',(87.0561658174368,63.2157116358559,13.4777600785576));
#80181=CARTESIAN_POINT('Ctrl Pts',(87.1074717340822,63.2202934129091,13.5124604810727));
#80182=CARTESIAN_POINT('Ctrl Pts',(87.1607069739893,63.2248751899622,13.5443843181029));
#80183=CARTESIAN_POINT('Ctrl Pts',(87.215536882838,63.2294569670154,13.573319894659));
#80184=CARTESIAN_POINT('Ctrl Pts',(87.2703534192588,63.2340376266222,13.6022484141378));
#80185=CARTESIAN_POINT('Ctrl Pts',(87.3267634025508,63.238618286229,13.6281898824503));
#80186=CARTESIAN_POINT('Ctrl Pts',(87.3844071542986,63.2431989458357,13.6509783094149));
#80187=CARTESIAN_POINT('Ctrl Pts',(87.4441333616792,63.2479450877387,13.6745899979934));
#80188=CARTESIAN_POINT('Ctrl Pts',(87.5051836700963,63.2526912296417,13.6948161946898));
#80189=CARTESIAN_POINT('Ctrl Pts',(87.5671373018131,63.2574373715447,13.7115274962024));
#80190=CARTESIAN_POINT('Ctrl Pts',(87.6270065555069,63.2620238334805,13.7276765599794));
#80191=CARTESIAN_POINT('Ctrl Pts',(87.687718779297,63.2666102954163,13.7405434605201));
#80192=CARTESIAN_POINT('Ctrl Pts',(87.748883177254,63.2711967573522,13.7500634212623));
#80193=CARTESIAN_POINT('Ctrl Pts',(87.8132417788889,63.2760227392387,13.7600805452992));
#80194=CARTESIAN_POINT('Ctrl Pts',(87.8781004378546,63.2808487211253,13.7663914943369));
#80195=CARTESIAN_POINT('Ctrl Pts',(87.9430001797093,63.2856747030118,13.7689829300496));
#80196=CARTESIAN_POINT('Ctrl Pts',(88.0078999215639,63.2905006848984,13.7715743657623));
#80197=CARTESIAN_POINT('Ctrl Pts',(88.0728400997638,63.2953266667849,13.7704463767699));
#80198=CARTESIAN_POINT('Ctrl Pts',(88.1373675896353,63.3001526486715,13.7656488072216));
#80199=CARTESIAN_POINT('Ctrl Pts',(88.1988364307533,63.3047498755962,13.7610786458702));
#80200=CARTESIAN_POINT('Ctrl Pts',(88.2601832066688,63.3093471025209,13.753160215809));
#80201=CARTESIAN_POINT('Ctrl Pts',(88.321014167319,63.3139443294457,13.741907530761));
#80202=CARTESIAN_POINT('Ctrl Pts',(88.3828866691991,63.3186202696002,13.730462178438));
#80203=CARTESIAN_POINT('Ctrl Pts',(88.4442249902356,63.3232962097547,13.7155672636015));
#80204=CARTESIAN_POINT('Ctrl Pts',(88.5046175526032,63.3279721499093,13.6972929066731));
#80205=CARTESIAN_POINT('Ctrl Pts',(88.5638301665237,63.3325567316563,13.6793755936957));
#80206=CARTESIAN_POINT('Ctrl Pts',(88.6221331352863,63.3371413134033,13.6582098604404));
#80207=CARTESIAN_POINT('Ctrl Pts',(88.6791488201293,63.3417258951503,13.6339132596416));
#80208=CARTESIAN_POINT('Ctrl Pts',(88.7361296580817,63.3463076748891,13.6096315084581));
#80209=CARTESIAN_POINT('Ctrl Pts',(88.791824304825,63.3508894546279,13.5822228831234));
#80210=CARTESIAN_POINT('Ctrl Pts',(88.8458733945532,63.3554712343667,13.5518537110588));
#80211=CARTESIAN_POINT('Ctrl Pts',(88.8999093024665,63.3600518966737,13.5214919456093));
#80212=CARTESIAN_POINT('Ctrl Pts',(88.9523000064715,63.3646325589806,13.4881713160261));
#80213=CARTESIAN_POINT('Ctrl Pts',(89.0027109653233,63.3692132212876,13.4521039632212));
#80214=CARTESIAN_POINT('Ctrl Pts',(89.0549430265505,63.3739593606099,13.4147336726551));
#80215=CARTESIAN_POINT('Ctrl Pts',(89.1050490569066,63.3787054999321,13.3744146941797));
#80216=CARTESIAN_POINT('Ctrl Pts',(89.1526921134748,63.3834516392544,13.3314303432546));
#80217=CARTESIAN_POINT('Ctrl Pts',(89.1987323115123,63.3880381038948,13.2898921177154));
#80218=CARTESIAN_POINT('Ctrl Pts',(89.2424723179012,63.3926245685351,13.2458654513764));
#80219=CARTESIAN_POINT('Ctrl Pts',(89.2836457449736,63.3972110331755,13.1996435257173));
#80220=CARTESIAN_POINT('Ctrl Pts',(89.326969309805,63.4020370098387,13.1510078221746));
#80221=CARTESIAN_POINT('Ctrl Pts',(89.367450475186,63.4068629865019,13.0999417908209));
#80222=CARTESIAN_POINT('Ctrl Pts',(89.4048290890655,63.4116889631651,13.0468237895131));
#80223=CARTESIAN_POINT('Ctrl Pts',(89.442207702945,63.4165149398283,12.9937057882052));
#80224=CARTESIAN_POINT('Ctrl Pts',(89.476483489092,63.4213409164915,12.9385364081796));
#80225=CARTESIAN_POINT('Ctrl Pts',(89.5074525489028,63.4261668931547,12.881723362717));
#80226=CARTESIAN_POINT('Ctrl Pts',(89.5369535985093,63.4307641065609,12.8276033964433));
#80227=CARTESIAN_POINT('Ctrl Pts',(89.563575507742,63.4353613199671,12.7717698886372));
#80228=CARTESIAN_POINT('Ctrl Pts',(89.5871164801729,63.4399585333734,12.7145612357576));
#80229=CARTESIAN_POINT('Ctrl Pts',(89.6110605976892,63.4446344752177,12.6563728702804));
#80230=CARTESIAN_POINT('Ctrl Pts',(89.6318169242142,63.4493104170621,12.5967622370934));
#80231=CARTESIAN_POINT('Ctrl Pts',(89.6492211283399,63.4539863589064,12.5361131462324));
#80232=CARTESIAN_POINT('Ctrl Pts',(89.6662852330027,63.4585709271207,12.4766492128819));
#80233=CARTESIAN_POINT('Ctrl Pts',(89.6801268988914,63.4631554953349,12.4161875550014));
#80234=CARTESIAN_POINT('Ctrl Pts',(89.6906400536717,63.4677400635492,12.3551091933886));
#80235=CARTESIAN_POINT('Ctrl Pts',(89.7011467830677,63.4723218297869,12.2940681613835));
#80236=CARTESIAN_POINT('Ctrl Pts',(89.7083289489158,63.4769035960247,12.2324116736439));
#80237=CARTESIAN_POINT('Ctrl Pts',(89.7121313667431,63.4814853622625,12.1705318548713));
#80238=CARTESIAN_POINT('Ctrl Pts',(89.7159328572555,63.4860660111217,12.1086671270431));
#80239=CARTESIAN_POINT('Ctrl Pts',(89.7163562047732,63.490646659981,12.0465796841666));
#80240=CARTESIAN_POINT('Ctrl Pts',(89.7133981785168,63.4952273088402,11.9846656445125));
#80241=CARTESIAN_POINT('Ctrl Pts',(89.7103332757384,63.49997346124,11.9205145871154));
#80242=CARTESIAN_POINT('Ctrl Pts',(89.7036379391208,63.5047196136398,11.8565502871672));
#80243=CARTESIAN_POINT('Ctrl Pts',(89.693367431562,63.5094657660396,11.793209492798));
#80244=CARTESIAN_POINT('Ctrl Pts',(89.6834425112015,63.514052217519,11.7320000213007));
#80245=CARTESIAN_POINT('Ctrl Pts',(89.670179395771,63.5186386689983,11.6713732593582));
#80246=CARTESIAN_POINT('Ctrl Pts',(89.6536799050908,63.5232251204777,11.61171202414));
#80247=CARTESIAN_POINT('Ctrl Pts',(89.6363186423432,63.5280511233377,11.548934669339));
#80248=CARTESIAN_POINT('Ctrl Pts',(89.6153738562178,63.5328771261977,11.4872270800027));
#80249=CARTESIAN_POINT('Ctrl Pts',(89.5910223117948,63.5377031290578,11.4270130440841));
#80250=CARTESIAN_POINT('Ctrl Pts',(89.5666707673718,63.5425291319178,11.3667990081655));
#80251=CARTESIAN_POINT('Ctrl Pts',(89.5389128115545,63.5473551347778,11.3080790784421));
#80252=CARTESIAN_POINT('Ctrl Pts',(89.5079803849733,63.5521811376379,11.2512457041505));
#80253=CARTESIAN_POINT('Ctrl Pts',(89.4785142705607,63.5567783699971,11.1971064433675));
#80254=CARTESIAN_POINT('Ctrl Pts',(89.4460469112061,63.5613756023564,11.1444566023782));
#80255=CARTESIAN_POINT('Ctrl Pts',(89.4107531490587,63.5659728347156,11.0936492622));
#80256=CARTESIAN_POINT('Ctrl Pts',(89.3748551385258,63.5706487741909,11.0419720727507));
#80257=CARTESIAN_POINT('Ctrl Pts',(89.3360332053818,63.5753247136661,10.9922015782452));
#80258=CARTESIAN_POINT('Ctrl Pts',(89.2945206623623,63.5800006531413,10.9446840120247));
#80259=CARTESIAN_POINT('Ctrl Pts',(89.2538191386571,63.5845852400529,10.8980947836311));
#80260=CARTESIAN_POINT('Ctrl Pts',(89.2105315420466,63.5891698269645,10.8536716471459));
#80261=CARTESIAN_POINT('Ctrl Pts',(89.1649204445675,63.5937544138761,10.8117103830418));
#80262=CARTESIAN_POINT('Ctrl Pts',(89.1193372248128,63.598336198666,10.7697747658661));
#80263=CARTESIAN_POINT('Ctrl Pts',(89.0714336939611,63.6029179834558,10.7302983813848));
#80264=CARTESIAN_POINT('Ctrl Pts',(89.0215093541727,63.6074997682456,10.6935402808354));
#80265=CARTESIAN_POINT('Ctrl Pts',(88.9715971915321,63.6120804354829,10.6567911460294));
#80266=CARTESIAN_POINT('Ctrl Pts',(88.9196656081722,63.6166611027203,10.6227592806352));
#80267=CARTESIAN_POINT('Ctrl Pts',(88.8660456409869,63.6212417699576,10.5916622546278));
#80268=CARTESIAN_POINT('Ctrl Pts',(88.8104887636248,63.6259879043046,10.5594419130104));
#80269=CARTESIAN_POINT('Ctrl Pts',(88.7531196593087,63.6307340386515,10.5303728470156));
#80270=CARTESIAN_POINT('Ctrl Pts',(88.6943352168073,63.6354801729985,10.5046455184453));
#80271=CARTESIAN_POINT('Ctrl Pts',(88.6375283469838,63.6400666422162,10.4797836852322));
#80272=CARTESIAN_POINT('Ctrl Pts',(88.5794003798237,63.6446531114339,10.4580424230845));
#80273=CARTESIAN_POINT('Ctrl Pts',(88.5203281570851,63.6492395806516,10.4395438327455));
#80274=CARTESIAN_POINT('Ctrl Pts',(88.4581712824178,63.6540655475632,10.420079277191));
#80275=CARTESIAN_POINT('Ctrl Pts',(88.3949694553103,63.6588915144748,10.4042055000808));
#80276=CARTESIAN_POINT('Ctrl Pts',(88.3311745735203,63.6637174813864,10.3920038596009));
#80277=CARTESIAN_POINT('Ctrl Pts',(88.2673796917304,63.668543448298,10.379802219121));
#80278=CARTESIAN_POINT('Ctrl Pts',(88.2029924077756,63.6733694152096,10.3712727236636));
#80279=CARTESIAN_POINT('Ctrl Pts',(88.1384682187076,63.6781953821212,10.366433382059));
#80280=CARTESIAN_POINT('Ctrl Pts',(88.0770020850411,63.6827926274573,10.3618233959092));
#80281=CARTESIAN_POINT('Ctrl Pts',(88.0151593784975,63.6873898727934,10.3605427020705));
#80282=CARTESIAN_POINT('Ctrl Pts',(87.9533315665747,63.6919871181294,10.3626359204837));
#80283=CARTESIAN_POINT('Ctrl Pts',(87.8904454282439,63.6966630559826,10.3647649691853));
#80284=CARTESIAN_POINT('Ctrl Pts',(87.8275752209313,63.7013389938357,10.3703846559915));
#80285=CARTESIAN_POINT('Ctrl Pts',(87.7651383693305,63.7060149316888,10.3794867643079));
#80286=CARTESIAN_POINT('Ctrl Pts',(87.7039211269101,63.7105995321893,10.3884110767462));
#80287=CARTESIAN_POINT('Ctrl Pts',(87.6431209903504,63.7151841326898,10.4006829093132));
#80288=CARTESIAN_POINT('Ctrl Pts',(87.5831288716814,63.7197687331902,10.4162420986244));
#80289=CARTESIAN_POINT('Ctrl Pts',(87.5231734179149,63.7243505317572,10.4317917787505));
#80290=CARTESIAN_POINT('Ctrl Pts',(87.4640254945627,63.7289323303241,10.4506247043206));
#80291=CARTESIAN_POINT('Ctrl Pts',(87.4060651872506,63.733514128891,10.4726297643285));
#80292=CARTESIAN_POINT('Ctrl Pts',(87.3481190150353,63.7380948100697,10.4946294578422));
#80293=CARTESIAN_POINT('Ctrl Pts',(87.2913603595842,63.7426754912483,10.5197995694711));
#80294=CARTESIAN_POINT('Ctrl Pts',(87.2361515614434,63.747256172427,10.5479799958938));
#80295=CARTESIAN_POINT('Ctrl Pts',(87.1789487926766,63.7520022936085,10.5771782119517));
#80296=CARTESIAN_POINT('Ctrl Pts',(87.1234105231449,63.7567484147899,10.6096081442033));
#80297=CARTESIAN_POINT('Ctrl Pts',(87.0699120307322,63.7614945359714,10.6450396663878));
#80298=CARTESIAN_POINT('Ctrl Pts',(87.0182129826056,63.7660810193713,10.6792794344261));
#80299=CARTESIAN_POINT('Ctrl Pts',(86.9684190441821,63.7706675027713,10.7163216925554));
#80300=CARTESIAN_POINT('Ctrl Pts',(86.9208371947618,63.7752539861712,10.7559160738047));
#80301=CARTESIAN_POINT('Ctrl Pts',(86.8707711346017,63.7800799262434,10.7975776463956));
#80302=CARTESIAN_POINT('Ctrl Pts',(86.8231549564592,63.7849058663156,10.8420647046982));
#80303=CARTESIAN_POINT('Ctrl Pts',(86.7783021135038,63.7897318063878,10.8890417355625));
#80304=CARTESIAN_POINT('Ctrl Pts',(86.7334492705484,63.79455774646,10.9360187664268));
#80305=CARTESIAN_POINT('Ctrl Pts',(86.6913601237379,63.7993836865322,10.9854852262386));
#80306=CARTESIAN_POINT('Ctrl Pts',(86.6522968591971,63.8042096266043,11.0370682186013));
#80307=CARTESIAN_POINT('Ctrl Pts',(86.6149869464817,63.8088189547027,11.0863359120538));
#80308=CARTESIAN_POINT('Ctrl Pts',(86.580282212688,63.8134282828011,11.1377385149235));
#80309=CARTESIAN_POINT('Ctrl Pts',(86.5484343454252,63.8180376108995,11.1909705481196));
#80310=CARTESIAN_POINT('Ctrl Pts',(86.5166358475953,63.8226397937812,11.244120062908));
#80311=CARTESIAN_POINT('Ctrl Pts',(86.4876856912155,63.8272419766628,11.2990929549601));
#80312=CARTESIAN_POINT('Ctrl Pts',(86.4617940000144,63.8318441595444,11.3555525317038));
#80313=CARTESIAN_POINT('Ctrl Pts',(86.4359346122434,63.8364406005728,11.4119416673944));
#80314=CARTESIAN_POINT('Ctrl Pts',(86.4131263256213,63.8410370416011,11.4698133498059));
#80315=CARTESIAN_POINT('Ctrl Pts',(86.3935337383234,63.8456334826294,11.5288056888443));
#80316=CARTESIAN_POINT('Ctrl Pts',(86.3739560463781,63.8502264291927,11.5877531786919));
#80317=CARTESIAN_POINT('Ctrl Pts',(86.3575893621039,63.8548193757561,11.6478191568059));
#80318=CARTESIAN_POINT('Ctrl Pts',(86.3445497596784,63.8594123223195,11.7086228432984));
#80319=CARTESIAN_POINT('Ctrl Pts',(86.3315110747425,63.864004945715,11.7694222515353));
#80320=CARTESIAN_POINT('Ctrl Pts',(86.3217991299969,63.8685975691104,11.8309587750666));
#80321=CARTESIAN_POINT('Ctrl Pts',(86.3154793842121,63.8731901925059,11.892839158473));
#80322=CARTESIAN_POINT('Ctrl Pts',(86.3095624341705,63.8774901001472,11.9507755295932));
#80323=CARTESIAN_POINT('Ctrl Pts',(86.3066186245782,63.8817900077885,12.0090128773501));
#80324=CARTESIAN_POINT('Ctrl Pts',(86.3066604397209,63.8860899154298,12.0672242824529));
#80325=CARTESIAN_POINT('Ctrl Pts',(86.3066604397214,63.8860899154862,12.067224283217));
#80326=CARTESIAN_POINT('Ctrl Pts',(86.3067115579032,63.8913464639361,12.1383865259391));
#80327=CARTESIAN_POINT('Ctrl Pts',(86.3112236097562,63.896603012386,12.2093698792769));
#80328=CARTESIAN_POINT('Ctrl Pts',(86.3201057341301,63.9018595608358,12.2796619227856));
#80329=CARTESIAN_POINT('Ctrl Pts',(86.3290710981618,63.9071653715202,12.350612714742));
#80330=CARTESIAN_POINT('Ctrl Pts',(86.3424887120832,63.9124711822046,12.4208589876627));
#80331=CARTESIAN_POINT('Ctrl Pts',(86.3602155595618,63.917776992889,12.4898933436694));
#80332=CARTESIAN_POINT('Ctrl Pts',(86.374077337685,63.9219259522885,12.5438758087973));
#80333=CARTESIAN_POINT('Ctrl Pts',(86.3905730726722,63.926074911688,12.5971175918686));
#80334=CARTESIAN_POINT('Ctrl Pts',(86.409614244658,63.9302238710876,12.6493853770775));
#80335=CARTESIAN_POINT('Ctrl Pts',(86.4307130937734,63.934821186233,12.7073014609478));
#80336=CARTESIAN_POINT('Ctrl Pts',(86.4550012082824,63.9394185013784,12.7641903405576));
#80337=CARTESIAN_POINT('Ctrl Pts',(86.4823581174278,63.9440158165238,12.819676874029));
#80338=CARTESIAN_POINT('Ctrl Pts',(86.5101828290803,63.9486917456508,12.8761122259262));
#80339=CARTESIAN_POINT('Ctrl Pts',(86.5411821822989,63.9533676747777,12.9310962899627));
#80340=CARTESIAN_POINT('Ctrl Pts',(86.5751768783403,63.9580436039047,12.984252034524));
#80341=CARTESIAN_POINT('Ctrl Pts',(86.6085080940721,63.9626282721214,13.0363703293074));
#80342=CARTESIAN_POINT('Ctrl Pts',(86.6447184943683,63.9672129403381,13.0867305814165));
#80343=CARTESIAN_POINT('Ctrl Pts',(86.6835923425951,63.9717976085548,13.1350012846871));
#80344=CARTESIAN_POINT('Ctrl Pts',(86.7224424248471,63.9763794738818,13.1832424771074));
#80345=CARTESIAN_POINT('Ctrl Pts',(86.7639524076726,63.9809613392088,13.2293962581041));
#80346=CARTESIAN_POINT('Ctrl Pts',(86.8078645788163,63.9855432045358,13.2731619584352));
#80347=CARTESIAN_POINT('Ctrl Pts',(86.851766030899,63.990123951419,13.3169169754592));
#80348=CARTESIAN_POINT('Ctrl Pts',(86.8980681468718,63.9947046983023,13.3582847098619));
#80349=CARTESIAN_POINT('Ctrl Pts',(86.9464758684385,63.9992854451855,13.3970008297981));
#80350=CARTESIAN_POINT('Ctrl Pts',(86.9966305171738,64.0040315010509,13.437114128523));
#80351=CARTESIAN_POINT('Ctrl Pts',(87.0490452375039,64.0087775569164,13.4743803574942));
#80352=CARTESIAN_POINT('Ctrl Pts',(87.103355859577,64.0135236127818,13.5085522347408));
#80353=CARTESIAN_POINT('Ctrl Pts',(87.1558411568784,64.0181101585366,13.5415756299474));
#80354=CARTESIAN_POINT('Ctrl Pts',(87.2100964340709,64.0226967042913,13.571709190194));
#80355=CARTESIAN_POINT('Ctrl Pts',(87.2657671565741,64.027283250046,13.598776188711));
#80356=CARTESIAN_POINT('Ctrl Pts',(87.3243420395011,64.0321090609668,13.6272551844564));
#80357=CARTESIAN_POINT('Ctrl Pts',(87.3844835014319,64.0369348718876,13.6523386513244));
#80358=CARTESIAN_POINT('Ctrl Pts',(87.4457567944024,64.0417606828084,13.6738790234734));
#80359=CARTESIAN_POINT('Ctrl Pts',(87.5070300873729,64.0465864937292,13.6954193956224));
#80360=CARTESIAN_POINT('Ctrl Pts',(87.5694345675354,64.05141230465,13.7134165678344));
#80361=CARTESIAN_POINT('Ctrl Pts',(87.6325225185108,64.0562381155708,13.7277850738304));
#80362=CARTESIAN_POINT('Ctrl Pts',(87.6926238497539,64.0608354698386,13.7414733665232));
#80363=CARTESIAN_POINT('Ctrl Pts',(87.7535920397938,64.0654328241065,13.7519250364605));
#80364=CARTESIAN_POINT('Ctrl Pts',(87.8150465687771,64.0700301783744,13.7590378283996));
#80365=CARTESIAN_POINT('Ctrl Pts',(87.8775513714924,64.074706102611,13.7662721797853));
#80366=CARTESIAN_POINT('Ctrl Pts',(87.9405587967322,64.0793820268477,13.7700522461079));
#80367=CARTESIAN_POINT('Ctrl Pts',(88.0036548428794,64.0840579510843,13.7703241722944));
#80368=CARTESIAN_POINT('Ctrl Pts',(88.0655200941409,64.0886426635258,13.7705907941015));
#80369=CARTESIAN_POINT('Ctrl Pts',(88.1274700066235,64.0932273759673,13.767484909079));
#80370=CARTESIAN_POINT('Ctrl Pts',(88.1891090515675,64.0978120884088,13.7610079649812));
#80371=CARTESIAN_POINT('Ctrl Pts',(88.2507104367725,64.1023939997188,13.7545349781158));
#80372=CARTESIAN_POINT('Ctrl Pts',(88.3120008258701,64.1069759110287,13.7446950692036));
#80373=CARTESIAN_POINT('Ctrl Pts',(88.372587831095,64.1115578223386,13.7315416764536));
#80374=CARTESIAN_POINT('Ctrl Pts',(88.4331600690939,64.1161386168725,13.7183914896572));
#80375=CARTESIAN_POINT('Ctrl Pts',(88.4930287663523,64.1207194114063,13.7019295302079));
#80376=CARTESIAN_POINT('Ctrl Pts',(88.5518118080388,64.1253002059401,13.6822603205814));
#80377=CARTESIAN_POINT('Ctrl Pts',(88.6127150135252,64.130046218783,13.6618816895805));
#80378=CARTESIAN_POINT('Ctrl Pts',(88.6724521808621,64.1347922316258,13.6380601538275));
#80379=CARTESIAN_POINT('Ctrl Pts',(88.7306180579729,64.1395382444686,13.6109675356587));
#80380=CARTESIAN_POINT('Ctrl Pts',(88.7868301759858,64.1441248414094,13.5847849432965));
#80381=CARTESIAN_POINT('Ctrl Pts',(88.8415744630186,64.1487114383501,13.5555478589231));
#80382=CARTESIAN_POINT('Ctrl Pts',(88.8945101450594,64.1532980352908,13.5234582872855));
#80383=CARTESIAN_POINT('Ctrl Pts',(88.9502056475994,64.1581237560847,13.4896957144849));
#80384=CARTESIAN_POINT('Ctrl Pts',(89.0038982612178,64.1629494768786,13.4527754365747));
#80385=CARTESIAN_POINT('Ctrl Pts',(89.0552282352508,64.1677751976725,13.4129826384571));
#80386=CARTESIAN_POINT('Ctrl Pts',(89.1065582092839,64.1726009184663,13.3731898403395));
#80387=CARTESIAN_POINT('Ctrl Pts',(89.1555251062022,64.1774266392602,13.3305250057805));
#80388=CARTESIAN_POINT('Ctrl Pts',(89.2018143077068,64.1822523600541,13.2853178913477));
#80389=CARTESIAN_POINT('Ctrl Pts',(89.2459054887831,64.1868489338214,13.2422574149602));
#80390=CARTESIAN_POINT('Ctrl Pts',(89.2877486809983,64.1914455075887,13.1967137742867));
#80391=CARTESIAN_POINT('Ctrl Pts',(89.3270516149251,64.196042081356,13.148951052658));
#80392=CARTESIAN_POINT('Ctrl Pts',(89.3670338680375,64.2007181031553,13.1003627913069));
#80393=CARTESIAN_POINT('Ctrl Pts',(89.4043867701727,64.2053941249545,13.0494783130407));
#80394=CARTESIAN_POINT('Ctrl Pts',(89.4388403952444,64.2100701467537,12.9966162696345));
#80395=CARTESIAN_POINT('Ctrl Pts',(89.4726154597161,64.2146540747848,12.9447953387328));
#80396=CARTESIAN_POINT('Ctrl Pts',(89.5036041219738,64.2192380028159,12.8910744794241));
#80397=CARTESIAN_POINT('Ctrl Pts',(89.5315930892139,64.2238219308471,12.835786653973));
#80398=CARTESIAN_POINT('Ctrl Pts',(89.5595649573351,64.2284030584487,12.7805326051557));
#80399=CARTESIAN_POINT('Ctrl Pts',(89.5845405346355,64.2329841860503,12.7237139417204));
#80400=CARTESIAN_POINT('Ctrl Pts',(89.6063519077611,64.2375653136519,12.6656891911675));
#80401=CARTESIAN_POINT('Ctrl Pts',(89.6281579731013,64.2421453264387,12.6076785609048));
#80402=CARTESIAN_POINT('Ctrl Pts',(89.6468011837455,64.2467253392255,12.548462902594));
#80403=CARTESIAN_POINT('Ctrl Pts',(89.6621621144506,64.2513053520123,12.4884198236389));
#80404=CARTESIAN_POINT('Ctrl Pts',(89.6780823366137,64.256052123056,12.4261905762921));
#80405=CARTESIAN_POINT('Ctrl Pts',(89.6904764459661,64.2607988940998,12.3630730413557));
#80406=CARTESIAN_POINT('Ctrl Pts',(89.6992689453396,64.2655456651435,12.2995011858686));
#80407=CARTESIAN_POINT('Ctrl Pts',(89.7077633300022,64.2701314942051,12.2380847704347));
#80408=CARTESIAN_POINT('Ctrl Pts',(89.7128964682595,64.2747173232667,12.176244883587));
#80409=CARTESIAN_POINT('Ctrl Pts',(89.7146532730937,64.2793031523283,12.1143772743872));
#80410=CARTESIAN_POINT('Ctrl Pts',(89.7165025618545,64.2841303943632,12.0492527527987));
#80411=CARTESIAN_POINT('Ctrl Pts',(89.7146102193961,64.288957636398,11.9840981549112));
#80412=CARTESIAN_POINT('Ctrl Pts',(89.7090208327119,64.2937848784328,11.9193709194039));
#80413=CARTESIAN_POINT('Ctrl Pts',(89.7034314460276,64.2986121204676,11.8546436838966));
#80414=CARTESIAN_POINT('Ctrl Pts',(89.6941451849246,64.3034393625024,11.7903444424305));
#80415=CARTESIAN_POINT('Ctrl Pts',(89.6812686762512,64.3082666045373,11.7269168468735));
#80416=CARTESIAN_POINT('Ctrl Pts',(89.669003364973,64.3128647163138,11.6664999106631));
#80417=CARTESIAN_POINT('Ctrl Pts',(89.653430589109,64.3174628280904,11.6066254977153));
#80418=CARTESIAN_POINT('Ctrl Pts',(89.6346138356892,64.322060939867,11.5476825797268));
#80419=CARTESIAN_POINT('Ctrl Pts',(89.6154790395132,64.326736769415,11.4877434023053));
#80420=CARTESIAN_POINT('Ctrl Pts',(89.5929895988853,64.3314125989631,11.428768039135));
#80421=CARTESIAN_POINT('Ctrl Pts',(89.5672668221473,64.3360884285111,11.3711558348209));
#80422=CARTESIAN_POINT('Ctrl Pts',(89.5420412208347,64.3406738826084,11.3146571717266));
#80423=CARTESIAN_POINT('Ctrl Pts',(89.5137063783026,64.3452593367056,11.259469927865));
#80424=CARTESIAN_POINT('Ctrl Pts',(89.482426458777,64.3498447908028,11.2059540640111));
#80425=CARTESIAN_POINT('Ctrl Pts',(89.4511657010337,64.3544274358943,11.1524709834684));
#80426=CARTESIAN_POINT('Ctrl Pts',(89.4169636999067,64.3590100809858,11.1006576911016));
#80427=CARTESIAN_POINT('Ctrl Pts',(89.3800307091691,64.3635927260773,11.0508498864937));
#80428=CARTESIAN_POINT('Ctrl Pts',(89.343106791367,64.368174245399,11.0010543176401));
#80429=CARTESIAN_POINT('Ctrl Pts',(89.3034535187289,64.3727557647208,10.9532636670647));
#80430=CARTESIAN_POINT('Ctrl Pts',(89.2613234747187,64.3773372840426,10.9077832481926));
#80431=CARTESIAN_POINT('Ctrl Pts',(89.2176873879003,64.3820825811241,10.8606770190616));
#80432=CARTESIAN_POINT('Ctrl Pts',(89.1713944443903,64.3868278782055,10.816049791169));
#80433=CARTESIAN_POINT('Ctrl Pts',(89.1227677915072,64.391573175287,10.7742000103084));
#80434=CARTESIAN_POINT('Ctrl Pts',(89.0757602773068,64.3961604665505,10.7337437162506));
#80435=CARTESIAN_POINT('Ctrl Pts',(89.0265724969234,64.400747757814,10.6958830645894));
#80436=CARTESIAN_POINT('Ctrl Pts',(88.975528858915,64.4053350490775,10.660845590008));
#80437=CARTESIAN_POINT('Ctrl Pts',(88.9218479809821,64.410159349068,10.6239978560009));
#80438=CARTESIAN_POINT('Ctrl Pts',(88.8661148135088,64.4149836490585,10.5902732849022));
#80439=CARTESIAN_POINT('Ctrl Pts',(88.8087368562257,64.419807949049,10.5598822277727));
#80440=CARTESIAN_POINT('Ctrl Pts',(88.7513588989427,64.4246322490395,10.5294911706431));
#80441=CARTESIAN_POINT('Ctrl Pts',(88.6923367711396,64.42945654903,10.5024338269264));
#80442=CARTESIAN_POINT('Ctrl Pts',(88.6321000033795,64.4342808490205,10.4788611839534));
#80443=CARTESIAN_POINT('Ctrl Pts',(88.5746901027678,64.4388787481654,10.4563947877545));
#80444=CARTESIAN_POINT('Ctrl Pts',(88.5159421840625,64.4434766473103,10.4370013802393));
#80445=CARTESIAN_POINT('Ctrl Pts',(88.4562174867713,64.4480745464552,10.4208385413361));
#80446=CARTESIAN_POINT('Ctrl Pts',(88.3954801624058,64.4527504025822,10.404401662898));
#80447=CARTESIAN_POINT('Ctrl Pts',(88.3337330873303,64.4574262587092,10.3913062036751));
#80448=CARTESIAN_POINT('Ctrl Pts',(88.2713776271557,64.4621021148362,10.3816668005182));
#80449=CARTESIAN_POINT('Ctrl Pts',(88.2102300152025,64.4666873979085,10.3722141161493));
#80450=CARTESIAN_POINT('Ctrl Pts',(88.148497904085,64.4712726809809,10.3660848723485));
#80451=CARTESIAN_POINT('Ctrl Pts',(88.0865727498605,64.4758579640532,10.363336323557));
#80452=CARTESIAN_POINT('Ctrl Pts',(88.0246853185018,64.4804404539145,10.3605894490953));
#80453=CARTESIAN_POINT('Ctrl Pts',(87.9626055845292,64.4850229437759,10.361219208585));
#80454=CARTESIAN_POINT('Ctrl Pts',(87.9007296089269,64.4896054336373,10.3652309749844));
#80455=CARTESIAN_POINT('Ctrl Pts',(87.8388686195203,64.4941868136319,10.3692417697447));
#80456=CARTESIAN_POINT('Ctrl Pts',(87.7772117980863,64.4987681936265,10.3766329124122));
#80457=CARTESIAN_POINT('Ctrl Pts',(87.7161526250997,64.5033495736211,10.3873577328345));
#80458=CARTESIAN_POINT('Ctrl Pts',(87.6529066462057,64.5080950336113,10.3984666577167));
#80459=CARTESIAN_POINT('Ctrl Pts',(87.5903025204143,64.5128404936015,10.4131525448178));
#80460=CARTESIAN_POINT('Ctrl Pts',(87.5287662939644,64.5175859535917,10.4313056896278));
#80461=CARTESIAN_POINT('Ctrl Pts',(87.4692823831931,64.5221731461271,10.4488534027132));
#80462=CARTESIAN_POINT('Ctrl Pts',(87.4107967292947,64.5267603386625,10.4696404779147));
#80463=CARTESIAN_POINT('Ctrl Pts',(87.3536764029595,64.5313475311979,10.4935177188999));
#80464=CARTESIAN_POINT('Ctrl Pts',(87.2935999257984,64.5361721249155,10.5186306798151));
#80465=CARTESIAN_POINT('Ctrl Pts',(87.2350345197086,64.5409967186332,10.5471620804812));
#80466=CARTESIAN_POINT('Ctrl Pts',(87.1783779586482,64.5458213123508,10.5788835378979));
#80467=CARTESIAN_POINT('Ctrl Pts',(87.1217213975878,64.5506459060684,10.6106049953145));
#80468=CARTESIAN_POINT('Ctrl Pts',(87.0669741850425,64.5554704997861,10.6455160969614));
#80469=CARTESIAN_POINT('Ctrl Pts',(87.0144961418063,64.5602950935037,10.6833377504954));
#80470=CARTESIAN_POINT('Ctrl Pts',(86.9649314865339,64.5648518435214,10.7190596849206));
#80471=CARTESIAN_POINT('Ctrl Pts',(86.9171792470767,64.569408593539,10.7575301788349));
#80472=CARTESIAN_POINT('Ctrl Pts',(86.8715645979647,64.5739653435567,10.7985372588559));
#80473=CARTESIAN_POINT('Ctrl Pts',(86.8260299695178,64.5785140997791,10.8394724011576));
#80474=CARTESIAN_POINT('Ctrl Pts',(86.7826258723447,64.5830628560014,10.8829349551343));
#80475=CARTESIAN_POINT('Ctrl Pts',(86.7416468352425,64.5876116122238,10.9286709452756));
#80476=CARTESIAN_POINT('Ctrl Pts',(86.7007077913486,64.592155929119,10.9743622996933));
#80477=CARTESIAN_POINT('Ctrl Pts',(86.6621894639922,64.5967002460141,11.0223223109148));
#80478=CARTESIAN_POINT('Ctrl Pts',(86.626350443695,64.6012445629093,11.0722593689375));
#80479=CARTESIAN_POINT('Ctrl Pts',(86.5905326579707,64.6057861873026,11.1221668393184));
#80480=CARTESIAN_POINT('Ctrl Pts',(86.5573913350624,64.6103278116959,11.1740486141513));
#80481=CARTESIAN_POINT('Ctrl Pts',(86.5271441651915,64.6148694360892,11.2275808344839));
#80482=CARTESIAN_POINT('Ctrl Pts',(86.4969033197675,64.6194101108643,11.2811018616473));
#80483=CARTESIAN_POINT('Ctrl Pts',(86.4695556810674,64.6239507856394,11.3362721974733));
#80484=CARTESIAN_POINT('Ctrl Pts',(86.4452739044528,64.6284914604146,11.3927417810954));
#80485=CARTESIAN_POINT('Ctrl Pts',(86.4209711114364,64.6330360652417,11.4492602403611));
#80486=CARTESIAN_POINT('Ctrl Pts',(86.3997396873906,64.6375806700689,11.5070797162322));
#80487=CARTESIAN_POINT('Ctrl Pts',(86.3817042747851,64.642125274896,11.5658297535875));
#80488=CARTESIAN_POINT('Ctrl Pts',(86.3636611137683,64.6466718321857,11.6246050312552));
#80489=CARTESIAN_POINT('Ctrl Pts',(86.3488168244642,64.6512183894753,11.6843111623066));
#80490=CARTESIAN_POINT('Ctrl Pts',(86.3372453945193,64.655764946765,11.7445651602077));
#80491=CARTESIAN_POINT('Ctrl Pts',(86.3256530493151,64.6603197219176,11.8049280666883));
#80492=CARTESIAN_POINT('Ctrl Pts',(86.3173454475435,64.6648744970702,11.8658403024834));
#80493=CARTESIAN_POINT('Ctrl Pts',(86.3123448009796,64.6694292722228,11.9269124360668));
#80494=CARTESIAN_POINT('Ctrl Pts',(86.3085348838982,64.6728994866108,11.9734423721382));
#80495=CARTESIAN_POINT('Ctrl Pts',(86.3066434735053,64.6763697009989,12.0200649769014));
#80496=CARTESIAN_POINT('Ctrl Pts',(86.3066601088578,64.6798399153869,12.0666091481311));
#80497=CARTESIAN_POINT('Origin',(88.011,66.41344859951,12.066));
#80498=CARTESIAN_POINT('',(88.2080236424798,49.5646,13.3206241207246));
#80499=CARTESIAN_POINT('Ctrl Pts',(88.2080236424798,49.5646,13.3206241207246));
#80500=CARTESIAN_POINT('Ctrl Pts',(88.2097267967144,49.5647720436039,13.3203566608173));
#80501=CARTESIAN_POINT('Ctrl Pts',(88.2114293848816,49.5649442914476,13.3200857362535));
#80502=CARTESIAN_POINT('Ctrl Pts',(88.2180820755138,49.5656183417018,13.3190132321809));
#80503=CARTESIAN_POINT('Ctrl Pts',(88.2230278040899,49.5661216278726,13.3181858300697));
#80504=CARTESIAN_POINT('Ctrl Pts',(88.23517546855,49.5673629764069,13.3160795429129));
#80505=CARTESIAN_POINT('Ctrl Pts',(88.24237135194,49.5681027991327,13.314767709552));
#80506=CARTESIAN_POINT('Ctrl Pts',(88.2684291775434,49.5707972735995,13.3097843361335));
#80507=CARTESIAN_POINT('Ctrl Pts',(88.2872170891576,49.572769374158,13.3057472475379));
#80508=CARTESIAN_POINT('Ctrl Pts',(88.3236804028145,49.5766462220168,13.2970422258303));
#80509=CARTESIAN_POINT('Ctrl Pts',(88.3413616954967,49.5785491700862,13.2924155353734));
#80510=CARTESIAN_POINT('Ctrl Pts',(88.3592479869665,49.5804945016824,13.2873203694679));
#80511=CARTESIAN_POINT('Ctrl Pts',(88.3595600417179,49.5805284474264,13.2872313468875));
#80512=CARTESIAN_POINT('Ctrl Pts',(88.3602208395918,49.5806003433312,13.2870425614078));
#80513=CARTESIAN_POINT('Ctrl Pts',(88.3605695741056,49.5806382941348,13.2869427686971));
#80514=CARTESIAN_POINT('Ctrl Pts',(88.3613076933374,49.5807186361706,13.2867312087848));
#80515=CARTESIAN_POINT('Ctrl Pts',(88.3616970673495,49.5807610281884,13.2866194046731));
#80516=CARTESIAN_POINT('Ctrl Pts',(88.4253992750408,49.5876980346645,13.2682950768527));
#80517=CARTESIAN_POINT('Ctrl Pts',(88.4871985938793,49.5946799449541,13.2451841330288));
#80518=CARTESIAN_POINT('Ctrl Pts',(88.6039655922378,49.6081902466906,13.1908333883167));
#80519=CARTESIAN_POINT('Ctrl Pts',(88.6589629424759,49.6147072468449,13.1600773964497));
#80520=CARTESIAN_POINT('Ctrl Pts',(88.7272693192359,49.6230072425402,13.1149124474686));
#80521=CARTESIAN_POINT('Ctrl Pts',(88.742840582761,49.6249149311283,13.1041081447339));
#80522=CARTESIAN_POINT('Ctrl Pts',(88.7665779572615,49.6278498719295,13.0868379820414));
#80523=CARTESIAN_POINT('Ctrl Pts',(88.7749153990046,49.6288860402733,13.0806139731869));
#80524=CARTESIAN_POINT('Ctrl Pts',(88.7902467120687,49.6308019513485,13.0688728156558));
#80525=CARTESIAN_POINT('Ctrl Pts',(88.7972607507153,49.6316826818768,13.0633832586405));
#80526=CARTESIAN_POINT('Ctrl Pts',(88.8127417394313,49.6336365544447,13.0510022054533));
#80527=CARTESIAN_POINT('Ctrl Pts',(88.8211788486992,49.6347081970147,13.0440743389822));
#80528=CARTESIAN_POINT('Ctrl Pts',(88.8424392148344,49.6374273553418,13.0261531501222));
#80529=CARTESIAN_POINT('Ctrl Pts',(88.8551347783218,49.6390688961246,13.0150109469476));
#80530=CARTESIAN_POINT('Ctrl Pts',(88.9327304991544,49.6492285974841,12.9441197426848));
#80531=CARTESIAN_POINT('Ctrl Pts',(88.9914838492493,49.6574651478001,12.8779949834701));
#80532=CARTESIAN_POINT('Ctrl Pts',(89.0820913064662,49.6720721464964,12.751696996699));
#80533=CARTESIAN_POINT('Ctrl Pts',(89.1168643005801,49.6784030292887,12.6940745755641));
#80534=CARTESIAN_POINT('Ctrl Pts',(89.1518942754838,49.6860669652867,12.6240183029856));
#80535=CARTESIAN_POINT('Ctrl Pts',(89.1567462445896,49.6871636958455,12.6139869404145));
#80536=CARTESIAN_POINT('Ctrl Pts',(89.1639489257088,49.6888490569957,12.5985816003658));
#80537=CARTESIAN_POINT('Ctrl Pts',(89.1663956380392,49.6894322529589,12.5932525969323));
#80538=CARTESIAN_POINT('Ctrl Pts',(89.1706709432374,49.6904709118824,12.5837682049443));
#80539=CARTESIAN_POINT('Ctrl Pts',(89.1725142958538,49.6909254860735,12.5796196537934));
#80540=CARTESIAN_POINT('Ctrl Pts',(89.1768425177269,49.6920090955987,12.5697363248419));
#80541=CARTESIAN_POINT('Ctrl Pts',(89.1793072743075,49.6926392609403,12.5639931404312));
#80542=CARTESIAN_POINT('Ctrl Pts',(89.1866225910927,49.694549323352,12.5465943265912));
#80543=CARTESIAN_POINT('Ctrl Pts',(89.1913416025946,49.6958361342485,12.5348848916557));
#80544=CARTESIAN_POINT('Ctrl Pts',(89.2166700803913,49.7030520011094,12.4692300765583));
#80545=CARTESIAN_POINT('Ctrl Pts',(89.233753468218,49.7091209351502,12.4140043593033));
#80546=CARTESIAN_POINT('Ctrl Pts',(89.2582780324403,49.7203661131374,12.3101279387641));
#80547=CARTESIAN_POINT('Ctrl Pts',(89.2667683271879,49.7255303507395,12.2618249914497));
#80548=CARTESIAN_POINT('Ctrl Pts',(89.2768023995989,49.7345651663758,12.1758075580762));
#80549=CARTESIAN_POINT('Ctrl Pts',(89.2794986063008,49.7384533214004,12.1382864548802));
#80550=CARTESIAN_POINT('Ctrl Pts',(89.2808679774468,49.743574598978,12.0881821904661));
#80551=CARTESIAN_POINT('Ctrl Pts',(89.281024955551,49.7448484466321,12.0756627844987));
#80552=CARTESIAN_POINT('Ctrl Pts',(89.2809554966367,49.7479758956335,12.0447917202294));
#80553=CARTESIAN_POINT('Ctrl Pts',(89.2805164709481,49.7498228270648,12.0264427717425));
#80554=CARTESIAN_POINT('Ctrl Pts',(89.2792131731109,49.7526810803647,11.9978812628543));
#80555=CARTESIAN_POINT('Ctrl Pts',(89.2786228217866,49.7537006807676,11.9876596390929));
#80556=CARTESIAN_POINT('Ctrl Pts',(89.2772917453297,49.7555946032449,11.9686164517072));
#80557=CARTESIAN_POINT('Ctrl Pts',(89.2765822832286,49.7564698333374,11.9597934365416));
#80558=CARTESIAN_POINT('Ctrl Pts',(89.2747884997344,49.7584219338046,11.9400689662973));
#80559=CARTESIAN_POINT('Ctrl Pts',(89.2736552430741,49.7594972250645,11.9291725436642));
#80560=CARTESIAN_POINT('Ctrl Pts',(89.2703876841445,49.7622441576368,11.9012686428281));
#80561=CARTESIAN_POINT('Ctrl Pts',(89.268049767619,49.7639094681629,11.8842867470458));
#80562=CARTESIAN_POINT('Ctrl Pts',(89.251236965595,49.7742944310938,11.7781194541695));
#80563=CARTESIAN_POINT('Ctrl Pts',(89.2276228109176,49.7827121408086,11.6906398508275));
#80564=CARTESIAN_POINT('Ctrl Pts',(89.1771211686856,49.7957967287859,11.5605494805665));
#80565=CARTESIAN_POINT('Ctrl Pts',(89.1566764850031,49.800418142471,11.5157789811439));
#80566=CARTESIAN_POINT('Ctrl Pts',(89.1255005810498,49.8068177676603,11.4568240057862));
#80567=CARTESIAN_POINT('Ctrl Pts',(89.1169916844225,49.808510645063,11.4415088170721));
#80568=CARTESIAN_POINT('Ctrl Pts',(89.1017129321302,49.8114699739381,11.4153006511157));
#80569=CARTESIAN_POINT('Ctrl Pts',(89.0950895700466,49.8127288578755,11.4043247768336));
#80570=CARTESIAN_POINT('Ctrl Pts',(89.0850052107525,49.8146139431511,11.3881714403324));
#80571=CARTESIAN_POINT('Ctrl Pts',(89.0816700833126,49.8152324856734,11.3829155866702));
#80572=CARTESIAN_POINT('Ctrl Pts',(89.0756099051925,49.8163481584418,11.3735187200292));
#80573=CARTESIAN_POINT('Ctrl Pts',(89.0728990389651,49.816844362743,11.3693688195465));
#80574=CARTESIAN_POINT('Ctrl Pts',(89.0667387015753,49.8179656635505,11.3600578440382));
#80575=CARTESIAN_POINT('Ctrl Pts',(89.063275703445,49.8185916024393,11.3549062146613));
#80576=CARTESIAN_POINT('Ctrl Pts',(89.0525149978231,49.8205227854085,11.3391490906937));
#80577=CARTESIAN_POINT('Ctrl Pts',(89.0450940469585,49.8218354573217,11.3286295430065));
#80578=CARTESIAN_POINT('Ctrl Pts',(89.0009668713741,49.8295244803619,11.2680535275324));
#80579=CARTESIAN_POINT('Ctrl Pts',(88.9607943955332,49.8360640746927,11.2206352447754));
#80580=CARTESIAN_POINT('Ctrl Pts',(88.8664774014941,49.8502636790895,11.1245506705821));
#80581=CARTESIAN_POINT('Ctrl Pts',(88.8112764688783,49.8578970151876,11.0771980894698));
#80582=CARTESIAN_POINT('Ctrl Pts',(88.7248876936699,49.8688410286114,11.0150927181668));
#80583=CARTESIAN_POINT('Ctrl Pts',(88.696672564676,49.8722787828295,10.9964695262743));
#80584=CARTESIAN_POINT('Ctrl Pts',(88.6568307076361,49.8769567664032,10.9723980215661));
#80585=CARTESIAN_POINT('Ctrl Pts',(88.6458177159904,49.8782321354836,10.965968596664));
#80586=CARTESIAN_POINT('Ctrl Pts',(88.6268559678826,49.8803989406136,10.9552782961078));
#80587=CARTESIAN_POINT('Ctrl Pts',(88.6189555334498,49.8812933050731,10.9509343710858));
#80588=CARTESIAN_POINT('Ctrl Pts',(88.6038076589692,49.8829925504876,10.9428144210141));
#80589=CARTESIAN_POINT('Ctrl Pts',(88.5965687760746,49.8837979219343,10.9390235221062));
#80590=CARTESIAN_POINT('Ctrl Pts',(88.5795068212498,49.8856810675994,10.9302972090153));
#80591=CARTESIAN_POINT('Ctrl Pts',(88.5696551095875,49.8867568115958,10.9254188664166));
#80592=CARTESIAN_POINT('Ctrl Pts',(88.534802397185,49.8905238598128,10.9087205433447));
#80593=CARTESIAN_POINT('Ctrl Pts',(88.5094783147442,49.893191688466,10.8975889756812));
#80594=CARTESIAN_POINT('Ctrl Pts',(88.3979685283161,49.9046879380422,10.8528596554389));
#80595=CARTESIAN_POINT('Ctrl Pts',(88.3086236644899,49.9132397237372,10.8279064161989));
#80596=CARTESIAN_POINT('Ctrl Pts',(88.167010391284,49.9267384098283,10.8045864166829));
#80597=CARTESIAN_POINT('Ctrl Pts',(88.1162186372644,49.9315750897967,10.7993387370236));
#80598=CARTESIAN_POINT('Ctrl Pts',(88.0527885201105,49.9377692844856,10.7966263369692));
#80599=CARTESIAN_POINT('Ctrl Pts',(88.0403125399372,49.9389950426173,10.7962769953361));
#80600=CARTESIAN_POINT('Ctrl Pts',(88.0217112071195,49.9408365785735,10.7960304062589));
#80601=CARTESIAN_POINT('Ctrl Pts',(88.0155878327021,49.9414450493578,10.7959935256065));
#80602=CARTESIAN_POINT('Ctrl Pts',(88.0050119260407,49.9425002522374,10.7960063110774));
#80603=CARTESIAN_POINT('Ctrl Pts',(88.0005595153956,49.942945820831,10.7960351104507));
#80604=CARTESIAN_POINT('Ctrl Pts',(87.9900840314062,49.9439972945511,10.7961579595303));
#80605=CARTESIAN_POINT('Ctrl Pts',(87.9840615062244,49.944604227458,10.796271447286));
#80606=CARTESIAN_POINT('Ctrl Pts',(87.9665604181,49.9463745822525,10.7967257984163));
#80607=CARTESIAN_POINT('Ctrl Pts',(87.9550858795067,49.9475436195289,10.7971795032423));
#80608=CARTESIAN_POINT('Ctrl Pts',(87.8584984547107,49.9574463036794,10.8023112025123));
#80609=CARTESIAN_POINT('Ctrl Pts',(87.7740585656811,49.9664934828993,10.8153913956363));
#80610=CARTESIAN_POINT('Ctrl Pts',(87.6405645101739,49.9810035402672,10.8500825418811));
#80611=CARTESIAN_POINT('Ctrl Pts',(87.5904230273555,49.9865078328281,10.8665025304761));
#80612=CARTESIAN_POINT('Ctrl Pts',(87.5206497744989,49.9942259419302,10.8942673622174));
#80613=CARTESIAN_POINT('Ctrl Pts',(87.5000794495506,49.9965094760542,10.9030893997864));
#80614=CARTESIAN_POINT('Ctrl Pts',(87.463455266699,50.0005920438064,10.9199560862405));
#80615=CARTESIAN_POINT('Ctrl Pts',(87.4473189863176,50.0023969038322,10.9278059539436));
#80616=CARTESIAN_POINT('Ctrl Pts',(87.4223397919524,50.0052024371873,10.9406192723622));
#80617=CARTESIAN_POINT('Ctrl Pts',(87.4133815135729,50.006210979588,10.945350731677));
#80618=CARTESIAN_POINT('Ctrl Pts',(87.3967276717559,50.008090970631,10.9544032331983));
#80619=CARTESIAN_POINT('Ctrl Pts',(87.3890187607374,50.0089632692538,10.9586982285163));
#80620=CARTESIAN_POINT('Ctrl Pts',(87.3717963706809,50.010917253196,10.9685302441104));
#80621=CARTESIAN_POINT('Ctrl Pts',(87.3623087317852,50.0119972957776,10.9741113600636));
#80622=CARTESIAN_POINT('Ctrl Pts',(87.3380155570588,50.0147734747744,10.988830286705));
#80623=CARTESIAN_POINT('Ctrl Pts',(87.3233226328539,50.0164629915661,10.9981504980386));
#80624=CARTESIAN_POINT('Ctrl Pts',(87.2516525011199,50.0247683884528,11.0457063077488));
#80625=CARTESIAN_POINT('Ctrl Pts',(87.197643026823,50.0312240934094,11.0882165308644));
#80626=CARTESIAN_POINT('Ctrl Pts',(87.1001233262038,50.0436948393222,11.1786731864601));
#80627=CARTESIAN_POINT('Ctrl Pts',(87.0563226578107,50.0496958081879,11.2259792957401));
#80628=CARTESIAN_POINT('Ctrl Pts',(87.0069289657661,50.0572897765511,11.2882027357601));
#80629=CARTESIAN_POINT('Ctrl Pts',(86.997768409111,50.0587385520758,11.3001743568044));
#80630=CARTESIAN_POINT('Ctrl Pts',(86.978230636241,50.0619261235956,11.3266718945819));
#80631=CARTESIAN_POINT('Ctrl Pts',(86.9679426576656,50.0636687822992,11.3412587561351));
#80632=CARTESIAN_POINT('Ctrl Pts',(86.9540079240187,50.0661293241174,11.361927635367));
#80633=CARTESIAN_POINT('Ctrl Pts',(86.950098804876,50.0668312249718,11.367831833372));
#80634=CARTESIAN_POINT('Ctrl Pts',(86.9434870877152,50.0680391902686,11.3780016858574));
#80635=CARTESIAN_POINT('Ctrl Pts',(86.9407601780801,50.068543660943,11.3822513474958));
#80636=CARTESIAN_POINT('Ctrl Pts',(86.9350333616865,50.0696167182829,11.3912943116648));
#80637=CARTESIAN_POINT('Ctrl Pts',(86.9320401380705,50.0701856639433,11.3960913611524));
#80638=CARTESIAN_POINT('Ctrl Pts',(86.9238215641207,50.0717702159644,11.4094607105698));
#80639=CARTESIAN_POINT('Ctrl Pts',(86.9186658693362,50.0727899407057,11.4180749163416));
#80640=CARTESIAN_POINT('Ctrl Pts',(86.881935893481,50.0802405721036,11.4811283693055));
#80641=CARTESIAN_POINT('Ctrl Pts',(86.8543493269671,50.0868575860968,11.5377790442601));
#80642=CARTESIAN_POINT('Ctrl Pts',(86.812454297466,50.0987970659119,11.6430070212977));
#80643=CARTESIAN_POINT('Ctrl Pts',(86.7966277352883,50.1041052975822,11.690852657582));
#80644=CARTESIAN_POINT('Ctrl Pts',(86.7742169967274,50.1131970337355,11.7750985650213));
#80645=CARTESIAN_POINT('Ctrl Pts',(86.7663020745541,50.1170034884842,11.8110813444863));
#80646=CARTESIAN_POINT('Ctrl Pts',(86.7578398617064,50.1220240544275,11.8595016823623));
#80647=CARTESIAN_POINT('Ctrl Pts',(86.7558949005567,50.1232776581811,11.8716726906734));
#80648=CARTESIAN_POINT('Ctrl Pts',(86.7515286101213,50.1263611558463,11.9018044087611));
#80649=CARTESIAN_POINT('Ctrl Pts',(86.7493138483551,50.1281844627442,11.9197929007142));
#80650=CARTESIAN_POINT('Ctrl Pts',(86.7464594032621,50.1310111940452,11.9479310154748));
#80651=CARTESIAN_POINT('Ctrl Pts',(86.7455553657337,50.1320227075707,11.9580504798649));
#80652=CARTESIAN_POINT('Ctrl Pts',(86.7440943866172,50.1339041400774,11.9769620836901));
#80653=CARTESIAN_POINT('Ctrl Pts',(86.7435073097484,50.1347749421174,11.985751175705));
#80654=CARTESIAN_POINT('Ctrl Pts',(86.742396603616,50.1367202429151,12.0054612178035));
#80655=CARTESIAN_POINT('Ctrl Pts',(86.7419224490456,50.137793145599,12.0163843829065));
#80656=CARTESIAN_POINT('Ctrl Pts',(86.7409178801289,50.1410166907371,12.0493464034488));
#80657=CARTESIAN_POINT('Ctrl Pts',(86.7408201065641,50.1431539473633,12.0713952958311));
#80658=CARTESIAN_POINT('Ctrl Pts',(86.7434309180857,50.1547883986694,12.192215236219));
#80659=CARTESIAN_POINT('Ctrl Pts',(86.7570841460695,50.1639311885861,12.2904085065647));
#80660=CARTESIAN_POINT('Ctrl Pts',(86.7919085474611,50.1769266341357,12.4241437042271));
#80661=CARTESIAN_POINT('Ctrl Pts',(86.803598653043,50.1806504833118,12.4617678724369));
#80662=CARTESIAN_POINT('Ctrl Pts',(86.8247021576846,50.1866123166092,12.519989167242));
#80663=CARTESIAN_POINT('Ctrl Pts',(86.8329510883193,50.1888045104766,12.5409834460733));
#80664=CARTESIAN_POINT('Ctrl Pts',(86.8447618621988,50.1917859489306,12.5688399332129));
#80665=CARTESIAN_POINT('Ctrl Pts',(86.8478345370942,50.1925487627717,12.5759073321859));
#80666=CARTESIAN_POINT('Ctrl Pts',(86.8530678356417,50.1938277713648,12.5876508741064));
#80667=CARTESIAN_POINT('Ctrl Pts',(86.855193026749,50.194341867765,12.5923428253558));
#80668=CARTESIAN_POINT('Ctrl Pts',(86.859325052362,50.1953316563716,12.60131972009));
#80669=CARTESIAN_POINT('Ctrl Pts',(86.8613273941846,50.1958070430285,12.6056066015568));
#80670=CARTESIAN_POINT('Ctrl Pts',(86.8668669989379,50.1971105524673,12.6172957304816));
#80671=CARTESIAN_POINT('Ctrl Pts',(86.8704520023896,50.1979414377093,12.6246748237477));
#80672=CARTESIAN_POINT('Ctrl Pts',(86.8851175486864,50.2012891743505,12.6541317178038));
#80673=CARTESIAN_POINT('Ctrl Pts',(86.8967686881854,50.2038351105929,12.6759168182268));
#80674=CARTESIAN_POINT('Ctrl Pts',(86.945528234777,50.2140291023914,12.7610219413424));
#80675=CARTESIAN_POINT('Ctrl Pts',(86.9874592028914,50.2218137436217,12.8214132528099));
#80676=CARTESIAN_POINT('Ctrl Pts',(87.0652277460183,50.2345903651937,12.9149671626036));
#80677=CARTESIAN_POINT('Ctrl Pts',(87.0981821164097,50.2396193089436,12.9503048677441));
#80678=CARTESIAN_POINT('Ctrl Pts',(87.1484102351758,50.2467530109683,12.998356906835));
#80679=CARTESIAN_POINT('Ctrl Pts',(87.1641136814851,50.2489163345288,13.0126436505277));
#80680=CARTESIAN_POINT('Ctrl Pts',(87.1803269728098,50.2510849025526,13.0266676665082));
#80681=CARTESIAN_POINT('Ctrl Pts',(87.1804848873278,50.2511060179337,13.026804189832));
#80682=CARTESIAN_POINT('Ctrl Pts',(87.1806428354213,50.2511271317289,13.0269406741484));
#80683=CARTESIAN_POINT('',(89.2765936958547,49.5646,12.1717005062084));
#80684=CARTESIAN_POINT('Origin',(88.011,49.5646,12.066));
#80685=CARTESIAN_POINT('Ctrl Pts',(89.2765936958547,49.5645999999999,12.1717005062084));
#80686=CARTESIAN_POINT('Ctrl Pts',(89.2769323000493,49.5650046868909,12.1676462651325));
#80687=CARTESIAN_POINT('Ctrl Pts',(89.2772514280172,49.565408516634,12.1635903372669));
#80688=CARTESIAN_POINT('Ctrl Pts',(89.2779126985219,49.5662979343296,12.1546359137711));
#80689=CARTESIAN_POINT('Ctrl Pts',(89.2782459359607,49.5667831431295,12.1497367954486));
#80690=CARTESIAN_POINT('Ctrl Pts',(89.2792425199579,49.5683658484442,12.133713345017));
#80691=CARTESIAN_POINT('Ctrl Pts',(89.2797878903809,49.5694586556053,12.1225817908385));
#80692=CARTESIAN_POINT('Ctrl Pts',(89.2822519137991,49.5761806799657,12.0537650718098));
#80693=CARTESIAN_POINT('Ctrl Pts',(89.2803831184224,49.5816768845998,11.996004944591));
#80694=CARTESIAN_POINT('Ctrl Pts',(89.2687771479741,49.5926656596804,11.8809244195437));
#80695=CARTESIAN_POINT('Ctrl Pts',(89.2590269501668,49.5981458364218,11.8237510638077));
#80696=CARTESIAN_POINT('Ctrl Pts',(89.2374492555629,49.6069527026906,11.7345356591435));
#80697=CARTESIAN_POINT('Ctrl Pts',(89.2281776015839,49.6102236370538,11.7019605849923));
#80698=CARTESIAN_POINT('Ctrl Pts',(89.2142958350412,49.614570312701,11.6596843173648));
#80699=CARTESIAN_POINT('Ctrl Pts',(89.2108482338348,49.6156134279439,11.6496137588617));
#80700=CARTESIAN_POINT('Ctrl Pts',(89.20377286592,49.6176858602253,11.6297642152997));
#80701=CARTESIAN_POINT('Ctrl Pts',(89.2001504054557,49.6187149499584,11.6199842287395));
#80702=CARTESIAN_POINT('Ctrl Pts',(89.1928303632922,49.6207349684929,11.6009447504895));
#80703=CARTESIAN_POINT('Ctrl Pts',(89.1891433682059,49.6217255104158,11.5916819806983));
#80704=CARTESIAN_POINT('Ctrl Pts',(89.1808121183426,49.6239072545291,11.5714481557508));
#80705=CARTESIAN_POINT('Ctrl Pts',(89.1761218268057,49.6250998091589,11.5604972557697));
#80706=CARTESIAN_POINT('Ctrl Pts',(89.159600459255,49.6291845559768,11.5233750253254));
#80707=CARTESIAN_POINT('Ctrl Pts',(89.1470370362848,49.6320995648524,11.4975420805315));
#80708=CARTESIAN_POINT('Ctrl Pts',(89.0875690162719,49.6451333895115,11.3851223167385));
#80709=CARTESIAN_POINT('Ctrl Pts',(89.0315711283794,49.6555434747946,11.3037523224961));
#80710=CARTESIAN_POINT('Ctrl Pts',(88.9381047214701,49.6705770056107,11.1969371953824));
#80711=CARTESIAN_POINT('Ctrl Pts',(88.9077845422685,49.6751734267477,11.1656825692961));
#80712=CARTESIAN_POINT('Ctrl Pts',(88.8638279400527,49.6814238595994,11.124800196136));
#80713=CARTESIAN_POINT('Ctrl Pts',(88.851519825673,49.6831328581012,11.1137925287434));
#80714=CARTESIAN_POINT('Ctrl Pts',(88.8299400521271,49.6860554884921,11.0952374395651));
#80715=CARTESIAN_POINT('Ctrl Pts',(88.820770343694,49.6872753468725,11.0875753549224));
#80716=CARTESIAN_POINT('Ctrl Pts',(88.8075623427943,49.6890000720258,11.0768518453986));
#80717=CARTESIAN_POINT('Ctrl Pts',(88.8036122516282,49.6895118489977,11.0736837905623));
#80718=CARTESIAN_POINT('Ctrl Pts',(88.7956901350752,49.6905300833802,11.0674075773513));
#80719=CARTESIAN_POINT('Ctrl Pts',(88.7917183237476,49.6910365460048,11.064299277719));
#80720=CARTESIAN_POINT('Ctrl Pts',(88.7833942769881,49.692089442313,11.0578645504107));
#80721=CARTESIAN_POINT('Ctrl Pts',(88.7790388626329,49.6926355248832,11.0545424812232));
#80722=CARTESIAN_POINT('Ctrl Pts',(88.7668631370902,49.6941492085432,11.0453795092804));
#80723=CARTESIAN_POINT('Ctrl Pts',(88.758996442199,49.6951125394715,11.0396001690265));
#80724=CARTESIAN_POINT('Ctrl Pts',(88.7027752587467,49.7019010551538,10.9992865207747));
#80725=CARTESIAN_POINT('Ctrl Pts',(88.6521062282323,49.7075222453052,10.9680854424479));
#80726=CARTESIAN_POINT('Ctrl Pts',(88.5353566848549,49.7198880030529,10.907044717012));
#80727=CARTESIAN_POINT('Ctrl Pts',(88.4685450207078,49.7265937271633,10.8790799166231));
#80728=CARTESIAN_POINT('Ctrl Pts',(88.3625541117604,49.7371500013212,10.8450029978505));
#80729=CARTESIAN_POINT('Ctrl Pts',(88.3248630363222,49.7408871104389,10.8347756959694));
#80730=CARTESIAN_POINT('Ctrl Pts',(88.2740052622932,49.7459517859196,10.8234626382528));
#80731=CARTESIAN_POINT('Ctrl Pts',(88.2612032162937,49.7472284190329,10.8208216263615));
#80732=CARTESIAN_POINT('Ctrl Pts',(88.2397019262584,49.7493770455482,10.8167309484277));
#80733=CARTESIAN_POINT('Ctrl Pts',(88.2310239460632,49.7502454521437,10.8151733984029));
#80734=CARTESIAN_POINT('Ctrl Pts',(88.2138481733429,49.7519671286929,10.8122749019376));
#80735=CARTESIAN_POINT('Ctrl Pts',(88.2053515711777,49.752820209205,10.8109296991635));
#80736=CARTESIAN_POINT('Ctrl Pts',(88.1845611057612,49.7549115226841,10.807854273543));
#80737=CARTESIAN_POINT('Ctrl Pts',(88.1722546044664,49.7561527576014,10.8062178563233));
#80738=CARTESIAN_POINT('Ctrl Pts',(88.1291301060743,49.760515681839,10.8011257255669));
#80739=CARTESIAN_POINT('Ctrl Pts',(88.0982145124258,49.7636676128701,10.798618907008));
#80740=CARTESIAN_POINT('Ctrl Pts',(87.9655774587639,49.7773124396985,10.7927393429728));
#80741=CARTESIAN_POINT('Ctrl Pts',(87.8637565256329,49.7881363221284,10.8004697136525));
#80742=CARTESIAN_POINT('Ctrl Pts',(87.7319622453892,49.8023197095386,10.8266037199878));
#80743=CARTESIAN_POINT('Ctrl Pts',(87.7002014977306,49.8057471915974,10.8341843042755));
#80744=CARTESIAN_POINT('Ctrl Pts',(87.6496795407766,49.8111852152096,10.8483217522422));
#80745=CARTESIAN_POINT('Ctrl Pts',(87.6307193950464,49.8132226659892,10.854109075081));
#80746=CARTESIAN_POINT('Ctrl Pts',(87.6051532890732,49.8159588637391,10.8625719954764));
#80747=CARTESIAN_POINT('Ctrl Pts',(87.5984245293166,49.8166779403467,10.8648622039702));
#80748=CARTESIAN_POINT('Ctrl Pts',(87.5870617769268,49.8178900281601,10.868836400174));
#80749=CARTESIAN_POINT('Ctrl Pts',(87.5824181004758,49.8183847211985,10.8704909621451));
#80750=CARTESIAN_POINT('Ctrl Pts',(87.5726900960301,49.8194197803,10.8740210609205));
#80751=CARTESIAN_POINT('Ctrl Pts',(87.5676080355378,49.8199598005803,10.8759021329875));
#80752=CARTESIAN_POINT('Ctrl Pts',(87.5541286333398,49.8213906505748,10.8809897275288));
#80753=CARTESIAN_POINT('Ctrl Pts',(87.545752762003,49.8222782288989,10.8842530659663));
#80754=CARTESIAN_POINT('Ctrl Pts',(87.5070460980611,49.8263761616861,10.8998089896386));
#80755=CARTESIAN_POINT('Ctrl Pts',(87.4771591065237,49.8295296518795,10.913183660978));
#80756=CARTESIAN_POINT('Ctrl Pts',(87.38702977778,49.8391125782347,10.9577757674378));
#80757=CARTESIAN_POINT('Ctrl Pts',(87.3287432147873,49.8454182479325,10.9926748033746));
#80758=CARTESIAN_POINT('Ctrl Pts',(87.2215263468942,49.8577704798631,11.0691500172164));
#80759=CARTESIAN_POINT('Ctrl Pts',(87.17241272399,49.8637929224047,11.1100983730446));
#80760=CARTESIAN_POINT('Ctrl Pts',(87.1130599642401,49.8717831167394,11.1676909324373));
#80761=CARTESIAN_POINT('Ctrl Pts',(87.099823689606,49.873615909198,11.1811197073028));
#80762=CARTESIAN_POINT('Ctrl Pts',(87.0797676074864,49.8764782507339,11.2023947067934));
#80763=CARTESIAN_POINT('Ctrl Pts',(87.0727364437849,49.8774987776753,11.210038929206));
#80764=CARTESIAN_POINT('Ctrl Pts',(87.0598490037513,49.8794021763518,11.2243996359065));
#80765=CARTESIAN_POINT('Ctrl Pts',(87.0539680795527,49.8802839542825,11.2310932485596));
#80766=CARTESIAN_POINT('Ctrl Pts',(87.0410212097189,49.8822554486975,11.2461457827901));
#80767=CARTESIAN_POINT('Ctrl Pts',(87.0339920173032,49.8833465675926,11.2545351678547));
#80768=CARTESIAN_POINT('Ctrl Pts',(87.0163349803454,49.8861420245164,11.2761709702983));
#80769=CARTESIAN_POINT('Ctrl Pts',(87.0058632180014,49.8878522817962,11.2895411300496));
#80770=CARTESIAN_POINT('Ctrl Pts',(86.9436470725428,49.8983465691198,11.3723458184373));
#80771=CARTESIAN_POINT('Ctrl Pts',(86.8988594413864,49.9073829336367,11.4466978875224));
#80772=CARTESIAN_POINT('Ctrl Pts',(86.8412933146105,49.921594676046,11.5689621292214));
#80773=CARTESIAN_POINT('Ctrl Pts',(86.8231357400698,49.9267083943839,11.6140714077037));
#80774=CARTESIAN_POINT('Ctrl Pts',(86.8020477176019,49.9335591036386,11.6765941462585));
#80775=CARTESIAN_POINT('Ctrl Pts',(86.7968275469791,49.9353553051812,11.6931892194839));
#80776=CARTESIAN_POINT('Ctrl Pts',(86.7883669080754,49.9384469312673,11.7221518154864));
#80777=CARTESIAN_POINT('Ctrl Pts',(86.7849692360516,49.939748526432,11.7344704220278));
#80778=CARTESIAN_POINT('Ctrl Pts',(86.7801776564371,49.9416767465736,11.7529250953683));
#80779=CARTESIAN_POINT('Ctrl Pts',(86.7786426253116,49.9423103754458,11.7590230556088));
#80780=CARTESIAN_POINT('Ctrl Pts',(86.7759570545057,49.9434481646863,11.7700364838419));
#80781=CARTESIAN_POINT('Ctrl Pts',(86.7747904528073,49.943953163568,11.7749477033214));
#80782=CARTESIAN_POINT('Ctrl Pts',(86.772212475991,49.9450940953002,11.7860958104379));
#80783=CARTESIAN_POINT('Ctrl Pts',(86.7708188743494,49.9457290402113,11.7923365808807));
#80784=CARTESIAN_POINT('Ctrl Pts',(86.7666112371446,49.9477056514021,11.8118715861533));
#80785=CARTESIAN_POINT('Ctrl Pts',(86.7639632290181,49.9490386622054,11.8252013507172));
#80786=CARTESIAN_POINT('Ctrl Pts',(86.7444921589084,49.9596305486429,11.9321737957046));
#80787=CARTESIAN_POINT('Ctrl Pts',(86.7380234189308,49.9684302105805,12.0274116063342));
#80788=CARTESIAN_POINT('Ctrl Pts',(86.7449602574838,49.9830791329554,12.1832013170017));
#80789=CARTESIAN_POINT('Ctrl Pts',(86.7520166093667,49.9888219618752,12.2436282975283));
#80790=CARTESIAN_POINT('Ctrl Pts',(86.7667991746953,49.9964713448086,12.321345425353));
#80791=CARTESIAN_POINT('Ctrl Pts',(86.7706197367687,49.9982569606994,12.3393014844075));
#80792=CARTESIAN_POINT('Ctrl Pts',(86.777175719583,50.001057743096,12.3671353822076));
#80793=CARTESIAN_POINT('Ctrl Pts',(86.7796439706478,50.0020644326792,12.3770742471473));
#80794=CARTESIAN_POINT('Ctrl Pts',(86.7844696811376,50.0039486620166,12.395547811436));
#80795=CARTESIAN_POINT('Ctrl Pts',(86.7867967480551,50.0048251770037,12.4040898859954));
#80796=CARTESIAN_POINT('Ctrl Pts',(86.7922034086236,50.0067930955415,12.4231483434946));
#80797=CARTESIAN_POINT('Ctrl Pts',(86.7953301427021,50.0078859600801,12.4336504443208));
#80798=CARTESIAN_POINT('Ctrl Pts',(86.8036969718199,50.010700414025,12.4604786129577));
#80799=CARTESIAN_POINT('Ctrl Pts',(86.8091323121346,50.0124281786764,12.4767407521832));
#80800=CARTESIAN_POINT('Ctrl Pts',(86.8452534301501,50.0233246196986,12.5779494240839));
#80801=CARTESIAN_POINT('Ctrl Pts',(86.8845919924673,50.0327740382255,12.6595103748224));
#80802=CARTESIAN_POINT('Ctrl Pts',(86.9581998254973,50.0474828835358,12.7779925928973));
#80803=CARTESIAN_POINT('Ctrl Pts',(86.986577962565,50.0526752123085,12.8182511529358));
#80804=CARTESIAN_POINT('Ctrl Pts',(87.0281349537844,50.0596163826883,12.8704771215578));
#80805=CARTESIAN_POINT('Ctrl Pts',(87.0393305894005,50.0614287681075,12.8839644145795));
#80806=CARTESIAN_POINT('Ctrl Pts',(87.0591952191831,50.0645420993583,12.9069114614065));
#80807=CARTESIAN_POINT('Ctrl Pts',(87.0677347606364,50.0658495787102,12.9164793709917));
#80808=CARTESIAN_POINT('Ctrl Pts',(87.0806340466589,50.0677775640108,12.9304986739871));
#80809=CARTESIAN_POINT('Ctrl Pts',(87.0848835456706,50.0684053772195,12.9350495287782));
#80810=CARTESIAN_POINT('Ctrl Pts',(87.0925767687912,50.0695286145152,12.9431677996641));
#80811=CARTESIAN_POINT('Ctrl Pts',(87.0960080982478,50.0700249054027,12.9467465036873));
#80812=CARTESIAN_POINT('Ctrl Pts',(87.1037832604899,50.0711389669835,12.9547611198974));
#80813=CARTESIAN_POINT('Ctrl Pts',(87.1081387736843,50.0717558231018,12.9591853966009));
#80814=CARTESIAN_POINT('Ctrl Pts',(87.1216251817373,50.0736445564625,12.9726852605607));
#80815=CARTESIAN_POINT('Ctrl Pts',(87.1308622393573,50.0749086055255,12.9816545737792));
#80816=CARTESIAN_POINT('Ctrl Pts',(87.1534450821938,50.0779338965543,13.0029252358484));
#80817=CARTESIAN_POINT('Ctrl Pts',(87.1669176652258,50.0796858746954,13.0150806361318));
#80818=CARTESIAN_POINT('Ctrl Pts',(87.1806428554372,50.081424866233,13.0269406914443));
#80819=CARTESIAN_POINT('Origin',(88.011,49.5646,12.066));
#80820=CARTESIAN_POINT('',(87.4793792431904,49.5646,10.446693294484));
#80821=CARTESIAN_POINT('',(86.30666,49.5646,12.066));
#80822=CARTESIAN_POINT('Origin',(88.011,49.5646,12.066));
#80823=CARTESIAN_POINT('Ctrl Pts',(87.4793792431904,49.5646000000001,10.446693294484));
#80824=CARTESIAN_POINT('Ctrl Pts',(87.5432134943017,49.5646000000001,10.4346997308512));
#80825=CARTESIAN_POINT('Ctrl Pts',(87.607765068069,49.5646000000001,10.4266992315549));
#80826=CARTESIAN_POINT('Ctrl Pts',(87.6726821165043,49.5646000000001,10.422592732542));
#80827=CARTESIAN_POINT('Ctrl Pts',(87.7301000591824,49.5646,10.4189606092306));
#80828=CARTESIAN_POINT('Ctrl Pts',(87.7878044036963,49.5646000000001,10.4183758163793));
#80829=CARTESIAN_POINT('Ctrl Pts',(87.8455396127937,49.5646000000001,10.4208015589989));
#80830=CARTESIAN_POINT('Ctrl Pts',(87.8597334500476,49.5646000000001,10.4213979125326));
#80831=CARTESIAN_POINT('Ctrl Pts',(87.8739193815678,49.5646,10.4221759525792));
#80832=CARTESIAN_POINT('Ctrl Pts',(87.888092217474,49.5646,10.4231345189642));
#80833=CARTESIAN_POINT('Ctrl Pts',(87.9516421369536,49.5646,10.4274326578117));
#80834=CARTESIAN_POINT('Ctrl Pts',(88.0149405906727,49.5646,10.4353571812218));
#80835=CARTESIAN_POINT('Ctrl Pts',(88.0776421524961,49.5646,10.446837972588));
#80836=CARTESIAN_POINT('Ctrl Pts',(88.1194110731014,49.5646,10.4544859521457));
#80837=CARTESIAN_POINT('Ctrl Pts',(88.1609147379759,49.5646,10.4637130627391));
#80838=CARTESIAN_POINT('Ctrl Pts',(88.2020432503533,49.5646,10.4745089165249));
#80839=CARTESIAN_POINT('Ctrl Pts',(88.217204017084,49.5646,10.4784884774535));
#80840=CARTESIAN_POINT('Ctrl Pts',(88.2323177970543,49.5646,10.482682610884));
#80841=CARTESIAN_POINT('Ctrl Pts',(88.2473520841595,49.5646,10.487082783089));
#80842=CARTESIAN_POINT('Ctrl Pts',(88.3060841492863,49.5646,10.5042722380133));
#80843=CARTESIAN_POINT('Ctrl Pts',(88.3636811048161,49.5646,10.5246207416929));
#80844=CARTESIAN_POINT('Ctrl Pts',(88.4198383627968,49.5646,10.5480572671525));
#80845=CARTESIAN_POINT('Ctrl Pts',(88.4751444718139,49.5646,10.5711385762949));
#80846=CARTESIAN_POINT('Ctrl Pts',(88.5290549999893,49.5646,10.5972155885462));
#80847=CARTESIAN_POINT('Ctrl Pts',(88.5812452068814,49.5646,10.6262565481873));
#80848=CARTESIAN_POINT('Ctrl Pts',(88.6126791782889,49.5646,10.6437478123414));
#80849=CARTESIAN_POINT('Ctrl Pts',(88.6434883754159,49.5646,10.662314937626));
#80850=CARTESIAN_POINT('Ctrl Pts',(88.6735939944165,49.5646,10.6819561549177));
#80851=CARTESIAN_POINT('Ctrl Pts',(88.6985873415264,49.5646,10.6982620731393));
#80852=CARTESIAN_POINT('Ctrl Pts',(88.7230956814319,49.5646,10.7153083477659));
#80853=CARTESIAN_POINT('Ctrl Pts',(88.7470702501294,49.5646,10.7330956630536));
#80854=CARTESIAN_POINT('Ctrl Pts',(88.7576802894461,49.5646,10.7409675091303));
#80855=CARTESIAN_POINT('Ctrl Pts',(88.7681881486854,49.5646,10.7489865796549));
#80856=CARTESIAN_POINT('Ctrl Pts',(88.7785699894182,49.5646,10.7571372605137));
#80857=CARTESIAN_POINT('Ctrl Pts',(88.8233248591948,49.5646,10.7922738677701));
#80858=CARTESIAN_POINT('Ctrl Pts',(88.8658175386404,49.5646,10.8299084505779));
#80859=CARTESIAN_POINT('Ctrl Pts',(88.9057642508585,49.5646,10.8700060633041));
#80860=CARTESIAN_POINT('Ctrl Pts',(88.9108943848685,49.5646,10.8751555766269));
#80861=CARTESIAN_POINT('Ctrl Pts',(88.9159824695673,49.5646,10.8803457510599));
#80862=CARTESIAN_POINT('Ctrl Pts',(88.9210278497657,49.5646,10.885576545595));
#80863=CARTESIAN_POINT('Ctrl Pts',(88.961402604043,49.5646,10.9274350450001));
#80864=CARTESIAN_POINT('Ctrl Pts',(88.9990468409029,49.5646,10.9718936611491));
#80865=CARTESIAN_POINT('Ctrl Pts',(89.0338429995909,49.5646,11.0186424351575));
#80866=CARTESIAN_POINT('Ctrl Pts',(89.0640183489715,49.5646,11.059183133959));
#80867=CARTESIAN_POINT('Ctrl Pts',(89.0920511066818,49.5646,11.1014469418056));
#80868=CARTESIAN_POINT('Ctrl Pts',(89.1178329221646,49.5646,11.1452333647597));
#80869=CARTESIAN_POINT('Ctrl Pts',(89.1229657557734,49.5646,11.1539506881576));
#80870=CARTESIAN_POINT('Ctrl Pts',(89.1280104794418,49.5646,11.1627305054241));
#80871=CARTESIAN_POINT('Ctrl Pts',(89.1329621268224,49.5646,11.1715640955915));
#80872=CARTESIAN_POINT('Ctrl Pts',(89.1604471489843,49.5646,11.2205965494101));
#80873=CARTESIAN_POINT('Ctrl Pts',(89.1849976183063,49.5646,11.2711543804104));
#80874=CARTESIAN_POINT('Ctrl Pts',(89.206531164753,49.5646,11.3229450829069));
#80875=CARTESIAN_POINT('Ctrl Pts',(89.2278894852167,49.5646,11.3743143463813));
#80876=CARTESIAN_POINT('Ctrl Pts',(89.2462797865637,49.5646,11.4268976855764));
#80877=CARTESIAN_POINT('Ctrl Pts',(89.2615710260204,49.5646,11.4804105356582));
#80878=CARTESIAN_POINT('Ctrl Pts',(89.2765031578003,49.5646,11.5326666612395));
#80879=CARTESIAN_POINT('Ctrl Pts',(89.2884799242348,49.5646,11.5858101238446));
#80880=CARTESIAN_POINT('Ctrl Pts',(89.2973320937201,49.5646,11.6395609907597));
#80881=CARTESIAN_POINT('Ctrl Pts',(89.2991414178106,49.5646,11.6505473075663));
#80882=CARTESIAN_POINT('Ctrl Pts',(89.3008200504352,49.5646,11.6615589214129));
#80883=CARTESIAN_POINT('Ctrl Pts',(89.3023663054708,49.5646,11.672593307726));
#80884=CARTESIAN_POINT('Ctrl Pts',(89.3036790583404,49.5646,11.6819613757116));
#80885=CARTESIAN_POINT('Ctrl Pts',(89.3048950581329,49.5646,11.6913363184933));
#80886=CARTESIAN_POINT('Ctrl Pts',(89.3060138301966,49.5646,11.700716616931));
#80887=CARTESIAN_POINT('Ctrl Pts',(89.3122581336349,49.5646,11.7530717227543));
#80888=CARTESIAN_POINT('Ctrl Pts',(89.3154777290993,49.5646,11.8055958073229));
#80889=CARTESIAN_POINT('Ctrl Pts',(89.3155636653537,49.5646,11.8580373686408));
#80890=CARTESIAN_POINT('Ctrl Pts',(89.3156502223929,49.5646,11.9108577563898));
#80891=CARTESIAN_POINT('Ctrl Pts',(89.3125576884502,49.5646,11.9635954633224));
#80892=CARTESIAN_POINT('Ctrl Pts',(89.3061247018758,49.5646,12.0159713836245));
#80893=CARTESIAN_POINT('Ctrl Pts',(89.3000447623628,49.5646,12.0654728746809));
#80894=CARTESIAN_POINT('Ctrl Pts',(89.2909804830363,49.5646,12.1146517005517));
#80895=CARTESIAN_POINT('Ctrl Pts',(89.2787553837174,49.5646,12.1632419914215));
#80896=CARTESIAN_POINT('Ctrl Pts',(89.2780455024135,49.5646,12.1660635095243));
#80897=CARTESIAN_POINT('Ctrl Pts',(89.2773249526241,49.5645999999999,12.1688830330924));
#80898=CARTESIAN_POINT('Ctrl Pts',(89.2765936958546,49.5646,12.1717005062084));
#80899=CARTESIAN_POINT('',(88.1950623699338,49.5639392675618,13.3237488200268));
#80900=CARTESIAN_POINT('Ctrl Pts',(88.2080236424798,49.5646,13.3206241207246));
#80901=CARTESIAN_POINT('Ctrl Pts',(88.2036514348987,49.5643797558539,13.3213107233884));
#80902=CARTESIAN_POINT('Ctrl Pts',(88.1992756381996,49.5641595117079,13.3219744709519));
#80903=CARTESIAN_POINT('Ctrl Pts',(88.1948964915141,49.5639392675618,13.3226153271422));
#80904=CARTESIAN_POINT('Ctrl Pts',(88.1951651089274,49.5646,13.3249038896975));
#80905=CARTESIAN_POINT('Ctrl Pts',(88.147583815449,49.5646,13.3404287431933));
#80906=CARTESIAN_POINT('Ctrl Pts',(88.0990977222012,49.5646,13.3528110980375));
#80907=CARTESIAN_POINT('Ctrl Pts',(88.0499901030814,49.5646,13.3622015070427));
#80908=CARTESIAN_POINT('Ctrl Pts',(88.0131050869839,49.5646,13.3692546974341));
#80909=CARTESIAN_POINT('Ctrl Pts',(87.9758684960568,49.5646,13.3746192028678));
#80910=CARTESIAN_POINT('Ctrl Pts',(87.9383887371113,49.5646,13.3783443583316));
#80911=CARTESIAN_POINT('Ctrl Pts',(87.9251861406984,49.5646,13.3796565792623));
#80912=CARTESIAN_POINT('Ctrl Pts',(87.9119513363239,49.5646,13.3807653943206));
#80913=CARTESIAN_POINT('Ctrl Pts',(87.8986950683556,49.5646,13.3816721668229));
#80914=CARTESIAN_POINT('Ctrl Pts',(87.8455772117481,49.5646,13.3853056036145));
#80915=CARTESIAN_POINT('Ctrl Pts',(87.7922338268483,49.5646,13.3856915703243));
#80916=CARTESIAN_POINT('Ctrl Pts',(87.7389685900434,49.5646,13.3829815726137));
#80917=CARTESIAN_POINT('Ctrl Pts',(87.7008670109547,49.5646,13.3810430626531));
#80918=CARTESIAN_POINT('Ctrl Pts',(87.662804589928,49.5646,13.3775194839648));
#80919=CARTESIAN_POINT('Ctrl Pts',(87.6248847851905,49.5646,13.3724519617938));
#80920=CARTESIAN_POINT('Ctrl Pts',(87.612841961819,49.5646,13.370842584455));
#80921=CARTESIAN_POINT('Ctrl Pts',(87.6008115951672,49.5646,13.3690770863748));
#80922=CARTESIAN_POINT('Ctrl Pts',(87.5888029110002,49.5646,13.3671574954402));
#80923=CARTESIAN_POINT('Ctrl Pts',(87.5342255989436,49.5646,13.3584332995169));
#80924=CARTESIAN_POINT('Ctrl Pts',(87.480254606079,49.5646,13.3465559506408));
#80925=CARTESIAN_POINT('Ctrl Pts',(87.4271969284901,49.5646,13.3316854838884));
#80926=CARTESIAN_POINT('Ctrl Pts',(87.3725247345629,49.5646,13.3163625169019));
#80927=CARTESIAN_POINT('Ctrl Pts',(87.318821216024,49.5646,13.2978617600648));
#80928=CARTESIAN_POINT('Ctrl Pts',(87.2664029391945,49.5646,13.2763069116344));
#80929=CARTESIAN_POINT('Ctrl Pts',(87.2141247648759,49.5646,13.2548096745673));
#80930=CARTESIAN_POINT('Ctrl Pts',(87.1631237126695,49.5646,13.2302745990502));
#80931=CARTESIAN_POINT('Ctrl Pts',(87.1137126784811,49.5646,13.2027729015126));
#80932=CARTESIAN_POINT('Ctrl Pts',(87.1044241328058,49.5646,13.1976029879918));
#80933=CARTESIAN_POINT('Ctrl Pts',(87.095191804154,49.5646,13.1923280933648));
#80934=CARTESIAN_POINT('Ctrl Pts',(87.0860178237703,49.5646,13.1869484894039));
#80935=CARTESIAN_POINT('Ctrl Pts',(87.0776898390854,49.5646,13.1820649756483));
#80936=CARTESIAN_POINT('Ctrl Pts',(87.0694132039564,49.5646,13.1770970225026));
#80937=CARTESIAN_POINT('Ctrl Pts',(87.0611963948787,49.5646,13.1720494758806));
#80938=CARTESIAN_POINT('Ctrl Pts',(87.0109104049247,49.5646,13.1411590321176));
#80939=CARTESIAN_POINT('Ctrl Pts',(86.9627871139725,49.5646,13.107246058951));
#80940=CARTESIAN_POINT('Ctrl Pts',(86.9171559545492,49.5646,13.0704523153941));
#80941=CARTESIAN_POINT('Ctrl Pts',(86.9114896833008,49.5646,13.0658834345269));
#80942=CARTESIAN_POINT('Ctrl Pts',(86.9058618367084,49.5646,13.0612700676731));
#80943=CARTESIAN_POINT('Ctrl Pts',(86.9002730461311,49.5646,13.0566124305091));
#80944=CARTESIAN_POINT('Ctrl Pts',(86.8568625806386,49.5646,13.0204346216277));
#80945=CARTESIAN_POINT('Ctrl Pts',(86.8158067936454,49.5646,12.9815899007508));
#80946=CARTESIAN_POINT('Ctrl Pts',(86.7771379528804,49.5646,12.9403791635712));
#80947=CARTESIAN_POINT('Ctrl Pts',(86.7561113369255,49.5646,12.9179703629257));
#80948=CARTESIAN_POINT('Ctrl Pts',(86.7357908280484,49.5646,12.8948611228301));
#80949=CARTESIAN_POINT('Ctrl Pts',(86.7161845486795,49.5646,12.871094260736));
#80950=CARTESIAN_POINT('Ctrl Pts',(86.7018051845722,49.5646,12.8536635000441));
#80951=CARTESIAN_POINT('Ctrl Pts',(86.6878100364862,49.5646,12.8358789337154));
#80952=CARTESIAN_POINT('Ctrl Pts',(86.6742031561875,49.5646,12.8177563007364));
#80953=CARTESIAN_POINT('Ctrl Pts',(86.6653701582013,49.5646,12.8059918714849));
#80954=CARTESIAN_POINT('Ctrl Pts',(86.6566978401993,49.5646,12.7940805137582));
#80955=CARTESIAN_POINT('Ctrl Pts',(86.6482054177523,49.5646,12.7820525218999));
#80956=CARTESIAN_POINT('Ctrl Pts',(86.6133892636089,49.5646,12.7327416896628));
#80957=CARTESIAN_POINT('Ctrl Pts',(86.5815409247293,49.5646,12.6814071691517));
#80958=CARTESIAN_POINT('Ctrl Pts',(86.5526856719227,49.5646,12.6284074774605));
#80959=CARTESIAN_POINT('Ctrl Pts',(86.523830419116,49.5646,12.5754077857694));
#80960=CARTESIAN_POINT('Ctrl Pts',(86.4979677303733,49.5646,12.5207421219677));
#80961=CARTESIAN_POINT('Ctrl Pts',(86.475150702407,49.5646,12.4647232688012));
#80962=CARTESIAN_POINT('Ctrl Pts',(86.451851227582,49.5646,12.4075199441172));
#80963=CARTESIAN_POINT('Ctrl Pts',(86.431726870377,49.5646,12.3489048167329));
#80964=CARTESIAN_POINT('Ctrl Pts',(86.4148726192312,49.5646,12.2891750718329));
#80965=CARTESIAN_POINT('Ctrl Pts',(86.4116417237766,49.5646,12.2777251082816));
#80966=CARTESIAN_POINT('Ctrl Pts',(86.4085311259145,49.5646,12.2662341026577));
#80967=CARTESIAN_POINT('Ctrl Pts',(86.4055416858706,49.5646,12.2547040415001));
#80968=CARTESIAN_POINT('Ctrl Pts',(86.4025231478382,49.5646,12.2430617514366));
#80969=CARTESIAN_POINT('Ctrl Pts',(86.3996302010096,49.5646,12.2313873791669));
#80970=CARTESIAN_POINT('Ctrl Pts',(86.3968649172368,49.5646,12.2196906431064));
#80971=CARTESIAN_POINT('Ctrl Pts',(86.3820925664019,49.5646,12.1572058122891));
#80972=CARTESIAN_POINT('Ctrl Pts',(86.3709436194787,49.5646,12.0940211401315));
#80973=CARTESIAN_POINT('Ctrl Pts',(86.3634668315128,49.5646,12.0304891040359));
#80974=CARTESIAN_POINT('Ctrl Pts',(86.3559769727694,49.5646,11.9668460024514));
#80975=CARTESIAN_POINT('Ctrl Pts',(86.3521715596108,49.5646,11.9028533267291));
#80976=CARTESIAN_POINT('Ctrl Pts',(86.3521409187914,49.5646,11.8388343782705));
#80977=CARTESIAN_POINT('Ctrl Pts',(86.3521105495977,49.5646,11.7753829468404));
#80978=CARTESIAN_POINT('Ctrl Pts',(86.3557878467311,49.5646,11.7119046684883));
#80979=CARTESIAN_POINT('Ctrl Pts',(86.3633089374713,49.5646,11.6486990891005));
#80980=CARTESIAN_POINT('Ctrl Pts',(86.364728299535,49.5646,11.6367710849457));
#80981=CARTESIAN_POINT('Ctrl Pts',(86.3662847067316,49.5646,11.6248527747873));
#80982=CARTESIAN_POINT('Ctrl Pts',(86.3679792906019,49.5646,11.6129461576272));
#80983=CARTESIAN_POINT('Origin',(88.011,49.5646,12.066));
#80984=CARTESIAN_POINT('Ctrl Pts',(87.4195227899263,65.1917000946238,13.1872458288696));
#80985=CARTESIAN_POINT('Ctrl Pts',(87.046706091828,65.1496953464628,12.9905783588265));
#80986=CARTESIAN_POINT('Ctrl Pts',(86.5192450187475,65.0656858501406,12.1991954050947));
#80987=CARTESIAN_POINT('Ctrl Pts',(87.0905702611622,64.9396716056574,10.8825794754981));
#80988=CARTESIAN_POINT('Ctrl Pts',(88.5057114362722,64.8136573611742,10.652019091688));
#80989=CARTESIAN_POINT('Ctrl Pts',(89.4673758848142,64.6876431166909,11.7140895996939));
#80990=CARTESIAN_POINT('Ctrl Pts',(89.0965192186417,64.5616288722077,13.0989494595771));
#80991=CARTESIAN_POINT('Ctrl Pts',(87.7320138686435,64.4356146277245,13.5380917202516));
#80992=CARTESIAN_POINT('Ctrl Pts',(86.6229267036533,64.3096003832413,12.63015179099));
#80993=CARTESIAN_POINT('Ctrl Pts',(86.7841629682104,64.1835861387581,11.2058088685007));
#80994=CARTESIAN_POINT('Ctrl Pts',(88.0682258576584,64.0575718942748,10.5687599281523));
#80995=CARTESIAN_POINT('Ctrl Pts',(89.2999043335523,63.9315576497916,11.3019663445296));
#80996=CARTESIAN_POINT('Ctrl Pts',(89.351979957255,63.8055434053084,12.7344294808954));
#80997=CARTESIAN_POINT('Ctrl Pts',(88.1767846159536,63.6795291608251,13.5551386896109));
#80998=CARTESIAN_POINT('Ctrl Pts',(86.8498641790876,63.553514916342,13.0129872916757));
#80999=CARTESIAN_POINT('Ctrl Pts',(86.5856174206176,63.4275006718586,11.6041493789204));
#81000=CARTESIAN_POINT('Ctrl Pts',(87.6258846736599,63.3014864273755,10.6179989983799));
#81001=CARTESIAN_POINT('Ctrl Pts',(89.0186102518103,63.1754721828922,10.9570623661457));
#81002=CARTESIAN_POINT('Ctrl Pts',(89.4891685219261,63.0494579384091,12.3110283750348));
#81003=CARTESIAN_POINT('Ctrl Pts',(88.6069032604118,62.9234436939258,13.4407437213165));
#81004=CARTESIAN_POINT('Ctrl Pts',(87.1792658825502,62.7974294494426,13.3122902566958));
#81005=CARTESIAN_POINT('Ctrl Pts',(86.5128336157025,62.6714152049593,12.0432288440844));
#81006=CARTESIAN_POINT('Ctrl Pts',(87.2175269354857,62.5454009604761,10.7950076606443));
#81007=CARTESIAN_POINT('Ctrl Pts',(88.6484087641475,62.4193867159929,10.7100018049911));
#81008=CARTESIAN_POINT('Ctrl Pts',(89.4959325163499,62.2933724715096,11.8660088547187));
#81009=CARTESIAN_POINT('Ctrl Pts',(88.9844423553679,62.1673582270265,13.2050482939942));
#81010=CARTESIAN_POINT('Ctrl Pts',(87.5820553429153,62.0413439825432,13.5016279174233));
#81011=CARTESIAN_POINT('Ctrl Pts',(86.5722395416138,61.91532973806,12.4843173189171));
#81012=CARTESIAN_POINT('Ctrl Pts',(86.8791808712292,61.7893154935768,11.0841616754428));
#81013=CARTESIAN_POINT('Ctrl Pts',(88.2219658674358,61.6633012490936,10.5825868954658));
#81014=CARTESIAN_POINT('Ctrl Pts',(89.3716743798821,61.5372870046104,11.4386354585839));
#81015=CARTESIAN_POINT('Ctrl Pts',(89.2760903337081,61.411272760127,12.8688496020078));
#81016=CARTESIAN_POINT('Ctrl Pts',(88.0226924844505,61.2852585156439,13.5642938035331));
#81017=CARTESIAN_POINT('Ctrl Pts',(86.7585936444956,61.1592442711607,12.8884958094639));
#81018=CARTESIAN_POINT('Ctrl Pts',(86.6407001993997,61.0332300266774,11.4599476158219));
#81019=CARTESIAN_POINT('Ctrl Pts',(87.7769085217668,60.9072157821942,10.5860600634779));
#81020=CARTESIAN_POINT('Ctrl Pts',(89.1273579441268,60.7812015377109,11.06661720223));
#81021=CARTESIAN_POINT('Ctrl Pts',(89.4561138142887,60.6551872932278,12.4618119498517));
#81022=CARTESIAN_POINT('Ctrl Pts',(88.4622979465789,60.5291730487445,13.4947586217789));
#81023=CARTESIAN_POINT('Ctrl Pts',(87.0554530817039,60.4031588042614,13.2201018684798));
#81024=CARTESIAN_POINT('Ctrl Pts',(86.5231271203599,60.277144559778,11.8892082300412));
#81025=CARTESIAN_POINT('Ctrl Pts',(87.3525060992781,60.151130315295,10.7201148568299));
#81026=CARTESIAN_POINT('Ctrl Pts',(88.7845403251703,60.0251160708116,10.7827788962033));
#81027=CARTESIAN_POINT('Ctrl Pts',(89.5086285318225,59.8991018263285,12.0198500643034));
#81028=CARTESIAN_POINT('Ctrl Pts',(88.862083401201,59.7730875818452,13.2991577677224));
#81029=CARTESIAN_POINT('Ctrl Pts',(87.4366246363239,59.647073337362,13.4498764314403));
#81030=CARTESIAN_POINT('Ctrl Pts',(86.5368356252177,59.5210590928787,12.3340679615629));
#81031=CARTESIAN_POINT('Ctrl Pts',(86.9862054968145,59.3950448483955,10.9729230300959));
#81032=CARTESIAN_POINT('Ctrl Pts',(88.3734698329432,59.2690306039123,10.6121648456238));
#81033=CARTESIAN_POINT('Ctrl Pts',(89.4290008812559,59.1430163594291,11.5819601910473));
#81034=CARTESIAN_POINT('Ctrl Pts',(89.1867740150826,59.0170021149458,12.9947499670796));
#81035=CARTESIAN_POINT('Ctrl Pts',(87.8684758615844,58.8909878704626,13.5575454756268));
#81036=CARTESIAN_POINT('Ctrl Pts',(86.6806161521516,58.7649736259794,12.7552748749792));
#81037=CARTESIAN_POINT('Ctrl Pts',(86.7103270314763,58.6389593814962,11.322178203569));
#81038=CARTESIAN_POINT('Ctrl Pts',(87.9304170293001,58.5129451370129,10.5698290803765));
#81039=CARTESIAN_POINT('Ctrl Pts',(89.2242567612607,58.3869308925298,11.1867792841674));
#81040=CARTESIAN_POINT('Ctrl Pts',(89.4077209038666,58.2609166480465,12.6083944621729));
#81041=CARTESIAN_POINT('Ctrl Pts',(88.3129026199372,58.1349024035633,13.5336088865802));
#81042=CARTESIAN_POINT('Ctrl Pts',(86.941782311371,58.0088881590801,13.1156640273043));
#81043=CARTESIAN_POINT('Ctrl Pts',(86.549212676552,57.8828739145968,11.7370640534991));
#81044=CARTESIAN_POINT('Ctrl Pts',(87.4944744164356,57.7568596701136,10.6595070716789));
#81045=CARTESIAN_POINT('Ctrl Pts',(88.9124616482187,57.6308454256303,10.8691758973496));
#81046=CARTESIAN_POINT('Ctrl Pts',(89.5054289494459,57.5048311811472,12.1741811025625));
#81047=CARTESIAN_POINT('Ctrl Pts',(88.730691179106,57.3788169366639,13.3801786950834));
#81048=CARTESIAN_POINT('Ctrl Pts',(87.2972902612201,57.2528026921807,13.3834366947466));
#81049=CARTESIAN_POINT('Ctrl Pts',(86.5170782618964,57.1267884476975,12.1809733722003));
#81050=CARTESIAN_POINT('Ctrl Pts',(87.1041071330646,57.0007742032142,10.8732861349864));
#81051=CARTESIAN_POINT('Ctrl Pts',(88.5211265995945,56.874759958731,10.6571735776611));
#81052=CARTESIAN_POINT('Ctrl Pts',(89.4712769401843,56.7487457142478,11.7304224473247));
#81053=CARTESIAN_POINT('Ctrl Pts',(89.0849782125712,56.6227314697646,13.1107927233745));
#81054=CARTESIAN_POINT('Ctrl Pts',(87.7157719679219,56.4967172252814,13.5349661143026));
#81055=CARTESIAN_POINT('Ctrl Pts',(86.6167591485887,56.3707029807981,12.6147380833783));
#81056=CARTESIAN_POINT('Ctrl Pts',(86.7937590056485,56.2446887363149,11.1923036010353));
#81057=CARTESIAN_POINT('Ctrl Pts',(88.0847808320441,56.1186744918317,10.5694782244428));
#81058=CARTESIAN_POINT('Ctrl Pts',(89.3082782584284,55.9926602473484,11.3162732790522));
#81059=CARTESIAN_POINT('Ctrl Pts',(89.3445034133909,55.8666460028653,12.7492200834052));
#81060=CARTESIAN_POINT('Ctrl Pts',(88.1603029454942,55.740631758382,13.5568821772229));
#81061=CARTESIAN_POINT('Ctrl Pts',(86.8394600525235,55.6146175138988,13.0000852141859));
#81062=CARTESIAN_POINT('Ctrl Pts',(86.5908134177302,55.4886032694155,11.5884111523135));
#81063=CARTESIAN_POINT('Ctrl Pts',(87.6419250563981,55.3625890249324,10.6138275853401));
#81064=CARTESIAN_POINT('Ctrl Pts',(89.0308149964968,55.2365747804491,10.9682758047605));
#81065=CARTESIAN_POINT('Ctrl Pts',(89.4863677289041,55.1105605359659,12.3273639232995));
#81066=CARTESIAN_POINT('Ctrl Pts',(88.5916602659388,54.9845462914826,13.4472511326524));
#81067=CARTESIAN_POINT('Ctrl Pts',(87.165531091104,54.8585320469995,13.3030138883554));
#81068=CARTESIAN_POINT('Ctrl Pts',(86.5131771532775,54.7325178025162,12.0266584732144));
#81069=CARTESIAN_POINT('Ctrl Pts',(87.2316343902018,54.606503558033,10.7863085207138));
#81070=CARTESIAN_POINT('Ctrl Pts',(88.6633689612688,54.4804893135498,10.7171353758561));
#81071=CARTESIAN_POINT('Ctrl Pts',(89.4980538451014,54.3544750690665,11.8824464719411));
#81072=CARTESIAN_POINT('Ctrl Pts',(88.9717833711079,54.2284608245833,13.2157462109946));
#81073=CARTESIAN_POINT('Ctrl Pts',(87.5662015790156,54.1024465801001,13.4967953734143));
#81074=CARTESIAN_POINT('Ctrl Pts',(86.5677004021856,53.9764323356168,12.4683770704725));
#81075=CARTESIAN_POINT('Ctrl Pts',(86.8901105878214,53.8504180911337,11.0717022772023));
#81076=CARTESIAN_POINT('Ctrl Pts',(88.2383615364273,53.7244038466504,10.5850112196082));
#81077=CARTESIAN_POINT('Ctrl Pts',(89.3785306444292,53.5983896021672,11.4537247576126));
#81078=CARTESIAN_POINT('Ctrl Pts',(89.2671323235476,53.4723753576839,12.8827941121466));
#81079=CARTESIAN_POINT('Ctrl Pts',(88.0061185926342,53.3463611132008,13.5643314745901));
#81080=CARTESIAN_POINT('Ctrl Pts',(86.7495723378244,53.2203468687175,12.8745921648102));
#81081=CARTESIAN_POINT('Ctrl Pts',(86.6474878000429,53.0943326242343,11.4448273054174));
#81082=CARTESIAN_POINT('Ctrl Pts',(87.7932930008493,52.9683183797511,10.5835612328527));
#81083=CARTESIAN_POINT('Ctrl Pts',(89.1383441858098,52.8423041352678,11.0790267872718));
#81084=CARTESIAN_POINT('Ctrl Pts',(89.4516471831037,52.7162898907846,12.4777726677943));
#81085=CARTESIAN_POINT('Ctrl Pts',(88.4464663142398,52.5902756463014,13.499663183749));
#81086=CARTESIAN_POINT('Ctrl Pts',(87.042745597686,52.4642614018182,13.2094616078837));
#81087=CARTESIAN_POINT('Ctrl Pts',(86.5251737046872,52.338247157335,11.8727611383899));
#81088=CARTESIAN_POINT('Ctrl Pts',(87.3674337144834,52.2122329128517,10.7129133557097));
#81089=CARTESIAN_POINT('Ctrl Pts',(88.7986871777436,52.0862186683684,10.7914138120163));
#81090=CARTESIAN_POINT('Ctrl Pts',(89.5090473935824,51.9602044238853,12.0364187112151));
#81091=CARTESIAN_POINT('Ctrl Pts',(88.8483909162438,51.834190179402,13.3084964581282));
#81092=CARTESIAN_POINT('Ctrl Pts',(87.42135222593,51.7081759349188,13.4434384147102));
#81093=CARTESIAN_POINT('Ctrl Pts',(86.5339605868047,51.5821616904356,12.3177452426549));
#81094=CARTESIAN_POINT('Ctrl Pts',(86.9983591733833,51.4561474459524,10.9616543695276));
#81095=CARTESIAN_POINT('Ctrl Pts',(88.389528948128,51.3301332014691,10.6162630137755));
#81096=CARTESIAN_POINT('Ctrl Pts',(89.434268496194,51.204118956986,11.597675205714));
#81097=CARTESIAN_POINT('Ctrl Pts',(89.1764283892337,51.0781047125027,13.0076980648546));
#81098=CARTESIAN_POINT('Ctrl Pts',(87.8519869502598,50.9520904680195,13.5558792121182));
#81099=CARTESIAN_POINT('Ctrl Pts',(86.6730714212938,50.8260762235362,12.740513844204));
#81100=CARTESIAN_POINT('Ctrl Pts',(86.7186378916432,50.7000619790531,11.3078424883874));
#81101=CARTESIAN_POINT('Ctrl Pts',(87.9469644498306,50.5740477345697,10.5690172567477));
#81102=CARTESIAN_POINT('Ctrl Pts',(89.2339223286193,50.4480334900867,11.2002773553426));
#81103=CARTESIAN_POINT('Ctrl Pts',(89.4016070035495,50.3220192456032,12.6237629030343));
#81104=CARTESIAN_POINT('Ctrl Pts',(88.2967080575638,50.1960050011202,13.536954610423));
#81105=CARTESIAN_POINT('Ctrl Pts',(86.9301216186333,50.0699907566368,13.1035806341709));
#81106=CARTESIAN_POINT('Ctrl Pts',(86.5531718275547,49.9439765121537,11.7212995011988));
#81107=CARTESIAN_POINT('Ctrl Pts',(87.5095953909142,49.8179622676705,10.6531063522201));
#81108=CARTESIAN_POINT('Ctrl Pts',(88.9267744927432,49.6919367901709,10.8808357729695));
#81109=CARTESIAN_POINT('Ctrl Pts',(89.3094755969595,49.6079160608325,11.7516938683196));
#81110=CARTESIAN_POINT('Ctrl Pts',(89.2742633450769,49.565900079655,12.1718452204411));
#81111=CARTESIAN_POINT('Ctrl Pts',(87.3512658244469,65.1072380988749,13.316638536706));
#81112=CARTESIAN_POINT('Ctrl Pts',(86.9354257671071,65.0652333507139,13.0972754758862));
#81113=CARTESIAN_POINT('Ctrl Pts',(86.3470952443779,64.9812238543917,12.2145662664107));
#81114=CARTESIAN_POINT('Ctrl Pts',(86.9843518983242,64.8552096099085,10.7460117557066));
#81115=CARTESIAN_POINT('Ctrl Pts',(88.5628015504014,64.7291953654253,10.4888445104814));
#81116=CARTESIAN_POINT('Ctrl Pts',(89.6354428818203,64.603181120942,11.6734788447291));
#81117=CARTESIAN_POINT('Ctrl Pts',(89.2217890457325,64.4771668764588,13.2181526924379));
#81118=CARTESIAN_POINT('Ctrl Pts',(87.6998186353989,64.3511526319757,13.7079723378312));
#81119=CARTESIAN_POINT('Ctrl Pts',(86.4627418825683,64.2251383874924,12.6952553802185));
#81120=CARTESIAN_POINT('Ctrl Pts',(86.6425849471111,64.0991241430091,11.1065420914071));
#81121=CARTESIAN_POINT('Ctrl Pts',(88.074829769566,63.9731098985258,10.3959771697335));
#81122=CARTESIAN_POINT('Ctrl Pts',(89.4486449732643,63.8470956540426,11.2137962207137));
#81123=CARTESIAN_POINT('Ctrl Pts',(89.5067301675622,63.7210814095594,12.8115668028847));
#81124=CARTESIAN_POINT('Ctrl Pts',(88.1959162995001,63.5950671650762,13.7269865417335));
#81125=CARTESIAN_POINT('Ctrl Pts',(86.7158681327567,63.469052920593,13.1222704183564));
#81126=CARTESIAN_POINT('Ctrl Pts',(86.421127077019,63.3430386761097,11.5508514303896));
#81127=CARTESIAN_POINT('Ctrl Pts',(87.5814420424177,63.2170244316266,10.4508984699093));
#81128=CARTESIAN_POINT('Ctrl Pts',(89.1348893188699,63.0910101871434,10.8290900343238));
#81129=CARTESIAN_POINT('Ctrl Pts',(89.6597504075091,62.9649959426601,12.339304854756));
#81130=CARTESIAN_POINT('Ctrl Pts',(88.6756709958075,62.8389816981769,13.5993902982778));
#81131=CARTESIAN_POINT('Ctrl Pts',(87.0832830687143,62.7129674536937,13.4561131962439));
#81132=CARTESIAN_POINT('Ctrl Pts',(86.3399439600512,62.5869532092103,12.040601033618));
#81133=CARTESIAN_POINT('Ctrl Pts',(87.1259594792068,62.4609389647273,10.6483340800663));
#81134=CARTESIAN_POINT('Ctrl Pts',(88.7219662694403,62.3349247202439,10.5535184774675));
#81135=CARTESIAN_POINT('Ctrl Pts',(89.6672949725552,62.2089104757607,11.8429297090355));
#81136=CARTESIAN_POINT('Ctrl Pts',(89.0967784185581,62.0828962312775,13.3364954212178));
#81137=CARTESIAN_POINT('Ctrl Pts',(87.5325547701926,61.9568819867942,13.6673005816136));
#81138=CARTESIAN_POINT('Ctrl Pts',(86.4062053795725,61.830867742311,12.5325914879137));
#81139=CARTESIAN_POINT('Ctrl Pts',(86.7485679957279,61.7048534978279,10.9708567103754));
#81140=CARTESIAN_POINT('Ctrl Pts',(88.2463115052484,61.5788392533447,10.4113997806569));
#81141=CARTESIAN_POINT('Ctrl Pts',(89.5286973430571,61.4528250088614,11.3662370650074));
#81142=CARTESIAN_POINT('Ctrl Pts',(89.4220828178908,61.3268107643783,12.9614991185673));
#81143=CARTESIAN_POINT('Ctrl Pts',(88.0240418069501,61.2007965198949,13.737198163471));
#81144=CARTESIAN_POINT('Ctrl Pts',(86.6140649020221,61.0747822754117,12.9834125148202));
#81145=CARTESIAN_POINT('Ctrl Pts',(86.4825664546115,60.9487680309286,11.3900086630425));
#81146=CARTESIAN_POINT('Ctrl Pts',(87.7498941690976,60.8227537864452,10.4152737551668));
#81147=CARTESIAN_POINT('Ctrl Pts',(89.2561865859698,60.696739541962,10.9512875902581));
#81148=CARTESIAN_POINT('Ctrl Pts',(89.622881158923,60.5707252974788,12.507488980407));
#81149=CARTESIAN_POINT('Ctrl Pts',(88.5143781076331,60.4447110529956,13.6596385634979));
#81150=CARTESIAN_POINT('Ctrl Pts',(86.9451821669415,60.3186968085123,13.3532861908084));
#81151=CARTESIAN_POINT('Ctrl Pts',(86.351425343768,60.1926825640292,11.8688063117025));
#81152=CARTESIAN_POINT('Ctrl Pts',(87.276515351563,60.066668319546,10.5647985839596));
#81153=CARTESIAN_POINT('Ctrl Pts',(88.8738075266325,59.9406540750628,10.6346941059655));
#81154=CARTESIAN_POINT('Ctrl Pts',(89.681456118848,59.8146398305795,12.0145243230676));
#81155=CARTESIAN_POINT('Ctrl Pts',(88.9602991385892,59.6886255860963,13.4414652070427));
#81156=CARTESIAN_POINT('Ctrl Pts',(87.3703412382439,59.562611341613,13.6095769307997));
#81157=CARTESIAN_POINT('Ctrl Pts',(86.3667158215692,59.4365970971297,12.3650032288681));
#81158=CARTESIAN_POINT('Ctrl Pts',(86.8679433527522,59.3105828526465,10.846781032179));
#81159=CARTESIAN_POINT('Ctrl Pts',(88.415299155279,59.1845686081633,10.4443910510384));
#81160=CARTESIAN_POINT('Ctrl Pts',(89.5926393707076,59.05855436368,11.5261015916497));
#81161=CARTESIAN_POINT('Ctrl Pts',(89.3224593212823,58.9325401191969,13.1019284912259));
#81162=CARTESIAN_POINT('Ctrl Pts',(87.8520284566294,58.8065258747136,13.7296710728716));
#81163=CARTESIAN_POINT('Ctrl Pts',(86.5270887417454,58.6805116302305,12.8348177729066));
#81164=CARTESIAN_POINT('Ctrl Pts',(86.5602282814311,58.5544973857473,11.2363405452162));
#81165=CARTESIAN_POINT('Ctrl Pts',(87.9211176869828,58.4284831412641,10.39716970302));
#81166=CARTESIAN_POINT('Ctrl Pts',(89.3642676077659,58.3024688967808,11.085316477102));
#81167=CARTESIAN_POINT('Ctrl Pts',(89.5689036661028,58.1764546522976,12.6709872374314));
#81168=CARTESIAN_POINT('Ctrl Pts',(88.3477424351596,58.0504404078143,13.7029721813991));
#81169=CARTESIAN_POINT('Ctrl Pts',(86.8183936944983,57.9244261633312,13.2367961352814));
#81170=CARTESIAN_POINT('Ctrl Pts',(86.3805211949948,57.7984119188478,11.6991045697475));
#81171=CARTESIAN_POINT('Ctrl Pts',(87.4348669314369,57.6723976743646,10.4971966096353));
#81172=CARTESIAN_POINT('Ctrl Pts',(89.0164910775108,57.5463834298814,10.7310613934125));
#81173=CARTESIAN_POINT('Ctrl Pts',(89.6778873019851,57.4203691853982,12.1866652924135));
#81174=CARTESIAN_POINT('Ctrl Pts',(88.8137441440068,57.2943549409149,13.5318360172864));
#81175=CARTESIAN_POINT('Ctrl Pts',(87.2149275595431,57.1683406964318,13.5354699928398));
#81176=CARTESIAN_POINT('Ctrl Pts',(86.3446784419712,57.0423264519486,12.1942413956571));
#81177=CARTESIAN_POINT('Ctrl Pts',(86.9994509365831,56.9163122074654,10.7356459559154));
#81178=CARTESIAN_POINT('Ctrl Pts',(88.5799956364829,56.7902979629822,10.4945938284533));
#81179=CARTESIAN_POINT('Ctrl Pts',(89.6397941222479,56.6642837184989,11.6916965166575));
#81180=CARTESIAN_POINT('Ctrl Pts',(89.2089161978942,56.5382694740156,13.2313626787977));
#81181=CARTESIAN_POINT('Ctrl Pts',(87.6817024057294,56.4122552295323,13.7044860343376));
#81182=CARTESIAN_POINT('Ctrl Pts',(86.4558625864833,56.2862409850493,12.6780629178376));
#81183=CARTESIAN_POINT('Ctrl Pts',(86.6532883753072,56.1602267405659,11.0914783047638));
#81184=CARTESIAN_POINT('Ctrl Pts',(88.0932952018629,56.0342124960827,10.3967783580177));
#81185=CARTESIAN_POINT('Ctrl Pts',(89.4579852560851,55.9081982515995,11.2297541874641));
#81186=CARTESIAN_POINT('Ctrl Pts',(89.4983908242738,55.7821840071162,12.8280642533132));
#81187=CARTESIAN_POINT('Ctrl Pts',(88.177532630464,55.6561697626331,13.7289312292763));
#81188=CARTESIAN_POINT('Ctrl Pts',(86.7042633612723,55.5301555181499,13.1078794303172));
#81189=CARTESIAN_POINT('Ctrl Pts',(86.4269226965508,55.4041412736666,11.5332969992495));
#81190=CARTESIAN_POINT('Ctrl Pts',(87.5993334987596,55.2781270291835,10.4462456723107));
#81191=CARTESIAN_POINT('Ctrl Pts',(89.1485025013162,55.1521127847002,10.8415975131473));
#81192=CARTESIAN_POINT('Ctrl Pts',(89.6566264006262,55.0260985402169,12.3575255389735));
#81193=CARTESIAN_POINT('Ctrl Pts',(88.6586689470046,54.9000842957338,13.6066486703326));
#81194=CARTESIAN_POINT('Ctrl Pts',(87.0679632708306,54.7740700512506,13.4457663272269));
#81195=CARTESIAN_POINT('Ctrl Pts',(86.3403271421501,54.6480558067672,12.0221184280699));
#81196=CARTESIAN_POINT('Ctrl Pts',(87.1416949460142,54.522041562284,10.6386310521009));
#81197=CARTESIAN_POINT('Ctrl Pts',(88.7386528858405,54.3960273178008,10.5614752683855));
#81198=CARTESIAN_POINT('Ctrl Pts',(89.6696611044214,54.2700130733175,11.8612642410538));
#81199=CARTESIAN_POINT('Ctrl Pts',(89.082658576911,54.1439988288344,13.3484278868009));
#81200=CARTESIAN_POINT('Ctrl Pts',(87.5148714686594,54.0179845843512,13.661910357978));
#81201=CARTESIAN_POINT('Ctrl Pts',(86.401142419652,53.891970339868,12.5148117214466));
#81202=CARTESIAN_POINT('Ctrl Pts',(86.7607590107698,53.7659560953848,10.9569594871417));
#81203=CARTESIAN_POINT('Ctrl Pts',(88.2645992481749,53.6399418509016,10.414103873836));
#81204=CARTESIAN_POINT('Ctrl Pts',(89.5363448262758,53.5139276064182,11.3830676817832));
#81205=CARTESIAN_POINT('Ctrl Pts',(89.4120910458545,53.3879133619351,12.9770528368564));
#81206=CARTESIAN_POINT('Ctrl Pts',(88.0055552741355,53.2618991174519,13.7372401817996));
#81207=CARTESIAN_POINT('Ctrl Pts',(86.6040025290045,53.1358848729685,12.9679043779273));
#81208=CARTESIAN_POINT('Ctrl Pts',(86.4901373500544,53.0098706284853,11.373143456152));
#81209=CARTESIAN_POINT('Ctrl Pts',(87.7681694307903,52.8838563840021,10.4124865573944));
#81210=CARTESIAN_POINT('Ctrl Pts',(89.2684406491452,52.7578421395189,10.9651292518083));
#81211=CARTESIAN_POINT('Ctrl Pts',(89.6178990747577,52.6318278950357,12.5252915785692));
#81212=CARTESIAN_POINT('Ctrl Pts',(88.4967194916609,52.5058136505524,13.6651091160275));
#81213=CARTESIAN_POINT('Ctrl Pts',(86.9310082286238,52.3797994060693,13.3414180352269));
#81214=CARTESIAN_POINT('Ctrl Pts',(86.353708105641,52.253785161586,11.8504612118982));
#81215=CARTESIAN_POINT('Ctrl Pts',(87.2931656260668,52.1277709171029,10.5567660235778));
#81216=CARTESIAN_POINT('Ctrl Pts',(88.8895869378427,52.0017566726195,10.6443254982963));
#81217=CARTESIAN_POINT('Ctrl Pts',(89.6819233176056,51.8757424281364,12.0330050057112));
#81218=CARTESIAN_POINT('Ctrl Pts',(88.9450265293989,51.7497281836532,13.4518815901437));
#81219=CARTESIAN_POINT('Ctrl Pts',(87.3533063788977,51.6237139391698,13.6023959615463));
#81220=CARTESIAN_POINT('Ctrl Pts',(86.3635090013151,51.4976996946866,12.3467968545257));
#81221=CARTESIAN_POINT('Ctrl Pts',(86.8814995737771,51.3716854502034,10.8342119587422));
#81222=CARTESIAN_POINT('Ctrl Pts',(88.4332115058078,51.2456712057202,10.4489621512275));
#81223=CARTESIAN_POINT('Ctrl Pts',(89.5985148728217,51.119656961237,11.5436301321723));
#81224=CARTESIAN_POINT('Ctrl Pts',(89.3109198015447,50.9936427167538,13.1163708103297));
#81225=CARTESIAN_POINT('Ctrl Pts',(87.8336367111264,50.8676284722706,13.7278125211585));
#81226=CARTESIAN_POINT('Ctrl Pts',(86.5186733426272,50.7416142277874,12.8183533068156));
#81227=CARTESIAN_POINT('Ctrl Pts',(86.5694982218224,50.6155999833041,11.2203504764948));
#81228=CARTESIAN_POINT('Ctrl Pts',(87.9395746937033,50.4895857388209,10.3962641942645));
#81229=CARTESIAN_POINT('Ctrl Pts',(89.3750485896936,50.3635714943377,11.1003722369971));
#81230=CARTESIAN_POINT('Ctrl Pts',(89.5620842165681,50.2375572498545,12.6881292092412));
#81231=CARTESIAN_POINT('Ctrl Pts',(88.3296790067231,50.1115430053713,13.7067040045759));
#81232=CARTESIAN_POINT('Ctrl Pts',(86.8053873480519,49.9855287608879,13.223318308459));
#81233=CARTESIAN_POINT('Ctrl Pts',(86.3849372353393,49.8595145164047,11.6815207749069));
#81234=CARTESIAN_POINT('Ctrl Pts',(87.4517328790361,49.7335002719215,10.4900572417896));
#81235=CARTESIAN_POINT('Ctrl Pts',(89.0324556362825,49.6074747944219,10.7440668284456));
#81236=CARTESIAN_POINT('Ctrl Pts',(89.4593207684858,49.5234540650835,11.7154226774526));
#81237=CARTESIAN_POINT('Ctrl Pts',(89.4200449932413,49.4814380839061,12.1840598475387));
#81238=CARTESIAN_POINT('Ctrl Pts',(87.2830088589676,65.022776103126,13.4460312445424));
#81239=CARTESIAN_POINT('Ctrl Pts',(86.8241454423862,64.9807713549649,13.2039725929459));
#81240=CARTESIAN_POINT('Ctrl Pts',(86.1749454700084,64.8967618586428,12.2299371277265));
#81241=CARTESIAN_POINT('Ctrl Pts',(86.8781335354862,64.7707476141595,10.609444035915));
#81242=CARTESIAN_POINT('Ctrl Pts',(88.6198916645305,64.6447333696763,10.3256699292747));
#81243=CARTESIAN_POINT('Ctrl Pts',(89.8035098788265,64.5187191251931,11.6328680897644));
#81244=CARTESIAN_POINT('Ctrl Pts',(89.347058872823,64.3927048807099,13.3373559252986));
#81245=CARTESIAN_POINT('Ctrl Pts',(87.6676234021542,64.2666906362266,13.8778529554108));
#81246=CARTESIAN_POINT('Ctrl Pts',(86.3025570614835,64.1406763917435,12.7603589694471));
#81247=CARTESIAN_POINT('Ctrl Pts',(86.5010069260116,64.0146621472602,11.0072753143134));
#81248=CARTESIAN_POINT('Ctrl Pts',(88.0814336814738,63.888647902777,10.2231944113149));
#81249=CARTESIAN_POINT('Ctrl Pts',(89.5973856129763,63.7626336582937,11.1256260968977));
#81250=CARTESIAN_POINT('Ctrl Pts',(89.6614803778694,63.6366194138105,12.8887041248741));
#81251=CARTESIAN_POINT('Ctrl Pts',(88.2150479830468,63.5106051693273,13.8988343938561));
#81252=CARTESIAN_POINT('Ctrl Pts',(86.5818720864256,63.3845909248441,13.2315535450371));
#81253=CARTESIAN_POINT('Ctrl Pts',(86.2566367334206,63.2585766803608,11.4975534818589));
#81254=CARTESIAN_POINT('Ctrl Pts',(87.5369994111753,63.1325624358777,10.2837979414388));
#81255=CARTESIAN_POINT('Ctrl Pts',(89.2511683859297,63.0065481913943,10.7011177025018));
#81256=CARTESIAN_POINT('Ctrl Pts',(89.830332293092,62.8805339469112,12.3675813344771));
#81257=CARTESIAN_POINT('Ctrl Pts',(88.7444387312032,62.7545197024279,13.7580368752391));
#81258=CARTESIAN_POINT('Ctrl Pts',(86.9873002548784,62.6285054579448,13.5999361357919));
#81259=CARTESIAN_POINT('Ctrl Pts',(86.1670543043998,62.5024912134615,12.0379732231516));
#81260=CARTESIAN_POINT('Ctrl Pts',(87.0343920229282,62.3764769689783,10.5016604994881));
#81261=CARTESIAN_POINT('Ctrl Pts',(88.7955237747332,62.2504627244951,10.3970351499439));
#81262=CARTESIAN_POINT('Ctrl Pts',(89.8386574287603,62.1244484800117,11.8198505633521));
#81263=CARTESIAN_POINT('Ctrl Pts',(89.2091144817484,61.9984342355287,13.4679425484414));
#81264=CARTESIAN_POINT('Ctrl Pts',(87.4830541974697,61.8724199910453,13.8329732458038));
#81265=CARTESIAN_POINT('Ctrl Pts',(86.2401712175313,61.7464057465622,12.5808656569103));
#81266=CARTESIAN_POINT('Ctrl Pts',(86.6179551202264,61.6203915020788,10.857551745308));
#81267=CARTESIAN_POINT('Ctrl Pts',(88.270657143061,61.4943772575958,10.240212665848));
#81268=CARTESIAN_POINT('Ctrl Pts',(89.6857203062321,61.3683630131124,11.293838671431));
#81269=CARTESIAN_POINT('Ctrl Pts',(89.5680753020734,61.2423487686293,13.0541486351269));
#81270=CARTESIAN_POINT('Ctrl Pts',(88.0253911294497,61.116334524146,13.9101025234088));
#81271=CARTESIAN_POINT('Ctrl Pts',(86.4695361595484,60.9903202796628,13.0783292201763));
#81272=CARTESIAN_POINT('Ctrl Pts',(86.3244327098233,60.8643060351796,11.320069710263));
#81273=CARTESIAN_POINT('Ctrl Pts',(87.7228798164282,60.7382917906963,10.2444874468557));
#81274=CARTESIAN_POINT('Ctrl Pts',(89.3850152278127,60.6122775462132,10.8359579782862));
#81275=CARTESIAN_POINT('Ctrl Pts',(89.789648503557,60.4862633017299,12.5531660109623));
#81276=CARTESIAN_POINT('Ctrl Pts',(88.5664582686874,60.3602490572467,13.8245185052168));
#81277=CARTESIAN_POINT('Ctrl Pts',(86.834911252179,60.2342348127635,13.486470513137));
#81278=CARTESIAN_POINT('Ctrl Pts',(86.1797235671763,60.1082205682802,11.8484043933639));
#81279=CARTESIAN_POINT('Ctrl Pts',(87.2005246038479,59.982206323797,10.4094823110891));
#81280=CARTESIAN_POINT('Ctrl Pts',(88.9630747280948,59.8561920793138,10.4866093157278));
#81281=CARTESIAN_POINT('Ctrl Pts',(89.8542837058732,59.7301778348306,12.0091985818318));
#81282=CARTESIAN_POINT('Ctrl Pts',(89.0585148759775,59.6041635903473,13.5837726463632));
#81283=CARTESIAN_POINT('Ctrl Pts',(87.304057840164,59.4781493458641,13.769277430159));
#81284=CARTESIAN_POINT('Ctrl Pts',(86.1965960179204,59.3521351013809,12.3959384961732));
#81285=CARTESIAN_POINT('Ctrl Pts',(86.74968120869,59.2261208568977,10.7206390342622));
#81286=CARTESIAN_POINT('Ctrl Pts',(88.4571284776149,59.1001066124145,10.2766172564529));
#81287=CARTESIAN_POINT('Ctrl Pts',(89.7562778601591,58.9740923679312,11.4702429922521));
#81288=CARTESIAN_POINT('Ctrl Pts',(89.4581446274822,58.848078123448,13.2091070153721));
#81289=CARTESIAN_POINT('Ctrl Pts',(87.8355810516741,58.7220638789647,13.9017966701166));
#81290=CARTESIAN_POINT('Ctrl Pts',(86.3735613313395,58.5960496344816,12.9143606708339));
#81291=CARTESIAN_POINT('Ctrl Pts',(86.4101295313855,58.4700353899983,11.1505028868634));
#81292=CARTESIAN_POINT('Ctrl Pts',(87.9118183446658,58.3440211455151,10.2245103256635));
#81293=CARTESIAN_POINT('Ctrl Pts',(89.5042784542709,58.2180069010319,10.9838536700367));
#81294=CARTESIAN_POINT('Ctrl Pts',(89.7300864283392,58.0919926565487,12.7335800126899));
#81295=CARTESIAN_POINT('Ctrl Pts',(88.3825822503817,57.9659784120654,13.8723354762181));
#81296=CARTESIAN_POINT('Ctrl Pts',(86.6950050776261,57.8399641675822,13.3579282432583));
#81297=CARTESIAN_POINT('Ctrl Pts',(86.2118297134374,57.713949923099,11.661145085996));
#81298=CARTESIAN_POINT('Ctrl Pts',(87.3752594464383,57.5879356786158,10.3348861475917));
#81299=CARTESIAN_POINT('Ctrl Pts',(89.1205205068032,57.4619214341325,10.5929468894755));
#81300=CARTESIAN_POINT('Ctrl Pts',(89.8503456545239,57.3359071896493,12.1991494822645));
#81301=CARTESIAN_POINT('Ctrl Pts',(88.8967971089079,57.209892945166,13.6834933394896));
#81302=CARTESIAN_POINT('Ctrl Pts',(87.132564857866,57.0838787006829,13.687503290933));
#81303=CARTESIAN_POINT('Ctrl Pts',(86.172278622046,56.9578644561996,12.2075094191137));
#81304=CARTESIAN_POINT('Ctrl Pts',(86.8947947401016,56.8318502117164,10.5980057768445));
#81305=CARTESIAN_POINT('Ctrl Pts',(88.6388646733714,56.7058359672331,10.3320140792455));
#81306=CARTESIAN_POINT('Ctrl Pts',(89.8083113043114,56.57982172275,11.6529705859901));
#81307=CARTESIAN_POINT('Ctrl Pts',(89.3328541832171,56.4538074782667,13.3519326342209));
#81308=CARTESIAN_POINT('Ctrl Pts',(87.6476328435369,56.3277932337835,13.8740059543726));
#81309=CARTESIAN_POINT('Ctrl Pts',(86.2949660243777,56.2017789893003,12.7413877522968));
#81310=CARTESIAN_POINT('Ctrl Pts',(86.5128177449663,56.0757647448171,10.9906530084923));
#81311=CARTESIAN_POINT('Ctrl Pts',(88.1018095716815,55.9497505003338,10.2240784915925));
#81312=CARTESIAN_POINT('Ctrl Pts',(89.6076922537419,55.8237362558506,11.143235095876));
#81313=CARTESIAN_POINT('Ctrl Pts',(89.6522782351566,55.6977220113674,12.9069084232212));
#81314=CARTESIAN_POINT('Ctrl Pts',(88.194762315434,55.5717077668842,13.9009802813298));
#81315=CARTESIAN_POINT('Ctrl Pts',(86.5690666700211,55.4456935224009,13.2156736464485));
#81316=CARTESIAN_POINT('Ctrl Pts',(86.2630319753712,55.3196792779177,11.4781828461855));
#81317=CARTESIAN_POINT('Ctrl Pts',(87.5567419411211,55.1936650334345,10.2786637592813));
#81318=CARTESIAN_POINT('Ctrl Pts',(89.2661900061356,55.0676507889513,10.7149192215342));
#81319=CARTESIAN_POINT('Ctrl Pts',(89.8268850723484,54.941636544468,12.3876871546476));
#81320=CARTESIAN_POINT('Ctrl Pts',(88.7256776280701,54.8156222999848,13.7660462080128));
#81321=CARTESIAN_POINT('Ctrl Pts',(86.9703954505572,54.6896080555015,13.5885187660983));
#81322=CARTESIAN_POINT('Ctrl Pts',(86.1674771310224,54.5635938110184,12.0175783829253));
#81323=CARTESIAN_POINT('Ctrl Pts',(87.0517555018266,54.4375795665351,10.4909535834882));
#81324=CARTESIAN_POINT('Ctrl Pts',(88.8139368104121,54.3115653220519,10.405815160915));
#81325=CARTESIAN_POINT('Ctrl Pts',(89.8412683637416,54.1855510775687,11.8400820101666));
#81326=CARTESIAN_POINT('Ctrl Pts',(89.193533782714,54.0595368330855,13.4811095626073));
#81327=CARTESIAN_POINT('Ctrl Pts',(87.4635413583032,53.9335225886023,13.8270253425417));
#81328=CARTESIAN_POINT('Ctrl Pts',(86.2345844371186,53.807508344119,12.5612463724207));
#81329=CARTESIAN_POINT('Ctrl Pts',(86.6314074337182,53.6814940996358,10.8422166970809));
#81330=CARTESIAN_POINT('Ctrl Pts',(88.2908369599225,53.5554798551525,10.2431965280638));
#81331=CARTESIAN_POINT('Ctrl Pts',(89.6941590081224,53.4294656106693,11.3124106059539));
#81332=CARTESIAN_POINT('Ctrl Pts',(89.5570497681611,53.3034513661862,13.0713115615662));
#81333=CARTESIAN_POINT('Ctrl Pts',(88.0049919556368,53.1774371217029,13.9101488890089));
#81334=CARTESIAN_POINT('Ctrl Pts',(86.4584327201847,53.0514228772197,13.0612165910444));
#81335=CARTESIAN_POINT('Ctrl Pts',(86.3327869000657,52.9254086327364,11.3014596068867));
#81336=CARTESIAN_POINT('Ctrl Pts',(87.7430458607311,52.7993943882532,10.2414118819361));
#81337=CARTESIAN_POINT('Ctrl Pts',(89.3985371124807,52.67338014377,10.8512317163449));
#81338=CARTESIAN_POINT('Ctrl Pts',(89.7841509664117,52.5473658992868,12.5728104893443));
#81339=CARTESIAN_POINT('Ctrl Pts',(88.5469726690822,52.4213516548036,13.830555048306));
#81340=CARTESIAN_POINT('Ctrl Pts',(86.8192708595616,52.2953374103203,13.4733744625701));
#81341=CARTESIAN_POINT('Ctrl Pts',(86.1822425065949,52.1693231658371,11.8281612854064));
#81342=CARTESIAN_POINT('Ctrl Pts',(87.2188975376501,52.0433089213539,10.4006186914459));
#81343=CARTESIAN_POINT('Ctrl Pts',(88.9804866979417,51.9172946768706,10.4972371845761));
#81344=CARTESIAN_POINT('Ctrl Pts',(89.8547992416286,51.7912804323874,12.0295913002075));
#81345=CARTESIAN_POINT('Ctrl Pts',(89.0416621425541,51.6652661879042,13.5952667221593));
#81346=CARTESIAN_POINT('Ctrl Pts',(87.2852605318656,51.539251943421,13.7613535083824));
#81347=CARTESIAN_POINT('Ctrl Pts',(86.1930574158255,51.4132376989378,12.3758484663964));
#81348=CARTESIAN_POINT('Ctrl Pts',(86.7646399741709,51.2872234544545,10.7067695479568));
#81349=CARTESIAN_POINT('Ctrl Pts',(88.4768940634877,51.1612092099713,10.2816612886795));
#81350=CARTESIAN_POINT('Ctrl Pts',(89.7627612494493,51.0351949654881,11.4895850586306));
#81351=CARTESIAN_POINT('Ctrl Pts',(89.4454112138556,50.9091807210049,13.2250435558049));
#81352=CARTESIAN_POINT('Ctrl Pts',(87.8152864719929,50.7831664765216,13.8997458301988));
#81353=CARTESIAN_POINT('Ctrl Pts',(86.3642752639605,50.6571522320384,12.8961927694272));
#81354=CARTESIAN_POINT('Ctrl Pts',(86.4203585520016,50.5311379875552,11.1328584646021));
#81355=CARTESIAN_POINT('Ctrl Pts',(87.9321849375758,50.4051237430719,10.2235111317813));
#81356=CARTESIAN_POINT('Ctrl Pts',(89.5161748507681,50.2791094985888,11.0004671186517));
#81357=CARTESIAN_POINT('Ctrl Pts',(89.7225614295866,50.1530952541055,12.7524955154482));
#81358=CARTESIAN_POINT('Ctrl Pts',(88.3626499558826,50.0270810096223,13.8764533987288));
#81359=CARTESIAN_POINT('Ctrl Pts',(86.6806530774701,49.901066765139,13.343055982747));
#81360=CARTESIAN_POINT('Ctrl Pts',(86.2167026431241,49.7750525206558,11.6417420486151));
#81361=CARTESIAN_POINT('Ctrl Pts',(87.3938703671579,49.6490382761727,10.3270081313591));
#81362=CARTESIAN_POINT('Ctrl Pts',(89.1381367798218,49.523012798673,10.6072978839217));
#81363=CARTESIAN_POINT('Ctrl Pts',(89.6091659400121,49.4389920693345,11.6791514865856));
#81364=CARTESIAN_POINT('Ctrl Pts',(89.5658266414056,49.3969760881572,12.1962744746363));
#81365=CARTESIAN_POINT('Ctrl Pts',(87.2147518934884,64.938314107377,13.5754239523789));
#81366=CARTESIAN_POINT('Ctrl Pts',(86.7128651176654,64.8963093592159,13.3106697100055));
#81367=CARTESIAN_POINT('Ctrl Pts',(86.0027956956387,64.8122998628938,12.2453079890425));
#81368=CARTESIAN_POINT('Ctrl Pts',(86.7719151726484,64.6862856184105,10.4728763161236));
#81369=CARTESIAN_POINT('Ctrl Pts',(88.6769817786594,64.5602713739274,10.1624953480681));
#81370=CARTESIAN_POINT('Ctrl Pts',(89.9715768758327,64.4342571294441,11.5922573347997));
#81371=CARTESIAN_POINT('Ctrl Pts',(89.4723286999136,64.3082428849609,13.4565591581593));
#81372=CARTESIAN_POINT('Ctrl Pts',(87.6354281689097,64.1822286404776,14.0477335729905));
#81373=CARTESIAN_POINT('Ctrl Pts',(86.1423722403985,64.0562143959944,12.8254625586757));
#81374=CARTESIAN_POINT('Ctrl Pts',(86.3594289049123,63.9302001515112,10.9080085372198));
#81375=CARTESIAN_POINT('Ctrl Pts',(88.0880375933813,63.804185907028,10.0504116528962));
#81376=CARTESIAN_POINT('Ctrl Pts',(89.7461262526883,63.6781716625447,11.0374559730818));
#81377=CARTESIAN_POINT('Ctrl Pts',(89.8162305881765,63.5521574180616,12.9658414468634));
#81378=CARTESIAN_POINT('Ctrl Pts',(88.2341796665934,63.4261431735783,14.0706822459788));
#81379=CARTESIAN_POINT('Ctrl Pts',(86.4478760400945,63.3001289290951,13.3408366717179));
#81380=CARTESIAN_POINT('Ctrl Pts',(86.092146389822,63.1741146846118,11.4442555333281));
#81381=CARTESIAN_POINT('Ctrl Pts',(87.4925567799329,63.0481004401286,10.1166974129684));
#81382=CARTESIAN_POINT('Ctrl Pts',(89.3674474529893,62.9220861956454,10.5731453706797));
#81383=CARTESIAN_POINT('Ctrl Pts',(90.0009141786748,62.7960719511622,12.3958578141983));
#81384=CARTESIAN_POINT('Ctrl Pts',(88.8132064665991,62.670057706679,13.9166834522003));
#81385=CARTESIAN_POINT('Ctrl Pts',(86.8913174410423,62.5440434621957,13.74375907534));
#81386=CARTESIAN_POINT('Ctrl Pts',(85.9941646487486,62.4180292177125,12.0353454126853));
#81387=CARTESIAN_POINT('Ctrl Pts',(86.9428245666493,62.2920149732293,10.3549869189101));
#81388=CARTESIAN_POINT('Ctrl Pts',(88.8690812800261,62.1660007287461,10.2405518224203));
#81389=CARTESIAN_POINT('Ctrl Pts',(90.0100198849654,62.0399864842628,11.7967714176689));
#81390=CARTESIAN_POINT('Ctrl Pts',(89.3214505449387,61.9139722397797,13.5993896756649));
#81391=CARTESIAN_POINT('Ctrl Pts',(87.4335536247469,61.7879579952963,13.998645909994));
#81392=CARTESIAN_POINT('Ctrl Pts',(86.0741370554901,61.6619437508132,12.6291398259069));
#81393=CARTESIAN_POINT('Ctrl Pts',(86.4873422447249,61.5359295063299,10.7442467802406));
#81394=CARTESIAN_POINT('Ctrl Pts',(88.2950027808736,61.4099152618468,10.0690255510391));
#81395=CARTESIAN_POINT('Ctrl Pts',(89.842743269407,61.2839010173635,11.2214402778546));
#81396=CARTESIAN_POINT('Ctrl Pts',(89.7140677862562,61.1578867728803,13.1467981516864));
#81397=CARTESIAN_POINT('Ctrl Pts',(88.0267404519492,61.031872528397,14.0830068833467));
#81398=CARTESIAN_POINT('Ctrl Pts',(86.325007417075,60.9058582839138,13.1732459255325));
#81399=CARTESIAN_POINT('Ctrl Pts',(86.1662989650349,60.7798440394306,11.2501307574836));
#81400=CARTESIAN_POINT('Ctrl Pts',(87.695865463759,60.6538297949474,10.0737011385446));
#81401=CARTESIAN_POINT('Ctrl Pts',(89.5138438696553,60.5278155504641,10.7206283663143));
#81402=CARTESIAN_POINT('Ctrl Pts',(89.9564158481913,60.401801305981,12.5988430415177));
#81403=CARTESIAN_POINT('Ctrl Pts',(88.6185384297414,60.2757870614977,13.9893984469357));
#81404=CARTESIAN_POINT('Ctrl Pts',(86.7246403374166,60.1497728170145,13.6196548354655));
#81405=CARTESIAN_POINT('Ctrl Pts',(86.0080217905846,60.0237585725313,11.8280024750253));
#81406=CARTESIAN_POINT('Ctrl Pts',(87.1245338561328,59.8977443280481,10.2541660382186));
#81407=CARTESIAN_POINT('Ctrl Pts',(89.0523419295571,59.7717300835648,10.33852452549));
#81408=CARTESIAN_POINT('Ctrl Pts',(90.0271112928982,59.6457158390816,12.0038728405961));
#81409=CARTESIAN_POINT('Ctrl Pts',(89.1567306133662,59.5197015945983,13.7260800856836));
#81410=CARTESIAN_POINT('Ctrl Pts',(87.2377744420838,59.3936873501152,13.9289779295184));
#81411=CARTESIAN_POINT('Ctrl Pts',(86.026476214272,59.2676731056318,12.4268737634783));
#81412=CARTESIAN_POINT('Ctrl Pts',(86.6314190646277,59.1416588611488,10.5944970363454));
#81413=CARTESIAN_POINT('Ctrl Pts',(88.4989577999506,59.0156446166654,10.1088434618676));
#81414=CARTESIAN_POINT('Ctrl Pts',(89.9199163496109,58.8896303721822,11.4143843928545));
#81415=CARTESIAN_POINT('Ctrl Pts',(89.5938299336816,58.763616127699,13.3162855395183));
#81416=CARTESIAN_POINT('Ctrl Pts',(87.8191336467193,58.6376018832158,14.0739222673615));
#81417=CARTESIAN_POINT('Ctrl Pts',(86.2200339209332,58.5115876387326,12.9939035687612));
#81418=CARTESIAN_POINT('Ctrl Pts',(86.2600307813403,58.3855733942493,11.0646652285107));
#81419=CARTESIAN_POINT('Ctrl Pts',(87.9025190023484,58.2595591497662,10.0518509483069));
#81420=CARTESIAN_POINT('Ctrl Pts',(89.644289300776,58.1335449052829,10.8823908629712));
#81421=CARTESIAN_POINT('Ctrl Pts',(89.8912691905753,58.0075306607997,12.7961727879484));
#81422=CARTESIAN_POINT('Ctrl Pts',(88.4174220656041,57.8815164163164,14.0416987710371));
#81423=CARTESIAN_POINT('Ctrl Pts',(86.5716164607535,57.7555021718333,13.4790603512354));
#81424=CARTESIAN_POINT('Ctrl Pts',(86.0431382318802,57.6294879273499,11.6231856022445));
#81425=CARTESIAN_POINT('Ctrl Pts',(87.3156519614396,57.5034736828668,10.1725756855481));
#81426=CARTESIAN_POINT('Ctrl Pts',(89.2245499360954,57.3774594383835,10.4548323855383));
#81427=CARTESIAN_POINT('Ctrl Pts',(90.0228040070628,57.2514451939003,12.2116336721156));
#81428=CARTESIAN_POINT('Ctrl Pts',(88.9798500738089,57.1254309494171,13.8351506616927));
#81429=CARTESIAN_POINT('Ctrl Pts',(87.0502021561888,56.9994167049339,13.8395365890262));
#81430=CARTESIAN_POINT('Ctrl Pts',(85.999878802121,56.8734024604507,12.2207774425703));
#81431=CARTESIAN_POINT('Ctrl Pts',(86.79013854362,56.7473882159674,10.4603655977736));
#81432=CARTESIAN_POINT('Ctrl Pts',(88.69773371026,56.6213739714842,10.1694343300376));
#81433=CARTESIAN_POINT('Ctrl Pts',(89.9768284863748,56.495359727001,11.6142446553228));
#81434=CARTESIAN_POINT('Ctrl Pts',(89.4567921685402,56.3693454825178,13.472502589644));
#81435=CARTESIAN_POINT('Ctrl Pts',(87.6135632813443,56.2433312380345,14.0435258744077));
#81436=CARTESIAN_POINT('Ctrl Pts',(86.1340694622722,56.1173169935513,12.8047125867561));
#81437=CARTESIAN_POINT('Ctrl Pts',(86.3723471146252,55.9913027490681,10.8898277122208));
#81438=CARTESIAN_POINT('Ctrl Pts',(88.1103239415,55.8652885045849,10.0513786251675));
#81439=CARTESIAN_POINT('Ctrl Pts',(89.757399251399,55.7392742601016,11.0567160042878));
#81440=CARTESIAN_POINT('Ctrl Pts',(89.8061656460392,55.6132600156184,12.9857525931292));
#81441=CARTESIAN_POINT('Ctrl Pts',(88.2119920004042,55.4872457711352,14.0730293333833));
#81442=CARTESIAN_POINT('Ctrl Pts',(86.4338699787695,55.3612315266519,13.3234678625798));
#81443=CARTESIAN_POINT('Ctrl Pts',(86.0991412541919,55.2352172821688,11.4230686931216));
#81444=CARTESIAN_POINT('Ctrl Pts',(87.5141503834826,55.1092030376855,10.1110818462519));
#81445=CARTESIAN_POINT('Ctrl Pts',(89.383877510955,54.9831887932023,10.588240929921));
#81446=CARTESIAN_POINT('Ctrl Pts',(89.9971437440707,54.8571745487191,12.4178487703216));
#81447=CARTESIAN_POINT('Ctrl Pts',(88.7926863091356,54.7311603042359,13.925443745693));
#81448=CARTESIAN_POINT('Ctrl Pts',(86.8728276302837,54.6051460597526,13.7312712049698));
#81449=CARTESIAN_POINT('Ctrl Pts',(85.9946271198952,54.4791318152694,12.0130383377808));
#81450=CARTESIAN_POINT('Ctrl Pts',(86.9618160576386,54.3531175707862,10.3432761148755));
#81451=CARTESIAN_POINT('Ctrl Pts',(88.889220734984,54.2271033263029,10.2501550534444));
#81452=CARTESIAN_POINT('Ctrl Pts',(90.0128756230614,54.1010890818197,11.8188997792793));
#81453=CARTESIAN_POINT('Ctrl Pts',(89.3044089885173,53.9750748373365,13.6137912384136));
#81454=CARTESIAN_POINT('Ctrl Pts',(87.4122112479467,53.8490605928533,13.9921403271053));
#81455=CARTESIAN_POINT('Ctrl Pts',(86.0680264545852,53.72304634837,12.6076810233948));
#81456=CARTESIAN_POINT('Ctrl Pts',(86.5020558566665,53.5970321038868,10.7274739070203));
#81457=CARTESIAN_POINT('Ctrl Pts',(88.3170746716699,53.4710178594036,10.0722891822916));
#81458=CARTESIAN_POINT('Ctrl Pts',(89.8519731899692,53.3450036149203,11.2417535301247));
#81459=CARTESIAN_POINT('Ctrl Pts',(89.7020084904678,53.2189893704372,13.165570286276));
#81460=CARTESIAN_POINT('Ctrl Pts',(88.0044286371382,53.0929751259539,14.0830575962183));
#81461=CARTESIAN_POINT('Ctrl Pts',(86.3128629113647,52.9669608814707,13.1545288041614));
#81462=CARTESIAN_POINT('Ctrl Pts',(86.1754364500773,52.8409466369875,11.2297757576214));
#81463=CARTESIAN_POINT('Ctrl Pts',(87.717922290672,52.7149323925042,10.0703372064778));
#81464=CARTESIAN_POINT('Ctrl Pts',(89.5286335758161,52.5889181480211,10.7373341808814));
#81465=CARTESIAN_POINT('Ctrl Pts',(89.9504028580656,52.4629039035377,12.6203294001193));
#81466=CARTESIAN_POINT('Ctrl Pts',(88.5972258465035,52.3368896590546,13.9960009805844));
#81467=CARTESIAN_POINT('Ctrl Pts',(86.7075334904992,52.2108754145714,13.6053308899133));
#81468=CARTESIAN_POINT('Ctrl Pts',(86.0107769075489,52.0848611700881,11.8058613589148));
#81469=CARTESIAN_POINT('Ctrl Pts',(87.1446294492335,51.9588469256049,10.244471359314));
#81470=CARTESIAN_POINT('Ctrl Pts',(89.0713864580408,51.8328326811216,10.3501488708561));
#81471=CARTESIAN_POINT('Ctrl Pts',(90.0276751656518,51.7068184366385,12.0261775947036));
#81472=CARTESIAN_POINT('Ctrl Pts',(89.1382977557091,51.5808041921552,13.7386518541748));
#81473=CARTESIAN_POINT('Ctrl Pts',(87.2172146848335,51.4547899476721,13.9203110552184));
#81474=CARTESIAN_POINT('Ctrl Pts',(86.0226058303358,51.3287757031887,12.4049000782672));
#81475=CARTESIAN_POINT('Ctrl Pts',(86.6477803745648,51.2027614587056,10.5793271371715));
#81476=CARTESIAN_POINT('Ctrl Pts',(88.5205766211674,51.0767472142223,10.1143604261315));
#81477=CARTESIAN_POINT('Ctrl Pts',(89.9270076260771,50.9507329697391,11.4355399850889));
#81478=CARTESIAN_POINT('Ctrl Pts',(89.5799026261666,50.8247187252559,13.33371630128));
#81479=CARTESIAN_POINT('Ctrl Pts',(87.7969362328594,50.6987044807726,14.071679139239));
#81480=CARTESIAN_POINT('Ctrl Pts',(86.2098771852938,50.5726902362894,12.9740322320388));
#81481=CARTESIAN_POINT('Ctrl Pts',(86.2712188821809,50.4466759918062,11.0453664527095));
#81482=CARTESIAN_POINT('Ctrl Pts',(87.9247951814485,50.320661747323,10.050758069298));
#81483=CARTESIAN_POINT('Ctrl Pts',(89.6573011118424,50.1946475028397,10.9005620003063));
#81484=CARTESIAN_POINT('Ctrl Pts',(89.8830386426052,50.0686332583566,12.8168618216552));
#81485=CARTESIAN_POINT('Ctrl Pts',(88.3956209050421,49.9426190138733,14.0462027928817));
#81486=CARTESIAN_POINT('Ctrl Pts',(86.5559188068883,49.8166047693901,13.4627936570351));
#81487=CARTESIAN_POINT('Ctrl Pts',(86.0484680509088,49.6905905249069,11.6019633223233));
#81488=CARTESIAN_POINT('Ctrl Pts',(87.3360078552799,49.5645762804237,10.1639590209286));
#81489=CARTESIAN_POINT('Ctrl Pts',(89.243817923361,49.4385508029241,10.4705289393977));
#81490=CARTESIAN_POINT('Ctrl Pts',(89.7590111115383,49.3545300735857,11.6428802957186));
#81491=CARTESIAN_POINT('Ctrl Pts',(89.71160828957,49.3125140924083,12.208489101734));
#81492=CARTESIAN_POINT('Ctrl Pts',(87.4571200021394,49.5646,10.4541712921126));
#81493=CARTESIAN_POINT('Ctrl Pts',(87.4645397491564,49.5646,10.4516786262364));
#81494=CARTESIAN_POINT('Ctrl Pts',(87.4719594961734,49.5646,10.4491859603602));
#81495=CARTESIAN_POINT('Ctrl Pts',(87.4793792431904,49.5646,10.446693294484));
#81496=CARTESIAN_POINT('',(87.2206343719404,64.9402624628529,11.0704469075988));
#81497=CARTESIAN_POINT('Ctrl Pts',(87.2198612186734,64.9396,11.0695788312558));
#81498=CARTESIAN_POINT('Ctrl Pts',(87.1759605752479,64.9396,11.0936148929512));
#81499=CARTESIAN_POINT('Ctrl Pts',(87.1337299408,64.9396,11.1204625428497));
#81500=CARTESIAN_POINT('Ctrl Pts',(87.0932536351023,64.9396,11.1498122632398));
#81501=CARTESIAN_POINT('Ctrl Pts',(87.06285156423,64.9396,11.1718570685649));
#81502=CARTESIAN_POINT('Ctrl Pts',(87.0334391262825,64.9396,11.1953146437608));
#81503=CARTESIAN_POINT('Ctrl Pts',(87.0050546235115,64.9396,11.2200722090875));
#81504=CARTESIAN_POINT('Ctrl Pts',(86.9950559696152,64.9396,11.2287932470784));
#81505=CARTESIAN_POINT('Ctrl Pts',(86.9851834629052,64.9396,11.2376770661783));
#81506=CARTESIAN_POINT('Ctrl Pts',(86.9754434689203,64.9396,11.2467149039896));
#81507=CARTESIAN_POINT('Ctrl Pts',(86.9364152092815,64.9396,11.2829296163624));
#81508=CARTESIAN_POINT('Ctrl Pts',(86.8995986840039,64.9396,11.3215328739256));
#81509=CARTESIAN_POINT('Ctrl Pts',(86.8650914925254,64.9396,11.3621996401194));
#81510=CARTESIAN_POINT('Ctrl Pts',(86.8404078686452,64.9396,11.3912893202161));
#81511=CARTESIAN_POINT('Ctrl Pts',(86.816905992572,64.9396,11.4214360951945));
#81512=CARTESIAN_POINT('Ctrl Pts',(86.7946267588473,64.9396,11.452536414632));
#81513=CARTESIAN_POINT('Ctrl Pts',(86.7875511713339,64.9396,11.462413461329));
#81514=CARTESIAN_POINT('Ctrl Pts',(86.7805978697889,64.9396,11.4723883600038));
#81515=CARTESIAN_POINT('Ctrl Pts',(86.7737716954075,64.9396,11.4824529995981));
#81516=CARTESIAN_POINT('Ctrl Pts',(86.7427479749459,64.9396,11.5281949551758));
#81517=CARTESIAN_POINT('Ctrl Pts',(86.7144370065936,64.9396,11.5756547454386));
#81518=CARTESIAN_POINT('Ctrl Pts',(86.6889324487018,64.9396,11.6244990730909));
#81519=CARTESIAN_POINT('Ctrl Pts',(86.6626517910026,64.9396,11.6748297261853));
#81520=CARTESIAN_POINT('Ctrl Pts',(86.6393500200212,64.9396,11.7266310638056));
#81521=CARTESIAN_POINT('Ctrl Pts',(86.619153825068,64.9396,11.7795877023749));
#81522=CARTESIAN_POINT('Ctrl Pts',(86.606400388163,64.9396,11.8130286129156));
#81523=CARTESIAN_POINT('Ctrl Pts',(86.594885871267,64.9396,11.8469311773599));
#81524=CARTESIAN_POINT('Ctrl Pts',(86.5846495052905,64.9396,11.8812237860087));
#81525=CARTESIAN_POINT('Ctrl Pts',(86.5756798766991,64.9396,11.9112727275679));
#81526=CARTESIAN_POINT('Ctrl Pts',(86.567691684042,64.9396,11.9416212794647));
#81527=CARTESIAN_POINT('Ctrl Pts',(86.5607158280894,64.9396,11.9722240399934));
#81528=CARTESIAN_POINT('Ctrl Pts',(86.5585702068065,64.9396,11.9816367822791));
#81529=CARTESIAN_POINT('Ctrl Pts',(86.5565212796045,64.9396,11.9910699427111));
#81530=CARTESIAN_POINT('Ctrl Pts',(86.5545713212498,64.9396,12.0005140259519));
#81531=CARTESIAN_POINT('Ctrl Pts',(86.5426377398758,64.9396,12.0583110222738));
#81532=CARTESIAN_POINT('Ctrl Pts',(86.5343877160295,64.9396,12.1166023576027));
#81533=CARTESIAN_POINT('Ctrl Pts',(86.529943591577,64.9396,12.175050903628));
#81534=CARTESIAN_POINT('Ctrl Pts',(86.5293917345136,64.9396,12.1823088558545));
#81535=CARTESIAN_POINT('Ctrl Pts',(86.5288986098997,64.9396,12.1895692794264));
#81536=CARTESIAN_POINT('Ctrl Pts',(86.5284644930199,64.9396,12.1968315665752));
#81537=CARTESIAN_POINT('Ctrl Pts',(86.5250925617142,64.9396,12.253240184917));
#81538=CARTESIAN_POINT('Ctrl Pts',(86.5252765631312,64.9396,12.3097596931312));
#81539=CARTESIAN_POINT('Ctrl Pts',(86.5288193552493,64.9396,12.3661604963907));
#81540=CARTESIAN_POINT('Ctrl Pts',(86.5307457881762,64.9396,12.3968290653843));
#81541=CARTESIAN_POINT('Ctrl Pts',(86.5336662011508,64.9396,12.4274628778467));
#81542=CARTESIAN_POINT('Ctrl Pts',(86.5375549590848,64.9396,12.4580266898644));
#81543=CARTESIAN_POINT('Ctrl Pts',(86.5404069972119,64.9396,12.4804423708263));
#81544=CARTESIAN_POINT('Ctrl Pts',(86.5437799813636,64.9396,12.5028204237354));
#81545=CARTESIAN_POINT('Ctrl Pts',(86.5476652186841,64.9396,12.5251471167369));
#81546=CARTESIAN_POINT('Ctrl Pts',(86.550187349591,64.9396,12.539640656725));
#81547=CARTESIAN_POINT('Ctrl Pts',(86.5529265884863,64.9396,12.5541177525244));
#81548=CARTESIAN_POINT('Ctrl Pts',(86.5558740228598,64.9396,12.5685436542528));
#81549=CARTESIAN_POINT('Ctrl Pts',(86.5678233329496,64.9396,12.6270282721379));
#81550=CARTESIAN_POINT('Ctrl Pts',(86.5832024740279,64.9396,12.6847536646261));
#81551=CARTESIAN_POINT('Ctrl Pts',(86.6017752752113,64.9396,12.7414644776671));
#81552=CARTESIAN_POINT('Ctrl Pts',(86.6207652315832,64.9396,12.7994490463292));
#81553=CARTESIAN_POINT('Ctrl Pts',(86.6430939545549,64.9396,12.8563738552118));
#81554=CARTESIAN_POINT('Ctrl Pts',(86.6685631613741,64.9396,12.911977439809));
#81555=CARTESIAN_POINT('Ctrl Pts',(86.6942849057222,64.9396,12.9681323565285));
#81556=CARTESIAN_POINT('Ctrl Pts',(86.7232099116878,64.9396,13.0229407764153));
#81557=CARTESIAN_POINT('Ctrl Pts',(86.7551867041488,64.9396,13.07612995671));
#81558=CARTESIAN_POINT('Ctrl Pts',(86.7613170644924,64.9396,13.0863270032708));
#81559=CARTESIAN_POINT('Ctrl Pts',(86.7675597386682,64.9396,13.0964644988554));
#81560=CARTESIAN_POINT('Ctrl Pts',(86.7739138682006,64.9396,13.1065404556599));
#81561=CARTESIAN_POINT('Ctrl Pts',(86.7803293490461,64.9396,13.1167136993038));
#81562=CARTESIAN_POINT('Ctrl Pts',(86.7868542233655,64.9396,13.126817407223));
#81563=CARTESIAN_POINT('Ctrl Pts',(86.7934828292441,64.9396,13.1368434139113));
#81564=CARTESIAN_POINT('Ctrl Pts',(86.82892240913,64.9396,13.1904470632271));
#81565=CARTESIAN_POINT('Ctrl Pts',(86.8673584956895,64.9396,13.2418863883912));
#81566=CARTESIAN_POINT('Ctrl Pts',(86.9085671282906,64.9396,13.2908837724665));
#81567=CARTESIAN_POINT('Ctrl Pts',(86.9498138259472,64.9396,13.3399264161883));
#81568=CARTESIAN_POINT('Ctrl Pts',(86.993838540083,64.9396,13.3865236975521));
#81569=CARTESIAN_POINT('Ctrl Pts',(87.0404676106388,64.9396,13.4303883642256));
#81570=CARTESIAN_POINT('Ctrl Pts',(87.0866458828893,64.9396,13.473828958166));
#81571=CARTESIAN_POINT('Ctrl Pts',(87.1353788326133,64.9396,13.5145905707275));
#81572=CARTESIAN_POINT('Ctrl Pts',(87.186541758314,64.9396,13.5523695888373));
#81573=CARTESIAN_POINT('Ctrl Pts',(87.1962049576915,64.9396,13.5595049545202));
#81574=CARTESIAN_POINT('Ctrl Pts',(87.2059549562448,64.9396,13.5665338266344));
#81575=CARTESIAN_POINT('Ctrl Pts',(87.2157910724421,64.9396,13.5734540116143));
#81576=CARTESIAN_POINT('Ctrl Pts',(87.2213448804068,64.9402624628529,11.0713418717467));
#81577=CARTESIAN_POINT('Ctrl Pts',(87.2248110539969,64.940041641902,11.0685900903627));
#81578=CARTESIAN_POINT('Ctrl Pts',(87.2282916117831,64.939820820951,11.065856427469));
#81579=CARTESIAN_POINT('Ctrl Pts',(87.2317863635668,64.9396,11.0631410324494));
#81580=CARTESIAN_POINT('Origin',(88.011,64.9396,12.066));
#81581=CARTESIAN_POINT('',(88.8267644998355,64.9396,13.5624301241315));
#81582=CARTESIAN_POINT('',(88.011,64.9396,10.36166));
#81583=CARTESIAN_POINT('Origin',(88.011,64.9396,12.066));
#81584=CARTESIAN_POINT('Ctrl Pts',(88.8267644998355,64.9396,13.5624301241314));
#81585=CARTESIAN_POINT('Ctrl Pts',(88.8792239118267,64.9396,13.5241330768566));
#81586=CARTESIAN_POINT('Ctrl Pts',(88.9292651527422,64.9396,13.4825784936921));
#81587=CARTESIAN_POINT('Ctrl Pts',(88.9767194214882,64.9396,13.4380905893019));
#81588=CARTESIAN_POINT('Ctrl Pts',(89.0186917952495,64.9396,13.39874190687));
#81589=CARTESIAN_POINT('Ctrl Pts',(89.0586399546992,64.9396,13.3570974140756));
#81590=CARTESIAN_POINT('Ctrl Pts',(89.0964156918618,64.9396,13.3133685018894));
#81591=CARTESIAN_POINT('Ctrl Pts',(89.1057026187326,64.9396,13.3026180244634));
#81592=CARTESIAN_POINT('Ctrl Pts',(89.1148517489142,64.9396,13.2917488694527));
#81593=CARTESIAN_POINT('Ctrl Pts',(89.1238603732724,64.9396,13.2807656128255));
#81594=CARTESIAN_POINT('Ctrl Pts',(89.1642153727066,64.9396,13.2315650581841));
#81595=CARTESIAN_POINT('Ctrl Pts',(89.2017612778272,64.9396,13.1800684361628));
#81596=CARTESIAN_POINT('Ctrl Pts',(89.2363131557526,64.9396,13.1265745930018));
#81597=CARTESIAN_POINT('Ctrl Pts',(89.2593857598928,64.9396,13.0908531694122));
#81598=CARTESIAN_POINT('Ctrl Pts',(89.2811223081476,64.9396,13.0542407522625));
#81599=CARTESIAN_POINT('Ctrl Pts',(89.3014548131317,64.9396,13.0168249099951));
#81600=CARTESIAN_POINT('Ctrl Pts',(89.3089388815175,64.9396,13.003052739647));
#81601=CARTESIAN_POINT('Ctrl Pts',(89.316234425451,64.9396,12.9891678435316));
#81602=CARTESIAN_POINT('Ctrl Pts',(89.3233253993205,64.9396,12.9751997511491));
#81603=CARTESIAN_POINT('Ctrl Pts',(89.3510266681094,64.9396,12.9206326509628));
#81604=CARTESIAN_POINT('Ctrl Pts',(89.3756487137203,64.9396,12.8647289665995));
#81605=CARTESIAN_POINT('Ctrl Pts',(89.3970346749571,64.9396,12.8077592753298));
#81606=CARTESIAN_POINT('Ctrl Pts',(89.4180965022183,64.9396,12.7516530389365));
#81607=CARTESIAN_POINT('Ctrl Pts',(89.4360197262363,64.9396,12.694511880481));
#81608=CARTESIAN_POINT('Ctrl Pts',(89.4506050688772,64.9396,12.6365941638578));
#81609=CARTESIAN_POINT('Ctrl Pts',(89.4593897614298,64.9396,12.6017105586925));
#81610=CARTESIAN_POINT('Ctrl Pts',(89.4669626385987,64.9396,12.5665453156468));
#81611=CARTESIAN_POINT('Ctrl Pts',(89.4732710163763,64.9396,12.5311570647892));
#81612=CARTESIAN_POINT('Ctrl Pts',(89.4785081647443,64.9396,12.50177811401));
#81613=CARTESIAN_POINT('Ctrl Pts',(89.4828736823687,64.9396,12.4722454765804));
#81614=CARTESIAN_POINT('Ctrl Pts',(89.486333671955,64.9396,12.4425942145647));
#81615=CARTESIAN_POINT('Ctrl Pts',(89.4878648992325,64.9396,12.4294719724081));
#81616=CARTESIAN_POINT('Ctrl Pts',(89.4892188715992,64.9396,12.4163233464084));
#81617=CARTESIAN_POINT('Ctrl Pts',(89.4903906388985,64.9396,12.4031763999801));
#81618=CARTESIAN_POINT('Ctrl Pts',(89.4954420029305,64.9396,12.3465013141025));
#81619=CARTESIAN_POINT('Ctrl Pts',(89.4971238769072,64.9396,12.2897636382346));
#81620=CARTESIAN_POINT('Ctrl Pts',(89.4952673630745,64.9396,12.2331940740218));
#81621=CARTESIAN_POINT('Ctrl Pts',(89.4950289427188,64.9396,12.2259292018803));
#81622=CARTESIAN_POINT('Ctrl Pts',(89.4947320962779,64.9396,12.2186671188516));
#81623=CARTESIAN_POINT('Ctrl Pts',(89.4943764048968,64.9396,12.2114083304016));
#81624=CARTESIAN_POINT('Ctrl Pts',(89.4915291054699,64.9396,12.1533019345514));
#81625=CARTESIAN_POINT('Ctrl Pts',(89.4849146853584,64.9396,12.0954043606453));
#81626=CARTESIAN_POINT('Ctrl Pts',(89.4746786054393,64.9396,12.0380138587617));
#81627=CARTESIAN_POINT('Ctrl Pts',(89.4658080685349,64.9396,11.988279529903));
#81628=CARTESIAN_POINT('Ctrl Pts',(89.4542166247864,64.9396,11.9389259734772));
#81629=CARTESIAN_POINT('Ctrl Pts',(89.4399760645016,64.9396,11.8901692188597));
#81630=CARTESIAN_POINT('Ctrl Pts',(89.4371398843635,64.9396,11.8804587203765));
#81631=CARTESIAN_POINT('Ctrl Pts',(89.4341978223645,64.9396,11.8707696187348));
#81632=CARTESIAN_POINT('Ctrl Pts',(89.4311528313475,64.9396,11.8611115055916));
#81633=CARTESIAN_POINT('Ctrl Pts',(89.4142502690964,64.9396,11.8074998996061));
#81634=CARTESIAN_POINT('Ctrl Pts',(89.3942260903348,64.9396,11.7549818499913));
#81635=CARTESIAN_POINT('Ctrl Pts',(89.3712370268497,64.9396,11.7038177520467));
#81636=CARTESIAN_POINT('Ctrl Pts',(89.3486106528764,64.9396,11.6534608501727));
#81637=CARTESIAN_POINT('Ctrl Pts',(89.3231113234063,64.9396,11.6044147668208));
#81638=CARTESIAN_POINT('Ctrl Pts',(89.294854050429,64.9396,11.5569631056049));
#81639=CARTESIAN_POINT('Ctrl Pts',(89.266830818113,64.9396,11.5099044624337));
#81640=CARTESIAN_POINT('Ctrl Pts',(89.2360943686532,64.9396,11.4644132591656));
#81641=CARTESIAN_POINT('Ctrl Pts',(89.2027349021024,64.9396,11.4208117620039));
#81642=CARTESIAN_POINT('Ctrl Pts',(89.1959684082983,64.9396,11.4119678178136));
#81643=CARTESIAN_POINT('Ctrl Pts',(89.1890939463749,64.9396,11.4032017907954));
#81644=CARTESIAN_POINT('Ctrl Pts',(89.182112201192,64.9396,11.3945166396301));
#81645=CARTESIAN_POINT('Ctrl Pts',(89.1761860368709,64.9396,11.3871446099138));
#81646=CARTESIAN_POINT('Ctrl Pts',(89.1701886137191,64.9396,11.3798383596809));
#81647=CARTESIAN_POINT('Ctrl Pts',(89.1641207087587,64.9396,11.3725992692063));
#81648=CARTESIAN_POINT('Ctrl Pts',(89.1302500105541,64.9396,11.3321910804916));
#81649=CARTESIAN_POINT('Ctrl Pts',(89.094184545402,64.9396,11.2938710507113));
#81650=CARTESIAN_POINT('Ctrl Pts',(89.0560329421154,64.9396,11.2578908221689));
#81651=CARTESIAN_POINT('Ctrl Pts',(89.0176057889962,64.9396,11.2216507265411));
#81652=CARTESIAN_POINT('Ctrl Pts',(88.9770615013913,64.9396,11.1877836370067));
#81653=CARTESIAN_POINT('Ctrl Pts',(88.934492924419,64.9395999999999,11.156598288569));
#81654=CARTESIAN_POINT('Ctrl Pts',(88.894260499953,64.9395999999999,11.1271243839967));
#81655=CARTESIAN_POINT('Ctrl Pts',(88.8522191812581,64.9395999999999,11.1000459568663));
#81656=CARTESIAN_POINT('Ctrl Pts',(88.8084418149977,64.9396,11.0756736932927));
#81657=CARTESIAN_POINT('Ctrl Pts',(88.8058998204431,64.9396,11.0742584834119));
#81658=CARTESIAN_POINT('Ctrl Pts',(88.8033519724573,64.9395999999999,11.0728524126409));
#81659=CARTESIAN_POINT('Ctrl Pts',(88.8007982854172,64.9396,11.0714555473222));
#81660=CARTESIAN_POINT('Origin',(88.011,64.9396,12.066));
#81661=CARTESIAN_POINT('Ctrl Pts',(89.0718796700043,65.1916319044036,10.7293673777971));
#81662=CARTESIAN_POINT('Ctrl Pts',(89.5164413428676,65.1496159224031,11.0821987329325));
#81663=CARTESIAN_POINT('Ctrl Pts',(90.0177633195797,65.0655951922414,12.2604733260601));
#81664=CARTESIAN_POINT('Ctrl Pts',(88.9345264728421,64.9395697139188,13.8604429432028));
#81665=CARTESIAN_POINT('Ctrl Pts',(87.0050126573686,64.8135554694356,13.81368644293));
#81666=CARTESIAN_POINT('Ctrl Pts',(85.9967684956509,64.6875412249523,12.1695349971148));
#81667=CARTESIAN_POINT('Ctrl Pts',(86.8316594286458,64.5615269804691,10.4295873623058));
#81668=CARTESIAN_POINT('Ctrl Pts',(88.7460330609348,64.4355127359859,10.1878084334815));
#81669=CARTESIAN_POINT('Ctrl Pts',(89.9876289924894,64.3094984915027,11.6646952830303));
#81670=CARTESIAN_POINT('Ctrl Pts',(89.4202459804645,64.1834842470194,13.50898705082));
#81671=CARTESIAN_POINT('Ctrl Pts',(87.5630991669237,64.0574700025362,14.0325885979808));
#81672=CARTESIAN_POINT('Ctrl Pts',(86.1158814976775,63.931455758053,12.7563958350616));
#81673=CARTESIAN_POINT('Ctrl Pts',(86.4030763747105,63.8054415135697,10.8483348815267));
#81674=CARTESIAN_POINT('Ctrl Pts',(88.1618492283001,63.6794272690866,10.054692161214));
#81675=CARTESIAN_POINT('Ctrl Pts',(89.7825633469161,63.5534130246033,11.1017992998498));
#81676=CARTESIAN_POINT('Ctrl Pts',(89.7819388816329,63.4273987801201,13.0313473293058));
#81677=CARTESIAN_POINT('Ctrl Pts',(88.1605464839761,63.3013845356368,14.0774060828112));
#81678=CARTESIAN_POINT('Ctrl Pts',(86.4022889175842,63.1753702911537,13.2826215191919));
#81679=CARTESIAN_POINT('Ctrl Pts',(86.1163276419185,63.0493560466704,11.3743816786031));
#81680=CARTESIAN_POINT('Ctrl Pts',(87.564375231372,62.9233418021872,10.0991127631089));
#81681=CARTESIAN_POINT('Ctrl Pts',(89.4211748960676,62.7973275577039,10.6239438494911));
#81682=CARTESIAN_POINT('Ctrl Pts',(89.9873790162293,62.6713133132208,12.4685483238613));
#81683=CARTESIAN_POINT('Ctrl Pts',(88.7447961669459,62.5452990687375,13.9447395605978));
#81684=CARTESIAN_POINT('Ctrl Pts',(86.8306412525868,62.4192848242543,13.7015037115908));
#81685=CARTESIAN_POINT('Ctrl Pts',(85.9967535828063,62.2932705797711,11.9614508157573));
#81686=CARTESIAN_POINT('Ctrl Pts',(87.0063092175991,62.1672563352878,10.3170815939551));
#81687=CARTESIAN_POINT('Ctrl Pts',(88.9353603416485,62.0412420908047,10.2733268229905));
#81688=CARTESIAN_POINT('Ctrl Pts',(90.0184345944058,61.9152278463213,11.8702309789716));
#81689=CARTESIAN_POINT('Ctrl Pts',(89.2642997401459,61.7892136018382,13.6463034270604));
#81690=CARTESIAN_POINT('Ctrl Pts',(87.3631418632286,61.6631993573549,13.976078269349));
#81691=CARTESIAN_POINT('Ctrl Pts',(86.0549053557891,61.5371851128717,12.5577447541679));
#81692=CARTESIAN_POINT('Ctrl Pts',(86.536891505879,61.4111708683884,10.6893652234866));
#81693=CARTESIAN_POINT('Ctrl Pts',(88.3679853965483,61.2851566239053,10.0808852458812));
#81694=CARTESIAN_POINT('Ctrl Pts',(89.8723653691606,61.159142379422,11.2891872021841));
#81695=CARTESIAN_POINT('Ctrl Pts',(89.6732191511257,61.0331281349388,13.2084301527842));
#81696=CARTESIAN_POINT('Ctrl Pts',(87.9528058538541,60.9071138904556,14.0821182013256));
#81697=CARTESIAN_POINT('Ctrl Pts',(86.2856519831005,60.7810996459724,13.110649884383));
#81698=CARTESIAN_POINT('Ctrl Pts',(86.197540885713,60.6550854014891,11.1831154089174));
#81699=CARTESIAN_POINT('Ctrl Pts',(87.7691120559976,60.529071157006,10.063599095359));
#81700=CARTESIAN_POINT('Ctrl Pts',(89.5620596710339,60.4030569125226,10.776685043423));
#81701=CARTESIAN_POINT('Ctrl Pts',(89.9354736380084,60.2770426680396,12.669755229354));
#81702=CARTESIAN_POINT('Ctrl Pts',(88.5476045705647,60.1510284235562,14.0102671357635));
#81703=CARTESIAN_POINT('Ctrl Pts',(86.6686336726467,60.0250141790731,13.5713809496431));
#81704=CARTESIAN_POINT('Ctrl Pts',(86.0181997583719,59.8989999345897,11.754766394281));
#81705=CARTESIAN_POINT('Ctrl Pts',(87.19158155518,59.7729856901067,10.2229936048267));
#81706=CARTESIAN_POINT('Ctrl Pts',(89.1148971398279,59.6469714456233,10.3779448276076));
#81707=CARTESIAN_POINT('Ctrl Pts',(90.0279233311991,59.5209572011402,12.0778083202041));
#81708=CARTESIAN_POINT('Ctrl Pts',(89.095056300235,59.3949429566568,13.7668648089374));
#81709=CARTESIAN_POINT('Ctrl Pts',(87.1700582614733,59.2689287121738,13.8992856167997));
#81710=CARTESIAN_POINT('Ctrl Pts',(86.0146921821982,59.1429144676904,12.3538788928424));
#81711=CARTESIAN_POINT('Ctrl Pts',(86.6863519563968,59.0169002232073,10.5450046939786));
#81712=CARTESIAN_POINT('Ctrl Pts',(88.5703328971182,58.890885978724,10.128149161942));
#81713=CARTESIAN_POINT('Ctrl Pts',(89.9424109866762,58.7648717342408,11.4848195109021));
#81714=CARTESIAN_POINT('Ctrl Pts',(89.5468569631531,58.6388574897575,13.3733876812541));
#81715=CARTESIAN_POINT('Ctrl Pts',(87.7456828474303,58.5128432452744,14.0654314114051));
#81716=CARTESIAN_POINT('Ctrl Pts',(86.1873276461012,58.3868290007911,12.9275905674894));
#81717=CARTESIAN_POINT('Ctrl Pts',(86.298001894603,58.2608147563079,11.0012199047376));
#81718=CARTESIAN_POINT('Ctrl Pts',(87.9764162469118,58.1348005118247,10.0493386193059));
#81719=CARTESIAN_POINT('Ctrl Pts',(89.686481735603,58.0087862673415,10.943110818459));
#81720=CARTESIAN_POINT('Ctrl Pts',(89.8631421949334,57.8827720228582,12.8645539744491));
#81721=CARTESIAN_POINT('Ctrl Pts',(88.3447175354873,57.756757778375,14.0551585574985));
#81722=CARTESIAN_POINT('Ctrl Pts',(86.520873761987,57.6307435338917,13.4252803077902));
#81723=CARTESIAN_POINT('Ctrl Pts',(86.0607972079062,57.5047292894086,11.5513853576991));
#81724=CARTESIAN_POINT('Ctrl Pts',(87.385551073713,57.3787150449253,10.1484670013355));
#81725=CARTESIAN_POINT('Ctrl Pts',(89.2827173441418,57.2527008004422,10.5004795890918));
#81726=CARTESIAN_POINT('Ctrl Pts',(90.0160047551388,57.1266865559588,12.2852603298174));
#81727=CARTESIAN_POINT('Ctrl Pts',(88.9143068540964,57.0006723114758,13.8693734742708));
#81728=CARTESIAN_POINT('Ctrl Pts',(86.985900285514,56.8746580669923,13.8030347537462));
#81729=CARTESIAN_POINT('Ctrl Pts',(85.9956675116008,56.7486438225092,12.1469575293814));
#81730=CARTESIAN_POINT('Ctrl Pts',(86.8498720167566,56.6226295780259,10.4167877738477));
#81731=CARTESIAN_POINT('Ctrl Pts',(88.7667437246655,56.4966153335428,10.1959811276381));
#81732=CARTESIAN_POINT('Ctrl Pts',(89.9919569061429,56.3706010890595,11.6866203796121));
#81733=CARTESIAN_POINT('Ctrl Pts',(89.4041934264733,56.2445868445763,13.5244687987039));
#81734=CARTESIAN_POINT('Ctrl Pts',(87.5413758763049,56.1185726000931,14.0275229651484));
#81735=CARTESIAN_POINT('Ctrl Pts',(86.1083594859353,55.9925583556099,12.7353864613211));
#81736=CARTESIAN_POINT('Ctrl Pts',(86.4166444009374,55.8665441111266,10.8306258121125));
#81737=CARTESIAN_POINT('Ctrl Pts',(88.1840875044425,55.7405298666434,10.0564826758231));
#81738=CARTESIAN_POINT('Ctrl Pts',(89.7931204956846,55.6145156221602,11.1214547659207));
#81739=CARTESIAN_POINT('Ctrl Pts',(89.771152400528,55.488501377677,13.050876990937));
#81740=CARTESIAN_POINT('Ctrl Pts',(88.1382884740062,55.3624871331937,14.0789373573826));
#81741=CARTESIAN_POINT('Ctrl Pts',(86.3889298211781,55.2364728887105,13.2647524745907));
#81742=CARTESIAN_POINT('Ctrl Pts',(86.1240938088108,55.1104586442273,11.3534663614863));
#81743=CARTESIAN_POINT('Ctrl Pts',(87.5861590105954,54.9844443997441,10.0942927970709));
#81744=CARTESIAN_POINT('Ctrl Pts',(89.4370397368875,54.8584301552608,10.6396305425386));
#81745=CARTESIAN_POINT('Ctrl Pts',(89.9828053681324,54.7324159107776,12.4903851441387));
#81746=CARTESIAN_POINT('Ctrl Pts',(88.723969848457,54.6064016662943,13.9527414119461));
#81747=CARTESIAN_POINT('Ctrl Pts',(86.8126225596736,54.4803874218113,13.6883472719729));
#81748=CARTESIAN_POINT('Ctrl Pts',(85.9980332689162,54.3543731773279,11.9391768952013));
#81749=CARTESIAN_POINT('Ctrl Pts',(87.0257161102803,54.2283589328448,10.3060753376864));
#81750=CARTESIAN_POINT('Ctrl Pts',(88.9551332049876,54.1023446883614,10.2836611849593));
#81751=CARTESIAN_POINT('Ctrl Pts',(90.0204772548203,53.9763304438783,11.8924479250456));
#81752=CARTESIAN_POINT('Ctrl Pts',(89.2467427498404,53.850316199395,13.6600699534772));
#81753=CARTESIAN_POINT('Ctrl Pts',(87.3420534231299,53.7243019549118,13.9687952169514));
#81754=CARTESIAN_POINT('Ctrl Pts',(86.0495856584636,53.5982877104286,12.5360775905908));
#81755=CARTESIAN_POINT('Ctrl Pts',(86.5522091514694,53.4722734659454,10.6731437904033));
#81756=CARTESIAN_POINT('Ctrl Pts',(88.3899216379232,53.3462592214621,10.0849554390021));
#81757=CARTESIAN_POINT('Ctrl Pts',(89.8808441039386,53.2202449769789,11.3098239706732));
#81758=CARTESIAN_POINT('Ctrl Pts',(89.6604806202747,53.0942307324956,13.2267466751012));
#81759=CARTESIAN_POINT('Ctrl Pts',(87.9305083923,52.9682164880125,14.0813511508713));
#81760=CARTESIAN_POINT('Ctrl Pts',(86.274202282863,52.8422022435292,13.0915012677515));
#81761=CARTESIAN_POINT('Ctrl Pts',(86.2074177406864,52.716187999046,11.1631100871809));
#81762=CARTESIAN_POINT('Ctrl Pts',(87.7912761442532,52.5901737545628,10.0610459889415));
#81763=CARTESIAN_POINT('Ctrl Pts',(89.5762263638141,52.4641595100796,10.7939207606738));
#81764=CARTESIAN_POINT('Ctrl Pts',(89.9286775437447,52.3381452655963,12.6910056011268));
#81765=CARTESIAN_POINT('Ctrl Pts',(88.5260654901182,52.2121310211131,14.016083765398));
#81766=CARTESIAN_POINT('Ctrl Pts',(86.6520642285717,52.0861167766299,13.5564404509969));
#81767=CARTESIAN_POINT('Ctrl Pts',(86.0217643411852,51.9601025321467,11.7327423332934));
#81768=CARTESIAN_POINT('Ctrl Pts',(87.2120178612602,51.8340882876634,10.2140424873741));
#81769=CARTESIAN_POINT('Ctrl Pts',(89.1335017885094,51.7080740431803,10.3902586769542));
#81770=CARTESIAN_POINT('Ctrl Pts',(90.0276693475674,51.5820597986969,12.1001175941515));
#81771=CARTESIAN_POINT('Ctrl Pts',(89.0761760395382,51.4560455542138,13.7787517583213));
#81772=CARTESIAN_POINT('Ctrl Pts',(87.1498311674703,51.3300313097305,13.8898717692197));
#81773=CARTESIAN_POINT('Ctrl Pts',(86.0116297763121,51.2040170652473,12.3317788383906));
#81774=CARTESIAN_POINT('Ctrl Pts',(86.7032576904153,51.0780028207641,10.530446430839));
#81775=CARTESIAN_POINT('Ctrl Pts',(88.5917331402567,50.9519885762809,10.1344524998545));
#81776=CARTESIAN_POINT('Ctrl Pts',(89.9487231068468,50.8259743317976,11.5062235195118));
#81777=CARTESIAN_POINT('Ctrl Pts',(89.5322982436163,50.6999600873144,13.3902875533465));
#81778=CARTESIAN_POINT('Ctrl Pts',(87.723589165804,50.5739458428312,14.0623919641885));
#81779=CARTESIAN_POINT('Ctrl Pts',(86.1778957835015,50.447931598348,12.9073302450681));
#81780=CARTESIAN_POINT('Ctrl Pts',(86.3099107531474,50.3219173538647,10.9824075787222));
#81781=CARTESIAN_POINT('Ctrl Pts',(87.998673098572,50.1959031093816,10.048938138889));
#81782=CARTESIAN_POINT('Ctrl Pts',(89.6989045810523,50.0698888648982,10.9619953922184));
#81783=CARTESIAN_POINT('Ctrl Pts',(89.8539859089795,49.9438746204151,12.8844261577189));
#81784=CARTESIAN_POINT('Ctrl Pts',(88.3231209088254,49.8178603759318,14.0598673879485));
#81785=CARTESIAN_POINT('Ctrl Pts',(86.5050006083808,49.6918461314486,13.4063554329357));
#81786=CARTESIAN_POINT('Ctrl Pts',(86.215092379416,49.6078366351265,12.1593708946452));
#81787=CARTESIAN_POINT('Ctrl Pts',(86.3659223664004,49.5658318869654,11.6123789721938));
#81788=CARTESIAN_POINT('Ctrl Pts',(88.9809519941789,65.1071878779614,10.8439297557986));
#81789=CARTESIAN_POINT('Ctrl Pts',(89.3874104204466,65.0651718959608,11.166520042142));
#81790=CARTESIAN_POINT('Ctrl Pts',(89.8457642420782,64.9811511657991,12.2438050760703));
#81791=CARTESIAN_POINT('Ctrl Pts',(88.8553712980253,64.8551256874765,13.7066417809788));
#81792=CARTESIAN_POINT('Ctrl Pts',(87.0912355284081,64.7291114429933,13.6638927662105));
#81793=CARTESIAN_POINT('Ctrl Pts',(86.1694076690113,64.60309719851,12.1606610438093));
#81794=CARTESIAN_POINT('Ctrl Pts',(86.9327403525165,64.4770829540269,10.5698437948154));
#81795=CARTESIAN_POINT('Ctrl Pts',(88.6830335994734,64.3510687095436,10.3487876648937));
#81796=CARTESIAN_POINT('Ctrl Pts',(89.8182127190535,64.2250544650604,11.6990909890124));
#81797=CARTESIAN_POINT('Ctrl Pts',(89.2994599334764,64.0990402205772,13.3853090668914));
#81798=CARTESIAN_POINT('Ctrl Pts',(87.6014886119317,63.9730259760939,13.8640328837232));
#81799=CARTESIAN_POINT('Ctrl Pts',(86.2783115316406,63.8470117316107,12.6972222167366));
#81800=CARTESIAN_POINT('Ctrl Pts',(86.5408910225787,63.7209974871275,10.952700590746));
#81801=CARTESIAN_POINT('Ctrl Pts',(88.1489199865423,63.5949832426443,10.2270807480829));
#81802=CARTESIAN_POINT('Ctrl Pts',(89.6307231879736,63.468968998161,11.1844406503936));
#81803=CARTESIAN_POINT('Ctrl Pts',(89.6301522454211,63.3429547536778,12.9486077015236));
#81804=CARTESIAN_POINT('Ctrl Pts',(88.1477289000405,63.2169405091946,13.9050090754766));
#81805=CARTESIAN_POINT('Ctrl Pts',(86.5401710581646,63.0909262647113,13.1783452565515));
#81806=CARTESIAN_POINT('Ctrl Pts',(86.2787194369936,62.9649120202282,11.4336600758624));
#81807=CARTESIAN_POINT('Ctrl Pts',(87.602655305282,62.8388977757449,10.2676940736172));
#81808=CARTESIAN_POINT('Ctrl Pts',(89.300309232004,62.7128835312617,10.7475420462355));
#81809=CARTESIAN_POINT('Ctrl Pts',(89.8179841681831,62.5868692867784,12.4340460287084));
#81810=CARTESIAN_POINT('Ctrl Pts',(88.6819027192945,62.4608550422953,13.7837133607787));
#81811=CARTESIAN_POINT('Ctrl Pts',(86.9318094440195,62.334840797812,13.5613251828629));
#81812=CARTESIAN_POINT('Ctrl Pts',(86.1693940343423,62.2088265533288,11.9704116947348));
#81813=CARTESIAN_POINT('Ctrl Pts',(87.0924209608531,62.0828123088455,10.4669808618608));
#81814=CARTESIAN_POINT('Ctrl Pts',(88.8561336961885,61.9567980643624,10.4269762990892));
#81815=CARTESIAN_POINT('Ctrl Pts',(89.846377982142,61.8307838198791,11.8870102825854));
#81816=CARTESIAN_POINT('Ctrl Pts',(89.1568797982749,61.7047695753959,13.5108560980332));
#81817=CARTESIAN_POINT('Ctrl Pts',(87.4186695882918,61.5787553309127,13.8123660382761));
#81818=CARTESIAN_POINT('Ctrl Pts',(86.2225616364411,61.4527410864295,12.5155974599365));
#81819=CARTESIAN_POINT('Ctrl Pts',(86.6632368993054,61.3267268419462,10.8073561740419));
#81820=CARTESIAN_POINT('Ctrl Pts',(88.3373882861223,61.2007125974631,10.2510288313811));
#81821=CARTESIAN_POINT('Ctrl Pts',(89.7128283060376,61.0746983529797,11.355767592264));
#81822=CARTESIAN_POINT('Ctrl Pts',(89.5307508501508,60.9486841084966,13.1105128097316));
#81823=CARTESIAN_POINT('Ctrl Pts',(87.957793656529,60.8226698640132,13.9093173197375));
#81824=CARTESIAN_POINT('Ctrl Pts',(86.4335310400774,60.6966556195302,13.0211132585772));
#81825=CARTESIAN_POINT('Ctrl Pts',(86.3529719182124,60.5706413750468,11.258787180334));
#81826=CARTESIAN_POINT('Ctrl Pts',(87.7898441985583,60.4446271305637,10.2352242715947));
#81827=CARTESIAN_POINT('Ctrl Pts',(89.4291188154956,60.3186128860804,10.8871918386073));
#81828=CARTESIAN_POINT('Ctrl Pts',(89.7705275842394,60.1925986415973,12.6180075511538));
#81829=CARTESIAN_POINT('Ctrl Pts',(88.5016123550305,60.0665843971139,13.843624587285));
#81830=CARTESIAN_POINT('Ctrl Pts',(86.7836874847833,59.9405701526308,13.4423552035072));
#81831=CARTESIAN_POINT('Ctrl Pts',(86.189002064683,59.8145559081475,11.781442132545));
#81832=CARTESIAN_POINT('Ctrl Pts',(87.2618136623853,59.6885416636643,10.380957125839));
#81833=CARTESIAN_POINT('Ctrl Pts',(89.0202824496677,59.5625274191811,10.5226275261552));
#81834=CARTESIAN_POINT('Ctrl Pts',(89.8550534421729,59.4365131746979,12.0767962326489));
#81835=CARTESIAN_POINT('Ctrl Pts',(89.0021421624386,59.3104989302146,13.6210842003138));
#81836=CARTESIAN_POINT('Ctrl Pts',(87.2421351236761,59.1844846857314,13.7421552607633));
#81837=CARTESIAN_POINT('Ctrl Pts',(86.1857951218026,59.0584704412482,12.3292048799591));
#81838=CARTESIAN_POINT('Ctrl Pts',(86.7998871397895,58.932456196765,10.6753687418796));
#81839=CARTESIAN_POINT('Ctrl Pts',(88.5223926435856,58.8064419522817,10.2942417714836));
#81840=CARTESIAN_POINT('Ctrl Pts',(89.7768703348499,58.6804277077986,11.534632314939));
#81841=CARTESIAN_POINT('Ctrl Pts',(89.4152191271117,58.5544134633152,13.2613318783009));
#81842=CARTESIAN_POINT('Ctrl Pts',(87.7684231003749,58.4283992188321,13.8940607495369));
#81843=CARTESIAN_POINT('Ctrl Pts',(86.3436340522804,58.3023849743488,12.853743900398));
#81844=CARTESIAN_POINT('Ctrl Pts',(86.4448224443983,58.1763707298656,11.0924818848327));
#81845=CARTESIAN_POINT('Ctrl Pts',(87.9793804099347,58.0503564853824,10.2221860566334));
#81846=CARTESIAN_POINT('Ctrl Pts',(89.5428767025218,57.9243422408992,11.0393533107734));
#81847=CARTESIAN_POINT('Ctrl Pts',(89.7043956472854,57.798327996416,12.796110154692));
#81848=CARTESIAN_POINT('Ctrl Pts',(88.3161147063994,57.6723137519327,13.8846683788333));
#81849=CARTESIAN_POINT('Ctrl Pts',(86.6485920314004,57.5462995074495,13.3087768035031));
#81850=CARTESIAN_POINT('Ctrl Pts',(86.2279484996942,57.4202852629663,11.595492823129));
#81851=CARTESIAN_POINT('Ctrl Pts',(87.4391581121195,57.294271018483,10.3128181750045));
#81852=CARTESIAN_POINT('Ctrl Pts',(89.1737188349997,57.1682567739999,10.6346598702733));
#81853=CARTESIAN_POINT('Ctrl Pts',(89.844156403664,57.0422425295165,12.2664675932285));
#81854=CARTESIAN_POINT('Ctrl Pts',(88.8368846966901,56.9162282850334,13.7148068789286));
#81855=CARTESIAN_POINT('Ctrl Pts',(87.0737612721676,56.7902140405501,13.6541540300867));
#81856=CARTESIAN_POINT('Ctrl Pts',(86.1684010499714,56.664199796067,12.1400186840105));
#81857=CARTESIAN_POINT('Ctrl Pts',(86.9493919452058,56.5381855515836,10.5581412552148));
#81858=CARTESIAN_POINT('Ctrl Pts',(88.7019691584764,56.4121713071005,10.3562598799046));
#81859=CARTESIAN_POINT('Ctrl Pts',(89.8221696885362,56.2861570626172,11.7191368921938));
#81860=CARTESIAN_POINT('Ctrl Pts',(89.2847832390352,56.1601428181341,13.3994638788441));
#81861=CARTESIAN_POINT('Ctrl Pts',(87.5816272179853,56.0341285736508,13.8594014247497));
#81862=CARTESIAN_POINT('Ctrl Pts',(86.271434229251,55.9081143291676,12.6780135500685));
#81863=CARTESIAN_POINT('Ctrl Pts',(86.5532961373791,55.7821000846843,10.936509360318));
#81864=CARTESIAN_POINT('Ctrl Pts',(88.1692522267591,55.6560858402012,10.2287177982261));
#81865=CARTESIAN_POINT('Ctrl Pts',(89.6403754867124,55.5300715957179,11.2024114524093));
#81866=CARTESIAN_POINT('Ctrl Pts',(89.6202902703509,55.4040573512348,12.9664634817599));
#81867=CARTESIAN_POINT('Ctrl Pts',(88.1273786173767,55.2780431067514,13.9064091049674));
#81868=CARTESIAN_POINT('Ctrl Pts',(86.5279569658731,55.1520288622683,13.1620077623615));
#81869=CARTESIAN_POINT('Ctrl Pts',(86.2858199680693,55.026014617785,11.4145374042533));
#81870=CARTESIAN_POINT('Ctrl Pts',(87.6225720033731,54.9000003733019,10.2632872254112));
#81871=CARTESIAN_POINT('Ctrl Pts',(89.3148143021131,54.7739861288185,10.7618842375638));
#81872=CARTESIAN_POINT('Ctrl Pts',(89.813802526082,54.6479718843354,12.4540112217209));
#81873=CARTESIAN_POINT('Ctrl Pts',(88.6628614182677,54.5219576398521,13.7910293758668));
#81874=CARTESIAN_POINT('Ctrl Pts',(86.9153351278294,54.3959433953689,13.5492963777076));
#81875=CARTESIAN_POINT('Ctrl Pts',(86.1705640389423,54.2699291508856,11.9500468651766));
#81876=CARTESIAN_POINT('Ctrl Pts',(87.110164494629,54.1439149064024,10.4569179484899));
#81877=CARTESIAN_POINT('Ctrl Pts',(88.8742118333879,54.0179006619192,10.4364249060175));
#81878=CARTESIAN_POINT('Ctrl Pts',(89.8482455667497,53.891886417436,11.9073230209273));
#81879=CARTESIAN_POINT('Ctrl Pts',(89.1408276123014,53.7658721729527,13.5234426996323));
#81880=CARTESIAN_POINT('Ctrl Pts',(87.3993886320191,53.6398579284696,13.8057072140979));
#81881=CARTESIAN_POINT('Ctrl Pts',(86.2176978887654,53.5138436839863,12.4957873823999));
#81882=CARTESIAN_POINT('Ctrl Pts',(86.6772416741224,53.3878294395032,10.7925250750846));
#81883=CARTESIAN_POINT('Ctrl Pts',(88.3574443788803,53.2618151950198,10.25475016948));
#81884=CARTESIAN_POINT('Ctrl Pts',(89.7205803310206,53.1358009505367,11.3746355895643));
#81885=CARTESIAN_POINT('Ctrl Pts',(89.5191041349285,53.0097867060534,13.1272594284577));
#81886=CARTESIAN_POINT('Ctrl Pts',(87.9374073036642,52.8837724615702,13.9086160129458));
#81887=CARTESIAN_POINT('Ctrl Pts',(86.4230626901862,52.7577582170869,13.0036058640888));
#81888=CARTESIAN_POINT('Ctrl Pts',(86.3620022309317,52.6317439726038,11.2404965086763));
#81889=CARTESIAN_POINT('Ctrl Pts',(87.8101086095093,52.5057297281205,10.2328899911565));
#81890=CARTESIAN_POINT('Ctrl Pts',(89.4420712853203,52.3797154836374,10.9029502877427));
#81891=CARTESIAN_POINT('Ctrl Pts',(89.7643139811604,52.253701239154,12.6374365599856));
#81892=CARTESIAN_POINT('Ctrl Pts',(88.4819193826581,52.1276869946709,13.848942675352));
#81893=CARTESIAN_POINT('Ctrl Pts',(86.7685382027512,52.0016727501876,13.4286952504836));
#81894=CARTESIAN_POINT('Ctrl Pts',(86.1922611281809,51.8756585057044,11.7613057471672));
#81895=CARTESIAN_POINT('Ctrl Pts',(87.2804983788489,51.7496442612212,10.3727732059575));
#81896=CARTESIAN_POINT('Ctrl Pts',(89.0372924995348,51.6236300167379,10.5338859591966));
#81897=CARTESIAN_POINT('Ctrl Pts',(89.8548212274014,51.4976157722547,12.0971933854702));
#81898=CARTESIAN_POINT('Ctrl Pts',(88.9848801231789,51.3716015277715,13.6319523228593));
#81899=CARTESIAN_POINT('Ctrl Pts',(87.2236416877859,51.2455872832883,13.7335482712137));
#81900=CARTESIAN_POINT('Ctrl Pts',(86.1829951937994,51.1195730388051,12.3089990144938));
#81901=CARTESIAN_POINT('Ctrl Pts',(86.8153438884555,50.9935587943218,10.6620582630729));
#81902=CARTESIAN_POINT('Ctrl Pts',(88.5419586783537,50.8675445498387,10.3000048522091));
#81903=CARTESIAN_POINT('Ctrl Pts',(89.7826414451086,50.7415303053553,11.5542017924411));
#81904=CARTESIAN_POINT('Ctrl Pts',(89.4019082310255,50.6155160608722,13.2767832674649));
#81905=CARTESIAN_POINT('Ctrl Pts',(87.7482230615222,50.4895018163889,13.8912818124225));
#81906=CARTESIAN_POINT('Ctrl Pts',(86.3350105917728,50.3634875719057,12.835220084087));
#81907=CARTESIAN_POINT('Ctrl Pts',(86.4557105982768,50.2374733274225,11.0752819575934));
#81908=CARTESIAN_POINT('Ctrl Pts',(87.9997296335672,50.1114590829393,10.221819901272));
#81909=CARTESIAN_POINT('Ctrl Pts',(89.5542347896429,49.985444838456,11.0566192934245));
#81910=CARTESIAN_POINT('Ctrl Pts',(89.6960241438328,49.8594305939729,12.814279099141));
#81911=CARTESIAN_POINT('Ctrl Pts',(88.2963691200802,49.7334163494895,13.8889736168488));
#81912=CARTESIAN_POINT('Ctrl Pts',(86.6340793609915,49.6074021050064,13.2914739739516));
#81913=CARTESIAN_POINT('Ctrl Pts',(86.3690190786956,49.5233926086842,12.15136810349));
#81914=CARTESIAN_POINT('Ctrl Pts',(86.5069214730896,49.4813878605231,11.6512586933631));
#81915=CARTESIAN_POINT('Ctrl Pts',(88.8900243183537,65.022743851519,10.9584921338002));
#81916=CARTESIAN_POINT('Ctrl Pts',(89.2583794980258,64.9807278695185,11.2508413513514));
#81917=CARTESIAN_POINT('Ctrl Pts',(89.6737651645768,64.8967071393568,12.2271368260806));
#81918=CARTESIAN_POINT('Ctrl Pts',(88.7762161232086,64.7706816610343,13.5528406187548));
#81919=CARTESIAN_POINT('Ctrl Pts',(87.1774583994475,64.644667416551,13.5140990894909));
#81920=CARTESIAN_POINT('Ctrl Pts',(86.3420468423718,64.5186531720677,12.151787090504));
#81921=CARTESIAN_POINT('Ctrl Pts',(87.0338212763872,64.3926389275846,10.7101002273247));
#81922=CARTESIAN_POINT('Ctrl Pts',(88.6200341380121,64.2666246831013,10.509766896306));
#81923=CARTESIAN_POINT('Ctrl Pts',(89.6487964456177,64.1406104386181,11.7334866949944));
#81924=CARTESIAN_POINT('Ctrl Pts',(89.1786738864885,64.0145961941349,13.2616310829627));
#81925=CARTESIAN_POINT('Ctrl Pts',(87.6398780569399,63.8885819496517,13.6954771694657));
#81926=CARTESIAN_POINT('Ctrl Pts',(86.4407415656038,63.7625677051684,12.6380485984115));
#81927=CARTESIAN_POINT('Ctrl Pts',(86.6787056704468,63.6365534606853,11.0570662999652));
#81928=CARTESIAN_POINT('Ctrl Pts',(88.1359907447846,63.5105392162019,10.3994693349518));
#81929=CARTESIAN_POINT('Ctrl Pts',(89.478883029031,63.3845249717188,11.2670820009376));
#81930=CARTESIAN_POINT('Ctrl Pts',(89.4783656092092,63.2585107272356,12.8658680737414));
#81931=CARTESIAN_POINT('Ctrl Pts',(88.1349113161049,63.1324964827523,13.732612068142));
#81932=CARTESIAN_POINT('Ctrl Pts',(86.678053198745,63.0064822382691,13.0740689939112));
#81933=CARTESIAN_POINT('Ctrl Pts',(86.4411112320687,62.8804679937859,11.4929384731217));
#81934=CARTESIAN_POINT('Ctrl Pts',(87.640935379192,62.7544537493026,10.4362753841254));
#81935=CARTESIAN_POINT('Ctrl Pts',(89.1794435679404,62.6284395048194,10.8711402429799));
#81936=CARTESIAN_POINT('Ctrl Pts',(89.6485893201372,62.5024252603362,12.3995437335558));
#81937=CARTESIAN_POINT('Ctrl Pts',(88.6190092716429,62.3764110158529,13.6226871609596));
#81938=CARTESIAN_POINT('Ctrl Pts',(87.0329776354527,62.2503967713698,13.4211466541349));
#81939=CARTESIAN_POINT('Ctrl Pts',(86.3420344858781,62.1243825268866,11.9793725737123));
#81940=CARTESIAN_POINT('Ctrl Pts',(87.1785327041071,61.9983682824033,10.6168801297665));
#81941=CARTESIAN_POINT('Ctrl Pts',(88.7769070507285,61.8723540379201,10.5806257751877));
#81942=CARTESIAN_POINT('Ctrl Pts',(89.6743213698781,61.7463397934368,11.9037895861992));
#81943=CARTESIAN_POINT('Ctrl Pts',(89.0494598564039,61.6203255489537,13.3754087690061));
#81944=CARTESIAN_POINT('Ctrl Pts',(87.474197313355,61.4943113044703,13.6486538072033));
#81945=CARTESIAN_POINT('Ctrl Pts',(86.3902179170933,61.3682970599872,12.4734501657051));
#81946=CARTESIAN_POINT('Ctrl Pts',(86.7895822927318,61.242282815504,10.9253471245972));
#81947=CARTESIAN_POINT('Ctrl Pts',(88.3067911756965,61.1162685710207,10.421172416881));
#81948=CARTESIAN_POINT('Ctrl Pts',(89.5532912429143,60.9902543265374,11.4223479823439));
#81949=CARTESIAN_POINT('Ctrl Pts',(89.3882825491763,60.8642400820543,13.012595466679));
#81950=CARTESIAN_POINT('Ctrl Pts',(87.9627814592036,60.738225837571,13.7365164381495));
#81951=CARTESIAN_POINT('Ctrl Pts',(86.5814100970547,60.6122115930879,12.9315766327714));
#81952=CARTESIAN_POINT('Ctrl Pts',(86.5084029507116,60.4861973486045,11.3344589517505));
#81953=CARTESIAN_POINT('Ctrl Pts',(87.810576341119,60.3601831041214,10.4068494478305));
#81954=CARTESIAN_POINT('Ctrl Pts',(89.2961779599576,60.2341688596381,10.9976986337916));
#81955=CARTESIAN_POINT('Ctrl Pts',(89.6055815304699,60.108154615155,12.5662598729536));
#81956=CARTESIAN_POINT('Ctrl Pts',(88.4556201394965,59.9821403706717,13.6769820388066));
#81957=CARTESIAN_POINT('Ctrl Pts',(86.8987412969199,59.8561261261885,13.3133294573713));
#81958=CARTESIAN_POINT('Ctrl Pts',(86.3598043709943,59.7301118817052,11.8081178708092));
#81959=CARTESIAN_POINT('Ctrl Pts',(87.3320457695907,59.6040976372221,10.5389206468513));
#81960=CARTESIAN_POINT('Ctrl Pts',(88.9256677595075,59.4780833927388,10.6673102247027));
#81961=CARTESIAN_POINT('Ctrl Pts',(89.6821835531468,59.3520691482556,12.0757841450938));
#81962=CARTESIAN_POINT('Ctrl Pts',(88.9092280246422,59.2260549037723,13.4753035916902));
#81963=CARTESIAN_POINT('Ctrl Pts',(87.314211985879,59.1000406592892,13.585024904727));
#81964=CARTESIAN_POINT('Ctrl Pts',(86.3568980614073,58.9740264148058,12.3045308670758));
#81965=CARTESIAN_POINT('Ctrl Pts',(86.9134223231819,58.8480121703227,10.8057327897807));
#81966=CARTESIAN_POINT('Ctrl Pts',(88.4744523900531,58.7219979258394,10.4603343810253));
#81967=CARTESIAN_POINT('Ctrl Pts',(89.6113296830234,58.5959836813563,11.584445118976));
#81968=CARTESIAN_POINT('Ctrl Pts',(89.2835812910705,58.469969436873,13.1492760753477));
#81969=CARTESIAN_POINT('Ctrl Pts',(87.7911633533195,58.3439551923898,13.7226900876687));
#81970=CARTESIAN_POINT('Ctrl Pts',(86.4999404584594,58.2179409479065,12.7798972333066));
#81971=CARTESIAN_POINT('Ctrl Pts',(86.5916429941938,58.0919267034233,11.1837438649278));
#81972=CARTESIAN_POINT('Ctrl Pts',(87.9823445729578,57.9659124589401,10.3950334939609));
#81973=CARTESIAN_POINT('Ctrl Pts',(89.3992716694407,57.8398982144569,11.1355958030878));
#81974=CARTESIAN_POINT('Ctrl Pts',(89.5456490996371,57.7138839699737,12.727666334935));
#81975=CARTESIAN_POINT('Ctrl Pts',(88.2875118773115,57.5878697254904,13.7141782001681));
#81976=CARTESIAN_POINT('Ctrl Pts',(86.7763103008137,57.4618554810072,13.192273299216));
#81977=CARTESIAN_POINT('Ctrl Pts',(86.3950997914827,57.335841236524,11.639600288559));
#81978=CARTESIAN_POINT('Ctrl Pts',(87.492765150526,57.2098269920407,10.4771693486735));
#81979=CARTESIAN_POINT('Ctrl Pts',(89.0647203258579,57.0838127475576,10.7688401514549));
#81980=CARTESIAN_POINT('Ctrl Pts',(89.6723080521893,56.9577985030743,12.2476748566395));
#81981=CARTESIAN_POINT('Ctrl Pts',(88.759462539284,56.8317842585912,13.5602402835864));
#81982=CARTESIAN_POINT('Ctrl Pts',(87.1616222588214,56.7057700141078,13.5052733064272));
#81983=CARTESIAN_POINT('Ctrl Pts',(86.3411345883419,56.5797557696247,12.1330798386397));
#81984=CARTESIAN_POINT('Ctrl Pts',(87.0489118736551,56.4537415251414,10.6994947365818));
#81985=CARTESIAN_POINT('Ctrl Pts',(88.6371945922872,56.3277272806582,10.5165386321713));
#81986=CARTESIAN_POINT('Ctrl Pts',(89.6523824709294,56.2017130361749,11.7516534047755));
#81987=CARTESIAN_POINT('Ctrl Pts',(89.1653730515974,56.0756987916918,13.2744589589843));
#81988=CARTESIAN_POINT('Ctrl Pts',(87.6218785596657,55.9496845472086,13.6912798843509));
#81989=CARTESIAN_POINT('Ctrl Pts',(86.4345089725667,55.8236703027253,12.620640638816));
#81990=CARTESIAN_POINT('Ctrl Pts',(86.6899478738208,55.6976560582421,11.0423929085234));
#81991=CARTESIAN_POINT('Ctrl Pts',(88.1544169490754,55.5716418137588,10.4009529206292));
#81992=CARTESIAN_POINT('Ctrl Pts',(89.4876304777402,55.4456275692756,11.2833681388979));
#81993=CARTESIAN_POINT('Ctrl Pts',(89.469428140174,55.3196133247924,12.8820499725828));
#81994=CARTESIAN_POINT('Ctrl Pts',(88.1164687607474,55.1935990803092,13.7338808525521));
#81995=CARTESIAN_POINT('Ctrl Pts',(86.6669841105681,55.067584835826,13.0592630501324));
#81996=CARTESIAN_POINT('Ctrl Pts',(86.4475461273278,54.9415705913427,11.4756084470202));
#81997=CARTESIAN_POINT('Ctrl Pts',(87.6589849961508,54.8155563468595,10.4322816537516));
#81998=CARTESIAN_POINT('Ctrl Pts',(89.1925888673385,54.6895421023763,10.8841379325889));
#81999=CARTESIAN_POINT('Ctrl Pts',(89.6447996840317,54.563527857893,12.4176372993032));
#82000=CARTESIAN_POINT('Ctrl Pts',(88.6017529880784,54.4375136134099,13.6293173397875));
#82001=CARTESIAN_POINT('Ctrl Pts',(87.0180476959851,54.3114993689266,13.4102454834423));
#82002=CARTESIAN_POINT('Ctrl Pts',(86.3430948089686,54.1854851244434,11.9609168351518));
#82003=CARTESIAN_POINT('Ctrl Pts',(87.1946128789778,54.0594708799602,10.6077605592933));
#82004=CARTESIAN_POINT('Ctrl Pts',(88.7932904617882,53.9334566354769,10.5891886270757));
#82005=CARTESIAN_POINT('Ctrl Pts',(89.6760138786792,53.8074423909938,11.922198116809));
#82006=CARTESIAN_POINT('Ctrl Pts',(89.0349124747621,53.6814281465105,13.3868154457874));
#82007=CARTESIAN_POINT('Ctrl Pts',(87.4567238409084,53.5554139020273,13.6426192112445));
#82008=CARTESIAN_POINT('Ctrl Pts',(86.385810119067,53.429399657544,12.4554971742089));
#82009=CARTESIAN_POINT('Ctrl Pts',(86.8022741967758,53.3033854130608,10.911906359766));
#82010=CARTESIAN_POINT('Ctrl Pts',(88.324967119837,53.1773711685776,10.4245448999579));
#82011=CARTESIAN_POINT('Ctrl Pts',(89.5603165581028,53.0513569240944,11.4394472084552));
#82012=CARTESIAN_POINT('Ctrl Pts',(89.3777276495823,52.9253426796111,13.0277721818141));
#82013=CARTESIAN_POINT('Ctrl Pts',(87.9443062150286,52.7993284351279,13.7358808750203));
#82014=CARTESIAN_POINT('Ctrl Pts',(86.5719230975097,52.6733141906447,12.9157104604262));
#82015=CARTESIAN_POINT('Ctrl Pts',(86.5165867211766,52.5472999461614,11.3178829301715));
#82016=CARTESIAN_POINT('Ctrl Pts',(87.8289410747657,52.4212857016782,10.4047339933716));
#82017=CARTESIAN_POINT('Ctrl Pts',(89.3079162068262,52.2952714571951,11.0119798148115));
#82018=CARTESIAN_POINT('Ctrl Pts',(89.5999504185763,52.1692572127118,12.5838675188445));
#82019=CARTESIAN_POINT('Ctrl Pts',(88.4377732751979,52.0432429682286,13.6818015853059));
#82020=CARTESIAN_POINT('Ctrl Pts',(86.885012176931,51.9172287237453,13.3009500499704));
#82021=CARTESIAN_POINT('Ctrl Pts',(86.3627579151766,51.7912144792622,11.7898691610409));
#82022=CARTESIAN_POINT('Ctrl Pts',(87.3489788964379,51.6652002347788,10.5315039245408));
#82023=CARTESIAN_POINT('Ctrl Pts',(88.9410832105601,51.5391859902957,10.677513241439));
#82024=CARTESIAN_POINT('Ctrl Pts',(89.6819731072355,51.4131717458124,12.0942691767888));
#82025=CARTESIAN_POINT('Ctrl Pts',(88.8935842068198,51.2871575013293,13.4851528873972));
#82026=CARTESIAN_POINT('Ctrl Pts',(87.2974522081011,51.1611432568459,13.5772247732078));
#82027=CARTESIAN_POINT('Ctrl Pts',(86.3543606112868,51.0351290123629,12.2862191905969));
#82028=CARTESIAN_POINT('Ctrl Pts',(86.9274300864957,50.9091147678794,10.7936700953069));
#82029=CARTESIAN_POINT('Ctrl Pts',(88.4921842164508,50.7831005233964,10.4655572045636));
#82030=CARTESIAN_POINT('Ctrl Pts',(89.6165597833704,50.6570862789131,11.6021800653702));
#82031=CARTESIAN_POINT('Ctrl Pts',(89.2715182184349,50.5310720344298,13.1632789815833));
#82032=CARTESIAN_POINT('Ctrl Pts',(87.7728569572402,50.4050577899467,13.7201716606564));
#82033=CARTESIAN_POINT('Ctrl Pts',(86.4921254000443,50.2790435454634,12.7631099231059));
#82034=CARTESIAN_POINT('Ctrl Pts',(86.6015104434062,50.1530293009802,11.1681563364645));
#82035=CARTESIAN_POINT('Ctrl Pts',(88.0007861685625,50.027015056497,10.3947016636549));
#82036=CARTESIAN_POINT('Ctrl Pts',(89.4095649982335,49.9010008120137,11.1512431946305));
#82037=CARTESIAN_POINT('Ctrl Pts',(89.538062378686,49.7749865675306,12.7441320405629));
#82038=CARTESIAN_POINT('Ctrl Pts',(88.269617331335,49.6489723230473,13.7180798457492));
#82039=CARTESIAN_POINT('Ctrl Pts',(86.7631581136022,49.5229580785641,13.1765925149675));
#82040=CARTESIAN_POINT('Ctrl Pts',(86.5229457779753,49.4389485822419,12.1433653123349));
#82041=CARTESIAN_POINT('Ctrl Pts',(86.6479205797788,49.3969438340809,11.6901384145323));
#82042=CARTESIAN_POINT('Ctrl Pts',(88.7990966425285,64.9382998250767,11.0730545118016));
#82043=CARTESIAN_POINT('Ctrl Pts',(89.1293485756048,64.8962838430762,11.3351626605608));
#82044=CARTESIAN_POINT('Ctrl Pts',(89.5017660870752,64.8122631129146,12.2104685760909));
#82045=CARTESIAN_POINT('Ctrl Pts',(88.697060948392,64.6862376345919,13.3990394565308));
#82046=CARTESIAN_POINT('Ctrl Pts',(87.2636812704869,64.5602233901086,13.3643054127713));
#82047=CARTESIAN_POINT('Ctrl Pts',(86.5146860157324,64.4342091456255,12.1429131371986));
#82048=CARTESIAN_POINT('Ctrl Pts',(87.134902200258,64.3081949011423,10.8503566598342));
#82049=CARTESIAN_POINT('Ctrl Pts',(88.5570346765508,64.1821806566591,10.6707461277182));
#82050=CARTESIAN_POINT('Ctrl Pts',(89.4793801721819,64.0561664121758,11.7678824009764));
#82051=CARTESIAN_POINT('Ctrl Pts',(89.0578878395004,63.9301521676926,13.1379530990341));
#82052=CARTESIAN_POINT('Ctrl Pts',(87.6782675019479,63.8041379232094,13.5269214552082));
#82053=CARTESIAN_POINT('Ctrl Pts',(86.603171599567,63.6781236787262,12.5788749800865));
#82054=CARTESIAN_POINT('Ctrl Pts',(86.8165203183149,63.5521094342429,11.1614320091845));
#82055=CARTESIAN_POINT('Ctrl Pts',(88.123061503027,63.4260951897596,10.5718579218206));
#82056=CARTESIAN_POINT('Ctrl Pts',(89.3270428700885,63.3000809452764,11.3497233514816));
#82057=CARTESIAN_POINT('Ctrl Pts',(89.3265789729973,63.1740667007934,12.7831284459591));
#82058=CARTESIAN_POINT('Ctrl Pts',(88.1220937321693,63.04805245631,13.5602150608074));
#82059=CARTESIAN_POINT('Ctrl Pts',(86.8159353393254,62.9220382118268,12.9697927312709));
#82060=CARTESIAN_POINT('Ctrl Pts',(86.6035030271439,62.7960239673435,11.5522168703809));
#82061=CARTESIAN_POINT('Ctrl Pts',(87.679215453102,62.6700097228603,10.6048566946338));
#82062=CARTESIAN_POINT('Ctrl Pts',(89.0585779038768,62.5439954783771,10.9947384397243));
#82063=CARTESIAN_POINT('Ctrl Pts',(89.4791944720911,62.4179812338939,12.365041438403));
#82064=CARTESIAN_POINT('Ctrl Pts',(88.5561158239914,62.2919669894107,13.4616609611405));
#82065=CARTESIAN_POINT('Ctrl Pts',(87.1341458268856,62.1659527449274,13.280968125407));
#82066=CARTESIAN_POINT('Ctrl Pts',(86.514674937414,62.0399385004443,11.9883334526898));
#82067=CARTESIAN_POINT('Ctrl Pts',(87.2646444473611,61.9139242559609,10.7667793976723));
#82068=CARTESIAN_POINT('Ctrl Pts',(88.6976804052685,61.7879100114779,10.7342752512863));
#82069=CARTESIAN_POINT('Ctrl Pts',(89.5022647576141,61.6618957669944,11.920568889813));
#82070=CARTESIAN_POINT('Ctrl Pts',(88.942039914533,61.5358815225114,13.2399614399788));
#82071=CARTESIAN_POINT('Ctrl Pts',(87.5297250384181,61.409867278028,13.4849415761304));
#82072=CARTESIAN_POINT('Ctrl Pts',(86.5578741977455,61.2838530335449,12.4313028714737));
#82073=CARTESIAN_POINT('Ctrl Pts',(86.9159276861581,61.1578387890616,11.0433380751525));
#82074=CARTESIAN_POINT('Ctrl Pts',(88.2761940652707,61.0318245445784,10.5913160023808));
#82075=CARTESIAN_POINT('Ctrl Pts',(89.3937541797914,60.9058103000952,11.4889283724238));
#82076=CARTESIAN_POINT('Ctrl Pts',(89.2458142482015,60.779796055612,12.9146781236264));
#82077=CARTESIAN_POINT('Ctrl Pts',(87.9677692618783,60.6537818111288,13.5637155565615));
#82078=CARTESIAN_POINT('Ctrl Pts',(86.7292891540317,60.5277675666455,12.8420400069658));
#82079=CARTESIAN_POINT('Ctrl Pts',(86.663833983211,60.4017533221623,11.4101307231672));
#82080=CARTESIAN_POINT('Ctrl Pts',(87.8313084836797,60.2757390776791,10.5784746240662));
#82081=CARTESIAN_POINT('Ctrl Pts',(89.1632371044194,60.1497248331959,11.1082054289759));
#82082=CARTESIAN_POINT('Ctrl Pts',(89.4406354767009,60.0237105887127,12.5145121947534));
#82083=CARTESIAN_POINT('Ctrl Pts',(88.4096279239622,59.8976963442293,13.5103394903283));
#82084=CARTESIAN_POINT('Ctrl Pts',(87.0137951090567,59.7716820997463,13.1843037112354));
#82085=CARTESIAN_POINT('Ctrl Pts',(86.5306066773052,59.6456678552628,11.8347936090732));
#82086=CARTESIAN_POINT('Ctrl Pts',(87.4022778767963,59.5196536107797,10.6968841678635));
#82087=CARTESIAN_POINT('Ctrl Pts',(88.8310530693473,59.3936393662964,10.8119929232504));
#82088=CARTESIAN_POINT('Ctrl Pts',(89.5093136641206,59.2676251218134,12.0747720575386));
#82089=CARTESIAN_POINT('Ctrl Pts',(88.8163138868459,59.14161087733,13.3295229830665));
#82090=CARTESIAN_POINT('Ctrl Pts',(87.3862888480817,59.0155966328469,13.4278945486906));
#82091=CARTESIAN_POINT('Ctrl Pts',(86.5280010010119,58.8895823883636,12.2798568541925));
#82092=CARTESIAN_POINT('Ctrl Pts',(87.0269575065745,58.7635681438805,10.9360968376817));
#82093=CARTESIAN_POINT('Ctrl Pts',(88.4265121365204,58.6375538993971,10.6264269905669));
#82094=CARTESIAN_POINT('Ctrl Pts',(89.4457890311971,58.511539654914,11.6342579230129));
#82095=CARTESIAN_POINT('Ctrl Pts',(89.1519434550291,58.3855254104306,13.0372202723946));
#82096=CARTESIAN_POINT('Ctrl Pts',(87.8139036062642,58.2595111659476,13.5513194258006));
#82097=CARTESIAN_POINT('Ctrl Pts',(86.6562468646385,58.1334969214642,12.7060505662153));
#82098=CARTESIAN_POINT('Ctrl Pts',(86.7384635439892,58.007482676981,11.2750058450229));
#82099=CARTESIAN_POINT('Ctrl Pts',(87.9853087359807,57.8814684324977,10.5678809312884));
#82100=CARTESIAN_POINT('Ctrl Pts',(89.2556666363595,57.7554541880146,11.2318382954022));
#82101=CARTESIAN_POINT('Ctrl Pts',(89.3869025519891,57.6294399435314,12.659222515178));
#82102=CARTESIAN_POINT('Ctrl Pts',(88.2589090482235,57.5034256990482,13.5436880215029));
#82103=CARTESIAN_POINT('Ctrl Pts',(86.904028570227,57.3774114545649,13.0757697949289));
#82104=CARTESIAN_POINT('Ctrl Pts',(86.5622510832708,57.2513972100816,11.6837077539889));
#82105=CARTESIAN_POINT('Ctrl Pts',(87.5463721889326,57.1253829655985,10.6415205223426));
#82106=CARTESIAN_POINT('Ctrl Pts',(88.9557218167158,56.9993687211153,10.9030204326364));
#82107=CARTESIAN_POINT('Ctrl Pts',(89.5004597007143,56.873354476632,12.2288821200505));
#82108=CARTESIAN_POINT('Ctrl Pts',(88.6820403818779,56.7473402321489,13.405673688244));
#82109=CARTESIAN_POINT('Ctrl Pts',(87.2494832454748,56.6213259876655,13.3563925827677));
#82110=CARTESIAN_POINT('Ctrl Pts',(86.5138681267126,56.4953117431823,12.1261409932689));
#82111=CARTESIAN_POINT('Ctrl Pts',(87.1484318021042,56.3692974986991,10.8408482179489));
#82112=CARTESIAN_POINT('Ctrl Pts',(88.5724200260982,56.243283254216,10.6768173844378));
#82113=CARTESIAN_POINT('Ctrl Pts',(89.4825952533226,56.1172690097327,11.7841699173571));
#82114=CARTESIAN_POINT('Ctrl Pts',(89.0459628641595,55.9912547652494,13.1494540391244));
#82115=CARTESIAN_POINT('Ctrl Pts',(87.662129901346,55.8652405207662,13.5231583439522));
#82116=CARTESIAN_POINT('Ctrl Pts',(86.5975837158827,55.7392262762831,12.5632677275634));
#82117=CARTESIAN_POINT('Ctrl Pts',(86.8265996102624,55.6132120317998,11.1482764567289));
#82118=CARTESIAN_POINT('Ctrl Pts',(88.139581671392,55.4871977873166,10.5731880430321));
#82119=CARTESIAN_POINT('Ctrl Pts',(89.334885468768,55.3611835428333,11.3643248253865));
#82120=CARTESIAN_POINT('Ctrl Pts',(89.3185660099971,55.2351692983502,12.7976364634058));
#82121=CARTESIAN_POINT('Ctrl Pts',(88.1055589041179,55.1091550538668,13.5613526001369));
#82122=CARTESIAN_POINT('Ctrl Pts',(86.8060112552633,54.9831408093836,12.9565183379033));
#82123=CARTESIAN_POINT('Ctrl Pts',(86.6092722865862,54.8571265649004,11.536679489787));
#82124=CARTESIAN_POINT('Ctrl Pts',(87.6953979889286,54.7311123204173,10.601276082092));
#82125=CARTESIAN_POINT('Ctrl Pts',(89.070363432564,54.6050980759339,11.0063916276142));
#82126=CARTESIAN_POINT('Ctrl Pts',(89.4757968419816,54.4790838314508,12.3812633768855));
#82127=CARTESIAN_POINT('Ctrl Pts',(88.540644557889,54.3530695869675,13.4676053037081));
#82128=CARTESIAN_POINT('Ctrl Pts',(87.1207602641408,54.2270553424844,13.271194589177));
#82129=CARTESIAN_POINT('Ctrl Pts',(86.5156255789948,54.101041098001,11.971786805127));
#82130=CARTESIAN_POINT('Ctrl Pts',(87.2790612633266,53.975026853518,10.7586031700967));
#82131=CARTESIAN_POINT('Ctrl Pts',(88.7123690901885,53.8490126090346,10.7419523481339));
#82132=CARTESIAN_POINT('Ctrl Pts',(89.5037821906086,53.7229983645515,11.9370732126907));
#82133=CARTESIAN_POINT('Ctrl Pts',(88.928997337223,53.5969841200682,13.2501881919425));
#82134=CARTESIAN_POINT('Ctrl Pts',(87.5140590497977,53.4709698755849,13.479531208391));
#82135=CARTESIAN_POINT('Ctrl Pts',(86.553922349369,53.3449556311017,12.415206966018));
#82136=CARTESIAN_POINT('Ctrl Pts',(86.9273067194287,53.2189413866186,11.0312876444473));
#82137=CARTESIAN_POINT('Ctrl Pts',(88.2924898607941,53.0929271421353,10.5943396304358));
#82138=CARTESIAN_POINT('Ctrl Pts',(89.400052785185,52.9669128976521,11.5042588273461));
#82139=CARTESIAN_POINT('Ctrl Pts',(89.2363511642362,52.8408986531688,12.9282849351706));
#82140=CARTESIAN_POINT('Ctrl Pts',(87.9512051263928,52.7148844086857,13.5631457370948));
#82141=CARTESIAN_POINT('Ctrl Pts',(86.7207835048331,52.5888701642023,12.8278150567635));
#82142=CARTESIAN_POINT('Ctrl Pts',(86.6711712114218,52.4628559197193,11.3952693516667));
#82143=CARTESIAN_POINT('Ctrl Pts',(87.8477735400219,52.3368416752359,10.5765779955867));
#82144=CARTESIAN_POINT('Ctrl Pts',(89.1737611283324,52.2108274307528,11.1210093418804));
#82145=CARTESIAN_POINT('Ctrl Pts',(89.435586855992,52.0848131862694,12.5302984777034));
#82146=CARTESIAN_POINT('Ctrl Pts',(88.3936271677379,51.9587989417864,13.5146604952599));
#82147=CARTESIAN_POINT('Ctrl Pts',(87.0014861511104,51.832784697303,13.1732048494572));
#82148=CARTESIAN_POINT('Ctrl Pts',(86.5332547021724,51.7067704528199,11.8184325749146));
#82149=CARTESIAN_POINT('Ctrl Pts',(87.4174594140269,51.5807562083366,10.6902346431241));
#82150=CARTESIAN_POINT('Ctrl Pts',(88.8448739215852,51.4547419638534,10.8211405236814));
#82151=CARTESIAN_POINT('Ctrl Pts',(89.5091249870697,51.3287277193701,12.0913449681073));
#82152=CARTESIAN_POINT('Ctrl Pts',(88.8022882904604,51.202713474887,13.3383534519352));
#82153=CARTESIAN_POINT('Ctrl Pts',(87.3712627284166,51.0766992304037,13.4209012752018));
#82154=CARTESIAN_POINT('Ctrl Pts',(86.5257260287742,50.9506849859204,12.2634393667001));
#82155=CARTESIAN_POINT('Ctrl Pts',(87.0395162845361,50.8246707414373,10.9252819275408));
#82156=CARTESIAN_POINT('Ctrl Pts',(88.4424097545478,50.698656496954,10.6311095569182));
#82157=CARTESIAN_POINT('Ctrl Pts',(89.4504781216323,50.5726422524708,11.6501583382993));
#82158=CARTESIAN_POINT('Ctrl Pts',(89.1411282058441,50.4466280079875,13.0497746957017));
#82159=CARTESIAN_POINT('Ctrl Pts',(87.7974908529584,50.3206137635044,13.5490615088904));
#82160=CARTESIAN_POINT('Ctrl Pts',(86.6492402083156,50.1945995190211,12.6909997621248));
#82161=CARTESIAN_POINT('Ctrl Pts',(86.7473102885359,50.0685852745379,11.2610307153356));
#82162=CARTESIAN_POINT('Ctrl Pts',(88.0018427035575,49.9425710300547,10.567583426038));
#82163=CARTESIAN_POINT('Ctrl Pts',(89.2648952068242,49.8165567855714,11.2458670958365));
#82164=CARTESIAN_POINT('Ctrl Pts',(89.3801006135392,49.6905425410883,12.673984981985));
#82165=CARTESIAN_POINT('Ctrl Pts',(88.2428655425899,49.564528296605,13.5471860746496));
#82166=CARTESIAN_POINT('Ctrl Pts',(86.8922368662129,49.4385140521219,13.0617110559835));
#82167=CARTESIAN_POINT('Ctrl Pts',(86.6768724772548,49.3545045557997,12.1353625211796));
#82168=CARTESIAN_POINT('Ctrl Pts',(86.788919686468,49.3124998076386,11.7290181357015));
#82169=CARTESIAN_POINT('Ctrl Pts',(88.8060699928714,64.9396,13.5735272939604));
#82170=CARTESIAN_POINT('Ctrl Pts',(88.8129681618595,64.9396,13.5698282373507));
#82171=CARTESIAN_POINT('Ctrl Pts',(88.8198663308475,64.9396,13.5661291807411));
#82172=CARTESIAN_POINT('Ctrl Pts',(88.8267644998355,64.9396,13.5624301241315));
#82173=CARTESIAN_POINT('Origin',(88.011,64.9396,12.066));
#82174=CARTESIAN_POINT('',(88.011,65.0896,10.21166));
#82175=CARTESIAN_POINT('Origin',(88.011,65.0896,12.066));
#82176=CARTESIAN_POINT('Origin',(88.011,64.9396,10.21166));
#82177=CARTESIAN_POINT('Origin',(88.011,65.0896,12.066));
#82178=CARTESIAN_POINT('',(85.1408,65.0896,12.066));
#82179=CARTESIAN_POINT('Origin',(88.011,65.0896,12.066));
#82180=CARTESIAN_POINT('Origin',(88.011,49.3896,12.066));
#82181=CARTESIAN_POINT('',(86.65666,49.2146,12.066));
#82182=CARTESIAN_POINT('',(86.48166,49.3896,12.066));
#82183=CARTESIAN_POINT('Origin',(88.011,49.2146,12.066));
#82184=CARTESIAN_POINT('Origin',(88.011,49.2146,12.066));
#82185=CARTESIAN_POINT('Origin',(91.160821247026,68.5948,11.6730697876423));
#82186=CARTESIAN_POINT('',(90.8451530928687,65.6896,11.6125418584009));
#82187=CARTESIAN_POINT('',(90.8451530928687,68.2948,11.6125418584009));
#82188=CARTESIAN_POINT('',(90.8451530928687,65.0896,11.6125418584009));
#82189=CARTESIAN_POINT('',(90.7194182823342,65.6896,11.5884327817804));
#82190=CARTESIAN_POINT('',(91.160821247026,65.6896,11.6730697876423));
#82191=CARTESIAN_POINT('',(90.7194182823342,68.4148,11.5884327817804));
#82192=CARTESIAN_POINT('',(90.7194182823342,68.5948,11.5884327817804));
#82193=CARTESIAN_POINT('Ctrl Pts',(90.8451530928688,68.2948,11.6125418584009));
#82194=CARTESIAN_POINT('Ctrl Pts',(90.780943418612,68.3562581248798,11.6002299461321));
#82195=CARTESIAN_POINT('Ctrl Pts',(90.7194182823342,68.4148,11.5884327817804));
#82196=CARTESIAN_POINT('Origin',(90.7194182823342,68.5948,11.5884327817804));
#82197=CARTESIAN_POINT('',(90.8293245661282,68.2948,11.5227738224662));
#82198=CARTESIAN_POINT('',(90.8293245661282,65.6896,11.5227738224662));
#82199=CARTESIAN_POINT('',(90.8293245661282,65.0896,11.5227738224662));
#82200=CARTESIAN_POINT('Ctrl Pts',(90.7194182823342,68.4148,11.5884327817804));
#82201=CARTESIAN_POINT('Ctrl Pts',(90.7731981310438,68.356258124881,11.5563042375657));
#82202=CARTESIAN_POINT('Ctrl Pts',(90.8293245661282,68.2948,11.5227738224661));
#82203=CARTESIAN_POINT('',(90.7194182823342,65.6896,11.5884327817804));
#82204=CARTESIAN_POINT('Origin',(90.9262279104668,65.6896,11.5519666644704));
#82205=CARTESIAN_POINT('Origin',(88.011,65.6896,12.066));
#82206=CARTESIAN_POINT('Origin',(88.011,68.4448,12.066));
#82207=CARTESIAN_POINT('',(85.2608,68.4148,12.066));
#82208=CARTESIAN_POINT('',(85.1411618809824,68.2948,12.1115764262924));
#82209=CARTESIAN_POINT('Ctrl Pts',(85.2608,68.4148,12.066));
#82210=CARTESIAN_POINT('Ctrl Pts',(85.2022581248795,68.3562581248795,12.0883016667126));
#82211=CARTESIAN_POINT('Ctrl Pts',(85.1411618809824,68.2948,12.1115764262924));
#82212=CARTESIAN_POINT('',(85.1768469071313,68.2948,12.5194581415991));
#82213=CARTESIAN_POINT('Origin',(88.011,68.2948,12.066));
#82214=CARTESIAN_POINT('',(85.3025817176658,68.4148,12.5435672182196));
#82215=CARTESIAN_POINT('Ctrl Pts',(85.1768469071312,68.2948,12.5194581415991));
#82216=CARTESIAN_POINT('Ctrl Pts',(85.2410565813881,68.3562581248799,12.5317700538679));
#82217=CARTESIAN_POINT('Ctrl Pts',(85.3025817176658,68.4148,12.5435672182196));
#82218=CARTESIAN_POINT('',(85.1926754338717,68.2948,12.6092261775339));
#82219=CARTESIAN_POINT('Ctrl Pts',(85.3025817176658,68.4148,12.5435672182196));
#82220=CARTESIAN_POINT('Ctrl Pts',(85.2488018689554,68.3562581248801,12.5756957624348));
#82221=CARTESIAN_POINT('Ctrl Pts',(85.1926754338717,68.2948,12.6092261775339));
#82222=CARTESIAN_POINT('',(85.2986462408562,68.2948,13.0047146133191));
#82223=CARTESIAN_POINT('Origin',(88.011,68.2948,12.066));
#82224=CARTESIAN_POINT('',(85.4266573543146,68.4148,13.0066237981742));
#82225=CARTESIAN_POINT('Ctrl Pts',(85.2986462408562,68.2948,13.0047146133191));
#82226=CARTESIAN_POINT('Ctrl Pts',(85.3640183670116,68.3562581248796,13.0056895870525));
#82227=CARTESIAN_POINT('Ctrl Pts',(85.4266573543146,68.4148,13.0066237981742));
#82228=CARTESIAN_POINT('',(85.3298223525619,68.2948,13.0903702762566));
#82229=CARTESIAN_POINT('Ctrl Pts',(85.4266573543146,68.4148,13.0066237981742));
#82230=CARTESIAN_POINT('Ctrl Pts',(85.3792736055028,68.3562581248801,13.0476030103342));
#82231=CARTESIAN_POINT('Ctrl Pts',(85.3298223525618,68.2948,13.0903702762567));
#82232=CARTESIAN_POINT('',(85.5028590710356,68.2948,13.4614487165259));
#82233=CARTESIAN_POINT('Origin',(88.011,68.2948,12.066));
#82234=CARTESIAN_POINT('',(85.629256934512,68.4148,13.4411));
#82235=CARTESIAN_POINT('Ctrl Pts',(85.5028590710356,68.2948,13.4614487165259));
#82236=CARTESIAN_POINT('Ctrl Pts',(85.5674073501147,68.3562581248781,13.4510571276407));
#82237=CARTESIAN_POINT('Ctrl Pts',(85.629256934512,68.4148,13.4411));
#82238=CARTESIAN_POINT('',(85.548435497328,68.2948,13.5403894024917));
#82239=CARTESIAN_POINT('Ctrl Pts',(85.629256934512,68.4148,13.4411));
#82240=CARTESIAN_POINT('Ctrl Pts',(85.5897090168301,68.3562581248814,13.4896847474785));
#82241=CARTESIAN_POINT('Ctrl Pts',(85.548435497328,68.2948,13.5403894024917));
#82242=CARTESIAN_POINT('',(85.783280494161,68.2948,13.8757828166121));
#82243=CARTESIAN_POINT('Origin',(88.011,68.2948,12.066));
#82244=CARTESIAN_POINT('',(85.9042245725342,68.4148,13.8337944841599));
#82245=CARTESIAN_POINT('Ctrl Pts',(85.783280494161,68.2948,13.8757828166121));
#82246=CARTESIAN_POINT('Ctrl Pts',(85.8450436593707,68.35625812488,13.8543404082776));
#82247=CARTESIAN_POINT('Ctrl Pts',(85.9042245725342,68.4148,13.8337944841599));
#82248=CARTESIAN_POINT('',(85.8418724183901,68.2948,13.9456099528092));
#82249=CARTESIAN_POINT('Ctrl Pts',(85.9042245725342,68.4148,13.8337944841599));
#82250=CARTESIAN_POINT('Ctrl Pts',(85.8737141294464,68.3562581248792,13.888508543993));
#82251=CARTESIAN_POINT('Ctrl Pts',(85.8418724183901,68.2948,13.9456099528092));
#82252=CARTESIAN_POINT('',(86.1313900471908,68.2948,14.2351275816099));
#82253=CARTESIAN_POINT('Origin',(88.011,68.2948,12.066));
#82254=CARTESIAN_POINT('',(86.2432055158401,68.4148,14.1727754274658));
#82255=CARTESIAN_POINT('Ctrl Pts',(86.1313900471908,68.2948,14.2351275816099));
#82256=CARTESIAN_POINT('Ctrl Pts',(86.1884914560068,68.3562581248789,14.2032858705537));
#82257=CARTESIAN_POINT('Ctrl Pts',(86.2432055158401,68.4148,14.1727754274658));
#82258=CARTESIAN_POINT('',(86.2012171833879,68.2948,14.293719505839));
#82259=CARTESIAN_POINT('Ctrl Pts',(86.2432055158401,68.4148,14.1727754274658));
#82260=CARTESIAN_POINT('Ctrl Pts',(86.2226595917223,68.3562581248796,14.2319563406297));
#82261=CARTESIAN_POINT('Ctrl Pts',(86.2012171833879,68.2948,14.293719505839));
#82262=CARTESIAN_POINT('',(86.5366105975083,68.2948,14.528564502672));
#82263=CARTESIAN_POINT('Origin',(88.011,68.2948,12.066));
#82264=CARTESIAN_POINT('',(86.6359,68.4148,14.447743065488));
#82265=CARTESIAN_POINT('Ctrl Pts',(86.5366105975083,68.2948,14.528564502672));
#82266=CARTESIAN_POINT('Ctrl Pts',(86.5873152525206,68.3562581248803,14.4872909831707));
#82267=CARTESIAN_POINT('Ctrl Pts',(86.6359,68.4148,14.447743065488));
#82268=CARTESIAN_POINT('',(86.6155512834742,68.2948,14.5741409289644));
#82269=CARTESIAN_POINT('Ctrl Pts',(86.6359,68.4148,14.447743065488));
#82270=CARTESIAN_POINT('Ctrl Pts',(86.6259428723596,68.3562581248798,14.5095926498835));
#82271=CARTESIAN_POINT('Ctrl Pts',(86.6155512834741,68.2948,14.5741409289644));
#82272=CARTESIAN_POINT('',(86.9866297237434,68.2948,14.7471776474381));
#82273=CARTESIAN_POINT('Origin',(88.011,68.2948,12.066));
#82274=CARTESIAN_POINT('',(87.0703762018258,68.4148,14.6503426456854));
#82275=CARTESIAN_POINT('Ctrl Pts',(86.9866297237434,68.2948,14.7471776474382));
#82276=CARTESIAN_POINT('Ctrl Pts',(87.029396989666,68.3562581248803,14.697726394497));
#82277=CARTESIAN_POINT('Ctrl Pts',(87.0703762018258,68.4148,14.6503426456854));
#82278=CARTESIAN_POINT('',(87.0722853866809,68.2948,14.7783537591437));
#82279=CARTESIAN_POINT('Ctrl Pts',(87.0703762018258,68.4148,14.6503426456854));
#82280=CARTESIAN_POINT('Ctrl Pts',(87.0713104129475,68.3562581248798,14.7129816329883));
#82281=CARTESIAN_POINT('Ctrl Pts',(87.0722853866809,68.2948,14.7783537591438));
#82282=CARTESIAN_POINT('',(87.4677738224661,68.2948,14.8843245661282));
#82283=CARTESIAN_POINT('Origin',(88.011,68.2948,12.066));
#82284=CARTESIAN_POINT('',(87.5334327817804,68.4148,14.7744182823342));
#82285=CARTESIAN_POINT('Ctrl Pts',(87.4677738224661,68.2948,14.8843245661283));
#82286=CARTESIAN_POINT('Ctrl Pts',(87.5013042375649,68.3562581248796,14.8281981310451));
#82287=CARTESIAN_POINT('Ctrl Pts',(87.5334327817804,68.4148,14.7744182823342));
#82288=CARTESIAN_POINT('',(87.5575418584009,68.2948,14.9001530928687));
#82289=CARTESIAN_POINT('Ctrl Pts',(87.5334327817804,68.4148,14.7744182823342));
#82290=CARTESIAN_POINT('Ctrl Pts',(87.545229946132,68.35625812488,14.8359434186118));
#82291=CARTESIAN_POINT('Ctrl Pts',(87.5575418584008,68.2948,14.9001530928687));
#82292=CARTESIAN_POINT('',(87.9654235737076,68.2948,14.9358381190176));
#82293=CARTESIAN_POINT('Origin',(88.011,68.2948,12.066));
#82294=CARTESIAN_POINT('',(88.011,68.4148,14.8162));
#82295=CARTESIAN_POINT('Ctrl Pts',(87.9654235737076,68.2948,14.9358381190176));
#82296=CARTESIAN_POINT('Ctrl Pts',(87.9886983332876,68.35625812488,14.87474187512));
#82297=CARTESIAN_POINT('Ctrl Pts',(88.011,68.4148,14.8162));
#82298=CARTESIAN_POINT('',(88.0565764262924,68.2948,14.9358381190176));
#82299=CARTESIAN_POINT('Ctrl Pts',(88.011,68.4148,14.8162));
#82300=CARTESIAN_POINT('Ctrl Pts',(88.0333016667125,68.3562581248797,14.8747418751203));
#82301=CARTESIAN_POINT('Ctrl Pts',(88.0565764262924,68.2948,14.9358381190176));
#82302=CARTESIAN_POINT('',(88.4644581415992,68.2948,14.9001530928687));
#82303=CARTESIAN_POINT('Origin',(88.011,68.2948,12.066));
#82304=CARTESIAN_POINT('',(88.4885672182196,68.4148,14.7744182823342));
#82305=CARTESIAN_POINT('Ctrl Pts',(88.4644581415992,68.2948,14.9001530928688));
#82306=CARTESIAN_POINT('Ctrl Pts',(88.476770053868,68.3562581248804,14.8359434186114));
#82307=CARTESIAN_POINT('Ctrl Pts',(88.4885672182196,68.4148,14.7744182823342));
#82308=CARTESIAN_POINT('',(88.5542261775338,68.2948,14.8843245661282));
#82309=CARTESIAN_POINT('Ctrl Pts',(88.4885672182196,68.4148,14.7744182823342));
#82310=CARTESIAN_POINT('Ctrl Pts',(88.5206957624349,68.3562581248798,14.8281981310449));
#82311=CARTESIAN_POINT('Ctrl Pts',(88.5542261775338,68.2948,14.8843245661283));
#82312=CARTESIAN_POINT('',(88.9497146133191,68.2948,14.7783537591437));
#82313=CARTESIAN_POINT('Origin',(88.011,68.2948,12.066));
#82314=CARTESIAN_POINT('',(88.9516237981743,68.4148,14.6503426456854));
#82315=CARTESIAN_POINT('Ctrl Pts',(88.9497146133191,68.2948,14.7783537591438));
#82316=CARTESIAN_POINT('Ctrl Pts',(88.9506895870525,68.3562581248811,14.7129816329868));
#82317=CARTESIAN_POINT('Ctrl Pts',(88.9516237981743,68.4148,14.6503426456854));
#82318=CARTESIAN_POINT('',(89.0353702762567,68.2948,14.7471776474381));
#82319=CARTESIAN_POINT('Ctrl Pts',(88.9516237981743,68.4148,14.6503426456854));
#82320=CARTESIAN_POINT('Ctrl Pts',(88.9926030103332,68.3562581248815,14.6977263944961));
#82321=CARTESIAN_POINT('Ctrl Pts',(89.0353702762566,68.2948,14.7471776474381));
#82322=CARTESIAN_POINT('',(89.4064487165259,68.2948,14.5741409289644));
#82323=CARTESIAN_POINT('Origin',(88.011,68.2948,12.066));
#82324=CARTESIAN_POINT('',(89.3861,68.4148,14.447743065488));
#82325=CARTESIAN_POINT('Ctrl Pts',(89.4064487165259,68.2948,14.5741409289644));
#82326=CARTESIAN_POINT('Ctrl Pts',(89.3960571276401,68.3562581248814,14.5095926498817));
#82327=CARTESIAN_POINT('Ctrl Pts',(89.3861,68.4148,14.447743065488));
#82328=CARTESIAN_POINT('',(89.4853894024917,68.2948,14.528564502672));
#82329=CARTESIAN_POINT('Ctrl Pts',(89.3861,68.4148,14.447743065488));
#82330=CARTESIAN_POINT('Ctrl Pts',(89.4346847474787,68.3562581248812,14.4872909831701));
#82331=CARTESIAN_POINT('Ctrl Pts',(89.4853894024917,68.2948,14.528564502672));
#82332=CARTESIAN_POINT('',(89.8207828166121,68.2948,14.293719505839));
#82333=CARTESIAN_POINT('Origin',(88.011,68.2948,12.066));
#82334=CARTESIAN_POINT('',(89.7787944841599,68.4148,14.1727754274658));
#82335=CARTESIAN_POINT('Ctrl Pts',(89.8207828166121,68.2948,14.293719505839));
#82336=CARTESIAN_POINT('Ctrl Pts',(89.7993404082776,68.35625812488,14.2319563406293));
#82337=CARTESIAN_POINT('Ctrl Pts',(89.7787944841599,68.4148,14.1727754274658));
#82338=CARTESIAN_POINT('',(89.8906099528091,68.2948,14.2351275816099));
#82339=CARTESIAN_POINT('Ctrl Pts',(89.7787944841599,68.4148,14.1727754274658));
#82340=CARTESIAN_POINT('Ctrl Pts',(89.8335085439913,68.3562581248809,14.2032858705527));
#82341=CARTESIAN_POINT('Ctrl Pts',(89.8906099528091,68.2948,14.2351275816099));
#82342=CARTESIAN_POINT('',(90.1801275816099,68.2948,13.9456099528092));
#82343=CARTESIAN_POINT('Origin',(88.011,68.2948,12.066));
#82344=CARTESIAN_POINT('',(90.1177754274658,68.4148,13.8337944841599));
#82345=CARTESIAN_POINT('Ctrl Pts',(90.1801275816099,68.2948,13.9456099528092));
#82346=CARTESIAN_POINT('Ctrl Pts',(90.1482858705531,68.3562581248803,13.8885085439919));
#82347=CARTESIAN_POINT('Ctrl Pts',(90.1177754274658,68.4148,13.8337944841599));
#82348=CARTESIAN_POINT('',(90.238719505839,68.2948,13.8757828166121));
#82349=CARTESIAN_POINT('Ctrl Pts',(90.1177754274658,68.4148,13.8337944841599));
#82350=CARTESIAN_POINT('Ctrl Pts',(90.176956340628,68.3562581248813,13.8543404082771));
#82351=CARTESIAN_POINT('Ctrl Pts',(90.238719505839,68.2948,13.8757828166121));
#82352=CARTESIAN_POINT('',(90.473564502672,68.2948,13.5403894024917));
#82353=CARTESIAN_POINT('Origin',(88.011,68.2948,12.066));
#82354=CARTESIAN_POINT('',(90.392743065488,68.4148,13.4411));
#82355=CARTESIAN_POINT('Ctrl Pts',(90.473564502672,68.2948,13.5403894024917));
#82356=CARTESIAN_POINT('Ctrl Pts',(90.4322909831698,68.3562581248816,13.4896847474783));
#82357=CARTESIAN_POINT('Ctrl Pts',(90.392743065488,68.4148,13.4411));
#82358=CARTESIAN_POINT('',(90.5191409289644,68.2948,13.4614487165259));
#82359=CARTESIAN_POINT('Ctrl Pts',(90.392743065488,68.4148,13.4411));
#82360=CARTESIAN_POINT('Ctrl Pts',(90.4545926498819,68.3562581248813,13.4510571276401));
#82361=CARTESIAN_POINT('Ctrl Pts',(90.5191409289644,68.2948,13.4614487165259));
#82362=CARTESIAN_POINT('',(90.6921776474381,68.2948,13.0903702762567));
#82363=CARTESIAN_POINT('Origin',(88.011,68.2948,12.066));
#82364=CARTESIAN_POINT('',(90.5953426456854,68.4148,13.0066237981743));
#82365=CARTESIAN_POINT('Ctrl Pts',(90.6921776474381,68.2948,13.0903702762567));
#82366=CARTESIAN_POINT('Ctrl Pts',(90.6427263944977,68.3562581248795,13.0476030103346));
#82367=CARTESIAN_POINT('Ctrl Pts',(90.5953426456854,68.4148,13.0066237981743));
#82368=CARTESIAN_POINT('',(90.7233537591437,68.2948,13.0047146133191));
#82369=CARTESIAN_POINT('Ctrl Pts',(90.5953426456854,68.4148,13.0066237981743));
#82370=CARTESIAN_POINT('Ctrl Pts',(90.6579816329875,68.3562581248805,13.0056895870525));
#82371=CARTESIAN_POINT('Ctrl Pts',(90.7233537591438,68.2948,13.0047146133191));
#82372=CARTESIAN_POINT('',(90.8293245661282,68.2948,12.6092261775338));
#82373=CARTESIAN_POINT('Origin',(88.011,68.2948,12.066));
#82374=CARTESIAN_POINT('',(90.7194182823342,68.4148,12.5435672182196));
#82375=CARTESIAN_POINT('Ctrl Pts',(90.8293245661282,68.2948,12.6092261775338));
#82376=CARTESIAN_POINT('Ctrl Pts',(90.7731981310446,68.3562581248802,12.5756957624347));
#82377=CARTESIAN_POINT('Ctrl Pts',(90.7194182823342,68.4148,12.5435672182196));
#82378=CARTESIAN_POINT('',(90.8451530928687,68.2948,12.5194581415991));
#82379=CARTESIAN_POINT('Ctrl Pts',(90.7194182823342,68.4148,12.5435672182196));
#82380=CARTESIAN_POINT('Ctrl Pts',(90.7809434186119,68.3562581248799,12.5317700538679));
#82381=CARTESIAN_POINT('Ctrl Pts',(90.8451530928687,68.2948,12.5194581415991));
#82382=CARTESIAN_POINT('',(90.8808381190176,68.2948,12.1115764262924));
#82383=CARTESIAN_POINT('Origin',(88.011,68.2948,12.066));
#82384=CARTESIAN_POINT('',(90.7612,68.4148,12.066));
#82385=CARTESIAN_POINT('Ctrl Pts',(90.8808381190176,68.2948,12.1115764262924));
#82386=CARTESIAN_POINT('Ctrl Pts',(90.81974187512,68.35625812488,12.0883016667124));
#82387=CARTESIAN_POINT('Ctrl Pts',(90.7612,68.4148,12.066));
#82388=CARTESIAN_POINT('',(90.8808381190176,68.2948,12.0204235737076));
#82389=CARTESIAN_POINT('Ctrl Pts',(90.7612,68.4148,12.066));
#82390=CARTESIAN_POINT('Ctrl Pts',(90.8197418751187,68.3562581248813,12.0436983332881));
#82391=CARTESIAN_POINT('Ctrl Pts',(90.8808381190176,68.2948,12.0204235737076));
#82392=CARTESIAN_POINT('Origin',(88.011,68.2948,12.066));
#82393=CARTESIAN_POINT('',(90.7233537591437,68.2948,11.1272853866809));
#82394=CARTESIAN_POINT('Origin',(88.011,68.2948,12.066));
#82395=CARTESIAN_POINT('',(90.5953426456854,68.4148,11.1253762018257));
#82396=CARTESIAN_POINT('Ctrl Pts',(90.7233537591438,68.2948,11.1272853866809));
#82397=CARTESIAN_POINT('Ctrl Pts',(90.6579816329897,68.3562581248785,11.1263104129475));
#82398=CARTESIAN_POINT('Ctrl Pts',(90.5953426456854,68.4148,11.1253762018257));
#82399=CARTESIAN_POINT('',(90.6921776474381,68.2948,11.0416297237434));
#82400=CARTESIAN_POINT('Ctrl Pts',(90.5953426456854,68.4148,11.1253762018257));
#82401=CARTESIAN_POINT('Ctrl Pts',(90.6427263944974,68.3562581248798,11.0843969896657));
#82402=CARTESIAN_POINT('Ctrl Pts',(90.6921776474382,68.2948,11.0416297237433));
#82403=CARTESIAN_POINT('',(90.5191409289644,68.2948,10.6705512834741));
#82404=CARTESIAN_POINT('Origin',(88.011,68.2948,12.066));
#82405=CARTESIAN_POINT('',(90.392743065488,68.4148,10.6909));
#82406=CARTESIAN_POINT('Ctrl Pts',(90.5191409289644,68.2948,10.6705512834741));
#82407=CARTESIAN_POINT('Ctrl Pts',(90.4545926498816,68.3562581248815,10.6809428723599));
#82408=CARTESIAN_POINT('Ctrl Pts',(90.392743065488,68.4148,10.6909));
#82409=CARTESIAN_POINT('',(90.473564502672,68.2948,10.5916105975083));
#82410=CARTESIAN_POINT('Ctrl Pts',(90.392743065488,68.4148,10.6909));
#82411=CARTESIAN_POINT('Ctrl Pts',(90.4322909831703,68.3562581248808,10.642315252521));
#82412=CARTESIAN_POINT('Ctrl Pts',(90.473564502672,68.2948,10.5916105975082));
#82413=CARTESIAN_POINT('',(90.238719505839,68.2948,10.2562171833879));
#82414=CARTESIAN_POINT('Origin',(88.011,68.2948,12.066));
#82415=CARTESIAN_POINT('',(90.1177754274658,68.4148,10.2982055158401));
#82416=CARTESIAN_POINT('Ctrl Pts',(90.238719505839,68.2948,10.2562171833879));
#82417=CARTESIAN_POINT('Ctrl Pts',(90.1769563406299,68.3562581248795,10.2776595917222));
#82418=CARTESIAN_POINT('Ctrl Pts',(90.1177754274658,68.4148,10.2982055158401));
#82419=CARTESIAN_POINT('',(90.1801275816099,68.2948,10.1863900471908));
#82420=CARTESIAN_POINT('Ctrl Pts',(90.1177754274658,68.4148,10.2982055158401));
#82421=CARTESIAN_POINT('Ctrl Pts',(90.1482858705526,68.3562581248811,10.2434914560088));
#82422=CARTESIAN_POINT('Ctrl Pts',(90.1801275816099,68.2948,10.1863900471908));
#82423=CARTESIAN_POINT('',(89.8906099528092,68.2948,9.89687241839011));
#82424=CARTESIAN_POINT('Origin',(88.011,68.2948,12.066));
#82425=CARTESIAN_POINT('',(89.7787944841599,68.4148,9.95922457253419));
#82426=CARTESIAN_POINT('Ctrl Pts',(89.8906099528092,68.2948,9.8968724183901));
#82427=CARTESIAN_POINT('Ctrl Pts',(89.8335085439914,68.3562581248809,9.92871412944728));
#82428=CARTESIAN_POINT('Ctrl Pts',(89.7787944841599,68.4148,9.95922457253419));
#82429=CARTESIAN_POINT('',(89.8207828166121,68.2948,9.838280494161));
#82430=CARTESIAN_POINT('Ctrl Pts',(89.7787944841599,68.4148,9.95922457253419));
#82431=CARTESIAN_POINT('Ctrl Pts',(89.7993404082777,68.3562581248795,9.9000436593701));
#82432=CARTESIAN_POINT('Ctrl Pts',(89.8207828166121,68.2948,9.83828049416098));
#82433=CARTESIAN_POINT('',(89.4853894024917,68.2948,9.60343549732802));
#82434=CARTESIAN_POINT('Origin',(88.011,68.2948,12.066));
#82435=CARTESIAN_POINT('',(89.3861,68.4148,9.68425693451204));
#82436=CARTESIAN_POINT('Ctrl Pts',(89.4853894024917,68.2948,9.60343549732801));
#82437=CARTESIAN_POINT('Ctrl Pts',(89.4346847474794,68.3562581248803,9.64470901682936));
#82438=CARTESIAN_POINT('Ctrl Pts',(89.3861,68.4148,9.68425693451204));
#82439=CARTESIAN_POINT('',(89.4064487165258,68.2948,9.55785907103561));
#82440=CARTESIAN_POINT('Ctrl Pts',(89.3861,68.4148,9.68425693451204));
#82441=CARTESIAN_POINT('Ctrl Pts',(89.3960571276404,68.3562581248794,9.62240735011616));
#82442=CARTESIAN_POINT('Ctrl Pts',(89.4064487165259,68.2948,9.5578590710356));
#82443=CARTESIAN_POINT('',(89.0353702762566,68.2948,9.38482235256186));
#82444=CARTESIAN_POINT('Origin',(88.011,68.2948,12.066));
#82445=CARTESIAN_POINT('',(88.9516237981742,68.4148,9.48165735431459));
#82446=CARTESIAN_POINT('Ctrl Pts',(89.0353702762567,68.2948,9.38482235256184));
#82447=CARTESIAN_POINT('Ctrl Pts',(88.9926030103341,68.3562581248802,9.4342736055029));
#82448=CARTESIAN_POINT('Ctrl Pts',(88.9516237981742,68.4148,9.48165735431459));
#82449=CARTESIAN_POINT('',(88.9497146133191,68.2948,9.35364624085626));
#82450=CARTESIAN_POINT('Ctrl Pts',(88.9516237981742,68.4148,9.48165735431459));
#82451=CARTESIAN_POINT('Ctrl Pts',(88.9506895870525,68.3562581248798,9.41901836701178));
#82452=CARTESIAN_POINT('Ctrl Pts',(88.9497146133191,68.2948,9.35364624085623));
#82453=CARTESIAN_POINT('',(88.5542261775338,68.2948,9.24767543387175));
#82454=CARTESIAN_POINT('Origin',(88.011,68.2948,12.066));
#82455=CARTESIAN_POINT('',(88.4885672182196,68.4148,9.35758171766581));
#82456=CARTESIAN_POINT('Ctrl Pts',(88.5542261775338,68.2948,9.24767543387173));
#82457=CARTESIAN_POINT('Ctrl Pts',(88.5206957624345,68.3562581248806,9.30380186895581));
#82458=CARTESIAN_POINT('Ctrl Pts',(88.4885672182196,68.4148,9.35758171766581));
#82459=CARTESIAN_POINT('',(88.4644581415991,68.2948,9.23184690713126));
#82460=CARTESIAN_POINT('Ctrl Pts',(88.4885672182196,68.4148,9.35758171766581));
#82461=CARTESIAN_POINT('Ctrl Pts',(88.4767700538679,68.3562581248799,9.29605658138816));
#82462=CARTESIAN_POINT('Ctrl Pts',(88.4644581415991,68.2948,9.23184690713123));
#82463=CARTESIAN_POINT('',(88.0565764262924,68.2948,9.19616188098241));
#82464=CARTESIAN_POINT('Origin',(88.011,68.2948,12.066));
#82465=CARTESIAN_POINT('',(88.011,68.4148,9.3158));
#82466=CARTESIAN_POINT('Ctrl Pts',(88.0565764262924,68.2948,9.19616188098239));
#82467=CARTESIAN_POINT('Ctrl Pts',(88.0333016667122,68.3562581248804,9.25725812488037));
#82468=CARTESIAN_POINT('Ctrl Pts',(88.011,68.4148,9.3158));
#82469=CARTESIAN_POINT('',(87.9654235737076,68.2948,9.19616188098241));
#82470=CARTESIAN_POINT('Ctrl Pts',(88.011,68.4148,9.3158));
#82471=CARTESIAN_POINT('Ctrl Pts',(87.9886983332877,68.3562581248803,9.2572581248803));
#82472=CARTESIAN_POINT('Ctrl Pts',(87.9654235737076,68.2948,9.19616188098239));
#82473=CARTESIAN_POINT('',(87.5575418584008,68.2948,9.23184690713126));
#82474=CARTESIAN_POINT('Origin',(88.011,68.2948,12.066));
#82475=CARTESIAN_POINT('',(87.5334327817804,68.4148,9.35758171766581));
#82476=CARTESIAN_POINT('Ctrl Pts',(87.5575418584008,68.2948,9.23184690713124));
#82477=CARTESIAN_POINT('Ctrl Pts',(87.545229946132,68.3562581248804,9.29605658138868));
#82478=CARTESIAN_POINT('Ctrl Pts',(87.5334327817804,68.4148,9.35758171766581));
#82479=CARTESIAN_POINT('',(87.4677738224661,68.2948,9.24767543387176));
#82480=CARTESIAN_POINT('Ctrl Pts',(87.5334327817804,68.4148,9.35758171766581));
#82481=CARTESIAN_POINT('Ctrl Pts',(87.5013042375654,68.3562581248805,9.30380186895576));
#82482=CARTESIAN_POINT('Ctrl Pts',(87.4677738224661,68.2948,9.24767543387173));
#82483=CARTESIAN_POINT('',(87.0722853866809,68.2948,9.35364624085626));
#82484=CARTESIAN_POINT('Origin',(88.011,68.2948,12.066));
#82485=CARTESIAN_POINT('',(87.0703762018258,68.4148,9.48165735431459));
#82486=CARTESIAN_POINT('Ctrl Pts',(87.0722853866809,68.2948,9.35364624085623));
#82487=CARTESIAN_POINT('Ctrl Pts',(87.0713104129475,68.3562581248812,9.41901836701324));
#82488=CARTESIAN_POINT('Ctrl Pts',(87.0703762018258,68.4148,9.48165735431459));
#82489=CARTESIAN_POINT('',(86.9866297237434,68.2948,9.38482235256186));
#82490=CARTESIAN_POINT('Ctrl Pts',(87.0703762018257,68.4148,9.48165735431459));
#82491=CARTESIAN_POINT('Ctrl Pts',(87.0293969896666,68.3562581248812,9.43427360550364));
#82492=CARTESIAN_POINT('Ctrl Pts',(86.9866297237434,68.2948,9.38482235256185));
#82493=CARTESIAN_POINT('',(86.6155512834741,68.2948,9.55785907103562));
#82494=CARTESIAN_POINT('Origin',(88.011,68.2948,12.066));
#82495=CARTESIAN_POINT('',(86.6359,68.4148,9.68425693451204));
#82496=CARTESIAN_POINT('Ctrl Pts',(86.6155512834741,68.2948,9.55785907103559));
#82497=CARTESIAN_POINT('Ctrl Pts',(86.6259428723597,68.3562581248802,9.62240735011689));
#82498=CARTESIAN_POINT('Ctrl Pts',(86.6359,68.4148,9.68425693451204));
#82499=CARTESIAN_POINT('',(86.5366105975083,68.2948,9.60343549732803));
#82500=CARTESIAN_POINT('Ctrl Pts',(86.6359,68.4148,9.68425693451204));
#82501=CARTESIAN_POINT('Ctrl Pts',(86.587315252521,68.3562581248808,9.64470901682966));
#82502=CARTESIAN_POINT('Ctrl Pts',(86.5366105975082,68.2948,9.60343549732803));
#82503=CARTESIAN_POINT('',(86.2012171833879,68.2948,9.838280494161));
#82504=CARTESIAN_POINT('Origin',(88.011,68.2948,12.066));
#82505=CARTESIAN_POINT('',(86.2432055158401,68.4148,9.95922457253419));
#82506=CARTESIAN_POINT('Ctrl Pts',(86.2012171833879,68.2948,9.83828049416098));
#82507=CARTESIAN_POINT('Ctrl Pts',(86.2226595917224,68.35625812488,9.90004365937064));
#82508=CARTESIAN_POINT('Ctrl Pts',(86.2432055158401,68.4148,9.95922457253419));
#82509=CARTESIAN_POINT('',(86.1313900471908,68.2948,9.89687241839012));
#82510=CARTESIAN_POINT('Ctrl Pts',(86.2432055158401,68.4148,9.95922457253419));
#82511=CARTESIAN_POINT('Ctrl Pts',(86.1884914560078,68.35625812488,9.92871412944681));
#82512=CARTESIAN_POINT('Ctrl Pts',(86.1313900471908,68.2948,9.89687241839012));
#82513=CARTESIAN_POINT('',(85.8418724183901,68.2948,10.1863900471908));
#82514=CARTESIAN_POINT('Origin',(88.011,68.2948,12.066));
#82515=CARTESIAN_POINT('',(85.9042245725342,68.4148,10.2982055158401));
#82516=CARTESIAN_POINT('Ctrl Pts',(85.8418724183901,68.2948,10.1863900471908));
#82517=CARTESIAN_POINT('Ctrl Pts',(85.8737141294469,68.3562581248803,10.2434914560081));
#82518=CARTESIAN_POINT('Ctrl Pts',(85.9042245725342,68.4148,10.2982055158401));
#82519=CARTESIAN_POINT('',(85.783280494161,68.2948,10.2562171833879));
#82520=CARTESIAN_POINT('Ctrl Pts',(85.9042245725342,68.4148,10.2982055158401));
#82521=CARTESIAN_POINT('Ctrl Pts',(85.8450436593716,68.3562581248809,10.2776595917227));
#82522=CARTESIAN_POINT('Ctrl Pts',(85.783280494161,68.2948,10.2562171833879));
#82523=CARTESIAN_POINT('',(85.548435497328,68.2948,10.5916105975083));
#82524=CARTESIAN_POINT('Origin',(88.011,68.2948,12.066));
#82525=CARTESIAN_POINT('',(85.629256934512,68.4148,10.6909));
#82526=CARTESIAN_POINT('Ctrl Pts',(85.548435497328,68.2948,10.5916105975083));
#82527=CARTESIAN_POINT('Ctrl Pts',(85.5897090168295,68.3562581248805,10.6423152525208));
#82528=CARTESIAN_POINT('Ctrl Pts',(85.629256934512,68.4148,10.6909));
#82529=CARTESIAN_POINT('',(85.5028590710356,68.2948,10.6705512834741));
#82530=CARTESIAN_POINT('Ctrl Pts',(85.629256934512,68.4148,10.6909));
#82531=CARTESIAN_POINT('Ctrl Pts',(85.5674073501174,68.3562581248806,10.6809428723598));
#82532=CARTESIAN_POINT('Ctrl Pts',(85.5028590710356,68.2948,10.6705512834741));
#82533=CARTESIAN_POINT('',(85.3298223525619,68.2948,11.0416297237433));
#82534=CARTESIAN_POINT('Origin',(88.011,68.2948,12.066));
#82535=CARTESIAN_POINT('',(85.4266573543146,68.4148,11.1253762018257));
#82536=CARTESIAN_POINT('Ctrl Pts',(85.3298223525618,68.2948,11.0416297237433));
#82537=CARTESIAN_POINT('Ctrl Pts',(85.3792736055027,68.35625812488,11.0843969896658));
#82538=CARTESIAN_POINT('Ctrl Pts',(85.4266573543146,68.4148,11.1253762018257));
#82539=CARTESIAN_POINT('',(85.2986462408563,68.2948,11.1272853866809));
#82540=CARTESIAN_POINT('Ctrl Pts',(85.4266573543146,68.4148,11.1253762018257));
#82541=CARTESIAN_POINT('Ctrl Pts',(85.3640183670115,68.3562581248796,11.1263104129475));
#82542=CARTESIAN_POINT('Ctrl Pts',(85.2986462408562,68.2948,11.1272853866809));
#82543=CARTESIAN_POINT('',(85.1926754338717,68.2948,11.5227738224661));
#82544=CARTESIAN_POINT('Origin',(88.011,68.2948,12.066));
#82545=CARTESIAN_POINT('',(85.3025817176658,68.4148,11.5884327817804));
#82546=CARTESIAN_POINT('Ctrl Pts',(85.1926754338717,68.2948,11.5227738224661));
#82547=CARTESIAN_POINT('Ctrl Pts',(85.2488018689556,68.3562581248803,11.5563042375653));
#82548=CARTESIAN_POINT('Ctrl Pts',(85.3025817176658,68.4148,11.5884327817804));
#82549=CARTESIAN_POINT('',(85.1768469071313,68.2948,11.6125418584009));
#82550=CARTESIAN_POINT('Ctrl Pts',(85.3025817176658,68.4148,11.5884327817804));
#82551=CARTESIAN_POINT('Ctrl Pts',(85.2410565813872,68.356258124879,11.6002299461323));
#82552=CARTESIAN_POINT('Ctrl Pts',(85.1768469071312,68.2948,11.6125418584009));
#82553=CARTESIAN_POINT('',(85.1411618809824,68.2948,12.0204235737076));
#82554=CARTESIAN_POINT('Origin',(88.011,68.2948,12.066));
#82555=CARTESIAN_POINT('Ctrl Pts',(85.1411618809824,68.2948,12.0204235737076));
#82556=CARTESIAN_POINT('Ctrl Pts',(85.2022581248785,68.3562581248785,12.0436983332871));
#82557=CARTESIAN_POINT('Ctrl Pts',(85.2608,68.4148,12.066));
#82558=CARTESIAN_POINT('',(85.4408,68.5948,12.066));
#82559=CARTESIAN_POINT('',(85.2908,68.4448,12.066));
#82560=CARTESIAN_POINT('Origin',(88.011,68.5948,12.066));
#82561=CARTESIAN_POINT('Origin',(91.0447367693476,68.5948,11.1320785609547));
#82562=CARTESIAN_POINT('',(90.7233537591437,65.6896,11.1272853866809));
#82563=CARTESIAN_POINT('',(90.7233537591437,65.0896,11.1272853866809));
#82564=CARTESIAN_POINT('',(90.5953426456854,65.6896,11.1253762018257));
#82565=CARTESIAN_POINT('',(91.0447367693476,65.6896,11.1320785609547));
#82566=CARTESIAN_POINT('',(90.5953426456854,68.5948,11.1253762018257));
#82567=CARTESIAN_POINT('Origin',(90.5953426456854,68.5948,11.1253762018257));
#82568=CARTESIAN_POINT('',(90.6921776474381,65.6896,11.0416297237434));
#82569=CARTESIAN_POINT('',(90.6921776474381,65.0896,11.0416297237434));
#82570=CARTESIAN_POINT('',(90.5953426456854,65.6896,11.1253762018257));
#82571=CARTESIAN_POINT('Origin',(90.7926780960505,65.6896,11.0535519717273));
#82572=CARTESIAN_POINT('Origin',(88.011,65.6896,12.066));
#82573=CARTESIAN_POINT('Origin',(90.8364737350774,68.5948,10.6194640646055));
#82574=CARTESIAN_POINT('',(90.5191409289644,65.6896,10.6705512834741));
#82575=CARTESIAN_POINT('',(90.5191409289644,65.0896,10.6705512834741));
#82576=CARTESIAN_POINT('',(90.392743065488,65.6896,10.6909));
#82577=CARTESIAN_POINT('',(90.8364737350774,65.6896,10.6194640646055));
#82578=CARTESIAN_POINT('',(90.392743065488,68.5948,10.6909));
#82579=CARTESIAN_POINT('Origin',(90.392743065488,68.5948,10.6909));
#82580=CARTESIAN_POINT('',(90.473564502672,65.6896,10.5916105975083));
#82581=CARTESIAN_POINT('',(90.473564502672,65.0896,10.5916105975083));
#82582=CARTESIAN_POINT('',(90.392743065488,65.6896,10.6909));
#82583=CARTESIAN_POINT('Origin',(90.5746084002827,65.6896,10.5859));
#82584=CARTESIAN_POINT('Origin',(88.011,65.6896,12.066));
#82585=CARTESIAN_POINT('Origin',(90.5423601111256,68.5948,10.1508018306708));
#82586=CARTESIAN_POINT('',(90.238719505839,65.6896,10.2562171833879));
#82587=CARTESIAN_POINT('',(90.238719505839,65.0896,10.2562171833879));
#82588=CARTESIAN_POINT('',(90.1177754274658,65.6896,10.2982055158401));
#82589=CARTESIAN_POINT('',(90.5423601111256,65.6896,10.1508018306708));
#82590=CARTESIAN_POINT('',(90.1177754274658,68.5948,10.2982055158401));
#82591=CARTESIAN_POINT('Origin',(90.1177754274658,68.5948,10.2982055158401));
#82592=CARTESIAN_POINT('',(90.1801275816099,65.6896,10.1863900471908));
#82593=CARTESIAN_POINT('',(90.1801275816099,65.0896,10.1863900471908));
#82594=CARTESIAN_POINT('',(90.1177754274658,65.6896,10.2982055158401));
#82595=CARTESIAN_POINT('Origin',(90.2786447605208,65.6896,10.1632201178059));
#82596=CARTESIAN_POINT('Origin',(88.011,65.6896,12.066));
#82597=CARTESIAN_POINT('Origin',(90.1713323911273,68.5948,9.74033192397407));
#82598=CARTESIAN_POINT('',(89.8906099528092,65.6896,9.89687241839011));
#82599=CARTESIAN_POINT('',(89.8906099528092,65.0896,9.89687241839011));
#82600=CARTESIAN_POINT('',(89.7787944841599,65.6896,9.95922457253418));
#82601=CARTESIAN_POINT('',(90.1713323911273,65.6896,9.74033192397407));
#82602=CARTESIAN_POINT('',(89.7787944841599,68.5948,9.95922457253418));
#82603=CARTESIAN_POINT('Origin',(89.7787944841599,68.5948,9.95922457253418));
#82604=CARTESIAN_POINT('',(89.8207828166121,65.6896,9.838280494161));
#82605=CARTESIAN_POINT('',(89.8207828166121,65.0896,9.838280494161));
#82606=CARTESIAN_POINT('',(89.7787944841599,65.6896,9.95922457253418));
#82607=CARTESIAN_POINT('Origin',(89.9137798821941,65.6896,9.79835523947919));
#82608=CARTESIAN_POINT('Origin',(88.011,65.6896,12.066));
#82609=CARTESIAN_POINT('Origin',(89.7346640646055,68.5948,9.40052626492258));
#82610=CARTESIAN_POINT('',(89.4853894024917,65.6896,9.60343549732802));
#82611=CARTESIAN_POINT('',(89.4853894024917,65.0896,9.60343549732802));
#82612=CARTESIAN_POINT('',(89.3861,65.6896,9.68425693451204));
#82613=CARTESIAN_POINT('',(89.7346640646055,65.6896,9.40052626492258));
#82614=CARTESIAN_POINT('',(89.3861,68.5948,9.68425693451204));
#82615=CARTESIAN_POINT('Origin',(89.3861,68.5948,9.68425693451204));
#82616=CARTESIAN_POINT('',(89.4064487165258,65.6896,9.55785907103561));
#82617=CARTESIAN_POINT('',(89.4064487165258,65.0896,9.55785907103561));
#82618=CARTESIAN_POINT('',(89.3861,65.6896,9.68425693451204));
#82619=CARTESIAN_POINT('Origin',(89.4911,65.6896,9.5023915997173));
#82620=CARTESIAN_POINT('Origin',(88.011,65.6896,12.066));
#82621=CARTESIAN_POINT('Origin',(89.2456230776968,68.5948,9.14170967651661));
#82622=CARTESIAN_POINT('',(89.0353702762566,65.6896,9.38482235256186));
#82623=CARTESIAN_POINT('',(89.0353702762566,65.0896,9.38482235256186));
#82624=CARTESIAN_POINT('',(88.9516237981742,65.6896,9.48165735431459));
#82625=CARTESIAN_POINT('',(89.2456230776968,65.6896,9.14170967651661));
#82626=CARTESIAN_POINT('',(88.9516237981742,68.5948,9.48165735431459));
#82627=CARTESIAN_POINT('Origin',(88.9516237981742,68.5948,9.48165735431459));
#82628=CARTESIAN_POINT('',(88.9497146133191,65.6896,9.35364624085626));
#82629=CARTESIAN_POINT('',(88.9497146133191,65.0896,9.35364624085626));
#82630=CARTESIAN_POINT('',(88.9516237981742,65.6896,9.48165735431459));
#82631=CARTESIAN_POINT('Origin',(89.0234480282727,65.6896,9.28432190394954));
#82632=CARTESIAN_POINT('Origin',(88.011,65.6896,12.066));
#82633=CARTESIAN_POINT('Origin',(88.7190686933216,68.5948,8.9717461698274));
#82634=CARTESIAN_POINT('',(88.5542261775338,65.6896,9.24767543387175));
#82635=CARTESIAN_POINT('',(88.5542261775338,65.0896,9.24767543387175));
#82636=CARTESIAN_POINT('',(88.4885672182196,65.6896,9.35758171766581));
#82637=CARTESIAN_POINT('',(88.7190686933216,65.6896,8.9717461698274));
#82638=CARTESIAN_POINT('',(88.4885672182196,68.5948,9.35758171766581));
#82639=CARTESIAN_POINT('Origin',(88.4885672182196,68.5948,9.35758171766581));
#82640=CARTESIAN_POINT('',(88.4644581415991,65.6896,9.23184690713126));
#82641=CARTESIAN_POINT('',(88.4644581415991,65.0896,9.23184690713126));
#82642=CARTESIAN_POINT('',(88.4885672182196,65.6896,9.35758171766581));
#82643=CARTESIAN_POINT('Origin',(88.5250333355296,65.6896,9.15077208953324));
#82644=CARTESIAN_POINT('Origin',(88.011,65.6896,12.066));
#82645=CARTESIAN_POINT('Origin',(88.171,68.5948,8.8958));
#82646=CARTESIAN_POINT('',(88.0565764262924,65.6896,9.19616188098241));
#82647=CARTESIAN_POINT('',(88.0565764262924,65.0896,9.19616188098241));
#82648=CARTESIAN_POINT('',(88.011,65.6896,9.3158));
#82649=CARTESIAN_POINT('',(88.171,65.6896,8.8958));
#82650=CARTESIAN_POINT('',(88.011,68.5948,9.3158));
#82651=CARTESIAN_POINT('Origin',(88.011,68.5948,9.3158));
#82652=CARTESIAN_POINT('',(87.9654235737076,65.6896,9.19616188098241));
#82653=CARTESIAN_POINT('',(87.9654235737076,65.0896,9.19616188098241));
#82654=CARTESIAN_POINT('',(88.011,65.6896,9.3158));
#82655=CARTESIAN_POINT('Origin',(88.011,65.6896,9.1058));
#82656=CARTESIAN_POINT('Origin',(88.011,65.6896,12.066));
#82657=CARTESIAN_POINT('Origin',(87.6180697876423,68.5948,8.91617875297397));
#82658=CARTESIAN_POINT('',(87.5575418584008,65.6896,9.23184690713126));
#82659=CARTESIAN_POINT('',(87.5575418584008,65.0896,9.23184690713126));
#82660=CARTESIAN_POINT('',(87.5334327817804,65.6896,9.35758171766581));
#82661=CARTESIAN_POINT('',(87.6180697876423,65.6896,8.91617875297397));
#82662=CARTESIAN_POINT('',(87.5334327817804,68.5948,9.35758171766581));
#82663=CARTESIAN_POINT('Origin',(87.5334327817804,68.5948,9.35758171766581));
#82664=CARTESIAN_POINT('',(87.4677738224661,65.6896,9.24767543387176));
#82665=CARTESIAN_POINT('',(87.4677738224661,65.0896,9.24767543387176));
#82666=CARTESIAN_POINT('',(87.5334327817804,65.6896,9.35758171766581));
#82667=CARTESIAN_POINT('Origin',(87.4969666644703,65.6896,9.15077208953324));
#82668=CARTESIAN_POINT('Origin',(88.011,65.6896,12.066));
#82669=CARTESIAN_POINT('Origin',(87.0770785609547,68.5948,9.03226323065242));
#82670=CARTESIAN_POINT('',(87.0722853866809,65.6896,9.35364624085626));
#82671=CARTESIAN_POINT('',(87.0722853866809,65.0896,9.35364624085626));
#82672=CARTESIAN_POINT('',(87.0703762018258,65.6896,9.48165735431459));
#82673=CARTESIAN_POINT('',(87.0770785609547,65.6896,9.03226323065242));
#82674=CARTESIAN_POINT('',(87.0703762018258,68.5948,9.48165735431459));
#82675=CARTESIAN_POINT('Origin',(87.0703762018258,68.5948,9.48165735431459));
#82676=CARTESIAN_POINT('',(86.9866297237434,65.6896,9.38482235256186));
#82677=CARTESIAN_POINT('',(86.9866297237434,65.0896,9.38482235256186));
#82678=CARTESIAN_POINT('',(87.0703762018258,65.6896,9.48165735431459));
#82679=CARTESIAN_POINT('Origin',(86.9985519717274,65.6896,9.28432190394956));
#82680=CARTESIAN_POINT('Origin',(88.011,65.6896,12.066));
#82681=CARTESIAN_POINT('Origin',(86.5644640646055,68.5948,9.24052626492257));
#82682=CARTESIAN_POINT('',(86.6155512834741,65.6896,9.55785907103562));
#82683=CARTESIAN_POINT('',(86.6155512834741,65.0896,9.55785907103562));
#82684=CARTESIAN_POINT('',(86.6359,65.6896,9.68425693451204));
#82685=CARTESIAN_POINT('',(86.5644640646055,65.6896,9.24052626492257));
#82686=CARTESIAN_POINT('',(86.6359,68.5948,9.68425693451204));
#82687=CARTESIAN_POINT('Origin',(86.6359,68.5948,9.68425693451204));
#82688=CARTESIAN_POINT('',(86.5366105975083,65.6896,9.60343549732803));
#82689=CARTESIAN_POINT('',(86.5366105975083,65.0896,9.60343549732803));
#82690=CARTESIAN_POINT('',(86.6359,65.6896,9.68425693451204));
#82691=CARTESIAN_POINT('Origin',(86.5309,65.6896,9.5023915997173));
#82692=CARTESIAN_POINT('Origin',(88.011,65.6896,12.066));
#82693=CARTESIAN_POINT('Origin',(86.0958018306708,68.5948,9.53463988887438));
#82694=CARTESIAN_POINT('',(86.2012171833879,65.6896,9.838280494161));
#82695=CARTESIAN_POINT('',(86.2012171833879,65.0896,9.838280494161));
#82696=CARTESIAN_POINT('',(86.2432055158401,65.6896,9.95922457253419));
#82697=CARTESIAN_POINT('',(86.0958018306708,65.6896,9.53463988887438));
#82698=CARTESIAN_POINT('',(86.2432055158401,68.5948,9.95922457253419));
#82699=CARTESIAN_POINT('Origin',(86.2432055158401,68.5948,9.95922457253419));
#82700=CARTESIAN_POINT('',(86.1313900471908,65.6896,9.89687241839012));
#82701=CARTESIAN_POINT('',(86.1313900471908,65.0896,9.89687241839012));
#82702=CARTESIAN_POINT('',(86.2432055158401,65.6896,9.95922457253419));
#82703=CARTESIAN_POINT('Origin',(86.1082201178059,65.6896,9.7983552394792));
#82704=CARTESIAN_POINT('Origin',(88.011,65.6896,12.066));
#82705=CARTESIAN_POINT('Origin',(85.6853319239741,68.5948,9.90566760887269));
#82706=CARTESIAN_POINT('',(85.8418724183901,65.6896,10.1863900471908));
#82707=CARTESIAN_POINT('',(85.8418724183901,65.0896,10.1863900471908));
#82708=CARTESIAN_POINT('',(85.9042245725342,65.6896,10.2982055158401));
#82709=CARTESIAN_POINT('',(85.6853319239741,65.6896,9.90566760887269));
#82710=CARTESIAN_POINT('',(85.9042245725342,68.5948,10.2982055158401));
#82711=CARTESIAN_POINT('Origin',(85.9042245725342,68.5948,10.2982055158401));
#82712=CARTESIAN_POINT('',(85.783280494161,65.6896,10.2562171833879));
#82713=CARTESIAN_POINT('',(85.783280494161,65.0896,10.2562171833879));
#82714=CARTESIAN_POINT('',(85.9042245725342,65.6896,10.2982055158401));
#82715=CARTESIAN_POINT('Origin',(85.7433552394792,65.6896,10.1632201178059));
#82716=CARTESIAN_POINT('Origin',(88.011,65.6896,12.066));
#82717=CARTESIAN_POINT('Origin',(85.3455262649226,68.5948,10.3423359353945));
#82718=CARTESIAN_POINT('',(85.548435497328,65.6896,10.5916105975083));
#82719=CARTESIAN_POINT('',(85.548435497328,65.0896,10.5916105975083));
#82720=CARTESIAN_POINT('',(85.629256934512,65.6896,10.6909));
#82721=CARTESIAN_POINT('',(85.3455262649226,65.6896,10.3423359353945));
#82722=CARTESIAN_POINT('',(85.629256934512,68.5948,10.6909));
#82723=CARTESIAN_POINT('Origin',(85.629256934512,68.5948,10.6909));
#82724=CARTESIAN_POINT('',(85.5028590710356,65.6896,10.6705512834741));
#82725=CARTESIAN_POINT('',(85.5028590710356,65.0896,10.6705512834741));
#82726=CARTESIAN_POINT('',(85.629256934512,65.6896,10.6909));
#82727=CARTESIAN_POINT('Origin',(85.4473915997173,65.6896,10.5859));
#82728=CARTESIAN_POINT('Origin',(88.011,65.6896,12.066));
#82729=CARTESIAN_POINT('Origin',(85.0867096765166,68.5948,10.8313769223032));
#82730=CARTESIAN_POINT('',(85.3298223525619,65.6896,11.0416297237433));
#82731=CARTESIAN_POINT('',(85.3298223525619,65.0896,11.0416297237433));
#82732=CARTESIAN_POINT('',(85.4266573543146,65.6896,11.1253762018257));
#82733=CARTESIAN_POINT('',(85.0867096765166,65.6896,10.8313769223032));
#82734=CARTESIAN_POINT('',(85.4266573543146,68.5948,11.1253762018257));
#82735=CARTESIAN_POINT('Origin',(85.4266573543146,68.5948,11.1253762018257));
#82736=CARTESIAN_POINT('',(85.2986462408563,65.6896,11.1272853866809));
#82737=CARTESIAN_POINT('',(85.2986462408563,65.0896,11.1272853866809));
#82738=CARTESIAN_POINT('',(85.4266573543146,65.6896,11.1253762018257));
#82739=CARTESIAN_POINT('Origin',(85.2293219039495,65.6896,11.0535519717273));
#82740=CARTESIAN_POINT('Origin',(88.011,65.6896,12.066));
#82741=CARTESIAN_POINT('Origin',(84.9167461698274,68.5948,11.3579313066783));
#82742=CARTESIAN_POINT('',(85.1926754338717,65.6896,11.5227738224661));
#82743=CARTESIAN_POINT('',(85.1926754338717,65.0896,11.5227738224661));
#82744=CARTESIAN_POINT('',(85.3025817176658,65.6896,11.5884327817804));
#82745=CARTESIAN_POINT('',(84.9167461698274,65.6896,11.3579313066783));
#82746=CARTESIAN_POINT('',(85.3025817176658,68.5948,11.5884327817804));
#82747=CARTESIAN_POINT('Origin',(85.3025817176658,68.5948,11.5884327817804));
#82748=CARTESIAN_POINT('',(85.1768469071313,65.6896,11.6125418584009));
#82749=CARTESIAN_POINT('',(85.1768469071313,65.0896,11.6125418584009));
#82750=CARTESIAN_POINT('',(85.3025817176658,65.6896,11.5884327817804));
#82751=CARTESIAN_POINT('Origin',(85.0957720895332,65.6896,11.5519666644703));
#82752=CARTESIAN_POINT('Origin',(88.011,65.6896,12.066));
#82753=CARTESIAN_POINT('Origin',(84.8408,68.5948,11.906));
#82754=CARTESIAN_POINT('',(85.1411618809824,65.6896,12.0204235737076));
#82755=CARTESIAN_POINT('',(85.1411618809824,65.0896,12.0204235737076));
#82756=CARTESIAN_POINT('',(85.2608,65.6896,12.066));
#82757=CARTESIAN_POINT('',(84.8408,65.6896,11.906));
#82758=CARTESIAN_POINT('',(85.2608,68.5948,12.066));
#82759=CARTESIAN_POINT('Origin',(85.2608,68.5948,12.066));
#82760=CARTESIAN_POINT('',(85.1411618809824,65.6896,12.1115764262924));
#82761=CARTESIAN_POINT('',(85.1411618809824,65.0896,12.1115764262924));
#82762=CARTESIAN_POINT('',(85.2608,65.6896,12.066));
#82763=CARTESIAN_POINT('Origin',(85.0508,65.6896,12.066));
#82764=CARTESIAN_POINT('',(85.1408,65.6896,12.066));
#82765=CARTESIAN_POINT('Origin',(88.011,65.6896,12.066));
#82766=CARTESIAN_POINT('Origin',(88.011,65.6896,12.066));
#82767=CARTESIAN_POINT('Origin',(84.861178752974,68.5948,12.4589302123577));
#82768=CARTESIAN_POINT('',(85.1768469071313,65.6896,12.5194581415991));
#82769=CARTESIAN_POINT('',(85.1768469071313,65.0896,12.5194581415991));
#82770=CARTESIAN_POINT('',(85.3025817176658,65.6896,12.5435672182196));
#82771=CARTESIAN_POINT('',(84.861178752974,65.6896,12.4589302123577));
#82772=CARTESIAN_POINT('',(85.3025817176658,68.5948,12.5435672182196));
#82773=CARTESIAN_POINT('Origin',(85.3025817176658,68.5948,12.5435672182196));
#82774=CARTESIAN_POINT('',(85.1926754338717,65.6896,12.6092261775339));
#82775=CARTESIAN_POINT('',(85.1926754338717,65.0896,12.6092261775339));
#82776=CARTESIAN_POINT('',(85.3025817176658,65.6896,12.5435672182196));
#82777=CARTESIAN_POINT('Origin',(85.0957720895333,65.6896,12.5800333355296));
#82778=CARTESIAN_POINT('Origin',(88.011,65.6896,12.066));
#82779=CARTESIAN_POINT('Origin',(84.9772632306524,68.5948,12.9999214390453));
#82780=CARTESIAN_POINT('',(85.2986462408562,65.6896,13.0047146133191));
#82781=CARTESIAN_POINT('',(85.2986462408562,65.0896,13.0047146133191));
#82782=CARTESIAN_POINT('',(85.4266573543146,65.6896,13.0066237981742));
#82783=CARTESIAN_POINT('',(84.9772632306524,65.6896,12.9999214390453));
#82784=CARTESIAN_POINT('',(85.4266573543146,68.5948,13.0066237981742));
#82785=CARTESIAN_POINT('Origin',(85.4266573543146,68.5948,13.0066237981742));
#82786=CARTESIAN_POINT('',(85.3298223525619,65.6896,13.0903702762566));
#82787=CARTESIAN_POINT('',(85.3298223525619,65.0896,13.0903702762566));
#82788=CARTESIAN_POINT('',(85.4266573543146,65.6896,13.0066237981742));
#82789=CARTESIAN_POINT('Origin',(85.2293219039496,65.6896,13.0784480282726));
#82790=CARTESIAN_POINT('Origin',(88.011,65.6896,12.066));
#82791=CARTESIAN_POINT('Origin',(85.1855262649226,68.5948,13.5125359353945));
#82792=CARTESIAN_POINT('',(85.5028590710356,65.6896,13.4614487165259));
#82793=CARTESIAN_POINT('',(85.5028590710356,65.0896,13.4614487165259));
#82794=CARTESIAN_POINT('',(85.629256934512,65.6896,13.4411));
#82795=CARTESIAN_POINT('',(85.1855262649226,65.6896,13.5125359353945));
#82796=CARTESIAN_POINT('',(85.629256934512,68.5948,13.4411));
#82797=CARTESIAN_POINT('Origin',(85.629256934512,68.5948,13.4411));
#82798=CARTESIAN_POINT('',(85.548435497328,65.6896,13.5403894024917));
#82799=CARTESIAN_POINT('',(85.548435497328,65.0896,13.5403894024917));
#82800=CARTESIAN_POINT('',(85.629256934512,65.6896,13.4411));
#82801=CARTESIAN_POINT('Origin',(85.4473915997173,65.6896,13.5461));
#82802=CARTESIAN_POINT('Origin',(88.011,65.6896,12.066));
#82803=CARTESIAN_POINT('Origin',(85.4796398888744,68.5948,13.9811981693292));
#82804=CARTESIAN_POINT('',(85.783280494161,65.6896,13.8757828166121));
#82805=CARTESIAN_POINT('',(85.783280494161,65.0896,13.8757828166121));
#82806=CARTESIAN_POINT('',(85.9042245725342,65.6896,13.8337944841599));
#82807=CARTESIAN_POINT('',(85.4796398888744,65.6896,13.9811981693292));
#82808=CARTESIAN_POINT('',(85.9042245725342,68.5948,13.8337944841599));
#82809=CARTESIAN_POINT('Origin',(85.9042245725342,68.5948,13.8337944841599));
#82810=CARTESIAN_POINT('',(85.8418724183901,65.6896,13.9456099528092));
#82811=CARTESIAN_POINT('',(85.8418724183901,65.0896,13.9456099528092));
#82812=CARTESIAN_POINT('',(85.9042245725342,65.6896,13.8337944841599));
#82813=CARTESIAN_POINT('Origin',(85.7433552394792,65.6896,13.9687798821941));
#82814=CARTESIAN_POINT('Origin',(88.011,65.6896,12.066));
#82815=CARTESIAN_POINT('Origin',(85.8506676088727,68.5948,14.3916680760259));
#82816=CARTESIAN_POINT('',(86.1313900471908,65.6896,14.2351275816099));
#82817=CARTESIAN_POINT('',(86.1313900471908,65.0896,14.2351275816099));
#82818=CARTESIAN_POINT('',(86.2432055158401,65.6896,14.1727754274658));
#82819=CARTESIAN_POINT('',(85.8506676088727,65.6896,14.3916680760259));
#82820=CARTESIAN_POINT('',(86.2432055158401,68.5948,14.1727754274658));
#82821=CARTESIAN_POINT('Origin',(86.2432055158401,68.5948,14.1727754274658));
#82822=CARTESIAN_POINT('',(86.2012171833879,65.6896,14.293719505839));
#82823=CARTESIAN_POINT('',(86.2012171833879,65.0896,14.293719505839));
#82824=CARTESIAN_POINT('',(86.2432055158401,65.6896,14.1727754274658));
#82825=CARTESIAN_POINT('Origin',(86.1082201178059,65.6896,14.3336447605208));
#82826=CARTESIAN_POINT('Origin',(88.011,65.6896,12.066));
#82827=CARTESIAN_POINT('Origin',(86.2873359353945,68.5948,14.7314737350774));
#82828=CARTESIAN_POINT('',(86.5366105975083,65.6896,14.528564502672));
#82829=CARTESIAN_POINT('',(86.5366105975083,65.0896,14.528564502672));
#82830=CARTESIAN_POINT('',(86.6359,65.6896,14.447743065488));
#82831=CARTESIAN_POINT('',(86.2873359353945,65.6896,14.7314737350774));
#82832=CARTESIAN_POINT('',(86.6359,68.5948,14.447743065488));
#82833=CARTESIAN_POINT('Origin',(86.6359,68.5948,14.447743065488));
#82834=CARTESIAN_POINT('',(86.6155512834742,65.6896,14.5741409289644));
#82835=CARTESIAN_POINT('',(86.6155512834742,65.0896,14.5741409289644));
#82836=CARTESIAN_POINT('',(86.6359,65.6896,14.447743065488));
#82837=CARTESIAN_POINT('Origin',(86.5309,65.6896,14.6296084002827));
#82838=CARTESIAN_POINT('Origin',(88.011,65.6896,12.066));
#82839=CARTESIAN_POINT('Origin',(86.7763769223032,68.5948,14.9902903234834));
#82840=CARTESIAN_POINT('',(86.9866297237434,65.6896,14.7471776474381));
#82841=CARTESIAN_POINT('',(86.9866297237434,65.0896,14.7471776474381));
#82842=CARTESIAN_POINT('',(87.0703762018258,65.6896,14.6503426456854));
#82843=CARTESIAN_POINT('',(86.7763769223032,65.6896,14.9902903234834));
#82844=CARTESIAN_POINT('',(87.0703762018258,68.5948,14.6503426456854));
#82845=CARTESIAN_POINT('Origin',(87.0703762018258,68.5948,14.6503426456854));
#82846=CARTESIAN_POINT('',(87.0722853866809,65.6896,14.7783537591437));
#82847=CARTESIAN_POINT('',(87.0722853866809,65.0896,14.7783537591437));
#82848=CARTESIAN_POINT('',(87.0703762018258,65.6896,14.6503426456854));
#82849=CARTESIAN_POINT('Origin',(86.9985519717274,65.6896,14.8476780960505));
#82850=CARTESIAN_POINT('Origin',(88.011,65.6896,12.066));
#82851=CARTESIAN_POINT('Origin',(87.3029313066783,68.5948,15.1602538301726));
#82852=CARTESIAN_POINT('',(87.4677738224661,65.6896,14.8843245661282));
#82853=CARTESIAN_POINT('',(87.4677738224661,65.0896,14.8843245661282));
#82854=CARTESIAN_POINT('',(87.5334327817804,65.6896,14.7744182823342));
#82855=CARTESIAN_POINT('',(87.3029313066783,65.6896,15.1602538301726));
#82856=CARTESIAN_POINT('',(87.5334327817804,68.5948,14.7744182823342));
#82857=CARTESIAN_POINT('Origin',(87.5334327817804,68.5948,14.7744182823342));
#82858=CARTESIAN_POINT('',(87.5575418584009,65.6896,14.9001530928687));
#82859=CARTESIAN_POINT('',(87.5575418584009,65.0896,14.9001530928687));
#82860=CARTESIAN_POINT('',(87.5334327817804,65.6896,14.7744182823342));
#82861=CARTESIAN_POINT('Origin',(87.4969666644703,65.6896,14.9812279104668));
#82862=CARTESIAN_POINT('Origin',(88.011,65.6896,12.066));
#82863=CARTESIAN_POINT('Origin',(87.851,68.5948,15.2362));
#82864=CARTESIAN_POINT('',(87.9654235737076,65.6896,14.9358381190176));
#82865=CARTESIAN_POINT('',(87.9654235737076,65.0896,14.9358381190176));
#82866=CARTESIAN_POINT('',(88.011,65.6896,14.8162));
#82867=CARTESIAN_POINT('',(87.851,65.6896,15.2362));
#82868=CARTESIAN_POINT('',(88.011,68.5948,14.8162));
#82869=CARTESIAN_POINT('Origin',(88.011,68.5948,14.8162));
#82870=CARTESIAN_POINT('',(88.0565764262924,65.6896,14.9358381190176));
#82871=CARTESIAN_POINT('',(88.0565764262924,65.0896,14.9358381190176));
#82872=CARTESIAN_POINT('',(88.011,65.6896,14.8162));
#82873=CARTESIAN_POINT('Origin',(88.011,65.6896,15.0262));
#82874=CARTESIAN_POINT('Origin',(88.011,65.6896,12.066));
#82875=CARTESIAN_POINT('Origin',(88.4039302123577,68.5948,15.215821247026));
#82876=CARTESIAN_POINT('',(88.4644581415992,65.6896,14.9001530928687));
#82877=CARTESIAN_POINT('',(88.4644581415992,65.0896,14.9001530928687));
#82878=CARTESIAN_POINT('',(88.4885672182196,65.6896,14.7744182823342));
#82879=CARTESIAN_POINT('',(88.4039302123577,65.6896,15.215821247026));
#82880=CARTESIAN_POINT('',(88.4885672182196,68.5948,14.7744182823342));
#82881=CARTESIAN_POINT('Origin',(88.4885672182196,68.5948,14.7744182823342));
#82882=CARTESIAN_POINT('',(88.5542261775338,65.6896,14.8843245661282));
#82883=CARTESIAN_POINT('',(88.5542261775338,65.0896,14.8843245661282));
#82884=CARTESIAN_POINT('',(88.4885672182196,65.6896,14.7744182823342));
#82885=CARTESIAN_POINT('Origin',(88.5250333355296,65.6896,14.9812279104668));
#82886=CARTESIAN_POINT('Origin',(88.011,65.6896,12.066));
#82887=CARTESIAN_POINT('Origin',(88.9449214390453,68.5948,15.0997367693476));
#82888=CARTESIAN_POINT('',(88.9497146133191,65.6896,14.7783537591437));
#82889=CARTESIAN_POINT('',(88.9497146133191,65.0896,14.7783537591437));
#82890=CARTESIAN_POINT('',(88.9516237981743,65.6896,14.6503426456854));
#82891=CARTESIAN_POINT('',(88.9449214390453,65.6896,15.0997367693476));
#82892=CARTESIAN_POINT('',(88.9516237981743,68.5948,14.6503426456854));
#82893=CARTESIAN_POINT('Origin',(88.9516237981743,68.5948,14.6503426456854));
#82894=CARTESIAN_POINT('',(89.0353702762567,65.6896,14.7471776474381));
#82895=CARTESIAN_POINT('',(89.0353702762567,65.0896,14.7471776474381));
#82896=CARTESIAN_POINT('',(88.9516237981743,65.6896,14.6503426456854));
#82897=CARTESIAN_POINT('Origin',(89.0234480282727,65.6896,14.8476780960504));
#82898=CARTESIAN_POINT('Origin',(88.011,65.6896,12.066));
#82899=CARTESIAN_POINT('Origin',(89.4575359353945,68.5948,14.8914737350774));
#82900=CARTESIAN_POINT('',(89.4064487165259,65.6896,14.5741409289644));
#82901=CARTESIAN_POINT('',(89.4064487165259,65.0896,14.5741409289644));
#82902=CARTESIAN_POINT('',(89.3861,65.6896,14.447743065488));
#82903=CARTESIAN_POINT('',(89.4575359353945,65.6896,14.8914737350774));
#82904=CARTESIAN_POINT('',(89.3861,68.5948,14.447743065488));
#82905=CARTESIAN_POINT('Origin',(89.3861,68.5948,14.447743065488));
#82906=CARTESIAN_POINT('',(89.4853894024917,65.6896,14.528564502672));
#82907=CARTESIAN_POINT('',(89.4853894024917,65.0896,14.528564502672));
#82908=CARTESIAN_POINT('',(89.3861,65.6896,14.447743065488));
#82909=CARTESIAN_POINT('Origin',(89.4911,65.6896,14.6296084002827));
#82910=CARTESIAN_POINT('Origin',(88.011,65.6896,12.066));
#82911=CARTESIAN_POINT('Origin',(89.9261981693292,68.5948,14.5973601111256));
#82912=CARTESIAN_POINT('',(89.8207828166121,65.6896,14.293719505839));
#82913=CARTESIAN_POINT('',(89.8207828166121,65.0896,14.293719505839));
#82914=CARTESIAN_POINT('',(89.7787944841599,65.6896,14.1727754274658));
#82915=CARTESIAN_POINT('',(89.9261981693292,65.6896,14.5973601111256));
#82916=CARTESIAN_POINT('',(89.7787944841599,68.5948,14.1727754274658));
#82917=CARTESIAN_POINT('Origin',(89.7787944841599,68.5948,14.1727754274658));
#82918=CARTESIAN_POINT('',(89.8906099528091,65.6896,14.2351275816099));
#82919=CARTESIAN_POINT('',(89.8906099528091,65.0896,14.2351275816099));
#82920=CARTESIAN_POINT('',(89.7787944841599,65.6896,14.1727754274658));
#82921=CARTESIAN_POINT('Origin',(89.9137798821941,65.6896,14.3336447605208));
#82922=CARTESIAN_POINT('Origin',(88.011,65.6896,12.066));
#82923=CARTESIAN_POINT('Origin',(90.3366680760259,68.5948,14.2263323911273));
#82924=CARTESIAN_POINT('',(90.1801275816099,65.6896,13.9456099528092));
#82925=CARTESIAN_POINT('',(90.1801275816099,65.0896,13.9456099528092));
#82926=CARTESIAN_POINT('',(90.1177754274658,65.6896,13.8337944841599));
#82927=CARTESIAN_POINT('',(90.3366680760259,65.6896,14.2263323911273));
#82928=CARTESIAN_POINT('',(90.1177754274658,68.5948,13.8337944841599));
#82929=CARTESIAN_POINT('Origin',(90.1177754274658,68.5948,13.8337944841599));
#82930=CARTESIAN_POINT('',(90.238719505839,65.6896,13.8757828166121));
#82931=CARTESIAN_POINT('',(90.238719505839,65.0896,13.8757828166121));
#82932=CARTESIAN_POINT('',(90.1177754274658,65.6896,13.8337944841599));
#82933=CARTESIAN_POINT('Origin',(90.2786447605208,65.6896,13.9687798821941));
#82934=CARTESIAN_POINT('Origin',(88.011,65.6896,12.066));
#82935=CARTESIAN_POINT('Origin',(90.6764737350774,68.5948,13.7896640646055));
#82936=CARTESIAN_POINT('',(90.473564502672,65.6896,13.5403894024917));
#82937=CARTESIAN_POINT('',(90.473564502672,65.0896,13.5403894024917));
#82938=CARTESIAN_POINT('',(90.392743065488,65.6896,13.4411));
#82939=CARTESIAN_POINT('',(90.6764737350774,65.6896,13.7896640646055));
#82940=CARTESIAN_POINT('',(90.392743065488,68.5948,13.4411));
#82941=CARTESIAN_POINT('Origin',(90.392743065488,68.5948,13.4411));
#82942=CARTESIAN_POINT('',(90.5191409289644,65.6896,13.4614487165259));
#82943=CARTESIAN_POINT('',(90.5191409289644,65.0896,13.4614487165259));
#82944=CARTESIAN_POINT('',(90.392743065488,65.6896,13.4411));
#82945=CARTESIAN_POINT('Origin',(90.5746084002827,65.6896,13.5461));
#82946=CARTESIAN_POINT('Origin',(88.011,65.6896,12.066));
#82947=CARTESIAN_POINT('Origin',(90.9352903234834,68.5948,13.3006230776968));
#82948=CARTESIAN_POINT('',(90.6921776474381,65.6896,13.0903702762567));
#82949=CARTESIAN_POINT('',(90.6921776474381,65.0896,13.0903702762567));
#82950=CARTESIAN_POINT('',(90.5953426456854,65.6896,13.0066237981743));
#82951=CARTESIAN_POINT('',(90.9352903234834,65.6896,13.3006230776968));
#82952=CARTESIAN_POINT('',(90.5953426456854,68.5948,13.0066237981743));
#82953=CARTESIAN_POINT('Origin',(90.5953426456854,68.5948,13.0066237981743));
#82954=CARTESIAN_POINT('',(90.7233537591437,65.6896,13.0047146133191));
#82955=CARTESIAN_POINT('',(90.7233537591437,65.0896,13.0047146133191));
#82956=CARTESIAN_POINT('',(90.5953426456854,65.6896,13.0066237981743));
#82957=CARTESIAN_POINT('Origin',(90.7926780960505,65.6896,13.0784480282726));
#82958=CARTESIAN_POINT('Origin',(88.011,65.6896,12.066));
#82959=CARTESIAN_POINT('Origin',(91.1052538301726,68.5948,12.7740686933217));
#82960=CARTESIAN_POINT('',(90.8293245661282,65.6896,12.6092261775338));
#82961=CARTESIAN_POINT('',(90.8293245661282,65.0896,12.6092261775338));
#82962=CARTESIAN_POINT('',(90.7194182823342,65.6896,12.5435672182196));
#82963=CARTESIAN_POINT('',(91.1052538301726,65.6896,12.7740686933217));
#82964=CARTESIAN_POINT('',(90.7194182823342,68.5948,12.5435672182196));
#82965=CARTESIAN_POINT('Origin',(90.7194182823342,68.5948,12.5435672182196));
#82966=CARTESIAN_POINT('',(90.8451530928687,65.6896,12.5194581415991));
#82967=CARTESIAN_POINT('',(90.8451530928687,65.0896,12.5194581415991));
#82968=CARTESIAN_POINT('',(90.7194182823342,65.6896,12.5435672182196));
#82969=CARTESIAN_POINT('Origin',(90.9262279104668,65.6896,12.5800333355296));
#82970=CARTESIAN_POINT('Origin',(88.011,65.6896,12.066));
#82971=CARTESIAN_POINT('Origin',(91.1812,68.5948,12.226));
#82972=CARTESIAN_POINT('',(90.8808381190176,65.6896,12.1115764262924));
#82973=CARTESIAN_POINT('',(90.8808381190176,65.0896,12.1115764262924));
#82974=CARTESIAN_POINT('',(90.7612,65.6896,12.066));
#82975=CARTESIAN_POINT('',(91.1812,65.6896,12.226));
#82976=CARTESIAN_POINT('',(90.7612,68.5948,12.066));
#82977=CARTESIAN_POINT('Origin',(90.7612,68.5948,12.066));
#82978=CARTESIAN_POINT('',(90.8808381190176,65.6896,12.0204235737076));
#82979=CARTESIAN_POINT('',(90.8808381190176,65.0896,12.0204235737076));
#82980=CARTESIAN_POINT('',(90.7612,65.6896,12.066));
#82981=CARTESIAN_POINT('Origin',(90.9712,65.6896,12.066));
#82982=CARTESIAN_POINT('Origin',(88.011,65.6896,12.066));
#82983=CARTESIAN_POINT('Origin',(88.011,65.0896,12.066));
#82984=CARTESIAN_POINT('',(85.1408,65.0896,12.066));
#82985=CARTESIAN_POINT('Origin',(88.011,68.5948,12.066));
#82986=CARTESIAN_POINT('',(86.4070487834076,68.5948,12.066));
#82987=CARTESIAN_POINT('',(87.2090243917038,68.5948,10.6769375));
#82988=CARTESIAN_POINT('',(86.6075426854816,68.5948,11.718734375));
#82989=CARTESIAN_POINT('',(88.8129756082962,68.5948,10.6769375));
#82990=CARTESIAN_POINT('',(87.6100121958519,68.5948,10.6769375));
#82991=CARTESIAN_POINT('',(89.6149512165924,68.5948,12.066));
#82992=CARTESIAN_POINT('',(89.0134695103703,68.5948,11.024203125));
#82993=CARTESIAN_POINT('',(88.8129756082962,68.5948,13.4550625));
#82994=CARTESIAN_POINT('',(89.4144573145184,68.5948,12.413265625));
#82995=CARTESIAN_POINT('',(87.2090243917038,68.5948,13.4550625));
#82996=CARTESIAN_POINT('',(88.4119878041481,68.5948,13.4550625));
#82997=CARTESIAN_POINT('',(87.0085304896297,68.5948,13.107796875));
#82998=CARTESIAN_POINT('Origin',(89.6149512165924,66.7948,12.066));
#82999=CARTESIAN_POINT('',(86.4070487834076,66.7948,12.066));
#83000=CARTESIAN_POINT('',(87.2090243917038,66.7948,10.6769375));
#83001=CARTESIAN_POINT('',(86.4070487834076,66.7948,12.066));
#83002=CARTESIAN_POINT('Origin',(88.011,66.7948,12.066));
#83003=CARTESIAN_POINT('Origin',(89.6149512165924,66.7948,12.066));
#83004=CARTESIAN_POINT('',(88.8129756082962,66.7948,10.6769375));
#83005=CARTESIAN_POINT('',(87.2090243917038,66.7948,10.6769375));
#83006=CARTESIAN_POINT('Origin',(88.011,66.7948,12.066));
#83007=CARTESIAN_POINT('Origin',(89.6149512165924,66.7948,12.066));
#83008=CARTESIAN_POINT('',(89.6149512165924,66.7948,12.066));
#83009=CARTESIAN_POINT('',(88.8129756082962,66.7948,10.6769375));
#83010=CARTESIAN_POINT('Origin',(88.011,66.7948,12.066));
#83011=CARTESIAN_POINT('Origin',(89.6149512165924,66.7948,12.066));
#83012=CARTESIAN_POINT('',(88.8129756082962,66.7948,13.4550625));
#83013=CARTESIAN_POINT('',(89.6149512165924,66.7948,12.066));
#83014=CARTESIAN_POINT('Origin',(88.011,66.7948,12.066));
#83015=CARTESIAN_POINT('Origin',(89.6149512165924,66.7948,12.066));
#83016=CARTESIAN_POINT('',(87.2090243917038,66.7948,13.4550625));
#83017=CARTESIAN_POINT('',(88.8129756082962,66.7948,13.4550625));
#83018=CARTESIAN_POINT('Origin',(88.011,66.7948,12.066));
#83019=CARTESIAN_POINT('Origin',(89.6149512165924,66.7948,12.066));
#83020=CARTESIAN_POINT('',(87.2090243917038,66.7948,13.4550625));
#83021=CARTESIAN_POINT('Origin',(88.011,66.7948,12.066));
#83022=CARTESIAN_POINT('Origin',(88.011,66.7948,12.066));
#83023=CARTESIAN_POINT('',(88.011,65.8310488791083,12.066));
#83024=CARTESIAN_POINT('',(86.4070487834076,66.7948,12.066));
#83025=CARTESIAN_POINT('Origin',(86.4070487834076,68.5948,12.066));
#83026=CARTESIAN_POINT('',(86.4070487834076,68.5948,12.066));
#83027=CARTESIAN_POINT('',(87.2090243917038,68.5948,10.6769375));
#83028=CARTESIAN_POINT('Origin',(87.2090243917038,68.5948,13.4550625));
#83029=CARTESIAN_POINT('',(87.2090243917038,68.5948,13.4550625));
#83030=CARTESIAN_POINT('Origin',(88.8129756082962,68.5948,13.4550625));
#83031=CARTESIAN_POINT('',(88.8129756082962,68.5948,13.4550625));
#83032=CARTESIAN_POINT('Origin',(89.6149512165924,68.5948,12.066));
#83033=CARTESIAN_POINT('',(89.6149512165924,68.5948,12.066));
#83034=CARTESIAN_POINT('Origin',(88.8129756082962,68.5948,10.6769375));
#83035=CARTESIAN_POINT('',(88.8129756082962,68.5948,10.6769375));
#83036=CARTESIAN_POINT('Origin',(87.2090243917038,68.5948,10.6769375));
#83200=UNCERTAINTY_MEASURE_WITH_UNIT(LENGTH_MEASURE(0.01),#83220,
'DISTANCE_ACCURACY_VALUE',
'Maximum model space distance between geometric entities at asserted c
onnectivities');
#83203=UNCERTAINTY_MEASURE_WITH_UNIT(LENGTH_MEASURE(0.01),#83220,
'DISTANCE_ACCURACY_VALUE',
'Maximum model space distance between geometric entities at asserted c
onnectivities');
#83216=(
GEOMETRIC_REPRESENTATION_CONTEXT(3)
GLOBAL_UNCERTAINTY_ASSIGNED_CONTEXT((#83200))
GLOBAL_UNIT_ASSIGNED_CONTEXT((#83220,#83222,#83223))
REPRESENTATION_CONTEXT('','3D')
);
#83219=(
GEOMETRIC_REPRESENTATION_CONTEXT(3)
GLOBAL_UNCERTAINTY_ASSIGNED_CONTEXT((#83203))
GLOBAL_UNIT_ASSIGNED_CONTEXT((#83220,#83222,#83223))
REPRESENTATION_CONTEXT('','3D')
);
#83220=(
LENGTH_UNIT()
NAMED_UNIT(*)
SI_UNIT(.MILLI.,.METRE.)
);
#83222=(
NAMED_UNIT(*)
PLANE_ANGLE_UNIT()
SI_UNIT($,.RADIAN.)
);
#83223=(
NAMED_UNIT(*)
SI_UNIT($,.STERADIAN.)
SOLID_ANGLE_UNIT()
);
#83236=SHAPE_DEFINITION_REPRESENTATION(#83251,#83311);
#83251=PRODUCT_DEFINITION_SHAPE('',$,#83327);
#83311=SHAPE_REPRESENTATION('',(#28927),#83216);
#83314=PRODUCT_DEFINITION_CONTEXT('part definition',#83361,'design');
#83327=PRODUCT_DEFINITION('ASME B18.3 SHCS 6-32 UNC x 0.625',
'ASME B18.3 SHCS 6-32 UNC x 0.625',#83342,#83314);
#83342=PRODUCT_DEFINITION_FORMATION('',$,#83375);
#83361=APPLICATION_CONTEXT(
'Core Data for Automotive Mechanical Design Process');
#83362=PRODUCT_CONTEXT('part definition',#83361,'mechanical');
#83375=PRODUCT('ASME B18.3 SHCS 6-32 UNC x 0.625',
'ASME B18.3 SHCS 6-32 UNC x 0.625',$,(#83362));
#83390=PRESENTATION_STYLE_ASSIGNMENT((#83405));
#83405=SURFACE_STYLE_USAGE(.BOTH.,#83420);
#83420=SURFACE_SIDE_STYLE('',(#83435));
#83435=SURFACE_STYLE_FILL_AREA(#83450);
#83450=FILL_AREA_STYLE('Opaque(197,202,208)',(#83465));
#83465=FILL_AREA_STYLE_COLOUR('Opaque(197,202,208)',#83480);
#83480=COLOUR_RGB('Opaque(197,202,208)', 0.09019608, 0.27058824, 0.51372549);
ENDSEC;
END-ISO-10303-21;
